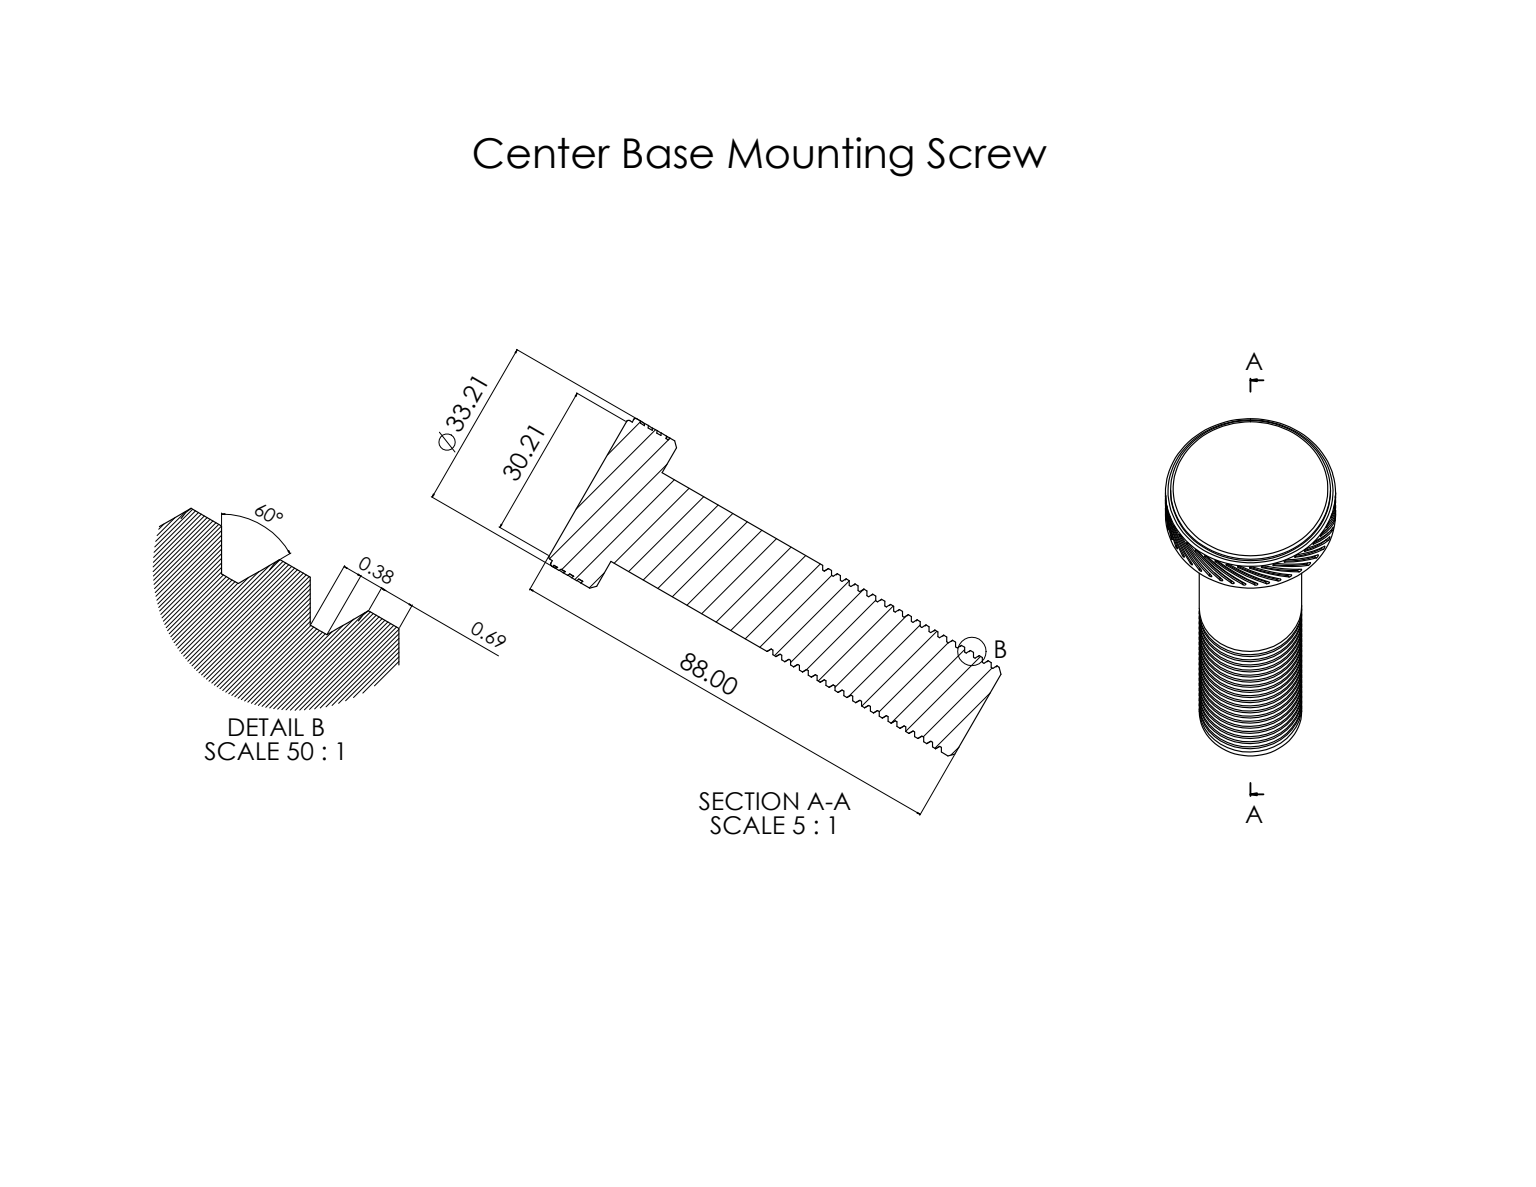
ISO-10303-21;
HEADER;
FILE_DESCRIPTION (('STEP AP214'),
    '1' );
FILE_NAME ('Center Base Mounting Screw.step',
    '2026-10-24T22:31:37',
    ( '' ),
    ( '' ),
    'SwSTEP 2.0',
    'SolidWorks 2025',
    '' );
FILE_SCHEMA (( 'AUTOMOTIVE_DESIGN' ));
ENDSEC;

DATA;
#1=CARTESIAN_POINT ( 'NONE',  ( 23.65144817020273749, 15.78380873178787347, -6.180339887498949025 ) ) ;
#3=DIRECTION ( 'NONE',  ( 0.6270036013472524150, 0.3336146661356817478, 0.7039657224870777830 ) ) ;
#10=CARTESIAN_POINT ( 'NONE',  ( 33.33147356615550194, 41.01751292744059896, 6.180339887498949913 ) ) ;
#11=CARTESIAN_POINT ( 'NONE',  ( 35.05240415091495976, 28.43677371833803846, -10.00000000000000355 ) ) ;
#13=CARTESIAN_POINT ( 'NONE',  ( 72.98662891910291250, 70.81012252529507123, 7.400885746516181030 ) ) ;
#14=CARTESIAN_POINT ( 'NONE',  ( 67.19710446998851694, 67.37600790391256567, -7.293204404656055573 ) ) ;
#18=CARTESIAN_POINT ( 'NONE',  ( 80.56168512721397690, 49.66943426028002762, 14.25699872614796249 ) ) ;
#25=CARTESIAN_POINT ( 'NONE',  ( 78.90549422596571105, 46.47045305960070039, 12.99985401326298984 ) ) ;
#28=CARTESIAN_POINT ( 'NONE',  ( 21.21387930172907588, 35.18080186712593616, 3.090169943749475401 ) ) ;
#37=CARTESIAN_POINT ( 'NONE',  ( 67.11298872355467893, 67.73948000908561085, -6.511686963657441929 ) ) ;
#38=CARTESIAN_POINT ( 'NONE',  ( 73.03670947328784280, 70.42367050102286896, -8.076464510798354368 ) ) ;
#40=CARTESIAN_POINT ( 'NONE',  ( 81.58428055322238492, 41.63658381244528073, 5.723166745212680873 ) ) ;
#45=CARTESIAN_POINT ( 'NONE',  ( 25.22600817569196963, 38.65659080271452552, -1.878358725466461243E-16 ) ) ;
#47=CARTESIAN_POINT ( 'NONE',  ( 87.34642337659644795, 43.20430561321286689, -4.696387144280492735E-07 ) ) ;
#53=CARTESIAN_POINT ( 'NONE',  ( 45.00959873851216031, 26.39040679176986970, 1.333680081654574804E-15 ) ) ;
#54=CARTESIAN_POINT ( 'NONE',  ( 82.57385212973971989, 41.04541115053230982, -1.138833187496899768 ) ) ;
#56=CARTESIAN_POINT ( 'NONE',  ( 66.42592059512334401, 67.89756533557547868, 6.603446877074300225 ) ) ;
#65=CARTESIAN_POINT ( 'NONE',  ( 15.07770630580378501, 30.74646525600389424, 2.839279412974139660 ) ) ;
#67=CARTESIAN_POINT ( 'NONE',  ( 71.88182444303143370, 59.07920979518379312, 15.37605134340125090 ) ) ;
#70=CARTESIAN_POINT ( 'NONE',  ( 4.275827057391709651, 20.65586893147753500, -7.433330006724137462 ) ) ;
#71=CARTESIAN_POINT ( 'NONE',  ( 75.23698744953621542, 53.54332355648684683, -16.05067780448434078 ) ) ;
#72=CARTESIAN_POINT ( 'NONE',  ( 87.14941533941508567, 43.54552546780055877, 0.3078308432578384934 ) ) ;
#77=CARTESIAN_POINT ( 'NONE',  ( 71.49780929996677514, 71.35361720523084728, -4.112299254006656746 ) ) ;
#78=CARTESIAN_POINT ( 'NONE',  ( 76.99791550217098290, 63.80129665876799550, 14.94914524525639266 ) ) ;
#80=ORIENTED_EDGE ( 'NONE', *, *, #23057, .F. ) ;
#86=CARTESIAN_POINT ( 'NONE',  ( 80.05322980421331636, 57.68292478952277946, 16.60179730502024853 ) ) ;
#87=CARTESIAN_POINT ( 'NONE',  ( 66.50947442187053582, 69.16636744153423422, -3.269992574601006119 ) ) ;
#95=ORIENTED_EDGE ( 'NONE', *, *, #9124, .F. ) ;
#98=CARTESIAN_POINT ( 'NONE',  ( 78.41477381124543911, 47.32040575020751305, -14.22103711521623559 ) ) ;
#103=CARTESIAN_POINT ( 'NONE',  ( 83.68415435101742617, 52.28560849428279766, 14.71934805883068975 ) ) ;
#115=CARTESIAN_POINT ( 'NONE',  ( 70.01037705890988150, 67.69997893903554598, 9.246301564518420335 ) ) ;
#119=CARTESIAN_POINT ( 'NONE',  ( 78.58712697892576671, 47.46528512289431490, 14.24466080792137923 ) ) ;
#121=VERTEX_POINT ( 'NONE', #65704 ) ;
#123=CARTESIAN_POINT ( 'NONE',  ( 70.63585127456710211, 66.25873673130102759, 11.15280021666221266 ) ) ;
#124=CARTESIAN_POINT ( 'NONE',  ( 87.74659634842467426, 45.27479573043824246, -7.097702524348068920 ) ) ;
#125=CARTESIAN_POINT ( 'NONE',  ( 79.09597600355056102, 46.01113921700726195, 13.22013416637107674 ) ) ;
#127=CARTESIAN_POINT ( 'NONE',  ( 80.54938030787035075, 54.28115242235315208, -16.20956398890630368 ) ) ;
#129=CARTESIAN_POINT ( 'NONE',  ( 69.87848390701969947, 64.97149032717396722, -11.85179110244203926 ) ) ;
#132=CARTESIAN_POINT ( 'NONE',  ( 72.22030775602182473, 71.51030902015637025, 5.034539909834746751 ) ) ;
#136=CARTESIAN_POINT ( 'NONE',  ( 67.15772368909350121, 67.74692886573922124, -6.548511843863573212 ) ) ;
#140=CARTESIAN_POINT ( 'NONE',  ( 85.75095722755503402, 48.73152497522561788, -11.95392408748539381 ) ) ;
#142=CARTESIAN_POINT ( 'NONE',  ( 70.62071346605948463, 62.04983420565448426, 13.98037766351442457 ) ) ;
#146=CARTESIAN_POINT ( 'NONE',  ( 82.03168081927420019, 41.83908362533459524, -5.586039627916139949 ) ) ;
#150=ORIENTED_EDGE ( 'NONE', *, *, #60128, .F. ) ;
#155=CARTESIAN_POINT ( 'NONE',  ( 17.22757050757671493, 15.11029122506293554, -8.090169943749478065 ) ) ;
#158=DIRECTION ( 'NONE',  ( -0.4755282581475737680, 0.8236391035463299648, -0.3090169943749573878 ) ) ;
#163=CARTESIAN_POINT ( 'NONE',  ( 72.59198933040177337, 57.21847231819964463, 16.35083922987430327 ) ) ;
#165=CARTESIAN_POINT ( 'NONE',  ( 66.48182541455327055, 68.83268692814938561, -4.376997617227660342 ) ) ;
#172=CARTESIAN_POINT ( 'NONE',  ( 30.35763184873497877, 26.03085787977764198, 9.188101187500006262 ) ) ;
#174=EDGE_CURVE ( 'NONE', #25263, #42575, #10857, .T. ) ;
#177=CARTESIAN_POINT ( 'NONE',  ( 68.73278530260755304, 67.96956153877513884, 8.699763636338595063 ) ) ;
#178=CARTESIAN_POINT ( 'NONE',  ( 66.40112479374357690, 68.71345452083818373, 2.354737509933789941 ) ) ;
#183=CARTESIAN_POINT ( 'NONE',  ( 16.06339478488542127, 14.98920272979925272, 7.433330006724137462 ) ) ;
#184=VERTEX_POINT ( 'NONE', #13527 ) ;
#193=ORIENTED_EDGE ( 'NONE', *, *, #79471, .F. ) ;
#196=CARTESIAN_POINT ( 'NONE',  ( 72.70339454587075068, 70.80219159916109106, 7.145408444353458677 ) ) ;
#204=CARTESIAN_POINT ( 'NONE',  ( 69.57540738265171854, 62.56329180587877659, 13.35759117457639533 ) ) ;
#208=CARTESIAN_POINT ( 'NONE',  ( 81.41173721124711449, 42.57291668893481784, -7.675381966840256531 ) ) ;
#218=EDGE_CURVE ( 'NONE', #7931, #29087, #34574, .T. ) ;
#220=CARTESIAN_POINT ( 'NONE',  ( 90.04477061917849312, 44.76220097505219542, 0.000000000000000000 ) ) ;
#224=CARTESIAN_POINT ( 'NONE',  ( 82.66575685400569284, 54.08976349579732812, -15.88644314918171929 ) ) ;
#227=CARTESIAN_POINT ( 'NONE',  ( 11.61360469066603507, 28.74646525600389069, 2.839279412974139660 ) ) ;
#229=CARTESIAN_POINT ( 'NONE',  ( 85.68485941944550177, 48.66523437743575187, 11.91861461389294163 ) ) ;
#238=CARTESIAN_POINT ( 'NONE',  ( 80.58987807051757102, 46.20205379198799989, -12.14270396900382742 ) ) ;
#248=B_SPLINE_CURVE_WITH_KNOTS ( 'NONE', 3,
 ( #65678, #27199, #81432, #4384, #59558, #20106, #51479, #97613, #89544, #13499, #59053, #74319, #21105, #43869, #50975, #81927, #67174, #28181, #12503, #36275, #83920, #90535, #6867, #75301, #21584, #82446, #82923, #43372, #90024, #4902, #51985, #5389, #13010, #98098, #74811, #52469, #20596, #35785, #67678, #29191, #68662, #60058, #44369, #28675, #66678, #13984 ),
 .UNSPECIFIED., .F., .F.,
 ( 4, 1, 1, 1, 2, 2, 1, 1, 1, 2, 2, 1, 1, 2, 2, 1, 1, 2, 2, 1, 1, 2, 2, 1, 2, 2, 1, 2, 2, 4 ),
 ( 0.000000000000000000, 0.06249999999999578115, 0.09374999999999281131, 0.1093749999999927697, 0.1171874999999917982, 0.1249999999999908268, 0.1874999999999810985, 0.2187499999999757694, 0.2343749999999731048, 0.2421874999999721889, 0.2499999999999712730, 0.3124999999999665823, 0.3437499999999636957, 0.3593749999999625855, 0.3749999999999614753, 0.4374999999999584777, 0.4687499999999559241, 0.4843749999999560907, 0.4999999999999562572, 0.5624999999999540368, 0.5937499999999539257, 0.6093749999999549249, 0.6249999999999558131, 0.6874999999999583666, 0.7187499999999606981, 0.7499999999999630296, 0.8124999999999696909, 0.8437499999999743538, 0.8749999999999790168, 1.000000000000000000 ),
 .UNSPECIFIED. ) ;
#258=CARTESIAN_POINT ( 'NONE',  ( 84.80990162342361316, 46.15601649245774496, -9.987538208358218483 ) ) ;
#263=CARTESIAN_POINT ( 'NONE',  ( 74.05204724713870235, 68.33764315531155376, -11.67956189741113349 ) ) ;
#277=DIRECTION ( 'NONE',  ( -0.8660254037844377084, -0.5000000000000015543, -0.000000000000000000 ) ) ;
#278=CARTESIAN_POINT ( 'NONE',  ( 69.28790557221618940, 69.26308972205728764, 6.048929301421852145 ) ) ;
#285=CARTESIAN_POINT ( 'NONE',  ( 17.19404571121151548, 18.43085787977762280, -9.188101187500008038 ) ) ;
#294=CARTESIAN_POINT ( 'NONE',  ( 43.17480782474465428, 33.43085787977766898, -9.188101187500008038 ) ) ;
#296=CARTESIAN_POINT ( 'NONE',  ( 81.30975366074838462, 56.24313983998633404, -16.44754541364716971 ) ) ;
#299=CARTESIAN_POINT ( 'NONE',  ( 33.38390286057418166, 24.98920272979928470, 7.433330006724137462 ) ) ;
#300=DIRECTION ( 'NONE',  ( 0.4145187862775202015, -0.7179675985244525771, -0.5591929034707450175 ) ) ;
#301=CARTESIAN_POINT ( 'NONE',  ( 81.38004395914478550, 48.63429429711172247, 14.01118663915790030 ) ) ;
#307=CARTESIAN_POINT ( 'NONE',  ( 84.83590989842353736, 50.19589791021755332, -13.76099895038702847 ) ) ;
#308=CARTESIAN_POINT ( 'NONE',  ( 75.63268008801900066, 65.14737934564519151, -14.41129995628930516 ) ) ;
#310=CARTESIAN_POINT ( 'NONE',  ( 73.99515186948657686, 54.97541550358009488, -16.60506967685200408 ) ) ;
#313=CARTESIAN_POINT ( 'NONE',  ( 73.43248428410468875, 69.89844921070914552, 9.717079046730820124 ) ) ;
#314=CARTESIAN_POINT ( 'NONE',  ( 38.69312636016019269, 30.84335787977765619, 9.188101187500006262 ) ) ;
#315=VERTEX_POINT ( 'NONE', #76800 ) ;
#319=ORIENTED_EDGE ( 'NONE', *, *, #9183, .T. ) ;
#320=CARTESIAN_POINT ( 'NONE',  ( 86.52915347386752387, 47.38364953835303339, -10.30352551399626648 ) ) ;
#324=CARTESIAN_POINT ( 'NONE',  ( 41.44395331530407844, 35.87878583063845639, -9.188101187500006262 ) ) ;
#325=CARTESIAN_POINT ( 'NONE',  ( 80.05943320740847469, 44.70013682444275815, 11.13689609985222617 ) ) ;
#329=VERTEX_POINT ( 'NONE', #37789 ) ;
#330=CARTESIAN_POINT ( 'NONE',  ( 81.35074466249913883, 55.80872010294902452, 16.38725056492407361 ) ) ;
#335=DIRECTION ( 'NONE',  ( -0.5000000000000015543, 0.8660254037844378194, 0.000000000000000000 ) ) ;
#336=CARTESIAN_POINT ( 'NONE',  ( 35.42939366167109938, 22.58380873178788306, 6.180339887498953466 ) ) ;
#339=CARTESIAN_POINT ( 'NONE',  ( 82.56576626489119519, 41.03778865018932720, 1.100605105531167416 ) ) ;
#342=EDGE_CURVE ( 'NONE', #62365, #23265, #62078, .T. ) ;
#347=CARTESIAN_POINT ( 'NONE',  ( 70.49910835669693654, 60.86989013130169468, -15.00567599565220434 ) ) ;
#348=CARTESIAN_POINT ( 'NONE',  ( 41.71939737199939202, 29.80170272979930246, 7.433330006724137462 ) ) ;
#351=EDGE_CURVE ( 'NONE', #45858, #78719, #48667, .T. ) ;
#358=CARTESIAN_POINT ( 'NONE',  ( 72.39980299547302423, 63.20348272691148139, 13.94953712136970836 ) ) ;
#361=ORIENTED_EDGE ( 'NONE', *, *, #84758, .T. ) ;
#374=CARTESIAN_POINT ( 'NONE',  ( 70.01283242295177445, 62.80173547756309915, -13.36538303052352816 ) ) ;
#378=CARTESIAN_POINT ( 'NONE',  ( 72.32867159652951727, 65.47220889536410482, 12.56686077310279082 ) ) ;
#385=CARTESIAN_POINT ( 'NONE',  ( 23.13271821863878230, 13.75978393459164195, -1.583844403245362020 ) ) ;
#388=CARTESIAN_POINT ( 'NONE',  ( 82.68215287466908592, 53.55713939286302150, -15.73562046651999502 ) ) ;
#396=CARTESIAN_POINT ( 'NONE',  ( 84.87359499838788679, 50.02211777990267194, -13.22747082306951327 ) ) ;
#398=CARTESIAN_POINT ( 'NONE',  ( 73.56775416758397057, 69.23451306489744184, -10.00871374113025070 ) ) ;
#399=CARTESIAN_POINT ( 'NONE',  ( 75.97293632993350343, 51.42040260576536781, 16.16535879681820731 ) ) ;
#409=CARTESIAN_POINT ( 'NONE',  ( 75.75493378409400691, 65.86437009324525604, -14.07593894684414693 ) ) ;
#410=EDGE_CURVE ( 'NONE', #10093, #75363, #77822, .T. ) ;
#413=CARTESIAN_POINT ( 'NONE',  ( 66.36268096397610350, 69.44190093015801324, 9.875986171954755521E-07 ) ) ;
#415=CARTESIAN_POINT ( 'NONE',  ( 27.04628097738780212, 27.56628583063842086, 9.188101187500006262 ) ) ;
#417=CARTESIAN_POINT ( 'NONE',  ( 81.38192374540615504, 47.39962897157295885, -12.69884445555879360 ) ) ;
#418=CARTESIAN_POINT ( 'NONE',  ( 11.61057445305848823, 22.10171378149917842, 9.188101187500008038 ) ) ;
#420=CARTESIAN_POINT ( 'NONE',  ( 77.30463285345523161, 63.36080703450485174, 15.53535672671000079 ) ) ;
#423=CARTESIAN_POINT ( 'NONE',  ( 67.41248320326423027, 66.37693208286884783, -8.946798147498746800 ) ) ;
#428=CARTESIAN_POINT ( 'NONE',  ( 80.28226457095783530, 55.01127608260450330, -15.95866588083628557 ) ) ;
#434=CARTESIAN_POINT ( 'NONE',  ( 82.50452235219570696, 53.86480448276186905, 15.85105177732747173 ) ) ;
#435=ORIENTED_EDGE ( 'NONE', *, *, #30362, .T. ) ;
#444=CARTESIAN_POINT ( 'NONE',  ( 82.09009853944208146, 44.85671956714123354, 10.87987463625776741 ) ) ;
#447=CARTESIAN_POINT ( 'NONE',  ( 23.73796034364816521, 35.74646525600390845, 2.839279412974139660 ) ) ;
#448=CARTESIAN_POINT ( 'NONE',  ( 79.97518497192163522, 44.56399469350409959, 11.74208085782137267 ) ) ;
#450=CARTESIAN_POINT ( 'NONE',  ( 75.08013308270209052, 67.09339902234967212, -13.09435070823463043 ) ) ;
#452=ORIENTED_EDGE ( 'NONE', *, *, #76491, .T. ) ;
#459=FACE_OUTER_BOUND ( 'NONE', #67397, .T. ) ;
#475=CARTESIAN_POINT ( 'NONE',  ( 67.16327201103491973, 67.73731889023997610, 6.573435314091265802 ) ) ;
#479=CARTESIAN_POINT ( 'NONE',  ( 81.11670802570714045, 56.15934143863493944, 16.10866441373284630 ) ) ;
#486=CARTESIAN_POINT ( 'NONE',  ( 82.41630873631589793, 41.31828431233920895, -3.367117793111288560 ) ) ;
#488=EDGE_LOOP ( 'NONE', ( #46553, #54812, #94039, #23503 ) ) ;
#489=CARTESIAN_POINT ( 'NONE',  ( 76.44840390471171077, 51.64438224287277279, -16.15499642960158155 ) ) ;
#497=CARTESIAN_POINT ( 'NONE',  ( 82.82785115793576836, 43.65967190867092285, -8.128949345812960914 ) ) ;
#500=CARTESIAN_POINT ( 'NONE',  ( 72.42095758685501039, 70.73706075180957953, 7.727740079816340035 ) ) ;
#501=CARTESIAN_POINT ( 'NONE',  ( 69.17735699518412673, 67.42632015883337715, -8.956856073786124028 ) ) ;
#502=ORIENTED_EDGE ( 'NONE', *, *, #85667, .F. ) ;
#508=EDGE_CURVE ( 'NONE', #53392, #59506, #69113, .T. ) ;
#516=FACE_BOUND ( 'NONE', #48775, .T. ) ;
#519=CARTESIAN_POINT ( 'NONE',  ( 32.89180500207565672, 24.15404122711135670, 8.090169943749479842 ) ) ;
#529=CARTESIAN_POINT ( 'NONE',  ( 13.40335115377346753, 31.23654200823201776, 1.583844403245363353 ) ) ;
#530=CARTESIAN_POINT ( 'NONE',  ( 81.82787295522399518, 41.24789425966510947, 5.851439987416612531 ) ) ;
#532=CARTESIAN_POINT ( 'NONE',  ( 22.06360519161784595, 36.23654200823203553, 1.583844403245363353 ) ) ;
#533=CARTESIAN_POINT ( 'NONE',  ( 30.89548221274965556, 26.03677371833803633, 10.00000000000000533 ) ) ;
#534=CARTESIAN_POINT ( 'NONE',  ( 86.35121876318000034, 43.08468197994678661, 0.3078304325362931637 ) ) ;
#538=CARTESIAN_POINT ( 'NONE',  ( 87.18439463908147502, 46.15779724344488244, -8.329569831597547491 ) ) ;
#544=CARTESIAN_POINT ( 'NONE',  ( 72.32117545662791258, 66.44659970230358681, -11.84374507886356831 ) ) ;
#548=CARTESIAN_POINT ( 'NONE',  ( 66.29454943693275482, 69.24199052626691753, -2.144636311159408226 ) ) ;
#552=LINE ( 'NONE', #17762, #100067 ) ;
#557=CARTESIAN_POINT ( 'NONE',  ( 19.25324864145614612, 26.51421378149919761, -9.188101187500004485 ) ) ;
#563=CARTESIAN_POINT ( 'NONE',  ( 7.601631632957885465, 27.49540643055185285, 3.479690158560446702E-15 ) ) ;
#564=DIRECTION ( 'NONE',  ( -0.4996954135095461047, 0.8654978445076770832, -0.03489949670251103753 ) ) ;
#568=CARTESIAN_POINT ( 'NONE',  ( 72.40022343535652283, 71.86297034063233014, -5.456689119915505870 ) ) ;
#571=ORIENTED_EDGE ( 'NONE', *, *, #75290, .T. ) ;
#572=ORIENTED_EDGE ( 'NONE', *, *, #79852, .F. ) ;
#574=CARTESIAN_POINT ( 'NONE',  ( 83.55937078812219454, 42.48588548430609535, -5.103737020810437564 ) ) ;
#577=PLANE ( 'NONE',  #1141 ) ;
#578=CARTESIAN_POINT ( 'NONE',  ( 72.73633344227268083, 57.02636325111804183, -16.39140812357083021 ) ) ;
#579=CARTESIAN_POINT ( 'NONE',  ( 76.64464310018406934, 63.53199411942404851, 15.34601863127964627 ) ) ;
#586=CARTESIAN_POINT ( 'NONE',  ( 26.72152145096863762, 27.37878583063842086, 9.188101187500006262 ) ) ;
#588=CARTESIAN_POINT ( 'NONE',  ( 78.31654463311403447, 47.36115395161638020, -14.27160036167827784 ) ) ;
#593=CARTESIAN_POINT ( 'NONE',  ( 83.35161352719694605, 52.40881748729520240, 14.85180384881482674 ) ) ;
#595=EDGE_LOOP ( 'NONE', ( #20192, #17699, #51168, #51804 ) ) ;
#596=CARTESIAN_POINT ( 'NONE',  ( 86.83016860379825630, 46.47919197584165119, 9.056981041330921300 ) ) ;
#597=CARTESIAN_POINT ( 'NONE',  ( 81.64670023727850889, 42.65128533460878657, -7.584980231169042852 ) ) ;
#601=ORIENTED_EDGE ( 'NONE', *, *, #47729, .T. ) ;
#608=ADVANCED_FACE ( 'NONE', ( #98877 ), #22352, .T. ) ;
#609=CARTESIAN_POINT ( 'NONE',  ( 69.00186724958503248, 65.47144582019447512, 10.96851354096545883 ) ) ;
#611=CARTESIAN_POINT ( 'NONE',  ( 67.43691672556117567, 66.98928061623196584, 9.017019808546432813 ) ) ;
#612=CARTESIAN_POINT ( 'NONE',  ( 70.21952773771840839, 65.49792867059230161, -11.57245437907510244 ) ) ;
#613=CARTESIAN_POINT ( 'NONE',  ( 78.41127520731549794, 47.42400182521100049, 14.27580055608907017 ) ) ;
#617=CARTESIAN_POINT ( 'NONE',  ( 69.93192355902827728, 64.35613849418326993, 12.34049615428977198 ) ) ;
#620=B_SPLINE_CURVE_WITH_KNOTS ( 'NONE', 3,
 ( #66257, #11575, #42433, #82510, #73367, #65740, #96694, #4966, #27759, #58631, #27263, #89605, #41953, #96197, #74384, #34355, #51036, #26758, #35849, #58146, #19678, #72382, #66742, #59118, #90091, #95716, #64767, #20659, #51548, #2992, #33882 ),
 .UNSPECIFIED., .F., .F.,
 ( 4, 3, 3, 3, 3, 3, 3, 3, 3, 3, 4 ),
 ( 0.000000000000000000, 0.1333490885032305451, 0.3007194338854253246, 0.4699862290244986029, 0.5844252810809236198, 0.6686540514502520294, 0.7354980260655306079, 0.8028463152565280536, 0.8633854507756927310, 0.9437142632666988273, 1.000000000000000000 ),
 .UNSPECIFIED. ) ;
#622=CARTESIAN_POINT ( 'NONE',  ( 83.88626965845651284, 51.63168102053428754, -14.39363241527635751 ) ) ;
#626=CARTESIAN_POINT ( 'NONE',  ( 72.54208641595317886, 71.58009272687419866, 5.313622202418648577 ) ) ;
#631=DIRECTION ( 'NONE',  ( -0.2347357813929480952, 0.4065742997269687908, 0.8829475928589233247 ) ) ;
#633=CARTESIAN_POINT ( 'NONE',  ( 83.18659939620825128, 40.82302332894202124, -0.8845490628100145525 ) ) ;
#636=CARTESIAN_POINT ( 'NONE',  ( 85.65412827366334625, 48.89905674914069067, -12.59087409094112253 ) ) ;
#638=DIRECTION ( 'NONE',  ( -0.2347357813929480952, 0.4065742997269687908, 0.8829475928589233247 ) ) ;
#646=CARTESIAN_POINT ( 'NONE',  ( 45.03145032967896100, 28.12755873383629890, -6.180339887498949025 ) ) ;
#649=CARTESIAN_POINT ( 'NONE',  ( 88.00349997577261263, 44.64923112938743088, 4.253506518527973235 ) ) ;
#651=CARTESIAN_POINT ( 'NONE',  ( 10.05297690690921897, 28.73705186507752529, -3.090169943749475845 ) ) ;
#653=CARTESIAN_POINT ( 'NONE',  ( 71.82703346931063493, 59.57451500028311386, -15.72875088550162914 ) ) ;
#658=CARTESIAN_POINT ( 'NONE',  ( 73.05975105895772970, 57.25024586824646633, 15.90232548103993615 ) ) ;
#660=CARTESIAN_POINT ( 'NONE',  ( 10.55946980724658069, 24.83478043621386888, -8.090169943749479842 ) ) ;
#662=AXIS2_PLACEMENT_3D ( 'NONE', #54067, #69781, #39856 ) ;
#667=CARTESIAN_POINT ( 'NONE',  ( 31.05045217176252237, 26.43085787977764767, -9.188101187500008038 ) ) ;
#670=EDGE_CURVE ( 'NONE', #48310, #39764, #20859, .T. ) ;
#675=CARTESIAN_POINT ( 'NONE',  ( 66.15645594251088824, 68.58591844969842555, 2.277906049505277863 ) ) ;
#681=CARTESIAN_POINT ( 'NONE',  ( 12.59929316974766955, 12.98920272979924739, 7.433330006724137462 ) ) ;
#685=CARTESIAN_POINT ( 'NONE',  ( 28.31825578742223115, 28.30066082961423390, -10.00000000000000533 ) ) ;
#692=FACE_OUTER_BOUND ( 'NONE', #1772, .T. ) ;
#693=ORIENTED_EDGE ( 'NONE', *, *, #11844, .T. ) ;
#698=CARTESIAN_POINT ( 'NONE',  ( 79.11723855630624769, 59.11194703662723526, -16.21433712332713739 ) ) ;
#700=CARTESIAN_POINT ( 'NONE',  ( 69.78994883848024244, 62.55969527080727488, 13.43020027970054819 ) ) ;
#708=CARTESIAN_POINT ( 'NONE',  ( 73.41033574890859370, 61.45318865418844467, 14.95304618059455670 ) ) ;
#718=CARTESIAN_POINT ( 'NONE',  ( 73.00396795756827828, 57.62093675928252878, -16.32480838619500219 ) ) ;
#719=CARTESIAN_POINT ( 'NONE',  ( 15.13723537722347778, 17.24335787977762280, -9.188101187500008038 ) ) ;
#722=CARTESIAN_POINT ( 'NONE',  ( 68.45344762042827824, 64.57392882346940155, 12.12708197196866600 ) ) ;
#729=CARTESIAN_POINT ( 'NONE',  ( 82.52967124556970191, 45.91001068904856197, -10.98309457076566886 ) ) ;
#733=DIRECTION ( 'NONE',  ( -0.8660254037844377084, -0.5000000000000014433, -0.000000000000000000 ) ) ;
#740=CARTESIAN_POINT ( 'NONE',  ( 82.39535249337586720, 40.37214158351728344, -0.8705103534316617209 ) ) ;
#743=CARTESIAN_POINT ( 'NONE',  ( 72.53309028193872621, 70.86290320417140265, 7.626211012637800657 ) ) ;
#745=CARTESIAN_POINT ( 'NONE',  ( 75.62238463899576857, 65.35737373615053514, 14.30258955018443956 ) ) ;
#747=ORIENTED_EDGE ( 'NONE', *, *, #72238, .F. ) ;
#749=VERTEX_POINT ( 'NONE', #78569 ) ;
#752=CARTESIAN_POINT ( 'NONE',  ( 85.52120238093419857, 46.04363271907506316, -9.405378037663709279 ) ) ;
#756=CARTESIAN_POINT ( 'NONE',  ( 74.45862791283336435, 68.29041308412308808, -11.43317454991487914 ) ) ;
#762=CARTESIAN_POINT ( 'NONE',  ( 30.11635425815369871, 39.16126292948897714, -6.180339887498951690 ) ) ;
#763=CARTESIAN_POINT ( 'NONE',  ( 80.25178558894602077, 57.14685393251872370, -16.23521980932009612 ) ) ;
#768=ADVANCED_FACE ( 'NONE', ( #79091 ), #73419, .T. ) ;
#774=DIRECTION ( 'NONE',  ( 0.000000000000000000, -0.5247752241694974007, 0.8512408378936325848 ) ) ;
#779=CARTESIAN_POINT ( 'NONE',  ( 10.91775413003093931, 21.70171378149917985, -9.188101187500004485 ) ) ;
#783=CARTESIAN_POINT ( 'NONE',  ( 66.10780414051450293, 68.63670250712272036, 1.777645618418523865 ) ) ;
#790=CARTESIAN_POINT ( 'NONE',  ( 85.94615330653621754, 47.59945275330427705, 10.87303975713271420 ) ) ;
#791=ORIENTED_EDGE ( 'NONE', *, *, #48139, .T. ) ;
#798=CARTESIAN_POINT ( 'NONE',  ( 84.41462708798377435, 43.37824213815624574, 7.154511429969321767 ) ) ;
#801=CARTESIAN_POINT ( 'NONE',  ( 72.40747426417379984, 71.81324781307232286, -5.589457107701495175 ) ) ;
#803=ORIENTED_EDGE ( 'NONE', *, *, #92983, .T. ) ;
#806=CARTESIAN_POINT ( 'NONE',  ( 41.82943821127123840, 26.01110640527295814, 2.839279412974134775 ) ) ;
#813=EDGE_LOOP ( 'NONE', ( #50961, #70079, #41428, #11684 ) ) ;
#814=CARTESIAN_POINT ( 'NONE',  ( 86.28449982416978514, 46.95005333036156969, -10.54182221192813884 ) ) ;
#816=B_SPLINE_CURVE_WITH_KNOTS ( 'NONE', 3,
 ( #20818, #38347, #96847, #7455, #100186, #69257, #36485, #58292, #57789, #43591, #88767, #82657, #28907, #43073, #13216, #19337 ),
 .UNSPECIFIED., .F., .F.,
 ( 4, 1, 2, 2, 2, 1, 2, 2, 4 ),
 ( 0.000000000000000000, 0.1249999999999972522, 0.1874999999999962530, 0.2499999999999952816, 0.4999999999999940048, 0.6249999999999944489, 0.6874999999999946709, 0.7499999999999947820, 1.000000000000000000 ),
 .UNSPECIFIED. ) ;
#819=CARTESIAN_POINT ( 'NONE',  ( 18.33840876668534037, 32.36126292948895866, 6.180339887498949913 ) ) ;
#822=CARTESIAN_POINT ( 'NONE',  ( 81.63517289312954972, 55.69097578121159131, -16.34528168754146904 ) ) ;
#826=VERTEX_POINT ( 'NONE', #48664 ) ;
#827=CARTESIAN_POINT ( 'NONE',  ( 77.13172709529845861, 49.47536214534034826, -14.94599358421776358 ) ) ;
#831=DIRECTION ( 'NONE',  ( -0.8660254037844378194, -0.5000000000000014433, -0.000000000000000000 ) ) ;
#832=CARTESIAN_POINT ( 'NONE',  ( 36.01802474176511026, 21.76426979415091978, 3.090169943749476733 ) ) ;
#833=CARTESIAN_POINT ( 'NONE',  ( 71.17767548612019368, 71.91738291818995776, 3.016136621268855844 ) ) ;
#840=CARTESIAN_POINT ( 'NONE',  ( 70.47294781783818962, 60.89548864084860469, -14.98891872237399348 ) ) ;
#841=CARTESIAN_POINT ( 'NONE',  ( 42.37730965384162829, 25.26216523072498532, -2.296566073217252530E-15 ) ) ;
#844=ADVANCED_FACE ( 'NONE', ( #61833 ), #9674, .T. ) ;
#845=CARTESIAN_POINT ( 'NONE',  ( 20.28716687417668751, 35.21091486745861232, 7.012934429366973338E-14 ) ) ;
#849=EDGE_CURVE ( 'NONE', #75378, #62754, #4045, .T. ) ;
#852=CARTESIAN_POINT ( 'NONE',  ( 71.63285926872011089, 60.29674625202430605, 14.96834098354499965 ) ) ;
#856=CARTESIAN_POINT ( 'NONE',  ( 76.73342198214220389, 54.11205231684652972, -16.50410611215824375 ) ) ;
#866=CYLINDRICAL_SURFACE ( 'NONE', #55855, 10.00000000000001066 ) ;
#883=CARTESIAN_POINT ( 'NONE',  ( 73.85662887421025857, 68.53912330967601463, 10.89787362795912884 ) ) ;
#892=CARTESIAN_POINT ( 'NONE',  ( 78.12422403393351544, 55.30668070268215075, 16.12263249026505108 ) ) ;
#896=B_SPLINE_CURVE_WITH_KNOTS ( 'NONE', 3,
 ( #59007, #89974, #13454, #81389, #49945, #20554, #82879, #57531, #35237, #51432, #12964, #43825, #5343, #36224, #19070, #67128, #59512, #90490, #21063, #37224, #7320, #38712, #91978, #13933, #99050, #14437, #61996, #23008, #75749, #53903, #38199, #68619, #99542, #68122, #14914, #21539, #36721, #5831, #45318, #45802, #69118, #100045, #76726, #23501, #52422, #69618 ),
 .UNSPECIFIED., .F., .F.,
 ( 4, 1, 2, 2, 1, 2, 2, 1, 1, 2, 2, 1, 1, 2, 2, 1, 1, 2, 2, 1, 1, 1, 2, 2, 1, 1, 1, 2, 2, 4 ),
 ( 0.000000000000000000, 0.06249999999999382438, 0.09374999999999200639, 0.1249999999999902023, 0.1874999999999839295, 0.2187499999999821532, 0.2499999999999804046, 0.3124999999999763522, 0.3437499999999758526, 0.3593749999999756306, 0.3749999999999754086, 0.4374999999999745759, 0.4687499999999757971, 0.4843749999999780731, 0.4999999999999803491, 0.5624999999999793499, 0.5937499999999791278, 0.6093749999999773515, 0.6249999999999755751, 0.6874999999999715783, 0.7187499999999709122, 0.7343749999999705791, 0.7421874999999703570, 0.7499999999999701350, 0.8124999999999732436, 0.8437499999999734657, 0.8593749999999736877, 0.8671874999999749090, 0.8749999999999761302, 1.000000000000000000 ),
 .UNSPECIFIED. ) ;
#897=CARTESIAN_POINT ( 'NONE',  ( 76.39060622948801438, 51.12702130622679420, 16.04935315526039474 ) ) ;
#904=CARTESIAN_POINT ( 'NONE',  ( 72.71381692756899895, 57.00322135356037023, -15.91178980316282043 ) ) ;
#905=EDGE_CURVE ( 'NONE', #18632, #67404, #6039, .T. ) ;
#909=CARTESIAN_POINT ( 'NONE',  ( 88.13330906385691321, 44.06097395418934326, 0.5526411241947467579 ) ) ;
#914=CARTESIAN_POINT ( 'NONE',  ( 77.22785773251615637, 49.24952049019824329, 15.36076451811752719 ) ) ;
#918=CARTESIAN_POINT ( 'NONE',  ( 33.49394369984602804, 21.19860640527294038, 2.839279412974134775 ) ) ;
#921=CARTESIAN_POINT ( 'NONE',  ( 17.79544559245429625, 15.98920272979925628, 7.433330006724137462 ) ) ;
#923=CARTESIAN_POINT ( 'NONE',  ( 76.72890798614155017, 63.86846200969244336, 14.87016573101661265 ) ) ;
#930=CARTESIAN_POINT ( 'NONE',  ( 79.71580056254293822, 55.22957162338799009, -16.02820282535946106 ) ) ;
#935=CARTESIAN_POINT ( 'NONE',  ( 77.14514041473603356, 49.33218330559527942, 15.40661048312039583 ) ) ;
#937=ORIENTED_EDGE ( 'NONE', *, *, #80216, .F. ) ;
#940=CARTESIAN_POINT ( 'NONE',  ( 70.23258906160542381, 68.89773635095485815, -7.744023681228862976 ) ) ;
#944=CARTESIAN_POINT ( 'NONE',  ( 79.57426776858704898, 46.24084366563779724, -13.18946159609117252 ) ) ;
#948=CARTESIAN_POINT ( 'NONE',  ( 33.34238925418374322, 21.11110640527294180, -2.839279412974138328 ) ) ;
#950=CARTESIAN_POINT ( 'NONE',  ( 80.01036472522686438, 44.36946922474368904, 11.55303063996890245 ) ) ;
#952=CARTESIAN_POINT ( 'NONE',  ( 75.00927956955034404, 66.36452684332685692, -13.11830550837433229 ) ) ;
#954=DIRECTION ( 'NONE',  ( -0.8845109580947964067, 0.1124011590738280275, 0.4527762631246092795 ) ) ;
#960=CARTESIAN_POINT ( 'NONE',  ( 67.96729249982780630, 66.07064282809847100, -10.47701906205939792 ) ) ;
#963=CARTESIAN_POINT ( 'NONE',  ( 32.41152252715882298, 42.21091486745863364, 7.012934429366973338E-14 ) ) ;
#969=EDGE_LOOP ( 'NONE', ( #9920, #90585, #63476, #91922 ) ) ;
#971=CARTESIAN_POINT ( 'NONE',  ( 77.91510949599519620, 62.18724900762369856, -15.97225761198294691 ) ) ;
#976=CARTESIAN_POINT ( 'NONE',  ( 79.89934654500854094, 44.60194503138297506, -11.13433824245048953 ) ) ;
#977=CARTESIAN_POINT ( 'NONE',  ( 66.62422707585170656, 67.62317984664836956, 6.187721633850552294 ) ) ;
#980=CARTESIAN_POINT ( 'NONE',  ( 83.22635668477047943, 47.66699298699816723, -12.18745831367220944 ) ) ;
#994=CARTESIAN_POINT ( 'NONE',  ( 88.25642124133898392, 44.32248799199468436, 4.097629997315074490 ) ) ;
#995=B_SPLINE_CURVE_WITH_KNOTS ( 'NONE', 3,
 ( #93557, #16517, #56515, #15503, #64120, #95070, #66486, #75593, #82240, #36571, #12816, #89829, #28998, #37076, #6178, #35591, #2850, #41302, #36075, #18038, #21388, #28478, #5193, #20405, #10938, #51799, #26130, #74107, #58860, #10430, #27981 ),
 .UNSPECIFIED., .F., .F.,
 ( 4, 3, 3, 3, 3, 3, 3, 3, 3, 3, 4 ),
 ( 0.000000000000000000, 0.1333490885032329043, 0.3007194338854308202, 0.4699862290245099827, 0.5844252810809248411, 0.6686540514502534727, 0.7354980260655189506, 0.8028463152565233907, 0.8633854507756654195, 0.9437142632666670750, 1.000000000000000000 ),
 .UNSPECIFIED. ) ;
#997=CARTESIAN_POINT ( 'NONE',  ( 81.50097959531993297, 43.67013008731806423, -9.164372295790522926 ) ) ;
#999=CARTESIAN_POINT ( 'NONE',  ( 36.28012939083434674, 26.11029122506296929, -8.090169943749478065 ) ) ;
#1003=CARTESIAN_POINT ( 'NONE',  ( 72.48280754011683769, 70.60311863597819126, 7.264376673680512653 ) ) ;
#1006=ORIENTED_EDGE ( 'NONE', *, *, #90756, .F. ) ;
#1009=CARTESIAN_POINT ( 'NONE',  ( 87.56313949369642557, 43.39506783062379469, 1.585011492977574488 ) ) ;
#1011=CARTESIAN_POINT ( 'NONE',  ( 83.81044542681900111, 52.09240911291835374, 14.60277729873947905 ) ) ;
#1018=FACE_BOUND ( 'NONE', #32836, .T. ) ;
#1020=CARTESIAN_POINT ( 'NONE',  ( 25.82140064434168636, 39.00034080476291365, -1.878358725466461243E-16 ) ) ;
#1033=CARTESIAN_POINT ( 'NONE',  ( 19.02883662497902861, 11.39040679176981996, 1.333680081654574804E-15 ) ) ;
#1037=CARTESIAN_POINT ( 'NONE',  ( 35.42939366167109938, 22.58380873178788306, 6.180339887498953466 ) ) ;
#1046=CARTESIAN_POINT ( 'NONE',  ( 73.36681650135379584, 66.22633458900254766, -12.49190051511774868 ) ) ;
#1047=B_SPLINE_CURVE_WITH_KNOTS ( 'NONE', 3,
 ( #4963, #35344, #52530, #58627, #50535, #97673, #89601, #44432, #35845, #21165 ),
 .UNSPECIFIED., .F., .F.,
 ( 4, 2, 2, 2, 4 ),
 ( 0.000000000000000000, 0.2499999999999983347, 0.4999999999999988898, 0.7499999999999994449, 1.000000000000000000 ),
 .UNSPECIFIED. ) ;
#1050=CARTESIAN_POINT ( 'NONE',  ( 72.74024025722111730, 70.77703717069299216, -7.960999691682594914 ) ) ;
#1058=CARTESIAN_POINT ( 'NONE',  ( 17.99393647837114329, 33.49540643055186706, 3.479690158560446702E-15 ) ) ;
#1065=CARTESIAN_POINT ( 'NONE',  ( 7.128892988474023085, 19.51421378149916563, -9.188101187500004485 ) ) ;
#1066=CARTESIAN_POINT ( 'NONE',  ( 88.24246443646677562, 44.29974554292944333, 4.047255302186846926 ) ) ;
#1067=CARTESIAN_POINT ( 'NONE',  ( 77.56650176279948994, 58.32259081542915879, -16.15928628467516859 ) ) ;
#1068=CARTESIAN_POINT ( 'NONE',  ( 87.95476553115707929, 44.23128429206734324, 2.820676398910382243 ) ) ;
#1069=ORIENTED_EDGE ( 'NONE', *, *, #50508, .F. ) ;
#1072=CARTESIAN_POINT ( 'NONE',  ( 72.37415438388894984, 71.90064624941815907, -5.324036893254605829 ) ) ;
#1074=CARTESIAN_POINT ( 'NONE',  ( 85.24521657786070250, 49.07911862026776362, 12.45208212324389763 ) ) ;
#1075=CARTESIAN_POINT ( 'NONE',  ( 84.13220800937075694, 41.60931624182121169, 2.733980135768734332 ) ) ;
#1079=CARTESIAN_POINT ( 'NONE',  ( 84.04471568993460551, 42.57412079040409481, -4.602180766856474037 ) ) ;
#1082=CARTESIAN_POINT ( 'NONE',  ( 72.09683433654826956, 72.38845567423071259, -3.220643376046866901 ) ) ;
#1084=CARTESIAN_POINT ( 'NONE',  ( 77.31919379202844311, 63.29706486701976331, 15.55867855103717545 ) ) ;
#1090=FACE_OUTER_BOUND ( 'NONE', #73993, .T. ) ;
#1094=CARTESIAN_POINT ( 'NONE',  ( 23.19008890107777177, 36.49540643055188838, 3.479690158560446702E-15 ) ) ;
#1099=CARTESIAN_POINT ( 'NONE',  ( 74.17419530692131957, 68.61376803465689989, 10.99684454571890591 ) ) ;
#1100=CARTESIAN_POINT ( 'NONE',  ( 82.15463706511577868, 40.84277258114416043, 1.595534587534165549 ) ) ;
#1104=CARTESIAN_POINT ( 'NONE',  ( 86.89671376885311815, 46.48613028513706524, 9.014139361656079430 ) ) ;
#1105=CARTESIAN_POINT ( 'NONE',  ( 85.23557152020472927, 43.11680246062262256, -4.179448767779550877 ) ) ;
#1115=CARTESIAN_POINT ( 'NONE',  ( 84.39378192592442929, 42.61420722820205498, -5.616381072414180942 ) ) ;
#1116=CARTESIAN_POINT ( 'NONE',  ( 67.53167658288728603, 67.09922345405099975, 8.942594108729585045 ) ) ;
#1117=CARTESIAN_POINT ( 'NONE',  ( 74.55495018319990663, 64.55344886072012400, -13.93350266944992555 ) ) ;
#1118=CARTESIAN_POINT ( 'NONE',  ( 78.05253372616796526, 47.80071866568432171, 14.02011486286742858 ) ) ;
#1128=CARTESIAN_POINT ( 'NONE',  ( 76.04961876167374157, 51.28812058955301723, -15.63847478383918421 ) ) ;
#1130=PLANE ( 'NONE',  #21880 ) ;
#1131=CARTESIAN_POINT ( 'NONE',  ( 71.96379157542388327, 72.26892066703038608, 0.6295764574549533865 ) ) ;
#1132=CARTESIAN_POINT ( 'NONE',  ( 72.04811769650319775, 71.35602353065117143, 5.168332083721276504 ) ) ;
#1137=B_SPLINE_CURVE_WITH_KNOTS ( 'NONE', 3,
 ( #78716, #23991, #63498, #54889, #85870, #16396, #88363, #18922, #65993, #11329 ),
 .UNSPECIFIED., .F., .F.,
 ( 4, 2, 2, 2, 4 ),
 ( 0.000000000000000000, 0.2500000000000000000, 0.5000000000000000000, 0.7500000000000000000, 1.000000000000000000 ),
 .UNSPECIFIED. ) ;
#1139=CARTESIAN_POINT ( 'NONE',  ( 83.55337146356914957, 41.01436309113273637, -0.4425042433306793921 ) ) ;
#1141=AXIS2_PLACEMENT_3D ( 'NONE', #13781, #6180, #37077 ) ;
#1142=CARTESIAN_POINT ( 'NONE',  ( 78.56356803705116931, 59.62236819939711552, -16.48917668510493684 ) ) ;
#1147=CARTESIAN_POINT ( 'NONE',  ( 67.71395807953069834, 69.70288697866548944, -0.3208651280214164792 ) ) ;
#1160=CARTESIAN_POINT ( 'NONE',  ( 18.95962131514559346, 16.11029122506294087, -8.090169943749478065 ) ) ;
#1163=CARTESIAN_POINT ( 'NONE',  ( 72.12578029244804156, 72.07013754146423423, 2.921549647394216631 ) ) ;
#1164=CARTESIAN_POINT ( 'NONE',  ( 2.161320418471442739, 24.18080186712590418, 3.090169943749475401 ) ) ;
#1169=CARTESIAN_POINT ( 'NONE',  ( 66.51865997380296847, 68.29495818825724029, -4.336921469600853563 ) ) ;
#1177=CARTESIAN_POINT ( 'NONE',  ( 27.72828276626169952, 36.98502408145593989, -5.678558825948271327 ) ) ;
#1183=CARTESIAN_POINT ( 'NONE',  ( 66.04647813311905225, 68.58207190585535784, 1.910909007557326511 ) ) ;
#1189=CARTESIAN_POINT ( 'NONE',  ( 8.675723883004064163, 25.98502408145591147, -5.678558825948271327 ) ) ;
#1200=CARTESIAN_POINT ( 'NONE',  ( 72.95595290250773246, 70.82077856083527934, 7.354924289292173789 ) ) ;
#1202=CARTESIAN_POINT ( 'NONE',  ( 69.03881359575697729, 65.98136758018425496, 11.20795008971583684 ) ) ;
#1206=CARTESIAN_POINT ( 'NONE',  ( 79.40841717930322829, 59.11818797871130471, -16.22797407547709625 ) ) ;
#1208=AXIS2_PLACEMENT_3D ( 'NONE', #24560, #55440, #15445 ) ;
#1209=CARTESIAN_POINT ( 'NONE',  ( 12.22230530498201873, 30.55466486950698624, -1.111400068045478839E-16 ) ) ;
#1219=CARTESIAN_POINT ( 'NONE',  ( 73.18653013103410387, 60.48222858781691258, 15.22147476568558844 ) ) ;
#1221=CARTESIAN_POINT ( 'NONE',  ( 67.16256804578091533, 66.80979783321161847, 8.146902435796070208 ) ) ;
#1230=CARTESIAN_POINT ( 'NONE',  ( 77.13133243787581250, 56.32679435582689109, -16.61903968960224276 ) ) ;
#1231=CARTESIAN_POINT ( 'NONE',  ( 17.52119783388727825, 25.51421378149919050, -9.188101187500004485 ) ) ;
#1240=ADVANCED_FACE ( 'NONE', ( #61718 ), #29070, .T. ) ;
#1241=CARTESIAN_POINT ( 'NONE',  ( 81.94105283978521470, 45.99306238629856836, -11.35642118984577742 ) ) ;
#1243=EDGE_CURVE ( 'NONE', #60091, #33639, #89459, .T. ) ;
#1249=EDGE_CURVE ( 'NONE', #55525, #87546, #43781, .T. ) ;
#1254=CARTESIAN_POINT ( 'NONE',  ( 82.12570432893160444, 40.77989999240937635, -1.063904901471852460 ) ) ;
#1259=CARTESIAN_POINT ( 'NONE',  ( 75.59751354683669433, 65.29851079375914935, 14.32525510856802065 ) ) ;
#1265=CYLINDRICAL_SURFACE ( 'NONE', #17844, 10.00000000000001066 ) ;
#1266=CARTESIAN_POINT ( 'NONE',  ( 33.48063555417975579, 19.73415679381824006, -6.890680421881970419E-14 ) ) ;
#1269=CARTESIAN_POINT ( 'NONE',  ( 74.16736989203016606, 68.80940149631990721, -11.31408104362165545 ) ) ;
#1274=ORIENTED_EDGE ( 'NONE', *, *, #51563, .T. ) ;
#1288=CARTESIAN_POINT ( 'NONE',  ( 69.81840073347110831, 69.95620362085875854, 5.184656770469231013 ) ) ;
#1295=CARTESIAN_POINT ( 'NONE',  ( 15.78795072819010770, 21.06628583063840665, -9.188101187500006262 ) ) ;
#1296=LINE ( 'NONE', #61575, #47588 ) ;
#1303=DIRECTION ( 'NONE',  ( 0.2925570654631164946, 0.000000000000000000, 0.9562480658530033706 ) ) ;
#1307=CARTESIAN_POINT ( 'NONE',  ( 86.22318085410130095, 47.68456650864125379, 10.79712569785469967 ) ) ;
#1308=ORIENTED_EDGE ( 'NONE', *, *, #3460, .T. ) ;
#1310=CARTESIAN_POINT ( 'NONE',  ( 75.53059436383961156, 63.11701598167661587, -15.26357697694628612 ) ) ;
#1313=CARTESIAN_POINT ( 'NONE',  ( 72.06470348997973474, 72.25603645428108734, 1.367373202405260946 ) ) ;
#1314=CARTESIAN_POINT ( 'NONE',  ( 79.30914410335456921, 50.55166203070548647, 14.90691090266632557 ) ) ;
#1322=CARTESIAN_POINT ( 'NONE',  ( 41.28156676870083430, 26.76004757982093452, 5.678558825948272215 ) ) ;
#1323=CARTESIAN_POINT ( 'NONE',  ( 86.25352412292622262, 43.32776165798921397, 4.621746443381918645 ) ) ;
#1328=CARTESIAN_POINT ( 'NONE',  ( 82.55913317860365908, 44.02162453438392475, -9.665417050538319899 ) ) ;
#1330=CARTESIAN_POINT ( 'NONE',  ( 86.50330892798304205, 47.09883604031134752, -10.56546389670383235 ) ) ;
#1340=DIRECTION ( 'NONE',  ( -0.8660254037844379305, -0.5000000000000014433, -0.000000000000000000 ) ) ;
#1343=CARTESIAN_POINT ( 'NONE',  ( 78.63827745602966957, 50.59572098740068924, 15.06237687010368909 ) ) ;
#1344=ORIENTED_EDGE ( 'NONE', *, *, #90823, .F. ) ;
#1349=CARTESIAN_POINT ( 'NONE',  ( 79.47185235748389687, 46.29617394947011633, 12.66262444679482257 ) ) ;
#1352=CARTESIAN_POINT ( 'NONE',  ( 76.90746743093833970, 62.93938289886319382, -15.23233999435671215 ) ) ;
#1357=VECTOR ( 'NONE', #24801, 1000.000000000000114 ) ;
#1358=ORIENTED_EDGE ( 'NONE', *, *, #76601, .F. ) ;
#1360=CARTESIAN_POINT ( 'NONE',  ( 82.07993970318088373, 43.40442941875307525, -9.247700843510214597 ) ) ;
#1367=CARTESIAN_POINT ( 'NONE',  ( 71.78650793969821109, 60.87908065824935022, 14.79100780097532919 ) ) ;
#1369=CARTESIAN_POINT ( 'NONE',  ( 79.51266829831004657, 58.44199966345352948, 16.61175003844716258 ) ) ;
#1375=CARTESIAN_POINT ( 'NONE',  ( 65.78143134570771622, 69.10410598619917266, -0.2546738380904993160 ) ) ;
#1391=CARTESIAN_POINT ( 'NONE',  ( 73.54766422090952460, 64.98954179014701538, 13.85985167941228546 ) ) ;
#1395=CARTESIAN_POINT ( 'NONE',  ( 74.07459009150333884, 68.62600853808264389, 11.43350474783683879 ) ) ;
#1397=CARTESIAN_POINT ( 'NONE',  ( 68.42167172887349125, 70.09380820080993146, 1.014016391010813978 ) ) ;
#1401=CARTESIAN_POINT ( 'NONE',  ( 66.81833236730544456, 68.44078315879002616, 5.955615777142785561 ) ) ;
#1405=CARTESIAN_POINT ( 'NONE',  ( 78.11592650351285272, 47.71665711652420327, 14.50685932715414239 ) ) ;
#1407=CARTESIAN_POINT ( 'NONE',  ( 78.06834474603437002, 54.98730760881699098, 16.09275306223789315 ) ) ;
#1409=CARTESIAN_POINT ( 'NONE',  ( 77.85473067527519220, 62.02510648819682615, 15.65027994488795215 ) ) ;
#1410=CARTESIAN_POINT ( 'NONE',  ( 67.05596152584389813, 66.86776152947172136, 8.884023177476819910 ) ) ;
#1411=CARTESIAN_POINT ( 'NONE',  ( 76.06974868155622005, 51.35906999481754553, 15.65069530268658404 ) ) ;
#1416=CARTESIAN_POINT ( 'NONE',  ( 71.65180518398884146, 72.09936778357817388, 3.358463432740978138 ) ) ;
#1421=CARTESIAN_POINT ( 'NONE',  ( 88.37445845132181432, 44.20200228399612286, 0.05334810252746784165 ) ) ;
#1425=CARTESIAN_POINT ( 'NONE',  ( 77.48284268753138804, 49.21606489196949497, 15.29539255787453911 ) ) ;
#1429=CARTESIAN_POINT ( 'NONE',  ( 29.91980124543643171, 22.98920272979927759, 7.433330006724137462 ) ) ;
#1431=CARTESIAN_POINT ( 'NONE',  ( 81.84538571332693380, 47.30605694451114829, -12.45174469400575035 ) ) ;
#1432=CARTESIAN_POINT ( 'NONE',  ( 8.584303441219292452, 23.14336893147753571, 7.433330006724141015 ) ) ;
#1441=CARTESIAN_POINT ( 'NONE',  ( 76.78612666066324266, 56.27578982940967478, -16.16415727311750672 ) ) ;
#1446=ORIENTED_EDGE ( 'NONE', *, *, #13820, .F. ) ;
#1447=CARTESIAN_POINT ( 'NONE',  ( 77.68170011982932976, 49.37347120871703510, 15.31094863473072998 ) ) ;
#1453=CARTESIAN_POINT ( 'NONE',  ( 72.78091084507063613, 68.76417989200491832, -9.950453267798913259 ) ) ;
#1457=CARTESIAN_POINT ( 'NONE',  ( 72.44040225518423881, 71.75621485965102408, 5.770394931239938963 ) ) ;
#1460=EDGE_LOOP ( 'NONE', ( #77178, #31949, #62735, #10441 ) ) ;
#1461=CARTESIAN_POINT ( 'NONE',  ( 28.30082151474694285, 24.84335787977763843, 9.188101187500006262 ) ) ;
#1463=CARTESIAN_POINT ( 'NONE',  ( 75.25625879159228759, 66.47192257091543865, -13.14164885170834829 ) ) ;
#1464=CARTESIAN_POINT ( 'NONE',  ( 83.51651814802133345, 48.25154606481438435, -12.48491116408185242 ) ) ;
#1467=ADVANCED_FACE ( 'NONE', ( #100006 ), #21020, .T. ) ;
#1471=CARTESIAN_POINT ( 'NONE',  ( 68.17803913764699075, 65.49435412443665427, 10.45721739836550945 ) ) ;
#1472=CARTESIAN_POINT ( 'NONE',  ( 67.95004079286472631, 65.25863045202757462, -10.56757888573983273 ) ) ;
#1483=CARTESIAN_POINT ( 'NONE',  ( 78.14988184308933228, 61.89697373328141339, -16.07278474554906467 ) ) ;
#1488=EDGE_CURVE ( 'NONE', #43189, #82089, #98518, .T. ) ;
#1489=CARTESIAN_POINT ( 'NONE',  ( 80.02629435240551459, 44.46182459010558574, -11.62687173039730304 ) ) ;
#1491=CARTESIAN_POINT ( 'NONE',  ( 81.20643963274024202, 55.68550677472633481, 16.38154045842715334 ) ) ;
#1500=EDGE_LOOP ( 'NONE', ( #32127, #61385, #61163, #87761 ) ) ;
#1503=CARTESIAN_POINT ( 'NONE',  ( 75.81625539762656274, 65.12695345013474935, -14.47344923651660054 ) ) ;
#1504=CARTESIAN_POINT ( 'NONE',  ( 19.15050853525752927, 34.55466486950700045, 7.012934429366973338E-14 ) ) ;
#1507=CARTESIAN_POINT ( 'NONE',  ( 87.82600437409995209, 44.28008912978396694, 4.743525404917309451 ) ) ;
#1509=CARTESIAN_POINT ( 'NONE',  ( 84.86869520348948015, 43.75225087683188718, -6.313702690781472171 ) ) ;
#1510=EDGE_CURVE ( 'NONE', #25763, #18263, #85329, .T. ) ;
#1520=VECTOR ( 'NONE', #88040, 1000.000000000000114 ) ;
#1522=DIRECTION ( 'NONE',  ( 0.8660254037844377084, 0.5000000000000015543, 0.000000000000000000 ) ) ;
#1531=CARTESIAN_POINT ( 'NONE',  ( 76.21540257404608099, 63.22959166649816609, -14.98001016604830937 ) ) ;
#1533=CARTESIAN_POINT ( 'NONE',  ( 73.83419370605903964, 55.14121766272175051, 16.60004764102358976 ) ) ;
#1535=CARTESIAN_POINT ( 'NONE',  ( 34.63914548426571827, 22.12755873383627758, -6.180339887498949025 ) ) ;
#1542=DIRECTION ( 'NONE',  ( 0.7467472232290855993, 0.000000000000000000, 0.6651079495838628786 ) ) ;
#1546=CARTESIAN_POINT ( 'NONE',  ( 81.38228331512368641, 42.18052851754683275, 8.075145019496558163 ) ) ;
#1549=FACE_OUTER_BOUND ( 'NONE', #81417, .T. ) ;
#1550=CARTESIAN_POINT ( 'NONE',  ( 32.81602777569660390, 24.11029122506295863, -8.090169943749478065 ) ) ;
#1554=CARTESIAN_POINT ( 'NONE',  ( 81.86130692232174511, 42.15755783746833885, 7.590521390274829194 ) ) ;
#1555=CARTESIAN_POINT ( 'NONE',  ( 87.17901322616850734, 46.26306768054848817, -8.477718022526687491 ) ) ;
#1559=CARTESIAN_POINT ( 'NONE',  ( 72.05627613218693739, 66.49406252133579187, -11.67341081358113009 ) ) ;
#1564=CARTESIAN_POINT ( 'NONE',  ( 77.21724311172287969, 49.67724645580758391, -14.99754053603360759 ) ) ;
#1566=EDGE_CURVE ( 'NONE', #78218, #96180, #31528, .T. ) ;
#1574=CARTESIAN_POINT ( 'NONE',  ( 23.25741983583088413, 25.37878583063841376, 9.188101187500006262 ) ) ;
#1580=CARTESIAN_POINT ( 'NONE',  ( 12.27453364332850505, 12.80170272979924739, 7.433330006724137462 ) ) ;
#1581=CARTESIAN_POINT ( 'NONE',  ( 75.89814051312130516, 58.95594745416783411, -15.95455651496020444 ) ) ;
#1582=CARTESIAN_POINT ( 'NONE',  ( 71.79363655647949827, 72.51690322118082577, -1.318798153274830076 ) ) ;
#1597=CARTESIAN_POINT ( 'NONE',  ( 71.80779569229208903, 72.11915028389421423, -3.640749997624285417 ) ) ;
#1598=CARTESIAN_POINT ( 'NONE',  ( 72.95919681002737889, 57.42441093631072846, -15.86686462681733900 ) ) ;
#1599=FACE_OUTER_BOUND ( 'NONE', #7023, .T. ) ;
#1601=B_SPLINE_CURVE_WITH_KNOTS ( 'NONE', 3,
 ( #2491, #88138, #64277, #3972, #56156, #87151, #33373, #49083, #10585, #17683, #48583, #1984, #65270, #18684, #19202, #72906, #86633, #80016 ),
 .UNSPECIFIED., .F., .F.,
 ( 4, 2, 2, 1, 2, 2, 2, 2, 1, 4 ),
 ( 0.000000000000000000, 0.1185760491640068387, 0.1482200614550078510, 0.1778640737460088217, 0.2371520983280109851, 0.2964401229100130930, 0.3557281474920152564, 0.3853721597830173096, 0.4150161720740193072, 0.4743041966560226363 ),
 .UNSPECIFIED. ) ;
#1607=ORIENTED_EDGE ( 'NONE', *, *, #96781, .F. ) ;
#1608=CARTESIAN_POINT ( 'NONE',  ( 21.45803809350889679, 35.49540643055188127, 3.479690158560446702E-15 ) ) ;
#1610=CARTESIAN_POINT ( 'NONE',  ( 78.58598452914725385, 47.91960314448038361, -14.47352538085859486 ) ) ;
#1613=CARTESIAN_POINT ( 'NONE',  ( 73.93840856004327122, 68.59252082510937498, 10.89217114877860659 ) ) ;
#1632=CARTESIAN_POINT ( 'NONE',  ( 75.85858666007513307, 65.60472725796547877, 13.84649109559921420 ) ) ;
#1633=CARTESIAN_POINT ( 'NONE',  ( 72.92312356590035449, 64.99263871788808444, -13.11958098651873250 ) ) ;
#1640=LINE ( 'NONE', #9219, #16588 ) ;
#1642=CARTESIAN_POINT ( 'NONE',  ( 83.70956241415673560, 51.66838590121233210, -14.83800726304596118 ) ) ;
#1648=CARTESIAN_POINT ( 'NONE',  ( 74.66818547213321722, 67.01009517369644186, 12.98877810528427013 ) ) ;
#1655=CARTESIAN_POINT ( 'NONE',  ( 85.67021663899103601, 48.38166113680176750, -11.71697781433778651 ) ) ;
#1656=CARTESIAN_POINT ( 'NONE',  ( 88.06181012395556706, 44.63806904432505007, -4.156701318329214523 ) ) ;
#1657=CARTESIAN_POINT ( 'NONE',  ( 80.12748291632911446, 44.63541364795098332, -11.72772784125804080 ) ) ;
#1659=CARTESIAN_POINT ( 'NONE',  ( 82.28509353309422636, 41.51255840690875232, -5.852911540032354587 ) ) ;
#1664=B_SPLINE_SURFACE_WITH_KNOTS ( 'NONE', 3, 1, ( 
 ( #78285, #14961 ),
 ( #70666, #32165 ),
 ( #63069, #94012 ),
 ( #47849, #40254 ),
 ( #71194, #1787 ),
 ( #53463, #45849 ),
 ( #7365, #38250 ),
 ( #65072, #96021 ),
 ( #95019, #26584 ),
 ( #79818, #3783 ),
 ( #80833, #33689 ),
 ( #4263, #10887 ),
 ( #57457, #65567 ),
 ( #49373, #88951 ),
 ( #80316, #64074 ),
 ( #35162, #72709 ),
 ( #64583, #19506 ),
 ( #18488, #73189 ),
 ( #34665, #3299 ),
 ( #95535, #66072 ),
 ( #88436, #48884 ),
 ( #17471, #41763 ),
 ( #81317, #25582 ),
 ( #50363, #2294 ),
 ( #11888, #34178 ),
 ( #18997, #25065 ),
 ( #9894, #26083 ),
 ( #55941, #2802 ),
 ( #49872, #33174 ),
 ( #72195, #11401 ),
 ( #56468, #86939 ) ),
 .UNSPECIFIED., .F., .F., .F.,
 ( 4, 3, 3, 3, 3, 3, 3, 3, 3, 3, 4 ),
 ( 2, 2 ),
 ( 0.000000000000000000, 0.1122669598086777770, 0.2243161639709639332, 0.3396355846219138996, 0.4553962076585105212, 0.5677860799922255230, 0.6749047109689485513, 0.7773884377078289498, 0.8775581155834147884, 0.9782364162377931160, 1.000000000000000000 ),
 ( 0.000000000000000000, 1.000000000000000000 ),
 .UNSPECIFIED. ) ;
#1665=CARTESIAN_POINT ( 'NONE',  ( 78.86766380650875874, 52.46362257666628182, -15.56641557883455818 ) ) ;
#1669=CARTESIAN_POINT ( 'NONE',  ( 87.74913801566610516, 44.74219947183942026, 5.012341453613225362 ) ) ;
#1671=CARTESIAN_POINT ( 'NONE',  ( 20.42956747364522485, 12.76426979415089313, 3.090169943749476733 ) ) ;
#1674=LINE ( 'NONE', #94391, #78214 ) ;
#1675=CARTESIAN_POINT ( 'NONE',  ( 12.36470590445056317, 8.108019796199268825, 3.090169943749476733 ) ) ;
#1680=CARTESIAN_POINT ( 'NONE',  ( 66.76293781782166548, 68.40909042380869209, -4.422493503458938768 ) ) ;
#1687=CARTESIAN_POINT ( 'NONE',  ( 41.60632629512001301, 26.94754757982092741, 5.678558825948272215 ) ) ;
#1694=CARTESIAN_POINT ( 'NONE',  ( 66.05284405871212527, 69.03255062257417762, 2.566972579851455993 ) ) ;
#1697=SHAPE_REPRESENTATION_RELATIONSHIP ( 'NONE' , 'NONE' ,  #46310, #3033 ) ;
#1700=CARTESIAN_POINT ( 'NONE',  ( 11.45782370926791849, 18.56628583063839244, 9.188101187500006262 ) ) ;
#1713=CARTESIAN_POINT ( 'NONE',  ( 86.11363163537949106, 47.05074959952599301, 10.74854466831323840 ) ) ;
#1714=ORIENTED_EDGE ( 'NONE', *, *, #95099, .F. ) ;
#1715=CARTESIAN_POINT ( 'NONE',  ( 20.44744908501035496, 27.50829794293880681, -10.00000000000000355 ) ) ;
#1719=CARTESIAN_POINT ( 'NONE',  ( 78.96380797632822635, 59.43460744216078950, -16.52597720501997358 ) ) ;
#1724=CARTESIAN_POINT ( 'NONE',  ( 20.43632886220093070, 13.92755873383625698, 6.180339887498953466 ) ) ;
#1727=CARTESIAN_POINT ( 'NONE',  ( 6.396987757676594555, 15.64441083166260427, 0.000000000000000000 ) ) ;
#1729=CARTESIAN_POINT ( 'NONE',  ( 34.97582608256301739, 32.14441083166263979, 10.00000000000000533 ) ) ;
#1735=CARTESIAN_POINT ( 'NONE',  ( 73.34097623508702668, 61.15009553395870512, 15.04177895589568337 ) ) ;
#1739=ADVANCED_FACE ( 'NONE', ( #30463 ), #38042, .T. ) ;
#1740=CARTESIAN_POINT ( 'NONE',  ( 82.34639549499804900, 46.43828254362050956, 11.54952222346724966 ) ) ;
#1741=CARTESIAN_POINT ( 'NONE',  ( 71.58674681710026277, 69.69452789951117211, 7.786173541551400845 ) ) ;
#1747=CARTESIAN_POINT ( 'NONE',  ( 22.57541804695699028, 15.96004757982090183, -5.678558825948276656 ) ) ;
#1751=ORIENTED_EDGE ( 'NONE', *, *, #46900, .F. ) ;
#1759=VERTEX_POINT ( 'NONE', #6673 ) ;
#1765=CARTESIAN_POINT ( 'NONE',  ( 82.46956611399556891, 40.45592067260756863, -1.389944151191353505 ) ) ;
#1768=EDGE_CURVE ( 'NONE', #70878, #65992, #27919, .T. ) ;
#1770=CARTESIAN_POINT ( 'NONE',  ( 75.94843506473843320, 65.47918399976401815, 14.33637728062728556 ) ) ;
#1772=EDGE_LOOP ( 'NONE', ( #89350, #83464, #66589, #34713 ) ) ;
#1776=CARTESIAN_POINT ( 'NONE',  ( 69.34433977682154193, 70.64122323216504640, 0.8389772499948148221 ) ) ;
#1777=CARTESIAN_POINT ( 'NONE',  ( 26.33642183074452703, 30.90829794293881960, 10.00000000000000355 ) ) ;
#1778=CARTESIAN_POINT ( 'NONE',  ( 82.35975313173908319, 41.41624149291901347, 5.521678208619407613 ) ) ;
#1779=CARTESIAN_POINT ( 'NONE',  ( 82.23066470189330346, 42.55849650999721945, 6.877359557377351607 ) ) ;
#1787=CARTESIAN_POINT ( 'NONE',  ( 68.78537064792701017, 63.83817091373786212, -12.21312428423394536 ) ) ;
#1795=ORIENTED_EDGE ( 'NONE', *, *, #38607, .F. ) ;
#1798=CARTESIAN_POINT ( 'NONE',  ( 11.52878981408637848, 24.84336893147754921, -7.433330006724137462 ) ) ;
#1800=DIRECTION ( 'NONE',  ( -0.8660254037844377084, -0.5000000000000014433, -0.000000000000000000 ) ) ;
#1804=CARTESIAN_POINT ( 'NONE',  ( 26.98754258172029452, 23.78052372038641238, -10.00000000000000355 ) ) ;
#1808=CARTESIAN_POINT ( 'NONE',  ( 86.36553431312867701, 47.62854645161011291, 10.65446341473505321 ) ) ;
#1809=ORIENTED_EDGE ( 'NONE', *, *, #66514, .F. ) ;
#1811=CARTESIAN_POINT ( 'NONE',  ( 16.82306525903893046, 33.21091486745860522, -1.111400068045478839E-16 ) ) ;
#1813=VERTEX_POINT ( 'NONE', #37550 ) ;
#1814=CARTESIAN_POINT ( 'NONE',  ( 72.10789540236547168, 72.29255521243572957, 1.270859788509655974 ) ) ;
#1816=CARTESIAN_POINT ( 'NONE',  ( 79.38695290519767411, 50.85501981317847964, 15.00243835328062936 ) ) ;
#1817=CARTESIAN_POINT ( 'NONE',  ( 83.90589546250612329, 51.88876590914236431, -14.49782437550669734 ) ) ;
#1818=EDGE_CURVE ( 'NONE', #2161, #41560, #5184, .T. ) ;
#1823=ADVANCED_FACE ( 'NONE', ( #29965 ), #60842, .T. ) ;
#1824=CARTESIAN_POINT ( 'NONE',  ( 37.26657704017246431, 36.91421378149922816, 9.188101187500008038 ) ) ;
#1832=CARTESIAN_POINT ( 'NONE',  ( 86.52979389935374854, 47.15173288509246419, -10.60481917042622868 ) ) ;
#1836=CARTESIAN_POINT ( 'NONE',  ( 6.965316927136144365, 15.97253583063838711, -10.00000000000000533 ) ) ;
#1837=CARTESIAN_POINT ( 'NONE',  ( 80.51741848527098000, 44.46186292381598548, 11.37106337338451922 ) ) ;
#1842=ORIENTED_EDGE ( 'NONE', *, *, #75121, .F. ) ;
#1843=CARTESIAN_POINT ( 'NONE',  ( 77.33513981957392502, 49.70526746924971206, -15.49639835079455352 ) ) ;
#1849=CARTESIAN_POINT ( 'NONE',  ( 25.52770680675560655, 38.23654200823203553, 1.583844403245397769 ) ) ;
#1854=LINE ( 'NONE', #84976, #51747 ) ;
#1857=CARTESIAN_POINT ( 'NONE',  ( 70.59331980588027022, 60.81386183084845243, -15.05063277410530276 ) ) ;
#1891=B_SPLINE_CURVE_WITH_KNOTS ( 'NONE', 3,
 ( #60396, #97942, #91352, #83761, #37601, #14322, #5232, #68512, #74655, #22417, #59399, #53308, #84263, #20442, #51311, #82281, #45693, #36112, #76621, #38090, #13342, #75143, #69002, #12853, #67016, #28516, #5721, #123, #32000, #8717, #17311, #16810, #92847, #8220, #77635, #85258, #39089, #23904, #617, #32522, #63415, #70002, #24416, #69509, #15804, #94354 ),
 .UNSPECIFIED., .F., .F.,
 ( 4, 1, 2, 2, 1, 2, 2, 1, 1, 2, 2, 1, 1, 2, 2, 1, 1, 2, 2, 1, 1, 1, 2, 2, 1, 1, 1, 2, 2, 4 ),
 ( 0.000000000000000000, 0.06249999999998623323, 0.09374999999997925271, 0.1249999999999722722, 0.1874999999999620859, 0.2187499999999555633, 0.2499999999999490408, 0.3124999999999369393, 0.3437499999999324984, 0.3593749999999296674, 0.3749999999999268363, 0.4374999999999081846, 0.4687499999998982481, 0.4843749999998948064, 0.4999999999998913092, 0.5624999999998865352, 0.5937499999998842037, 0.6093749999998808731, 0.6249999999998775424, 0.6874999999998750999, 0.7187499999998721023, 0.7343749999998727684, 0.7421874999998735456, 0.7499999999998744338, 0.8124999999998896438, 0.8437499999998965272, 0.8593749999999006350, 0.8671874999999048539, 0.8749999999999091838, 1.000000000000000000 ),
 .UNSPECIFIED. ) ;
#1893=CARTESIAN_POINT ( 'NONE',  ( 73.05912352472130067, 69.60491006942920933, 9.219028434792550186 ) ) ;
#1894=CARTESIAN_POINT ( 'NONE',  ( 74.40909250051804236, 68.25437571282814986, 11.42766049309473786 ) ) ;
#1896=CARTESIAN_POINT ( 'NONE',  ( 67.16990927169524639, 66.79708245693809943, -9.067759095298582039 ) ) ;
#1898=CARTESIAN_POINT ( 'NONE',  ( 67.12017456359353673, 66.69520300484214204, 8.276391925158705476 ) ) ;
#1899=CARTESIAN_POINT ( 'NONE',  ( 87.97374987192618789, 44.76517282144749288, -4.661398658539860129 ) ) ;
#1900=CARTESIAN_POINT ( 'NONE',  ( 76.48640248419295062, 51.58918322513654431, 15.64831315713033355 ) ) ;
#1905=CARTESIAN_POINT ( 'NONE',  ( 78.28914660356475963, 61.64131563665610969, 15.78308208647086985 ) ) ;
#1911=CARTESIAN_POINT ( 'NONE',  ( 77.74985625145598078, 55.20120347894719970, -16.12416396296487520 ) ) ;
#1915=CARTESIAN_POINT ( 'NONE',  ( 76.98305832116996328, 63.37377475765585899, -15.46912589935254623 ) ) ;
#1918=CARTESIAN_POINT ( 'NONE',  ( 88.06041215430452951, 44.01892986890200632, 0.5558169716948772043 ) ) ;
#1920=CARTESIAN_POINT ( 'NONE',  ( 82.34202771369412233, 42.93952482416137428, -8.411501796766556183 ) ) ;
#1923=CARTESIAN_POINT ( 'NONE',  ( 27.11724708220625857, 33.84336893147757763, -7.433330006724137462 ) ) ;
#1924=CARTESIAN_POINT ( 'NONE',  ( 80.93147017124917397, 45.39363699920941286, 11.98508622504169985 ) ) ;
#1927=CARTESIAN_POINT ( 'NONE',  ( 24.28581821943125263, 16.94754757982090254, 5.678558825948272215 ) ) ;
#1929=CARTESIAN_POINT ( 'NONE',  ( 76.59052817429427762, 63.78587366202882691, 14.87114199683171734 ) ) ;
#1930=CARTESIAN_POINT ( 'NONE',  ( 82.56047309644807797, 54.07683023134062239, -15.52634518316282630 ) ) ;
#1939=CARTESIAN_POINT ( 'NONE',  ( 82.31027433114240921, 53.67166805628563964, 15.82896004337745310 ) ) ;
#1948=CARTESIAN_POINT ( 'NONE',  ( 72.49874796052694137, 71.64632196231394801, 6.095118657294443132 ) ) ;
#1952=CARTESIAN_POINT ( 'NONE',  ( 30.11465696128792757, 23.10170272979928541, -7.433330006724141015 ) ) ;
#1953=CARTESIAN_POINT ( 'NONE',  ( 84.68046352546232924, 50.54697168049320055, -14.01127729920333742 ) ) ;
#1955=ORIENTED_EDGE ( 'NONE', *, *, #57301, .T. ) ;
#1962=CARTESIAN_POINT ( 'NONE',  ( 68.11204775988159099, 65.46590518901473388, 10.44757278393263888 ) ) ;
#1966=CARTESIAN_POINT ( 'NONE',  ( 38.51650576605270970, 30.43677371833804202, -10.00000000000000355 ) ) ;
#1970=CARTESIAN_POINT ( 'NONE',  ( 79.31323107047896315, 59.76145823410249136, 16.51491591541846304 ) ) ;
#1980=CARTESIAN_POINT ( 'NONE',  ( 80.04850862667662170, 44.86057290276260545, -11.28600205406214663 ) ) ;
#1984=CARTESIAN_POINT ( 'NONE',  ( 84.65630082135325551, 42.18976564707919152, -0.8137823442531888496 ) ) ;
#1985=CARTESIAN_POINT ( 'NONE',  ( 81.63649175858802209, 48.05684571567061880, -13.06511883598228430 ) ) ;
#1992=CARTESIAN_POINT ( 'NONE',  ( 75.86452061248199641, 65.14283366293828692, -14.47928019947265277 ) ) ;
#1996=CARTESIAN_POINT ( 'NONE',  ( 88.05221915382541908, 44.76013711945522289, 4.532355379009165297 ) ) ;
#2005=VERTEX_POINT ( 'NONE', #16260 ) ;
#2006=DIRECTION ( 'NONE',  ( -0.3213938048432640748, 0.5566703992264119272, -0.7660444431189857850 ) ) ;
#2010=CARTESIAN_POINT ( 'NONE',  ( 83.37579341631962393, 51.76272850660085822, 14.96038908820327507 ) ) ;
#2015=CARTESIAN_POINT ( 'NONE',  ( 76.47821338308438044, 63.12304481703771586, -15.07910235800729204 ) ) ;
#2017=CARTESIAN_POINT ( 'NONE',  ( 73.70322323093775196, 55.31382080484373631, 16.11694223268900927 ) ) ;
#2019=CARTESIAN_POINT ( 'NONE',  ( 31.51172446742527100, 30.14441083166263269, 10.00000000000000533 ) ) ;
#2028=CARTESIAN_POINT ( 'NONE',  ( 82.19827357919754718, 47.83406103887718075, 12.71279386660662958 ) ) ;
#2031=CARTESIAN_POINT ( 'NONE',  ( 26.65225264301594166, 37.16126292948896293, -6.180339887498951690 ) ) ;
#2033=CARTESIAN_POINT ( 'NONE',  ( 81.97703060113059337, 41.73519428853659718, 5.412281464924958208 ) ) ;
#2037=CARTESIAN_POINT ( 'NONE',  ( 37.82368544302515545, 30.03677371833804699, 10.00000000000000533 ) ) ;
#2041=CARTESIAN_POINT ( 'NONE',  ( 81.22934400301913627, 56.18010474871477555, 16.10233499384894174 ) ) ;
#2047=CARTESIAN_POINT ( 'NONE',  ( 84.02300986820688422, 51.73893231647485180, 14.78971152351953045 ) ) ;
#2051=CARTESIAN_POINT ( 'NONE',  ( 71.79182426994934474, 66.53813379304610010, -11.50093241856152559 ) ) ;
#2055=CARTESIAN_POINT ( 'NONE',  ( 67.31503155234506153, 66.65634768321555725, -8.484550801122479058 ) ) ;
#2058=CARTESIAN_POINT ( 'NONE',  ( 67.28733722124985661, 66.41312804726935326, -8.801120809818232971 ) ) ;
#2061=AXIS2_PLACEMENT_3D ( 'NONE', #98573, #23019, #29156 ) ;
#2066=CARTESIAN_POINT ( 'NONE',  ( 32.62131273085646654, 21.76004757982090965, 5.678558825948272215 ) ) ;
#2072=CARTESIAN_POINT ( 'NONE',  ( 14.66449673273962162, 9.262165230724928477, -2.296566073217252530E-15 ) ) ;
#2075=CARTESIAN_POINT ( 'NONE',  ( 73.31883174054932795, 59.80927123552942959, -15.43389514559521558 ) ) ;
#2076=CARTESIAN_POINT ( 'NONE',  ( 71.47791206682282450, 72.34364865201936823, -1.216664393387151488 ) ) ;
#2089=CARTESIAN_POINT ( 'NONE',  ( 73.12133584826474930, 57.41764960941905827, -15.88333458976553381 ) ) ;
#2090=LINE ( 'NONE', #85219, #22466 ) ;
#2091=B_SPLINE_CURVE_WITH_KNOTS ( 'NONE', 3,
 ( #32829, #40909, #48543, #9556, #85594, #39411, #85070, #62718, #93166, #100255, #79483, #10046, #93675, #31816, #31327, #94672, #30837, #16135, #47033, #71352, #61723, #94176, #77950, #940, #24239, #24727, #48025, #15617, #54112, #25229, #78969, #92670, #55117, #46515, #77453, #47526, #9036, #39908, #70841, #1453, #40419, #86594, #56116, #19162, #75216, #43788 ),
 .UNSPECIFIED., .F., .F.,
 ( 4, 1, 1, 1, 2, 2, 1, 1, 1, 2, 2, 1, 1, 2, 2, 1, 1, 2, 2, 1, 1, 2, 2, 1, 2, 2, 1, 2, 2, 4 ),
 ( 0.000000000000000000, 0.06250000000000756339, 0.09375000000001003364, 0.1093750000000108941, 0.1171875000000097977, 0.1250000000000086875, 0.1875000000000000278, 0.2187499999999972800, 0.2343749999999944489, 0.2421874999999930334, 0.2499999999999916178, 0.3124999999999925060, 0.3437499999999928946, 0.3593749999999915623, 0.3749999999999902300, 0.4374999999999908962, 0.4687499999999912292, 0.4843749999999913958, 0.4999999999999915623, 0.5624999999999952260, 0.5937499999999971134, 0.6093749999999963363, 0.6249999999999955591, 0.6874999999999895639, 0.7187499999999882316, 0.7499999999999868994, 0.8124999999999877875, 0.8437499999999895639, 0.8749999999999913403, 1.000000000000000000 ),
 .UNSPECIFIED. ) ;
#2099=CARTESIAN_POINT ( 'NONE',  ( 31.23567208480136514, 20.96004757982091604, -5.678558825948276656 ) ) ;
#2101=CARTESIAN_POINT ( 'NONE',  ( 71.07376813403469384, 70.69339414025402846, -6.375625711488249969 ) ) ;
#2103=CARTESIAN_POINT ( 'NONE',  ( 73.83553503644242255, 68.51229284434135991, 10.91127707145445314 ) ) ;
#2108=CARTESIAN_POINT ( 'NONE',  ( 76.22354811720457235, 58.03663319312042290, -16.07154475767281099 ) ) ;
#2109=CARTESIAN_POINT ( 'NONE',  ( 83.55665905661119552, 42.82685997504432862, -5.889658287066807496 ) ) ;
#2122=CARTESIAN_POINT ( 'NONE',  ( 67.25018235246020026, 66.88641011210830811, 9.010392920173572406 ) ) ;
#2123=CARTESIAN_POINT ( 'NONE',  ( 73.65118521283083908, 64.80899555395295408, -13.49371764281556807 ) ) ;
#2124=DIRECTION ( 'NONE',  ( -0.2033683215378938036, 0.3522442655536374700, -0.9135454576426059736 ) ) ;
#2132=CARTESIAN_POINT ( 'NONE',  ( 83.52018940653934465, 51.62319858702418429, -14.86581989589152819 ) ) ;
#2135=CARTESIAN_POINT ( 'NONE',  ( 80.34072333937859867, 58.10214405650913250, -16.60604606379114401 ) ) ;
#2137=CARTESIAN_POINT ( 'NONE',  ( 71.76701767287354983, 72.15843607843383722, 0.5844455542204934906 ) ) ;
#2141=EDGE_CURVE ( 'NONE', #77129, #80395, #48652, .T. ) ;
#2147=CARTESIAN_POINT ( 'NONE',  ( 85.47443485840854294, 48.29312219740740630, -11.73648896724759716 ) ) ;
#2152=CARTESIAN_POINT ( 'NONE',  ( 69.93729631481735964, 70.68432073330353660, -3.157426850868849666 ) ) ;
#2153=ADVANCED_FACE ( 'NONE', ( #3897 ), #88553, .T. ) ;
#2160=DIRECTION ( 'NONE',  ( 0.5000000000000014433, -0.8660254037844378194, 0.000000000000000000 ) ) ;
#2161=VERTEX_POINT ( 'NONE', #19119 ) ;
#2165=CARTESIAN_POINT ( 'NONE',  ( 13.94779419600527959, 26.79103043416548147, 8.090169943749478065 ) ) ;
#2167=CARTESIAN_POINT ( 'NONE',  ( 79.57660877456937953, 50.05937193655102391, -15.15852024261339537 ) ) ;
#2169=CARTESIAN_POINT ( 'NONE',  ( 71.88679598306705998, 71.95097395942667617, 2.841373724777338960 ) ) ;
#2178=EDGE_CURVE ( 'NONE', #53490, #54109, #93351, .T. ) ;
#2183=CARTESIAN_POINT ( 'NONE',  ( 34.65648599653719231, 40.98502408145595410, -5.678558825948271327 ) ) ;
#2186=FACE_OUTER_BOUND ( 'NONE', #78731, .T. ) ;
#2187=CARTESIAN_POINT ( 'NONE',  ( 21.78279761992806129, 35.68290643055188838, 3.479690158560446702E-15 ) ) ;
#2195=CARTESIAN_POINT ( 'NONE',  ( 10.59299460361177125, 21.51421378149917274, -9.188101187500004485 ) ) ;
#2197=CARTESIAN_POINT ( 'NONE',  ( 23.27484393518965788, 15.29860640527292226, -2.839279412974138328 ) ) ;
#2203=VERTEX_POINT ( 'NONE', #35786 ) ;
#2204=CARTESIAN_POINT ( 'NONE',  ( 32.31170220804710880, 20.78380873178788946, -6.180339887498949025 ) ) ;
#2206=DIRECTION ( 'NONE',  ( 0.2033683215378999376, -0.3522442655536480172, -0.9135454576426004225 ) ) ;
#2210=ORIENTED_EDGE ( 'NONE', *, *, #40001, .T. ) ;
#2213=CARTESIAN_POINT ( 'NONE',  ( 86.43056390414663781, 47.56170780119803254, 10.54448901942590311 ) ) ;
#2215=CARTESIAN_POINT ( 'NONE',  ( 77.75543676104368274, 57.50219656113497280, 16.18064258310643311 ) ) ;
#2218=CARTESIAN_POINT ( 'NONE',  ( 38.67678797688638070, 22.73415679381825072, -6.890680421881970419E-14 ) ) ;
#2219=CARTESIAN_POINT ( 'NONE',  ( 79.44952676368946243, 59.15621205895340040, -16.22681862362401262 ) ) ;
#2220=AXIS2_PLACEMENT_3D ( 'NONE', #6260, #68551, #76187 ) ;
#2221=CARTESIAN_POINT ( 'NONE',  ( 21.35627990119762032, 12.73415679381821519, 1.333680081654574804E-15 ) ) ;
#2228=EDGE_LOOP ( 'NONE', ( #75387, #38719, #43530, #51865 ) ) ;
#2230=CARTESIAN_POINT ( 'NONE',  ( 40.33962347462181697, 28.45404122711136452, -8.090169943749478065 ) ) ;
#2233=CARTESIAN_POINT ( 'NONE',  ( 74.06167665414214696, 64.39312597440692798, 13.88171286573246910 ) ) ;
#2237=CARTESIAN_POINT ( 'NONE',  ( 84.42663183290279960, 49.91580812419739743, -13.73522929182741059 ) ) ;
#2241=CARTESIAN_POINT ( 'NONE',  ( 73.13476967714908028, 57.39438153525127007, 15.88807208273858684 ) ) ;
#2242=DIRECTION ( 'NONE',  ( -0.2938926261462390666, 0.5090369604551334692, 0.8090169943749425663 ) ) ;
#2247=CARTESIAN_POINT ( 'NONE',  ( 22.22900788544320605, 15.76004757982089544, 5.678558825948272215 ) ) ;
#2252=FACE_OUTER_BOUND ( 'NONE', #24255, .T. ) ;
#2257=DIRECTION ( 'NONE',  ( 0.5000000000000013323, -0.8660254037844378194, 0.000000000000000000 ) ) ;
#2260=CARTESIAN_POINT ( 'NONE',  ( 7.095368192108828076, 22.83478043621386178, -8.090169943749479842 ) ) ;
#2266=CARTESIAN_POINT ( 'NONE',  ( 82.18753490691527475, 40.78579184768809540, -0.6546124752527298085 ) ) ;
#2270=CARTESIAN_POINT ( 'NONE',  ( 75.76889645089327985, 65.47676480558789081, 14.28475327549652540 ) ) ;
#2276=EDGE_CURVE ( 'NONE', #36092, #45167, #84729, .T. ) ;
#2278=CARTESIAN_POINT ( 'NONE',  ( 79.73293522532485156, 47.11546486241463327, -13.12060147480491601 ) ) ;
#2287=CIRCLE ( 'NONE', #37664, 0.5000000000000004441 ) ;
#2290=CARTESIAN_POINT ( 'NONE',  ( 82.56263159380813477, 44.11904566611071488, 8.977829394507185867 ) ) ;
#2291=VECTOR ( 'NONE', #19767, 1000.000000000000114 ) ;
#2294=CARTESIAN_POINT ( 'NONE',  ( 68.97555762870663898, 64.32427639738035907, -11.91833701315977301 ) ) ;
#2298=CARTESIAN_POINT ( 'NONE',  ( 73.52959106948154044, 67.84374563276222148, -11.86275638489837014 ) ) ;
#2306=CARTESIAN_POINT ( 'NONE',  ( 18.92609651878039756, 19.43085787977762280, -9.188101187500008038 ) ) ;
#2307=CARTESIAN_POINT ( 'NONE',  ( 75.25521838011508180, 66.92519264401985879, 13.27308740013157262 ) ) ;
#2311=EDGE_CURVE ( 'NONE', #56696, #93369, #14094, .T. ) ;
#2323=CARTESIAN_POINT ( 'NONE',  ( 79.86762560990425186, 52.96440835099240019, 15.56858714322070014 ) ) ;
#2326=CARTESIAN_POINT ( 'NONE',  ( 75.01736285511192648, 53.01766956676284792, -16.01582039744900143 ) ) ;
#2329=CARTESIAN_POINT ( 'NONE',  ( 35.68911091587340678, 42.64646525600393545, -2.839279412974133887 ) ) ;
#2334=CARTESIAN_POINT ( 'NONE',  ( 87.51038571601205263, 44.12602541333317419, -4.835627537363936135 ) ) ;
#2335=EDGE_LOOP ( 'NONE', ( #36448, #29872, #78999, #49639 ) ) ;
#2336=CARTESIAN_POINT ( 'NONE',  ( 78.82690945070837074, 60.06733921958858247, 16.11100571342160492 ) ) ;
#2338=CARTESIAN_POINT ( 'NONE',  ( 28.28448313147312021, 16.73415679381822230, 1.333680081654574804E-15 ) ) ;
#2339=CARTESIAN_POINT ( 'NONE',  ( 76.06280709947594687, 52.62385153157702433, -15.89955354223746298 ) ) ;
#2346=CARTESIAN_POINT ( 'NONE',  ( 81.19301662773271744, 55.65398007790845014, 16.37810844063417548 ) ) ;
#2348=ADVANCED_FACE ( 'NONE', ( #8376 ), #70664, .T. ) ;
#2350=CARTESIAN_POINT ( 'NONE',  ( 88.32078559155080200, 44.16791947909882765, 0.3596700509409204716 ) ) ;
#2351=CARTESIAN_POINT ( 'NONE',  ( 78.95994887262315842, 51.98449323110317266, 15.44357915373326406 ) ) ;
#2352=ORIENTED_EDGE ( 'NONE', *, *, #58095, .T. ) ;
#2366=CARTESIAN_POINT ( 'NONE',  ( 70.67451223566608576, 61.02758652436570941, -14.45160611066157941 ) ) ;
#2368=CARTESIAN_POINT ( 'NONE',  ( 41.76871284172324295, 36.06628583063844928, -9.188101187500006262 ) ) ;
#2370=CARTESIAN_POINT ( 'NONE',  ( 21.20711791317337003, 34.01751292744057054, 6.180339887498949913 ) ) ;
#2377=CARTESIAN_POINT ( 'NONE',  ( 76.87325692288003154, 51.52439226058535837, -16.07951750168037819 ) ) ;
#2384=VERTEX_POINT ( 'NONE', #69662 ) ;
#2398=CARTESIAN_POINT ( 'NONE',  ( 74.17388174154397973, 65.32774866087831356, -13.41372763693923531 ) ) ;
#2401=CARTESIAN_POINT ( 'NONE',  ( 73.76584831522595209, 68.38082682530665579, 11.49424229391075514 ) ) ;
#2403=CARTESIAN_POINT ( 'NONE',  ( 67.38523018514564455, 69.28993244173518917, 2.473534599136319123 ) ) ;
#2407=CARTESIAN_POINT ( 'NONE',  ( 88.06692388374393943, 44.73466778012474521, -4.429792403987857341 ) ) ;
#2411=CARTESIAN_POINT ( 'NONE',  ( 77.71263964979601724, 53.15247193762592559, 15.85337299538524469 ) ) ;
#2414=CARTESIAN_POINT ( 'NONE',  ( 76.47997935286269922, 51.56731111080835461, 15.64421333830926741 ) ) ;
#2416=CARTESIAN_POINT ( 'NONE',  ( 70.96429761875693032, 61.15374941679502996, 14.99935025239129871 ) ) ;
#2419=CARTESIAN_POINT ( 'NONE',  ( 79.14484663501158934, 45.92919831353032833, -13.14721640033899241 ) ) ;
#2422=CARTESIAN_POINT ( 'NONE',  ( 73.65406247650449245, 69.69847601991219221, 9.512545074604176421 ) ) ;
#2428=AXIS2_PLACEMENT_3D ( 'NONE', #79203, #33564, #78168 ) ;
#2429=CARTESIAN_POINT ( 'NONE',  ( 76.97945238447553606, 53.12258697838318966, -16.36430810493287424 ) ) ;
#2430=CARTESIAN_POINT ( 'NONE',  ( 85.19480112191604348, 49.06367757593693568, -12.43476213627227089 ) ) ;
#2434=CARTESIAN_POINT ( 'NONE',  ( 29.31840136419365450, 25.43085787977764056, -9.188101187500008038 ) ) ;
#2436=CARTESIAN_POINT ( 'NONE',  ( 79.40534888915426848, 47.81769003582009958, -13.62930039999817033 ) ) ;
#2438=CARTESIAN_POINT ( 'NONE',  ( 13.26084062165525523, 25.84336893147755276, -7.433330006724137462 ) ) ;
#2445=CARTESIAN_POINT ( 'NONE',  ( 86.50957498950597824, 47.24826369376732771, 10.71680696257866394 ) ) ;
#2448=CARTESIAN_POINT ( 'NONE',  ( 75.21948224091696034, 53.29821691096760361, 16.02883939873531105 ) ) ;
#2450=CARTESIAN_POINT ( 'NONE',  ( 82.12724052554919751, 54.15063765581061972, 15.62772812625948582 ) ) ;
#2455=EDGE_LOOP ( 'NONE', ( #48973, #51200, #92435, #11325 ) ) ;
#2458=CARTESIAN_POINT ( 'NONE',  ( 72.50318959249285911, 71.67715071215087619, 6.033079537162470807 ) ) ;
#2462=ORIENTED_EDGE ( 'NONE', *, *, #78688, .F. ) ;
#2464=CARTESIAN_POINT ( 'NONE',  ( 28.76090768559789979, 38.64646525600391413, -2.839279412974133887 ) ) ;
#2465=CARTESIAN_POINT ( 'NONE',  ( 80.08281979147555774, 44.31827980528016298, 11.46924030742146883 ) ) ;
#2466=CARTESIAN_POINT ( 'NONE',  ( 74.95832312740790826, 66.37231070943815325, -13.09348500807924509 ) ) ;
#2467=CARTESIAN_POINT ( 'NONE',  ( 82.43495555929192165, 48.51766243573657533, -13.06424617837711644 ) ) ;
#2473=CARTESIAN_POINT ( 'NONE',  ( 67.63749347275029322, 65.82635250199255950, 10.53419884080181035 ) ) ;
#2474=CARTESIAN_POINT ( 'NONE',  ( 87.85430303351097336, 43.89859490532884223, 0.3596698246726173775 ) ) ;
#2484=CARTESIAN_POINT ( 'NONE',  ( 78.08890065365325484, 61.45839965263433413, -16.15943835942215756 ) ) ;
#2488=CARTESIAN_POINT ( 'NONE',  ( 80.44297273222078104, 44.73620253183693762, -11.65665792485825669 ) ) ;
#2491=CARTESIAN_POINT ( 'NONE',  ( 82.41630873631589793, 41.31828431233920895, -3.367117793111288560 ) ) ;
#2492=CARTESIAN_POINT ( 'NONE',  ( 78.95335204094531889, 48.73056600144941086, -14.23687683951352412 ) ) ;
#2495=ORIENTED_EDGE ( 'NONE', *, *, #3717, .T. ) ;
#2499=B_SPLINE_SURFACE_WITH_KNOTS ( 'NONE', 3, 1, ( 
 ( #45972, #76888 ),
 ( #63193, #69789 ),
 ( #8994, #39865 ),
 ( #399, #85030 ),
 ( #46479, #46998 ),
 ( #99712, #84538 ),
 ( #53584, #94134 ),
 ( #31287, #15083 ),
 ( #70802, #16094 ),
 ( #77409, #8014 ),
 ( #38886, #54569 ),
 ( #62174, #77912 ),
 ( #93126, #38381 ),
 ( #8501, #1411 ),
 ( #32292, #30804 ),
 ( #68788, #85553 ),
 ( #39371, #70285 ),
 ( #24690, #55572 ),
 ( #897, #7488 ),
 ( #86556, #62679 ),
 ( #93632, #24199 ),
 ( #69294, #55080 ),
 ( #61684, #17088 ),
 ( #76420, #61186 ),
 ( #6992, #92634 ),
 ( #30301, #23183 ),
 ( #54075, #37877 ),
 ( #56589, #2414 ),
 ( #17596, #33292 ),
 ( #63697, #95145 ),
 ( #25710, #95655 ) ),
 .UNSPECIFIED., .F., .F., .F.,
 ( 4, 3, 3, 3, 3, 3, 3, 3, 3, 3, 4 ),
 ( 2, 2 ),
 ( 0.000000000000000000, 0.1122669598086765003, 0.2243161639709622401, 0.3396355846219112906, 0.4553962076585172380, 0.5677860799922342938, 0.6749047109689697566, 0.7773884377078434937, 0.8775581155834070168, 0.9782364162377823469, 1.000000000000000000 ),
 ( 0.000000000000000000, 1.000000000000000000 ),
 .UNSPECIFIED. ) ;
#2504=CARTESIAN_POINT ( 'NONE',  ( 71.61522850875250867, 69.38231080192815625, -8.322070056553526385 ) ) ;
#2505=CARTESIAN_POINT ( 'NONE',  ( 87.76310869853918462, 45.07707962072153407, -6.704660406813174767 ) ) ;
#2507=CARTESIAN_POINT ( 'NONE',  ( 88.26308438319264837, 44.34169033064829080, 4.149168146237482091 ) ) ;
#2508=VERTEX_POINT ( 'NONE', #48265 ) ;
#2514=ADVANCED_FACE ( 'NONE', ( #86321 ), #71585, .T. ) ;
#2521=CYLINDRICAL_SURFACE ( 'NONE', #94827, 10.00000000000001066 ) ;
#2523=CARTESIAN_POINT ( 'NONE',  ( 77.95656630038031665, 61.79485276963480089, 16.07049939491896851 ) ) ;
#2527=ORIENTED_EDGE ( 'NONE', *, *, #11654, .T. ) ;
#2533=CARTESIAN_POINT ( 'NONE',  ( 36.78662229117171734, 22.20801979619930933, -3.090169943749474069 ) ) ;
#2542=CARTESIAN_POINT ( 'NONE',  ( 81.86138060899043012, 46.81554957853204968, 12.09595161180856060 ) ) ;
#2545=LINE ( 'NONE', #70423, #19259 ) ;
#2546=CARTESIAN_POINT ( 'NONE',  ( 71.95319803722021845, 72.64445964553972601, -0.8526933041427806614 ) ) ;
#2549=CARTESIAN_POINT ( 'NONE',  ( 29.86737195101774844, 39.01751292744058475, 6.180339887498949913 ) ) ;
#2554=CARTESIAN_POINT ( 'NONE',  ( 73.34023794504622629, 66.76775327374055280, 12.61468185384920559 ) ) ;
#2555=CARTESIAN_POINT ( 'NONE',  ( 81.55798275936130892, 41.98492694272253800, 7.594723423486053449 ) ) ;
#2557=CARTESIAN_POINT ( 'NONE',  ( 83.61138909378800577, 52.00041238365412255, 15.00249647689079247 ) ) ;
#2559=( BOUNDED_CURVE ( )  B_SPLINE_CURVE ( 2, ( #99215, #23184, #22201, #45486, #53095, #99713, #69295 ),
 .UNSPECIFIED., .F., .T. ) 
 B_SPLINE_CURVE_WITH_KNOTS ( ( 3, 2, 2, 3 ),
 ( 0.000000000000000000, 0.005000000000000000104, 0.01000000000000000021, 0.01250000000000000243 ),
 .UNSPECIFIED. ) 
 CURVE ( )  GEOMETRIC_REPRESENTATION_ITEM ( )  RATIONAL_B_SPLINE_CURVE ( ( 1.000000000000000000, 0.9510565162951535312, 1.000000000000000000, 0.9510565162951535312, 1.000000000000000000, 0.9755282581475768211, 0.9755282581475768211 ) ) 
 REPRESENTATION_ITEM ( '' )  );
#2560=CARTESIAN_POINT ( 'NONE',  ( 70.52080361708803480, 66.70997956558090891, -10.64257139366791449 ) ) ;
#2561=CARTESIAN_POINT ( 'NONE',  ( 28.94742091202107304, 40.21091486745862653, 7.012934429366973338E-14 ) ) ;
#2570=CARTESIAN_POINT ( 'NONE',  ( 82.80564809338142140, 40.64392876451550762, -1.326136484204851973 ) ) ;
#2571=CARTESIAN_POINT ( 'NONE',  ( 66.06214068257196459, 68.71579393632853794, -0.4716098740908659659 ) ) ;
#2572=CARTESIAN_POINT ( 'NONE',  ( 85.64506726322308339, 45.94279376922860791, -9.832067947323890778 ) ) ;
#2573=CARTESIAN_POINT ( 'NONE',  ( 22.20737081713591010, 33.79752408145593279, -5.678558825948271327 ) ) ;
#2579=CARTESIAN_POINT ( 'NONE',  ( 11.83670304002995444, 9.760047579820874120, 5.678558825948272215 ) ) ;
#2584=CARTESIAN_POINT ( 'NONE',  ( 72.23967728755036433, 71.11445379834010794, -6.005443314427597379 ) ) ;
#2585=CARTESIAN_POINT ( 'NONE',  ( 85.04377965201177858, 48.84687674572034410, 12.36303725827022149 ) ) ;
#2587=LINE ( 'NONE', #33473, #33463 ) ;
#2595=CARTESIAN_POINT ( 'NONE',  ( 72.74059857843660382, 57.24590185972273559, -15.87550358816797136 ) ) ;
#2596=CARTESIAN_POINT ( 'NONE',  ( 76.69221233506321767, 63.60975152925200859, 15.32791472565302016 ) ) ;
#2605=CARTESIAN_POINT ( 'NONE',  ( 29.48198420892518357, 37.99752408145594273, 5.678558825948277544 ) ) ;
#2607=CARTESIAN_POINT ( 'NONE',  ( 78.53400660641976572, 48.00963154751628537, -13.98445158027483259 ) ) ;
#2609=CARTESIAN_POINT ( 'NONE',  ( 74.10605571268695257, 68.62492193873490010, 11.45106078344676526 ) ) ;
#2616=CARTESIAN_POINT ( 'NONE',  ( 84.43521566569499726, 42.96028256297638137, -5.024410855636625151 ) ) ;
#2621=CARTESIAN_POINT ( 'NONE',  ( 67.32255408704899935, 69.10951546266757362, -3.098682020105078649 ) ) ;
#2623=CARTESIAN_POINT ( 'NONE',  ( 82.02303788424785580, 52.21633268006980444, -15.43096719693068586 ) ) ;
#2628=CARTESIAN_POINT ( 'NONE',  ( 86.32721218574307898, 47.55264674982593931, -11.12316258729872054 ) ) ;
#2632=CARTESIAN_POINT ( 'NONE',  ( 87.33262174781505394, 44.32265804349968619, -4.467604021659223434 ) ) ;
#2633=CARTESIAN_POINT ( 'NONE',  ( 84.59927265645079331, 42.67612751815072869, 3.880141412610480955 ) ) ;
#2638=CARTESIAN_POINT ( 'NONE',  ( 83.80076462262509551, 51.77978008689729705, -14.86347872566931549 ) ) ;
#2640=CARTESIAN_POINT ( 'NONE',  ( 80.47503692277169307, 57.63887959601478883, -16.59359448248663682 ) ) ;
#2648=DIRECTION ( 'NONE',  ( 0.8660254037844379305, 0.5000000000000014433, 0.000000000000000000 ) ) ;
#2650=CARTESIAN_POINT ( 'NONE',  ( 85.51230132848702681, 48.33290926536287913, -12.21747540207229932 ) ) ;
#2659=CARTESIAN_POINT ( 'NONE',  ( 78.71885683147529278, 52.51053486998128506, -15.59668387851618476 ) ) ;
#2666=CARTESIAN_POINT ( 'NONE',  ( 16.38795500122288473, 25.16454794089041513, -10.00000000000000355 ) ) ;
#2673=CARTESIAN_POINT ( 'NONE',  ( 1.874387969441054569, 24.58029201028039168, 1.583844403245364241 ) ) ;
#2685=CARTESIAN_POINT ( 'NONE',  ( 40.97001837269192492, 24.44966523072497822, -2.296566073217252530E-15 ) ) ;
#2689=CARTESIAN_POINT ( 'NONE',  ( 31.10096393961467598, 36.14336893147757479, 7.433330006724141015 ) ) ;
#2693=CARTESIAN_POINT ( 'NONE',  ( 40.24855657362158468, 31.43677371833804912, -10.00000000000000355 ) ) ;
#2695=CARTESIAN_POINT ( 'NONE',  ( 16.39654754030849659, 10.26216523072493203, -2.296566073217252530E-15 ) ) ;
#2697=CARTESIAN_POINT ( 'NONE',  ( 23.10163885443276754, 15.19860640527292261, 2.839279412974134775 ) ) ;
#2710=CARTESIAN_POINT ( 'NONE',  ( 66.25740745690036704, 68.21673160025993354, 4.121950718744524345 ) ) ;
#2711=CARTESIAN_POINT ( 'NONE',  ( 87.85893154554855755, 45.08040635541047436, 6.601944857759015406 ) ) ;
#2716=CARTESIAN_POINT ( 'NONE',  ( 86.54431918921495992, 47.23684621844409293, 10.68448168089783756 ) ) ;
#2717=EDGE_LOOP ( 'NONE', ( #33273, #74366, #47400, #87529 ) ) ;
#2718=CARTESIAN_POINT ( 'NONE',  ( 77.90008039292268904, 58.37449120656814472, 16.15501551646137202 ) ) ;
#2722=CARTESIAN_POINT ( 'NONE',  ( 28.14208253200458287, 39.18080186712595037, 3.090169943749475401 ) ) ;
#2725=EDGE_CURVE ( 'NONE', #31346, #2508, #57850, .T. ) ;
#2731=VERTEX_POINT ( 'NONE', #90801 ) ;
#2739=LINE ( 'NONE', #56902, #44417 ) ;
#2741=CARTESIAN_POINT ( 'NONE',  ( 82.28003896795380001, 40.62557011406286733, -3.142018250819523129 ) ) ;
#2744=CARTESIAN_POINT ( 'NONE',  ( 71.79993839105814857, 70.08644720081231583, 7.366185827508974882 ) ) ;
#2746=CARTESIAN_POINT ( 'NONE',  ( 82.54140815357128247, 53.47864718817667296, -15.73643156343348615 ) ) ;
#2750=CARTESIAN_POINT ( 'NONE',  ( 25.69310950058096310, 17.76004757982090254, 5.678558825948272215 ) ) ;
#2758=ORIENTED_EDGE ( 'NONE', *, *, #49682, .F. ) ;
#2763=DIRECTION ( 'NONE',  ( 0.03487823687205911238, -0.06041087834082882468, 0.9975640502598247528 ) ) ;
#2774=CARTESIAN_POINT ( 'NONE',  ( 82.68332475418115735, 40.58172727773597899, -1.414306879930183003 ) ) ;
#2786=EDGE_CURVE ( 'NONE', #42053, #90329, #81164, .T. ) ;
#2788=EDGE_CURVE ( 'NONE', #19489, #21672, #32129, .T. ) ;
#2789=CARTESIAN_POINT ( 'NONE',  ( 68.71788151997813543, 70.18350386356217996, 1.720494083608670843 ) ) ;
#2790=AXIS2_PLACEMENT_3D ( 'NONE', #51162, #80630, #11206 ) ;
#2794=CARTESIAN_POINT ( 'NONE',  ( 68.80540557632873799, 64.07494415132596544, 12.03686799599169888 ) ) ;
#2799=CARTESIAN_POINT ( 'NONE',  ( 82.66344616542426138, 44.30278114141059831, 9.141997255372078968 ) ) ;
#2802=CARTESIAN_POINT ( 'NONE',  ( 69.10645821515414866, 64.33862435200268237, -11.96736273993547961 ) ) ;
#2806=CARTESIAN_POINT ( 'NONE',  ( 72.70941816336303987, 68.00343649803248525, -11.28160401705123306 ) ) ;
#2814=CARTESIAN_POINT ( 'NONE',  ( 24.72364882272980324, 19.98920272979926693, 7.433330006724137462 ) ) ;
#2820=VERTEX_POINT ( 'NONE', #28959 ) ;
#2826=CARTESIAN_POINT ( 'NONE',  ( 81.59257867409928622, 55.89534513097626700, -16.02158239418033503 ) ) ;
#2832=CARTESIAN_POINT ( 'NONE',  ( 72.12312422658187927, 72.33562412997507352, 0.9419202200955228976 ) ) ;
#2835=CARTESIAN_POINT ( 'NONE',  ( 83.60735424973495356, 51.47225398191811507, -14.39433507971101278 ) ) ;
#2836=CARTESIAN_POINT ( 'NONE',  ( 71.25277716278617390, 71.82511101822419164, -0.9037114356811193350 ) ) ;
#2840=CARTESIAN_POINT ( 'NONE',  ( 14.09675671201943992, 9.108019796199272378, 3.090169943749476733 ) ) ;
#2843=CARTESIAN_POINT ( 'NONE',  ( 78.20977235749720080, 61.70939135586247204, 16.12143617465002166 ) ) ;
#2847=EDGE_CURVE ( 'NONE', #31137, #38635, #21356, .T. ) ;
#2848=CARTESIAN_POINT ( 'NONE',  ( 79.12311323331778112, 59.82187722400571062, 16.49858871944914540 ) ) ;
#2850=CARTESIAN_POINT ( 'NONE',  ( 88.28491662655248717, 43.90562524633402575, -2.137378875048265403 ) ) ;
#2856=ADVANCED_FACE ( 'NONE', ( #60323 ), #21845, .T. ) ;
#2859=ADVANCED_FACE ( 'NONE', ( #54721 ), #40018, .T. ) ;
#2868=CARTESIAN_POINT ( 'NONE',  ( 82.15643586640744900, 40.65243239225524974, 3.555191510540661071 ) ) ;
#2873=CARTESIAN_POINT ( 'NONE',  ( 87.00377149549910882, 43.01292419151745605, -0.4974700842552756685 ) ) ;
#2877=CARTESIAN_POINT ( 'NONE',  ( 75.37843707191279918, 53.50823561223473490, 16.04097401286667335 ) ) ;
#2878=ORIENTED_EDGE ( 'NONE', *, *, #11365, .F. ) ;
#2879=CARTESIAN_POINT ( 'NONE',  ( 31.10880476808887352, 18.36477965099641096, 1.583844403245330712 ) ) ;
#2890=CARTESIAN_POINT ( 'NONE',  ( 76.32868100360434482, 51.65245485454531860, -16.17077658888306857 ) ) ;
#2895=CARTESIAN_POINT ( 'NONE',  ( 66.22186792372609432, 68.80901709827284662, 0.1133511356784482477 ) ) ;
#2896=EDGE_LOOP ( 'NONE', ( #21191, #88784, #5315, #91705 ) ) ;
#2898=PLANE ( 'NONE',  #3113 ) ;
#2899=EDGE_CURVE ( 'NONE', #63730, #72252, #75026, .T. ) ;
#2908=ORIENTED_EDGE ( 'NONE', *, *, #44734, .F. ) ;
#2909=CARTESIAN_POINT ( 'NONE',  ( 70.01283242295176024, 62.80173547756309915, -13.36538303052352283 ) ) ;
#2910=ADVANCED_FACE ( 'NONE', ( #3559 ), #18753, .T. ) ;
#2912=CARTESIAN_POINT ( 'NONE',  ( 70.18173327330886480, 66.19638441240277871, -10.95949337109657762 ) ) ;
#2915=CARTESIAN_POINT ( 'NONE',  ( 80.62087421845698998, 43.38634220051089585, -9.432027624119850628 ) ) ;
#2916=CARTESIAN_POINT ( 'NONE',  ( 69.27034135246833557, 70.64205536240437766, -0.1784889401922611085 ) ) ;
#2926=CARTESIAN_POINT ( 'NONE',  ( 81.59425157384957572, 59.39892931189028502, 0.4045084971874712831 ) ) ;
#2931=CARTESIAN_POINT ( 'NONE',  ( 76.52674025845067263, 55.63219038539143924, -16.16525125865949164 ) ) ;
#2934=CARTESIAN_POINT ( 'NONE',  ( 73.52963229642551823, 69.81563172817719476, 9.291775542480344541 ) ) ;
#2937=CARTESIAN_POINT ( 'NONE',  ( 76.67567146729665239, 63.34086528488000312, -15.41964329106466103 ) ) ;
#2938=EDGE_CURVE ( 'NONE', #92910, #45021, #93153, .T. ) ;
#2947=CARTESIAN_POINT ( 'NONE',  ( 34.12723495145388597, 35.10171378149922816, 9.188101187500008038 ) ) ;
#2948=CARTESIAN_POINT ( 'NONE',  ( 82.78961024920913303, 51.80492193425784819, 15.12833883139485636 ) ) ;
#2951=CARTESIAN_POINT ( 'NONE',  ( 11.39049277451480080, 29.68290643055186706, 3.479690158560446702E-15 ) ) ;
#2953=LINE ( 'NONE', #20500, #70774 ) ;
#2960=CARTESIAN_POINT ( 'NONE',  ( 72.16246046514868340, 71.47350907076796034, 5.042997787714098124 ) ) ;
#2963=CARTESIAN_POINT ( 'NONE',  ( 74.72784533871833901, 53.57696346259629649, 16.08082742858022129 ) ) ;
#2975=CARTESIAN_POINT ( 'NONE',  ( 72.09527832497458633, 71.67135281093830201, 5.495264124482682533 ) ) ;
#2979=ORIENTED_EDGE ( 'NONE', *, *, #57729, .F. ) ;
#2980=CARTESIAN_POINT ( 'NONE',  ( 27.02885687802902837, 37.64646525600391413, -2.839279412974133887 ) ) ;
#2981=CARTESIAN_POINT ( 'NONE',  ( 79.78397074742090922, 49.18318286717641286, -14.22441051831706460 ) ) ;
#2982=CARTESIAN_POINT ( 'NONE',  ( 79.11275361910446691, 46.11146926033848814, 13.27945046499837112 ) ) ;
#2983=ADVANCED_FACE ( 'NONE', ( #20247 ), #43009, .T. ) ;
#2986=ORIENTED_EDGE ( 'NONE', *, *, #68263, .F. ) ;
#2990=CARTESIAN_POINT ( 'NONE',  ( 68.23738887302573630, 65.53295183940775814, 10.45289023565593389 ) ) ;
#2992=CARTESIAN_POINT ( 'NONE',  ( 85.29796244568555608, 48.43343408700369679, 12.39349753750686034 ) ) ;
#2999=CARTESIAN_POINT ( 'NONE',  ( 79.22635074364777097, 59.80166750096645245, 16.50638431802919470 ) ) ;
#3005=ORIENTED_EDGE ( 'NONE', *, *, #44476, .T. ) ;
#3008=CARTESIAN_POINT ( 'NONE',  ( 32.64838280634442214, 30.80066082961423746, 10.00000000000000533 ) ) ;
#3010=DIRECTION ( 'NONE',  ( 0.9532659690011952014, -0.2314883312386644132, -0.1941575258509203872 ) ) ;
#3014=ORIENTED_EDGE ( 'NONE', *, *, #73824, .F. ) ;
#3018=CARTESIAN_POINT ( 'NONE',  ( 75.98901751930753790, 65.25029023645535631, -14.46192986472697584 ) ) ;
#3020=CARTESIAN_POINT ( 'NONE',  ( 69.59202289449447676, 69.33098532997668428, -6.332424716581326329 ) ) ;
#3023=CARTESIAN_POINT ( 'NONE',  ( 87.53579730927835101, 44.58748639555269477, 4.920146826978176513 ) ) ;
#3032=CARTESIAN_POINT ( 'NONE',  ( 81.13608137687064925, 42.60696278352305200, 7.988320930663086905 ) ) ;
#3033=ADVANCED_BREP_SHAPE_REPRESENTATION ( '', ( #9388, #68784 ), #26785 ) ;
#3038=CARTESIAN_POINT ( 'NONE',  ( 83.13802928724584262, 52.17454805837402176, 14.80588059101579645 ) ) ;
#3048=CARTESIAN_POINT ( 'NONE',  ( 28.38430345058481308, 38.16126292948897714, -6.180339887498951690 ) ) ;
#3053=CARTESIAN_POINT ( 'NONE',  ( 81.88482396345729342, 43.19773723414667188, -8.246544634686086894 ) ) ;
#3056=CARTESIAN_POINT ( 'NONE',  ( 81.05870138697780192, 44.81917051076717939, 10.73315104669606512 ) ) ;
#3060=CARTESIAN_POINT ( 'NONE',  ( 14.27891468289787191, 30.01751292744055633, 6.180339887498949913 ) ) ;
#3061=CARTESIAN_POINT ( 'NONE',  ( 72.09830524877247626, 72.30916584571114925, -0.9965686167420374497 ) ) ;
#3066=CARTESIAN_POINT ( 'NONE',  ( 31.25301259707286050, 39.81751292744058901, -6.180339887498951690 ) ) ;
#3074=CARTESIAN_POINT ( 'NONE',  ( 83.37296956034944628, 51.74080471427829764, 14.95189368521466733 ) ) ;
#3079=ORIENTED_EDGE ( 'NONE', *, *, #9028, .T. ) ;
#3088=CARTESIAN_POINT ( 'NONE',  ( 29.87828763904599683, 19.11110640527293469, -2.839279412974138328 ) ) ;
#3093=CARTESIAN_POINT ( 'NONE',  ( 15.46319120177094142, 20.87878583063840665, -9.188101187500006262 ) ) ;
#3113=AXIS2_PLACEMENT_3D ( 'NONE', #32758, #10474, #42348 ) ;
#3115=CARTESIAN_POINT ( 'NONE',  ( 72.99394114207360929, 57.42839372474189474, -15.86952975956620193 ) ) ;
#3116=CARTESIAN_POINT ( 'NONE',  ( 78.36638819403545142, 61.52197373328140628, -15.82278474554905578 ) ) ;
#3125=CARTESIAN_POINT ( 'NONE',  ( 30.86762485498029207, 38.79752408145593989, -5.678558825948271327 ) ) ;
#3127=CARTESIAN_POINT ( 'NONE',  ( 78.14223614238626681, 47.72510913427617396, -13.95591167936428612 ) ) ;
#3129=CARTESIAN_POINT ( 'NONE',  ( 73.79815732168846409, 68.46225211080071915, 10.93730676814644553 ) ) ;
#3133=EDGE_LOOP ( 'NONE', ( #72550, #571, #30596, #36949 ) ) ;
#3136=CARTESIAN_POINT ( 'NONE',  ( 78.70624514232692093, 57.96118622721134983, 16.60064729657024074 ) ) ;
#3149=CARTESIAN_POINT ( 'NONE',  ( 84.12081806601244693, 44.16637391680080782, -7.839909042555411212 ) ) ;
#3150=CARTESIAN_POINT ( 'NONE',  ( 83.43076169397228625, 41.65753570452999099, 2.225996872481429190 ) ) ;
#3154=DIRECTION ( 'NONE',  ( 0.9364604334398946017, -0.2023802897980881699, 0.2865031848039507056 ) ) ;
#3156=CARTESIAN_POINT ( 'NONE',  ( 80.24454609401104221, 57.41156006636176556, -16.59009416930489422 ) ) ;
#3167=CARTESIAN_POINT ( 'NONE',  ( 21.02495994229494514, 13.10801979619928304, 3.090169943749476733 ) ) ;
#3170=DIRECTION ( 'NONE',  ( -0.8660254037844361541, -0.5000000000000042188, 0.000000000000000000 ) ) ;
#3173=( BOUNDED_CURVE ( )  B_SPLINE_CURVE ( 2, ( #35403, #88672, #19246, #67297, #97243, #96753, #58203, #20722, #43983, #50596, #35899, #90145, #51607 ),
 .UNSPECIFIED., .F., .T. ) 
 B_SPLINE_CURVE_WITH_KNOTS ( ( 3, 2, 2, 2, 2, 2, 3 ),
 ( 0.1125000000000000028, 0.1150000000000000050, 0.1199999999999999956, 0.1250000000000000000, 0.1300000000000000044, 0.1350000000000000089, 0.1375000000000000111 ),
 .UNSPECIFIED. ) 
 CURVE ( )  GEOMETRIC_REPRESENTATION_ITEM ( )  RATIONAL_B_SPLINE_CURVE ( ( 0.9755282581475768211, 0.9755282581475768211, 1.000000000000000000, 0.9510565162951535312, 1.000000000000000000, 0.9510565162951535312, 1.000000000000000000, 0.9510565162951535312, 1.000000000000000000, 0.9510565162951535312, 1.000000000000000000, 0.9755282581475768211, 0.9755282581475768211 ) ) 
 REPRESENTATION_ITEM ( '' )  );
#3175=CARTESIAN_POINT ( 'NONE',  ( 76.43834045353088413, 53.21192047009603954, -15.94639307102674586 ) ) ;
#3180=B_SPLINE_CURVE_WITH_KNOTS ( 'NONE', 3,
 ( #99700, #14095, #46466, #54064, #85019, #44475, #91130, #75917, #22695, #5992 ),
 .UNSPECIFIED., .F., .F.,
 ( 4, 2, 2, 2, 4 ),
 ( 0.000000000000000000, 0.0002622400424272788768, 0.0005244800848545577536, 0.0007867201272818366304, 0.001048960169709115507 ),
 .UNSPECIFIED. ) ;
#3185=CARTESIAN_POINT ( 'NONE',  ( 26.76913962382671031, 17.58380873178787951, 6.180339887498953466 ) ) ;
#3187=CARTESIAN_POINT ( 'NONE',  ( 66.22544472841278207, 69.36168339246577830, 0.1681495645362227065 ) ) ;
#3190=CARTESIAN_POINT ( 'NONE',  ( 73.89341774252514483, 54.96439960668192981, -16.13050749448415289 ) ) ;
#3196=AXIS2_PLACEMENT_3D ( 'NONE', #73864, #72891, #65255 ) ;
#3201=CARTESIAN_POINT ( 'NONE',  ( 40.59535201087842182, 25.29860640527295601, -2.839279412974138328 ) ) ;
#3204=CARTESIAN_POINT ( 'NONE',  ( 29.80674373534435162, 38.18502408145592852, 5.678558825948277544 ) ) ;
#3205=CARTESIAN_POINT ( 'NONE',  ( 75.31289280905393468, 53.62176160565092431, -16.53289957284814093 ) ) ;
#3209=CARTESIAN_POINT ( 'NONE',  ( 4.886862741447147940, 23.79752408145590081, -5.678558825948271327 ) ) ;
#3211=CARTESIAN_POINT ( 'NONE',  ( 21.36958804686389612, 14.19860640527291906, 2.839279412974134775 ) ) ;
#3218=ORIENTED_EDGE ( 'NONE', *, *, #62509, .F. ) ;
#3220=CARTESIAN_POINT ( 'NONE',  ( 66.10853026158757473, 68.52245927072395659, 4.666879336207867546 ) ) ;
#3221=CARTESIAN_POINT ( 'NONE',  ( 87.62713558190685603, 45.48188874142729787, 6.789248154466972274 ) ) ;
#3223=ORIENTED_EDGE ( 'NONE', *, *, #23057, .T. ) ;
#3225=CARTESIAN_POINT ( 'NONE',  ( 86.35455787144825024, 47.24910468700996091, 10.80869237663237570 ) ) ;
#3226=ORIENTED_EDGE ( 'NONE', *, *, #91621, .T. ) ;
#3230=CARTESIAN_POINT ( 'NONE',  ( 78.32967510012902324, 61.10706999557027075, -15.90745784467399382 ) ) ;
#3233=CARTESIAN_POINT ( 'NONE',  ( 19.55501378379531019, 16.45404122711132899, -8.090169943749478065 ) ) ;
#3241=EDGE_LOOP ( 'NONE', ( #64627, #79209, #100249, #86032 ) ) ;
#3249=CARTESIAN_POINT ( 'NONE',  ( 69.97819147249884963, 66.34545571799995400, 10.67815867109653638 ) ) ;
#3250=LINE ( 'NONE', #26535, #30696 ) ;
#3256=CARTESIAN_POINT ( 'NONE',  ( 22.95008440877049338, 15.11110640527292226, -2.839279412974138328 ) ) ;
#3262=CARTESIAN_POINT ( 'NONE',  ( 69.40440858250356371, 62.73539878346245757, 13.77383303921267377 ) ) ;
#3275=FACE_OUTER_BOUND ( 'NONE', #67716, .T. ) ;
#3286=CARTESIAN_POINT ( 'NONE',  ( 88.30098027080434520, 44.15648434567072655, 0.4058311546344762766 ) ) ;
#3290=CARTESIAN_POINT ( 'NONE',  ( 68.55513178119723250, 64.39780669069259034, 11.67030924314737206 ) ) ;
#3296=CARTESIAN_POINT ( 'NONE',  ( 82.18584245047638603, 43.47170607935511555, 8.378381801397722484 ) ) ;
#3299=CARTESIAN_POINT ( 'NONE',  ( 68.82157586999431942, 64.23696645290118568, -11.91704851694915135 ) ) ;
#3301=DIRECTION ( 'NONE',  ( 0.2503889871761774688, 0.9681453171404013069, 0.000000000000000000 ) ) ;
#3303=DIRECTION ( 'NONE',  ( -1.000000000000000000, 0.000000000000000000, 0.000000000000000000 ) ) ;
#3307=EDGE_CURVE ( 'NONE', #70075, #55525, #71850, .T. ) ;
#3311=LINE ( 'NONE', #43763, #61127 ) ;
#3313=CARTESIAN_POINT ( 'NONE',  ( 22.55376741186237055, 15.94754757982089544, 5.678558825948272215 ) ) ;
#3314=CARTESIAN_POINT ( 'NONE',  ( 74.95681149046626501, 67.19672641238656752, 12.53511022654090290 ) ) ;
#3318=CARTESIAN_POINT ( 'NONE',  ( 22.49293824011677856, 13.39040679176982707, 1.333680081654574804E-15 ) ) ;
#3324=CARTESIAN_POINT ( 'NONE',  ( 81.44563236102617054, 56.14986361120382696, -16.42609089136781364 ) ) ;
#3326=CARTESIAN_POINT ( 'NONE',  ( 73.41722143124820832, 65.21547532963855076, -13.68388213405907194 ) ) ;
#3331=CARTESIAN_POINT ( 'NONE',  ( 71.92952260767445694, 72.55458961131338924, 1.705568256100856273 ) ) ;
#3333=CARTESIAN_POINT ( 'NONE',  ( 83.85849937899710937, 52.02177296427104380, -14.56386478986045496 ) ) ;
#3340=CARTESIAN_POINT ( 'NONE',  ( 1.572689338377429191, 25.00034080476287457, -1.878358725466461243E-16 ) ) ;
#3347=ORIENTED_EDGE ( 'NONE', *, *, #35077, .F. ) ;
#3348=CARTESIAN_POINT ( 'NONE',  ( 79.22635074364777097, 59.80166750096645245, 16.50638431802919825 ) ) ;
#3351=CARTESIAN_POINT ( 'NONE',  ( 77.21081030551935953, 52.27152845490210353, -15.72840955207014879 ) ) ;
#3353=CARTESIAN_POINT ( 'NONE',  ( 81.47460321488800616, 41.92273497686812789, -7.570820128221508405 ) ) ;
#3360=DIRECTION ( 'NONE',  ( -0.8660254037844379305, -0.5000000000000014433, -0.000000000000000000 ) ) ;
#3363=CARTESIAN_POINT ( 'NONE',  ( 74.25393038840245197, 55.45593832152543712, 16.12141555578006091 ) ) ;
#3365=ORIENTED_EDGE ( 'NONE', *, *, #21554, .T. ) ;
#3366=CARTESIAN_POINT ( 'NONE',  ( 82.30911433263591448, 41.22987874057414359, 3.253666625269970858 ) ) ;
#3370=B_SPLINE_CURVE_WITH_KNOTS ( 'NONE', 3,
 ( #69167, #62047, #37765, #84910, #75806, #29196, #14963, #15453, #93000, #38252, #45368, #36776, #6390, #46351, #31158, #76774 ),
 .UNSPECIFIED., .F., .F.,
 ( 4, 1, 2, 2, 2, 1, 2, 2, 4 ),
 ( 0.000000000000000000, 0.1249999999999972800, 0.1874999999999960310, 0.2499999999999947820, 0.4999999999999953371, 0.6249999999999955591, 0.6874999999999958922, 0.7499999999999961142, 1.000000000000000000 ),
 .UNSPECIFIED. ) ;
#3371=FACE_OUTER_BOUND ( 'NONE', #26021, .T. ) ;
#3377=CARTESIAN_POINT ( 'NONE',  ( 36.18707552304946518, 42.93396525600392977, 2.839279412974139660 ) ) ;
#3380=VERTEX_POINT ( 'NONE', #64739 ) ;
#3383=CARTESIAN_POINT ( 'NONE',  ( 76.27979237450192329, 64.97140225463311936, -14.28508825889822376 ) ) ;
#3388=CARTESIAN_POINT ( 'NONE',  ( 68.91022223105564137, 64.71151235087043574, -12.22836756590942997 ) ) ;
#3396=CARTESIAN_POINT ( 'NONE',  ( 81.27257538021680716, 44.83877995622705726, -10.61750955095084592 ) ) ;
#3399=CARTESIAN_POINT ( 'NONE',  ( 88.26624674143728555, 44.30546972661463911, 2.125762532784985837 ) ) ;
#3404=CARTESIAN_POINT ( 'NONE',  ( 80.26979669126045280, 58.08567880715743570, 16.26339599281328674 ) ) ;
#3408=CARTESIAN_POINT ( 'NONE',  ( 80.84396924949311369, 43.27153703455048372, -9.948315819065333798 ) ) ;
#3418=DIRECTION ( 'NONE',  ( -0.8660254037844379305, -0.5000000000000014433, -0.000000000000000000 ) ) ;
#3425=CARTESIAN_POINT ( 'NONE',  ( 82.03542799465949997, 53.49766676369745255, -15.45754095158874186 ) ) ;
#3428=CARTESIAN_POINT ( 'NONE',  ( 77.07149570696485341, 63.73492570656748057, -15.36167024187155228 ) ) ;
#3431=CARTESIAN_POINT ( 'NONE',  ( 87.73298548431468191, 44.18903561216112763, 4.633618514853090176 ) ) ;
#3436=CARTESIAN_POINT ( 'NONE',  ( 30.58134869734400851, 35.84336893147758474, -7.433330006724137462 ) ) ;
#3437=CARTESIAN_POINT ( 'NONE',  ( 77.56105267981614304, 49.72783448595330924, -15.46007777815280981 ) ) ;
#3440=CARTESIAN_POINT ( 'NONE',  ( 22.90017757337614768, 16.14754757982090183, -5.678558825948276656 ) ) ;
#3445=CARTESIAN_POINT ( 'NONE',  ( 86.61846192408904699, 47.19909516036467068, 10.60101820161781561 ) ) ;
#3446=CARTESIAN_POINT ( 'NONE',  ( 72.04811769650321196, 71.35602353065118564, 5.168332083721268511 ) ) ;
#3451=CARTESIAN_POINT ( 'NONE',  ( 20.95177465265983585, 30.83478043621388665, -8.090169943749479842 ) ) ;
#3460=EDGE_CURVE ( 'NONE', #15274, #25562, #39990, .T. ) ;
#3463=EDGE_CURVE ( 'NONE', #86428, #91729, #26751, .T. ) ;
#3466=CARTESIAN_POINT ( 'NONE',  ( 83.95255218473330672, 50.75189519228615609, 14.35568035062530967 ) ) ;
#3469=CARTESIAN_POINT ( 'NONE',  ( 31.76492312988469280, 26.84335787977765264, 9.188101187500006262 ) ) ;
#3470=CARTESIAN_POINT ( 'NONE',  ( 82.71201993963725840, 48.44912912001353789, -12.92290741477395422 ) ) ;
#3475=VECTOR ( 'NONE', #70481, 1000.000000000000114 ) ;
#3480=CARTESIAN_POINT ( 'NONE',  ( 85.35443477132466228, 48.30880629543902671, -11.80360700664790663 ) ) ;
#3494=CARTESIAN_POINT ( 'NONE',  ( 87.20555836939593064, 45.98127448902955905, -8.722945138008007859 ) ) ;
#3506=CARTESIAN_POINT ( 'NONE',  ( 29.94731862920856358, 22.45404122711134676, -8.090169943749478065 ) ) ;
#3508=CARTESIAN_POINT ( 'NONE',  ( 70.90832346156993538, 69.40020835857261261, -7.639751975664101025 ) ) ;
#3510=CARTESIAN_POINT ( 'NONE',  ( 69.68654088143662761, 62.27729828303051107, -13.56154521557472314 ) ) ;
#3512=DIRECTION ( 'NONE',  ( -0.4556638457577291690, 0.000000000000000000, -0.8901519306664882336 ) ) ;
#3516=CARTESIAN_POINT ( 'NONE',  ( 81.96170391062356941, 40.98971803353019538, -3.100310559334822802 ) ) ;
#3519=CARTESIAN_POINT ( 'NONE',  ( 83.13520543127567919, 52.15262426605146118, 14.79738518802719049 ) ) ;
#3526=CARTESIAN_POINT ( 'NONE',  ( 83.50487366122874278, 51.96486753097844513, 15.01313857892666803 ) ) ;
#3533=CARTESIAN_POINT ( 'NONE',  ( 84.14312167556933275, 48.98415679381830756, 0.000000000000000000 ) ) ;
#3535=CARTESIAN_POINT ( 'NONE',  ( 38.93409909807770219, 22.28848085856233752, 1.475505719884397138E-15 ) ) ;
#3540=CARTESIAN_POINT ( 'NONE',  ( 87.21930977929280004, 43.81522300531741365, -2.732277708072506250 ) ) ;
#3541=ADVANCED_FACE ( 'NONE', ( #73107 ), #23429, .T. ) ;
#3545=CARTESIAN_POINT ( 'NONE',  ( 87.29394575703194903, 46.02912284201620707, 8.718719511823859847 ) ) ;
#3549=CARTESIAN_POINT ( 'NONE',  ( 87.37270799788964837, 45.80620788475513905, 8.330021955613661433 ) ) ;
#3551=CARTESIAN_POINT ( 'NONE',  ( 41.47628181354097165, 29.11029122506297995, -8.090169943749478065 ) ) ;
#3557=CARTESIAN_POINT ( 'NONE',  ( 83.37579341631962393, 51.76272850660086533, 14.96038908820327329 ) ) ;
#3559=FACE_OUTER_BOUND ( 'NONE', #16522, .T. ) ;
#3563=ORIENTED_EDGE ( 'NONE', *, *, #24551, .F. ) ;
#3566=CARTESIAN_POINT ( 'NONE',  ( 67.26028111370726492, 66.44647860927366878, -8.734192759284999497 ) ) ;
#3567=EDGE_LOOP ( 'NONE', ( #87993, #56635, #95728, #2527 ) ) ;
#3571=CARTESIAN_POINT ( 'NONE',  ( 24.12344523961532161, 25.87878583063842086, -9.188101187500006262 ) ) ;
#3572=CARTESIAN_POINT ( 'NONE',  ( 73.06604476908140100, 70.70555935200820841, -7.638416365798065044 ) ) ;
#3576=ORIENTED_EDGE ( 'NONE', *, *, #62774, .T. ) ;
#3577=CARTESIAN_POINT ( 'NONE',  ( 14.66813190280496570, 26.65586893147755276, -7.433330006724137462 ) ) ;
#3579=CARTESIAN_POINT ( 'NONE',  ( 77.77867966053455007, 61.43039905302717330, -16.12786080876373873 ) ) ;
#3580=EDGE_CURVE ( 'NONE', #75751, #55973, #71245, .T. ) ;
#3582=CARTESIAN_POINT ( 'NONE',  ( 71.99762221142530905, 71.50039512193581004, -5.770478025556951884 ) ) ;
#3585=CARTESIAN_POINT ( 'NONE',  ( 70.85892616739612038, 65.15884113644888487, -12.74389673638816944 ) ) ;
#3593=CARTESIAN_POINT ( 'NONE',  ( 71.92782195476812035, 71.87540567707925732, -4.706787814905536216 ) ) ;
#3594=CARTESIAN_POINT ( 'NONE',  ( 77.99937045744943021, 62.11896432438783933, -16.00068414206377554 ) ) ;
#3598=EDGE_CURVE ( 'NONE', #18179, #41317, #8430, .T. ) ;
#3603=CARTESIAN_POINT ( 'NONE',  ( 37.81746515356308436, 24.76004757982092741, 5.678558825948272215 ) ) ;
#3611=ORIENTED_EDGE ( 'NONE', *, *, #57154, .T. ) ;
#3613=CARTESIAN_POINT ( 'NONE',  ( 77.41840195283046455, 57.61794442662724691, -16.16528434754481580 ) ) ;
#3614=CARTESIAN_POINT ( 'NONE',  ( 88.05252050592584112, 44.08395231509391721, 3.677241261923597460 ) ) ;
#3616=DIRECTION ( 'NONE',  ( -0.8660254037844378194, -0.5000000000000013323, -0.000000000000000000 ) ) ;
#3618=B_SPLINE_CURVE_WITH_KNOTS ( 'NONE', 3,
 ( #52140, #13174, #65841, #44030, #82608, #74971, #36437, #66355, #67344, #75463, #98271, #28859, #90705, #34458, #26864, #88720, #42538, #73471, #4054, #29848, #30347, #52632, #45038, #15626, #7538, #69344, #60223, #15124, #77464, #6556, #60717, #93175, #46525, #22242, #45529, #53143, #83588, #61233, #37429, #47043, #68835, #31339, #46019, #38429, #30845, #61731 ),
 .UNSPECIFIED., .F., .F.,
 ( 4, 1, 2, 2, 1, 2, 2, 1, 1, 2, 2, 1, 1, 2, 2, 1, 1, 2, 2, 1, 1, 1, 2, 2, 1, 1, 1, 2, 2, 4 ),
 ( 0.000000000000000000, 0.06250000000000467681, 0.09375000000000667522, 0.1250000000000086875, 0.1875000000000168754, 0.2187500000000201505, 0.2500000000000234257, 0.3125000000000278111, 0.3437500000000300870, 0.3593750000000310307, 0.3750000000000320299, 0.4375000000000314748, 0.4687500000000301426, 0.4843750000000304201, 0.5000000000000306422, 0.5625000000000296430, 0.5937500000000290878, 0.6093750000000288658, 0.6250000000000285327, 0.6875000000000228706, 0.7187500000000199840, 0.7343750000000185407, 0.7421875000000177636, 0.7500000000000169864, 0.8125000000000105471, 0.8437500000000067724, 0.8593750000000044409, 0.8671875000000036637, 0.8750000000000029976, 1.000000000000000000 ),
 .UNSPECIFIED. ) ;
#3624=CARTESIAN_POINT ( 'NONE',  ( 71.41016749218992743, 59.45273978182970609, 15.69346469599747174 ) ) ;
#3635=CARTESIAN_POINT ( 'NONE',  ( 75.51323141522172477, 65.35427051582675517, 13.87231131232226744 ) ) ;
#3637=ORIENTED_EDGE ( 'NONE', *, *, #82056, .F. ) ;
#3638=CARTESIAN_POINT ( 'NONE',  ( 80.41409615687595647, 57.98253562157035645, -16.60360993379744343 ) ) ;
#3649=CARTESIAN_POINT ( 'NONE',  ( 13.69704499135956155, 32.00034080476289944, -1.878358725466461243E-16 ) ) ;
#3657=EDGE_CURVE ( 'NONE', #99249, #18043, #18277, .T. ) ;
#3658=CARTESIAN_POINT ( 'NONE',  ( 78.05914692549418987, 52.71672065815211994, -15.71920831139273211 ) ) ;
#3659=ORIENTED_EDGE ( 'NONE', *, *, #78524, .F. ) ;
#3667=CARTESIAN_POINT ( 'NONE',  ( 20.17205688044380452, 16.81029122506294371, 8.090169943749479842 ) ) ;
#3670=CARTESIAN_POINT ( 'NONE',  ( 72.02714983513547509, 72.27104924840581646, -3.542005090554713576 ) ) ;
#3672=CARTESIAN_POINT ( 'NONE',  ( 73.91582514665041970, 54.93225018311873953, -16.13162452324062102 ) ) ;
#3675=CARTESIAN_POINT ( 'NONE',  ( 74.71692913107121115, 67.15988951933469764, 12.46506041926016728 ) ) ;
#3676=CARTESIAN_POINT ( 'NONE',  ( 27.47308016966368882, 31.56454794089043503, 10.00000000000000355 ) ) ;
#3680=CARTESIAN_POINT ( 'NONE',  ( 83.37296956034944628, 51.74080471427829764, 14.95189368521466733 ) ) ;
#3682=CARTESIAN_POINT ( 'NONE',  ( 37.28583507901048932, 30.03085787977765975, 9.188101187500006262 ) ) ;
#3685=CARTESIAN_POINT ( 'NONE',  ( 40.42214693012152793, 25.19860640527295104, 2.839279412974134775 ) ) ;
#3692=CARTESIAN_POINT ( 'NONE',  ( 6.089662503932698812, 18.91421378149916421, 9.188101187500008038 ) ) ;
#3694=CARTESIAN_POINT ( 'NONE',  ( 12.04840505635704417, 25.14336893147754282, 7.433330006724141015 ) ) ;
#3699=CARTESIAN_POINT ( 'NONE',  ( 81.10883903633204284, 42.55625711771581621, 7.933723778126640092 ) ) ;
#3704=CARTESIAN_POINT ( 'NONE',  ( 29.42114147039228200, 17.39040679176983772, 1.333680081654574804E-15 ) ) ;
#3709=CARTESIAN_POINT ( 'NONE',  ( 85.85265132163431190, 47.44586991713101298, 10.77177032529229983 ) ) ;
#3711=CARTESIAN_POINT ( 'NONE',  ( 77.46027058111894803, 55.89456704637984785, 16.15791935774714361 ) ) ;
#3713=ORIENTED_EDGE ( 'NONE', *, *, #64048, .T. ) ;
#3714=CARTESIAN_POINT ( 'NONE',  ( 38.63240046701410080, 22.70852965304481330, 1.583844403245330712 ) ) ;
#3715=CARTESIAN_POINT ( 'NONE',  ( 78.81221140396398539, 50.25556598462433300, -14.90820057926957176 ) ) ;
#3717=EDGE_CURVE ( 'NONE', #5821, #7928, #4334, .T. ) ;
#3719=CARTESIAN_POINT ( 'NONE',  ( 80.70996417611414131, 43.44255574045367041, 9.435838178707639301 ) ) ;
#3720=ORIENTED_EDGE ( 'NONE', *, *, #32301, .F. ) ;
#3723=CARTESIAN_POINT ( 'NONE',  ( 73.18824967679846338, 57.61170437758888596, 15.86128386422620196 ) ) ;
#3726=CARTESIAN_POINT ( 'NONE',  ( 42.18527710189642477, 24.75978393459168458, -1.583844403245396437 ) ) ;
#3736=CARTESIAN_POINT ( 'NONE',  ( 69.63741438990557242, 65.54831403221679409, 11.22893310010135437 ) ) ;
#3739=CARTESIAN_POINT ( 'NONE',  ( 86.61622014653730162, 43.24285245142148426, 0.7059395827112208144 ) ) ;
#3745=CARTESIAN_POINT ( 'NONE',  ( 28.38260615371904905, 22.10170272979928185, -7.433330006724141015 ) ) ;
#3761=CARTESIAN_POINT ( 'NONE',  ( 82.76725405737721530, 40.62549709574067691, -1.366123307036881229 ) ) ;
#3770=DIRECTION ( 'NONE',  ( 0.5000000000000014433, -0.8660254037844378194, 0.000000000000000000 ) ) ;
#3779=CARTESIAN_POINT ( 'NONE',  ( 83.35260738844563377, 45.68874033332231477, 10.31089094078401303 ) ) ;
#3783=CARTESIAN_POINT ( 'NONE',  ( 68.70848240496243875, 63.96496568607160071, -12.08092966280174529 ) ) ;
#3785=CARTESIAN_POINT ( 'NONE',  ( 81.07888283437659993, 54.57333583963867341, 16.21189145771869988 ) ) ;
#3794=CARTESIAN_POINT ( 'NONE',  ( 85.29362735876655677, 48.41412782346650800, 12.38048700662147716 ) ) ;
#3797=CARTESIAN_POINT ( 'NONE',  ( 19.57800816787531417, 26.70171378149919050, -9.188101187500004485 ) ) ;
#3807=CARTESIAN_POINT ( 'NONE',  ( 87.73298548431469612, 44.18903561216111342, 4.633618514853094617 ) ) ;
#3809=CARTESIAN_POINT ( 'NONE',  ( 81.78211920620266540, 55.43645730098403135, -15.94077319035399221 ) ) ;
#3813=CARTESIAN_POINT ( 'NONE',  ( 86.01647438233806042, 46.20655162549090988, 9.232364010202251947 ) ) ;
#3814=CARTESIAN_POINT ( 'NONE',  ( 80.05167170976248769, 53.91814069023228484, 15.77049608246057488 ) ) ;
#3819=CARTESIAN_POINT ( 'NONE',  ( 45.09207854535236493, 28.96004757982094446, -5.678558825948276656 ) ) ;
#3821=ORIENTED_EDGE ( 'NONE', *, *, #28259, .T. ) ;
#3822=DIRECTION ( 'NONE',  ( 0.5000000000000013323, -0.8660254037844378194, 0.000000000000000000 ) ) ;
#3826=CARTESIAN_POINT ( 'NONE',  ( 78.98760635313000478, 59.78900401997537273, 16.49402793498109432 ) ) ;
#3830=CARTESIAN_POINT ( 'NONE',  ( 76.49585787082935440, 52.49147331306175346, -15.83840385325085265 ) ) ;
#3831=CARTESIAN_POINT ( 'NONE',  ( 80.55977923476241642, 44.53388773478042140, 11.41474457639882978 ) ) ;
#3832=CARTESIAN_POINT ( 'NONE',  ( 84.51897762134323955, 49.81277137233040264, -13.22473897856888847 ) ) ;
#3838=CARTESIAN_POINT ( 'NONE',  ( 77.06564511512083016, 49.52831132331507291, 14.97822083552720329 ) ) ;
#3840=EDGE_CURVE ( 'NONE', #54783, #63867, #44032, .T. ) ;
#3841=CARTESIAN_POINT ( 'NONE',  ( 75.32469880294877385, 60.28293755603083071, 15.62353883029713408 ) ) ;
#3845=CARTESIAN_POINT ( 'NONE',  ( 82.34058838678610925, 40.67931664917913537, 3.225392581287613414 ) ) ;
#3853=CARTESIAN_POINT ( 'NONE',  ( 75.63696794127041301, 54.59993838101707553, 16.11484836142631494 ) ) ;
#3854=CARTESIAN_POINT ( 'NONE',  ( 11.99908958663318970, 18.87878583063839955, -9.188101187500006262 ) ) ;
#3856=CARTESIAN_POINT ( 'NONE',  ( 85.42558612123971784, 48.32295466858820987, -12.24938428992805406 ) ) ;
#3857=ORIENTED_EDGE ( 'NONE', *, *, #24551, .T. ) ;
#3866=CARTESIAN_POINT ( 'NONE',  ( 88.27690704811887201, 44.27260258506650814, -1.937958420041432595 ) ) ;
#3869=VECTOR ( 'NONE', #18612, 1000.000000000000114 ) ;
#3878=CARTESIAN_POINT ( 'NONE',  ( 88.01573842283471549, 44.26461227791823205, 2.810035873497462422 ) ) ;
#3883=CARTESIAN_POINT ( 'NONE',  ( 75.77888672275405213, 61.25515952569155331, -15.46323051080574373 ) ) ;
#3897=FACE_OUTER_BOUND ( 'NONE', #16165, .T. ) ;
#3904=CARTESIAN_POINT ( 'NONE',  ( 79.48115437758207236, 54.55162964910791601, -15.95922698054103783 ) ) ;
#3905=CARTESIAN_POINT ( 'NONE',  ( 75.20489394095216085, 55.31235798330321529, -16.61246018749456610 ) ) ;
#3909=CARTESIAN_POINT ( 'NONE',  ( 77.39025700982266187, 52.99708388390572367, -16.30678418076230329 ) ) ;
#3915=CARTESIAN_POINT ( 'NONE',  ( 84.05461052688725943, 48.09452081518995925, -12.67959057290721603 ) ) ;
#3917=VERTEX_POINT ( 'NONE', #4056 ) ;
#3918=CARTESIAN_POINT ( 'NONE',  ( 15.78795072819010770, 21.06628583063840665, -9.188101187500006262 ) ) ;
#3923=CARTESIAN_POINT ( 'NONE',  ( 86.32803123799460820, 47.24229282936711627, 10.81726845165080064 ) ) ;
#3926=LINE ( 'NONE', #42890, #56608 ) ;
#3929=CARTESIAN_POINT ( 'NONE',  ( 74.72588123256606707, 53.65605547442924461, 16.08708352512548245 ) ) ;
#3945=CARTESIAN_POINT ( 'NONE',  ( 32.45774345291223995, 27.24335787977765833, -9.188101187500008038 ) ) ;
#3946=CARTESIAN_POINT ( 'NONE',  ( 74.55827288133576758, 60.13454576714501343, -15.53984938263620030 ) ) ;
#3953=CARTESIAN_POINT ( 'NONE',  ( 68.19833798964504012, 65.85959993625948528, 10.83357887337748338 ) ) ;
#3955=CARTESIAN_POINT ( 'NONE',  ( 85.75965168945023720, 48.55180427257402442, -11.81072568050767657 ) ) ;
#3958=CARTESIAN_POINT ( 'NONE',  ( 70.40802990919080173, 60.99707565408044729, 14.93107424293364360 ) ) ;
#3969=CARTESIAN_POINT ( 'NONE',  ( 87.12419840511867619, 46.02342392002756810, -8.190366543198424054 ) ) ;
#3972=CARTESIAN_POINT ( 'NONE',  ( 83.30594405552706405, 41.61771957242412867, -2.403535763665288538 ) ) ;
#3980=ORIENTED_EDGE ( 'NONE', *, *, #55904, .F. ) ;
#3981=DIRECTION ( 'NONE',  ( -0.2925570654631255985, 0.000000000000000000, 0.9562480658530004840 ) ) ;
#3983=CARTESIAN_POINT ( 'NONE',  ( 68.68961001230228192, 69.20649816010151767, -5.408517505406226888 ) ) ;
#3985=CARTESIAN_POINT ( 'NONE',  ( 69.67644213241599971, 62.68400490086408183, -13.31948877326700931 ) ) ;
#3990=CARTESIAN_POINT ( 'NONE',  ( 81.51672219897599803, 48.01526152666208702, 13.05833413880630722 ) ) ;
#3993=CARTESIAN_POINT ( 'NONE',  ( 25.48331929688331243, 38.21091486745862653, 7.012934429366973338E-14 ) ) ;
#4000=CARTESIAN_POINT ( 'NONE',  ( 80.44641172169940546, 52.15703007935309188, 15.27578981345033959 ) ) ;
#4001=CARTESIAN_POINT ( 'NONE',  ( 69.44037796687385367, 70.26988621369126520, -3.529725965421429468 ) ) ;
#4003=CARTESIAN_POINT ( 'NONE',  ( 83.41128051646016672, 51.86661034151835281, 14.99497567496408479 ) ) ;
#4012=ADVANCED_FACE ( 'NONE', ( #54121 ), #76811, .T. ) ;
#4013=CARTESIAN_POINT ( 'NONE',  ( 28.14208253200458287, 39.18080186712595037, 3.090169943749475401 ) ) ;
#4016=CARTESIAN_POINT ( 'NONE',  ( 82.14625348271364658, 43.20029849263703170, -8.033064318764047584 ) ) ;
#4017=( BOUNDED_CURVE ( )  B_SPLINE_CURVE ( 2, ( #2561, #56737, #80086, #95798, #65822, #49633, #58228, #96787, #11658, #82086, #87719, #25861, #26848 ),
 .UNSPECIFIED., .F., .T. ) 
 B_SPLINE_CURVE_WITH_KNOTS ( ( 3, 2, 2, 2, 2, 2, 3 ),
 ( 0.7625000000000000666, 0.7650000000000000133, 0.7700000000000000178, 0.7750000000000000222, 0.7800000000000000266, 0.7850000000000000311, 0.7875000000000000888 ),
 .UNSPECIFIED. ) 
 CURVE ( )  GEOMETRIC_REPRESENTATION_ITEM ( )  RATIONAL_B_SPLINE_CURVE ( ( 0.9755282581475767101, 0.9755282581475772652, 1.000000000000000000, 0.9510565162951535312, 1.000000000000000000, 0.9510565162951535312, 1.000000000000000000, 0.9510565162951535312, 1.000000000000000000, 0.9510565162951535312, 1.000000000000000000, 0.9755282581475761550, 0.9755282581475767101 ) ) 
 REPRESENTATION_ITEM ( '' )  );
#4021=CARTESIAN_POINT ( 'NONE',  ( 86.79998443407272646, 45.86195168027221314, 8.882059948630848467 ) ) ;
#4023=CARTESIAN_POINT ( 'NONE',  ( 82.25567614043384879, 41.32243640453275901, 5.438163968954911276 ) ) ;
#4027=CARTESIAN_POINT ( 'NONE',  ( 38.71056063283548809, 34.30066082961425167, -10.00000000000000533 ) ) ;
#4043=CARTESIAN_POINT ( 'NONE',  ( 67.26837558547590845, 67.21133208665345649, -8.574135192023929264 ) ) ;
#4045=LINE ( 'NONE', #25870, #94487 ) ;
#4048=CARTESIAN_POINT ( 'NONE',  ( 31.76492312988469280, 26.84335787977765264, 9.188101187500006262 ) ) ;
#4050=CARTESIAN_POINT ( 'NONE',  ( 74.14312167556930433, 66.30466486950707861, 1.224646799147354045E-15 ) ) ;
#4053=CARTESIAN_POINT ( 'NONE',  ( 18.06126741312425921, 22.37878583063840310, 9.188101187500006262 ) ) ;
#4054=CARTESIAN_POINT ( 'NONE',  ( 75.93655505379200576, 59.57132730434130963, 15.86584733416168014 ) ) ;
#4056=CARTESIAN_POINT ( 'NONE',  ( 85.85265132163429769, 47.44586991713102009, 10.77177032529229450 ) ) ;
#4068=CARTESIAN_POINT ( 'NONE',  ( 66.35522338032015455, 68.72304060489808819, -2.132035597865990173 ) ) ;
#4070=CARTESIAN_POINT ( 'NONE',  ( 81.37739665788856769, 55.81704345181816507, 16.38624498997419110 ) ) ;
#4071=CARTESIAN_POINT ( 'NONE',  ( 79.14312167556931854, 57.64441083166269664, 0.000000000000000000 ) ) ;
#4075=ADVANCED_FACE ( 'NONE', ( #24250 ), #92238, .T. ) ;
#4078=ORIENTED_EDGE ( 'NONE', *, *, #41371, .T. ) ;
#4079=CARTESIAN_POINT ( 'NONE',  ( 33.64972468124413751, 31.37878583063843152, 9.188101187500006262 ) ) ;
#4106=CARTESIAN_POINT ( 'NONE',  ( 86.95125388468488836, 44.27950943365674163, -4.934478059872851041 ) ) ;
#4110=CARTESIAN_POINT ( 'NONE',  ( 75.31417462687399222, 64.08252782891483434, 14.41125185447981139 ) ) ;
#4121=CARTESIAN_POINT ( 'NONE',  ( 68.78984366447195953, 69.70809013107415808, 4.131647041545672749 ) ) ;
#4124=CARTESIAN_POINT ( 'NONE',  ( 14.28567607145357421, 31.18080186712592550, 3.090169943749475401 ) ) ;
#4140=CARTESIAN_POINT ( 'NONE',  ( 22.16161828121410338, 13.76426979415089491, 3.090169943749476733 ) ) ;
#4145=CARTESIAN_POINT ( 'NONE',  ( 73.80791270665581294, 55.11249867311061479, -16.60035380508545089 ) ) ;
#4147=CARTESIAN_POINT ( 'NONE',  ( 76.93253562831463910, 60.43031639469479188, 16.23105599402710197 ) ) ;
#4155=CARTESIAN_POINT ( 'NONE',  ( 80.63243328097439644, 57.57134443808153890, -16.24110709809310293 ) ) ;
#4158=CARTESIAN_POINT ( 'NONE',  ( 36.84800447571193160, 26.98920272979929180, 7.433330006724137462 ) ) ;
#4164=CARTESIAN_POINT ( 'NONE',  ( 8.259543914800127951, 22.95586893147753571, 7.433330006724141015 ) ) ;
#4166=CARTESIAN_POINT ( 'NONE',  ( 16.65397613197454518, 21.56628583063840310, 9.188101187500006262 ) ) ;
#4170=CARTESIAN_POINT ( 'NONE',  ( 18.55511606660780899, 34.21091486745861232, -1.111400068045478839E-16 ) ) ;
#4171=CARTESIAN_POINT ( 'NONE',  ( 74.93188263267299476, 53.45048654396977383, -16.53684691294480302 ) ) ;
#4177=CARTESIAN_POINT ( 'NONE',  ( 66.34264438788950713, 68.59982612598324181, 4.834438131297811303 ) ) ;
#4178=CARTESIAN_POINT ( 'NONE',  ( 87.53878856671160236, 45.51437473004847334, 6.953484175700196168 ) ) ;
#4180=EDGE_LOOP ( 'NONE', ( #9809, #20008, #50289, #27909 ) ) ;
#4201=EDGE_CURVE ( 'NONE', #45691, #25393, #5328, .T. ) ;
#4205=EDGE_CURVE ( 'NONE', #55813, #64236, #62786, .T. ) ;
#4208=FACE_OUTER_BOUND ( 'NONE', #14757, .T. ) ;
#4210=CARTESIAN_POINT ( 'NONE',  ( 82.40357584069326435, 53.81685777417739303, 15.85384499771503464 ) ) ;
#4218=CARTESIAN_POINT ( 'NONE',  ( 77.34929714582419535, 49.75066375701363341, -14.99659801915009893 ) ) ;
#4224=CARTESIAN_POINT ( 'NONE',  ( 41.98060738119045965, 32.43677371833805978, -10.00000000000000355 ) ) ;
#4238=CARTESIAN_POINT ( 'NONE',  ( 23.08833070876649529, 13.73415679381821874, 1.333680081654574804E-15 ) ) ;
#4246=CARTESIAN_POINT ( 'NONE',  ( 73.98997032606590096, 68.61244119570729083, 11.40121143613688304 ) ) ;
#4248=CARTESIAN_POINT ( 'NONE',  ( 74.62401959271109320, 66.89443057110609914, 13.05059976691390311 ) ) ;
#4254=CARTESIAN_POINT ( 'NONE',  ( 73.89337880468768560, 68.29732366427398915, -11.63451623248603006 ) ) ;
#4261=ADVANCED_FACE ( 'NONE', ( #28878 ), #5568, .T. ) ;
#4263=CARTESIAN_POINT ( 'NONE',  ( 68.48685824045450943, 64.40307437426383785, -12.27912010813812138 ) ) ;
#4270=CARTESIAN_POINT ( 'NONE',  ( 68.29626324166530082, 66.69358781172817885, 9.212701310791057807 ) ) ;
#4276=CARTESIAN_POINT ( 'NONE',  ( 15.95033727479334651, 30.18502408145591787, 5.678558825948277544 ) ) ;
#4277=CARTESIAN_POINT ( 'NONE',  ( 74.72173318163055455, 67.07206250228034605, 12.96729955693541747 ) ) ;
#4279=B_SPLINE_CURVE_WITH_KNOTS ( 'NONE', 3,
 ( #20640, #59097, #66236, #21630, #6433, #97173, #43418, #43914, #27739, #29234, #81969, #58608, #97655, #59603, #75344, #12045, #89584, #35324, #13053, #91066, #98145, #89107, #19657, #83460, #12545, #90070, #90583, #50519, #5434, #81471, #51525, #42898, #36316, #67220, #60101 ),
 .UNSPECIFIED., .F., .F.,
 ( 4, 2, 2, 2, 2, 2, 1, 2, 2, 1, 2, 2, 1, 2, 2, 1, 1, 1, 1, 2, 4 ),
 ( 0.000000000000000000, 0.1115121842044346223, 0.1672682763066525302, 0.2230243684088704381, 0.3345365526133051159, 0.3902926447155220524, 0.4460487368177389889, 0.4739267828688474293, 0.5018048289199559253, 0.5575609210221736944, 0.6133170131243914636, 0.6690731052266091217, 0.7248291973288267798, 0.7387682203543819437, 0.7527072433799371076, 0.7805852894310503221, 0.8363413815332770840, 0.8642194275843916307, 0.8781584506099474607, 0.8851279621227241545, 0.8920974736355009593 ),
 .UNSPECIFIED. ) ;
#4281=CARTESIAN_POINT ( 'NONE',  ( 74.96142304803882439, 67.14338225477067112, 13.01358479607535301 ) ) ;
#4282=CARTESIAN_POINT ( 'NONE',  ( 17.05992553822454383, 21.80066082961421259, 10.00000000000000533 ) ) ;
#4288=CARTESIAN_POINT ( 'NONE',  ( 81.60881798005151211, 55.57634303931474307, -16.32954282162994630 ) ) ;
#4289=ORIENTED_EDGE ( 'NONE', *, *, #15269, .T. ) ;
#4290=CARTESIAN_POINT ( 'NONE',  ( 68.82014897516015139, 66.62176625695347809, 9.652166363822647810 ) ) ;
#4292=CARTESIAN_POINT ( 'NONE',  ( 71.92208958328382096, 72.24687304073742666, 0.6003283116912437878 ) ) ;
#4293=CARTESIAN_POINT ( 'NONE',  ( 85.28397160125511789, 44.79186958938679197, 7.782623374060775312 ) ) ;
#4296=CARTESIAN_POINT ( 'NONE',  ( 72.21207746560659757, 71.58261399135965064, -5.866756630810175288 ) ) ;
#4300=CARTESIAN_POINT ( 'NONE',  ( 4.482002306134333480, 24.36126292948892669, 6.180339887498949913 ) ) ;
#4303=CARTESIAN_POINT ( 'NONE',  ( 73.75884458225044682, 55.19329439359383116, 16.59761296138449538 ) ) ;
#4307=CARTESIAN_POINT ( 'NONE',  ( 79.45469543192598394, 59.63697030301000979, 16.53293242656297224 ) ) ;
#4308=FACE_OUTER_BOUND ( 'NONE', #57649, .T. ) ;
#4309=CARTESIAN_POINT ( 'NONE',  ( 87.73591684602568819, 43.42914754852260018, 0.5750851355217611038 ) ) ;
#4314=CARTESIAN_POINT ( 'NONE',  ( 76.52406481382922721, 52.48284444663511294, -15.83437973198601867 ) ) ;
#4316=CARTESIAN_POINT ( 'NONE',  ( 73.31376544620394498, 70.15701068496694859, -9.311920139903870464 ) ) ;
#4317=CARTESIAN_POINT ( 'NONE',  ( 84.51862751403463392, 49.89385305662934655, -13.69084041065644897 ) ) ;
#4327=B_SPLINE_CURVE_WITH_KNOTS ( 'NONE', 3,
 ( #50927, #80392, #19573, #48953, #49942, #11473, #27654, #64653, #95603, #2873, #34245, #65634 ),
 .UNSPECIFIED., .F., .F.,
 ( 4, 2, 2, 2, 2, 4 ),
 ( 0.000000000000000000, 0.1937403633080442278, 0.3874807266160884556, 0.5812210899241326834, 0.6780912715781548528, 0.7749614532321769111 ),
 .UNSPECIFIED. ) ;
#4330=CARTESIAN_POINT ( 'NONE',  ( 75.64162694863910019, 61.89125772273574455, 15.26202274178806739 ) ) ;
#4334=( BOUNDED_CURVE ( )  B_SPLINE_CURVE ( 2, ( #4554, #81111, #5065, #97776, #82107, #35454, #51661, #82610, #34460, #26866, #13176, #96807, #27857 ),
 .UNSPECIFIED., .F., .T. ) 
 B_SPLINE_CURVE_WITH_KNOTS ( ( 3, 2, 2, 2, 2, 2, 3 ),
 ( 0.2374999999999999889, 0.2399999999999999911, 0.2449999999999999956, 0.2500000000000000000, 0.2550000000000000044, 0.2600000000000000089, 0.2625000000000000111 ),
 .UNSPECIFIED. ) 
 CURVE ( )  GEOMETRIC_REPRESENTATION_ITEM ( )  RATIONAL_B_SPLINE_CURVE ( ( 0.9755282581475768211, 0.9755282581475768211, 1.000000000000000000, 0.9510565162951535312, 1.000000000000000000, 0.9510565162951535312, 1.000000000000000000, 0.9510565162951535312, 1.000000000000000000, 0.9510565162951535312, 1.000000000000000000, 0.9755282581475768211, 0.9755282581475768211 ) ) 
 REPRESENTATION_ITEM ( '' )  );
#4335=CARTESIAN_POINT ( 'NONE',  ( 82.25473147846066979, 40.64636554663949397, 3.297339663603231941 ) ) ;
#4336=FACE_OUTER_BOUND ( 'NONE', #76567, .T. ) ;
#4340=CARTESIAN_POINT ( 'NONE',  ( 79.14312167556931854, 57.64441083166269664, 0.000000000000000000 ) ) ;
#4348=CARTESIAN_POINT ( 'NONE',  ( 85.51230132848702681, 48.33290926536287913, -12.21747540207229221 ) ) ;
#4358=CARTESIAN_POINT ( 'NONE',  ( 88.41177868068123757, 44.08414425260226466, -2.750064808092239410 ) ) ;
#4361=CARTESIAN_POINT ( 'NONE',  ( 66.34509500891661560, 68.88037130226740601, 0.1021054603021520624 ) ) ;
#4369=CARTESIAN_POINT ( 'NONE',  ( 88.15895072599572302, 44.32995048785090120, 2.709407056482791898 ) ) ;
#4375=CARTESIAN_POINT ( 'NONE',  ( 71.52376905861159173, 65.98510282706405405, -11.84387761488746804 ) ) ;
#4378=CARTESIAN_POINT ( 'NONE',  ( 80.77778805714483212, 43.59742387627670723, -9.572361431960153766 ) ) ;
#4384=CARTESIAN_POINT ( 'NONE',  ( 77.79465598582810060, 50.60749197390607890, 15.20047523612101692 ) ) ;
#4387=CARTESIAN_POINT ( 'NONE',  ( 77.50346144362303846, 52.20099699948093530, 15.68093582552386067 ) ) ;
#4391=CARTESIAN_POINT ( 'NONE',  ( 84.45465033531688448, 50.16481452220934756, 13.87013043972112847 ) ) ;
#4396=FACE_OUTER_BOUND ( 'NONE', #89210, .T. ) ;
#4400=CARTESIAN_POINT ( 'NONE',  ( 72.90436461565970205, 57.14737113808597258, 15.90414412829909629 ) ) ;
#4407=CARTESIAN_POINT ( 'NONE',  ( 34.84050961144773595, 32.06628583063844218, -9.188101187500006262 ) ) ;
#4410=ORIENTED_EDGE ( 'NONE', *, *, #58194, .T. ) ;
#4411=CARTESIAN_POINT ( 'NONE',  ( 28.70736568013821355, 22.28920272979928185, -7.433330006724141015 ) ) ;
#4413=CARTESIAN_POINT ( 'NONE',  ( 8.751641773298651117, 23.79103043416547081, 8.090169943749478065 ) ) ;
#4416=ORIENTED_EDGE ( 'NONE', *, *, #70885, .F. ) ;
#4417=CARTESIAN_POINT ( 'NONE',  ( 86.44281908042910345, 47.25702098485090374, 10.76508247627446302 ) ) ;
#4419=CARTESIAN_POINT ( 'NONE',  ( 72.42375743991897252, 71.58586897710435437, 5.137075947767138828 ) ) ;
#4422=CARTESIAN_POINT ( 'NONE',  ( 74.86122959240560704, 53.28810031052174168, 16.52678853274738913 ) ) ;
#4424=ORIENTED_EDGE ( 'NONE', *, *, #74556, .T. ) ;
#4426=VERTEX_POINT ( 'NONE', #91692 ) ;
#4428=CARTESIAN_POINT ( 'NONE',  ( 66.22369928180467014, 68.54468502351485881, 4.796181935161453858 ) ) ;
#4430=CARTESIAN_POINT ( 'NONE',  ( 77.15970654835309972, 62.92887492094936874, -15.28573681817205099 ) ) ;
#4433=CARTESIAN_POINT ( 'NONE',  ( 3.886609837484615415, 24.01751292744053856, 6.180339887498949913 ) ) ;
#4435=CARTESIAN_POINT ( 'NONE',  ( 87.89481703180801730, 44.20627101738029552, -4.400163950806246227 ) ) ;
#4436=CARTESIAN_POINT ( 'NONE',  ( 83.30270248594673888, 48.09331988551172543, 12.99346492355625493 ) ) ;
#4437=B_SPLINE_CURVE_WITH_KNOTS ( 'NONE', 3,
 ( #64718, #34306, #26215, #65206, #73806, #19134, #4400, #57591, #88572, #50007 ),
 .UNSPECIFIED., .F., .F.,
 ( 4, 2, 2, 2, 4 ),
 ( 0.000000000000000000, 0.2500000000000000000, 0.5000000000000000000, 0.7500000000000000000, 1.000000000000000000 ),
 .UNSPECIFIED. ) ;
#4438=CARTESIAN_POINT ( 'NONE',  ( 38.16387531507685793, 24.96004757982092315, -5.678558825948275768 ) ) ;
#4439=CARTESIAN_POINT ( 'NONE',  ( 75.11394087589162893, 59.95852931487045367, -15.66470097906968739 ) ) ;
#4446=CARTESIAN_POINT ( 'NONE',  ( 68.31114388777692170, 65.60375069781311197, 10.42464132957602096 ) ) ;
#4448=CARTESIAN_POINT ( 'NONE',  ( 85.65560247527419335, 48.36830939525689388, -11.71305587975093054 ) ) ;
#4458=ORIENTED_EDGE ( 'NONE', *, *, #93100, .T. ) ;
#4460=EDGE_CURVE ( 'NONE', #68256, #29855, #91909, .T. ) ;
#4466=ORIENTED_EDGE ( 'NONE', *, *, #77991, .F. ) ;
#4469=CARTESIAN_POINT ( 'NONE',  ( 71.48247391640994408, 59.13597001042445811, 15.29777321559891412 ) ) ;
#4481=CARTESIAN_POINT ( 'NONE',  ( 83.40135606954622460, 47.43196963034611002, 11.92714562067884465 ) ) ;
#4483=CARTESIAN_POINT ( 'NONE',  ( 69.54685086556757767, 62.58220806599024399, -13.90877278120082572 ) ) ;
#4486=CIRCLE ( 'NONE', #17429, 15.60714546451156970 ) ;
#4488=CARTESIAN_POINT ( 'NONE',  ( 71.05939029094800219, 61.29899699392983337, 14.43395936496894372 ) ) ;
#4489=CARTESIAN_POINT ( 'NONE',  ( 82.17449527959013267, 40.64114721183973700, -3.468282653352762424 ) ) ;
#4492=CARTESIAN_POINT ( 'NONE',  ( 76.13392677502470463, 51.08280539179364865, -16.07326884494762353 ) ) ;
#4495=CARTESIAN_POINT ( 'NONE',  ( 80.28488664218848214, 51.35788028056815335, 15.03242532107574903 ) ) ;
#4499=CARTESIAN_POINT ( 'NONE',  ( 77.74340892523753155, 61.62887588481113710, 16.08014808546132457 ) ) ;
#4504=CARTESIAN_POINT ( 'NONE',  ( 40.33962347462181697, 28.45404122711136452, -8.090169943749478065 ) ) ;
#4505=CARTESIAN_POINT ( 'NONE',  ( 67.16990927169524639, 66.79708245693809943, -9.067759095298582039 ) ) ;
#4508=CARTESIAN_POINT ( 'NONE',  ( 83.90373659686035523, 43.27808524138897894, -6.473827899055408786 ) ) ;
#4510=CARTESIAN_POINT ( 'NONE',  ( 71.29042387187584495, 72.21982342411818934, 1.426054166102403542 ) ) ;
#4512=VECTOR ( 'NONE', #59448, 1000.000000000000000 ) ;
#4514=CARTESIAN_POINT ( 'NONE',  ( 87.37955803993382631, 45.91052472906853410, 8.478299845497456744 ) ) ;
#4516=CARTESIAN_POINT ( 'NONE',  ( 71.70445494439258027, 72.46184198916859032, -1.357087204883099751 ) ) ;
#4518=AXIS2_PLACEMENT_3D ( 'NONE', #55902, #40207, #25540 ) ;
#4519=CARTESIAN_POINT ( 'NONE',  ( 86.99418556918212175, 46.03399372306155612, 8.963501050606421217 ) ) ;
#4522=CARTESIAN_POINT ( 'NONE',  ( 41.98060738119045254, 32.43677371833805978, -10.00000000000000355 ) ) ;
#4531=CARTESIAN_POINT ( 'NONE',  ( 87.65912573706349065, 45.31011780831707370, -7.252675111195947544 ) ) ;
#4537=ORIENTED_EDGE ( 'NONE', *, *, #66771, .F. ) ;
#4540=CARTESIAN_POINT ( 'NONE',  ( 67.30093204598001932, 67.22481299031751689, -8.581777852237747695 ) ) ;
#4541=ORIENTED_EDGE ( 'NONE', *, *, #13452, .F. ) ;
#4545=CARTESIAN_POINT ( 'NONE',  ( 26.65419051621551461, 38.49540643055190259, 3.479690158560446702E-15 ) ) ;
#4547=CARTESIAN_POINT ( 'NONE',  ( 86.44477669634372319, 47.51534994824657332, -10.48323238175251504 ) ) ;
#4551=CARTESIAN_POINT ( 'NONE',  ( 16.17646586176480739, 17.84335787977762422, 9.188101187500006262 ) ) ;
#4554=CARTESIAN_POINT ( 'NONE',  ( 20.76088743254790003, 12.39040679176982529, 1.333680081654574804E-15 ) ) ;
#4559=CARTESIAN_POINT ( 'NONE',  ( 70.29419212219671920, 65.26512559587472140, -12.42138800992322345 ) ) ;
#4568=CARTESIAN_POINT ( 'NONE',  ( 66.10902144195793539, 69.14947487106338997, -2.045211508994028815 ) ) ;
#4570=CARTESIAN_POINT ( 'NONE',  ( 82.39721099668476256, 40.42262220707492304, 1.474573639734339192 ) ) ;
#4571=CARTESIAN_POINT ( 'NONE',  ( 78.14027010749673252, 61.52421145379764766, -16.15198519767693242 ) ) ;
#4572=CARTESIAN_POINT ( 'NONE',  ( 72.08258120803394320, 72.26635199662449338, -1.519792127538861504 ) ) ;
#4579=B_SPLINE_CURVE_WITH_KNOTS ( 'NONE', 3,
 ( #95889, #89295, #94872, #19849, #9761, #87320, #12244, #98344, #59296, #5134 ),
 .UNSPECIFIED., .F., .F.,
 ( 4, 2, 2, 2, 4 ),
 ( 0.000000000000000000, 0.2500000000000000000, 0.5000000000000000000, 0.7500000000000000000, 1.000000000000000000 ),
 .UNSPECIFIED. ) ;
#4585=CARTESIAN_POINT ( 'NONE',  ( 75.06695094285400671, 67.05599132900850634, -12.66018568268392208 ) ) ;
#4589=CARTESIAN_POINT ( 'NONE',  ( 81.41589984655307433, 56.11952908245346805, 16.07747354504519421 ) ) ;
#4592=ORIENTED_EDGE ( 'NONE', *, *, #75401, .T. ) ;
#4593=CARTESIAN_POINT ( 'NONE',  ( 75.28832949877902081, 62.89817645449259942, -14.85265024749852003 ) ) ;
#4602=VECTOR ( 'NONE', #6037, 1000.000000000000114 ) ;
#4612=ORIENTED_EDGE ( 'NONE', *, *, #79519, .T. ) ;
#4613=CARTESIAN_POINT ( 'NONE',  ( 81.51908546427152658, 44.28658535684733266, -9.904776572929741008 ) ) ;
#4617=CARTESIAN_POINT ( 'NONE',  ( 74.48086480164226941, 59.59897794796569315, 15.66551120389625140 ) ) ;
#4620=CARTESIAN_POINT ( 'NONE',  ( 76.83839478644495102, 56.36739346141288109, 16.18311125838449627 ) ) ;
#4622=( BOUNDED_CURVE ( )  B_SPLINE_CURVE ( 2, ( #31584, #22005, #52901, #55868, #3233, #17397, #87872, #80247, #9306, #79749, #9825, #78718, #1209 ),
 .UNSPECIFIED., .F., .T. ) 
 B_SPLINE_CURVE_WITH_KNOTS ( ( 3, 2, 2, 2, 2, 2, 3 ),
 ( 0.2874999999999999778, 0.2899999999999999800, 0.2949999999999999845, 0.2999999999999999889, 0.3049999999999999933, 0.3099999999999999978, 0.3125000000000000000 ),
 .UNSPECIFIED. ) 
 CURVE ( )  GEOMETRIC_REPRESENTATION_ITEM ( )  RATIONAL_B_SPLINE_CURVE ( ( 0.9755282581475768211, 0.9755282581475768211, 1.000000000000000000, 0.9510565162951535312, 1.000000000000000000, 0.9510565162951535312, 1.000000000000000000, 0.9510565162951535312, 1.000000000000000000, 0.9510565162951535312, 1.000000000000000000, 0.9755282581475768211, 0.9755282581475768211 ) ) 
 REPRESENTATION_ITEM ( '' )  );
#4628=CARTESIAN_POINT ( 'NONE',  ( 68.45839193658751753, 69.34571607991892961, 4.633211366208406012 ) ) ;
#4632=CARTESIAN_POINT ( 'NONE',  ( 17.48767303752208235, 28.83478043621388309, -8.090169943749479842 ) ) ;
#4635=CARTESIAN_POINT ( 'NONE',  ( 41.24097861217908445, 35.76159833115055164, -9.594050593750004907 ) ) ;
#4642=EDGE_CURVE ( 'NONE', #14677, #64537, #68885, .T. ) ;
#4649=CARTESIAN_POINT ( 'NONE',  ( 19.14394661871191161, 29.79103043416549212, 8.090169943749478065 ) ) ;
#4650=CARTESIAN_POINT ( 'NONE',  ( 85.35014107232977665, 49.09618135595809463, 12.41884494283699070 ) ) ;
#4666=CARTESIAN_POINT ( 'NONE',  ( 72.69493809724967548, 71.16443809380129437, -7.267007365939472052 ) ) ;
#4667=CARTESIAN_POINT ( 'NONE',  ( 79.24135755033685768, 59.96798256686211204, 16.14279214841722521 ) ) ;
#4668=CARTESIAN_POINT ( 'NONE',  ( 37.36761971798259196, 27.28920272979929607, -7.433330006724141015 ) ) ;
#4676=VECTOR ( 'NONE', #52790, 1000.000000000000000 ) ;
#4677=CARTESIAN_POINT ( 'NONE',  ( 12.79778405566451482, 30.49540643055186351, 3.479690158560446702E-15 ) ) ;
#4678=CARTESIAN_POINT ( 'NONE',  ( 71.55389639452420170, 72.40420208557203807, 1.000837480472094088 ) ) ;
#4679=CARTESIAN_POINT ( 'NONE',  ( 82.40357584069326435, 53.81685777417738592, 15.85384499771503819 ) ) ;
#4682=VERTEX_POINT ( 'NONE', #72775 ) ;
#4685=CARTESIAN_POINT ( 'NONE',  ( 75.15016756581449897, 53.62953826938981905, -16.54102740569554086 ) ) ;
#4686=CARTESIAN_POINT ( 'NONE',  ( 81.35004932177496073, 42.10696970585722454, 7.989028237409868005 ) ) ;
#4696=EDGE_CURVE ( 'NONE', #44705, #30119, #60256, .T. ) ;
#4702=CARTESIAN_POINT ( 'NONE',  ( 80.75322455565131463, 57.27148952657292824, 16.56885343786527898 ) ) ;
#4705=DIRECTION ( 'NONE',  ( -0.8660254037844377084, -0.5000000000000014433, -0.000000000000000000 ) ) ;
#4706=CARTESIAN_POINT ( 'NONE',  ( 76.73837805473348794, 50.85003728428209513, -15.44848974388898810 ) ) ;
#4707=ADVANCED_FACE ( 'NONE', ( #4336 ), #34241, .T. ) ;
#4710=CARTESIAN_POINT ( 'NONE',  ( 80.96449997289272460, 43.55881912823607394, 9.398159779699934546 ) ) ;
#4715=CARTESIAN_POINT ( 'NONE',  ( 73.69818273017419585, 59.72407691843551447, 15.50369470924484716 ) ) ;
#4717=ORIENTED_EDGE ( 'NONE', *, *, #51666, .T. ) ;
#4727=CARTESIAN_POINT ( 'NONE',  ( 87.11349487006070547, 46.19076519147612458, 8.411924245371466213 ) ) ;
#4730=CARTESIAN_POINT ( 'NONE',  ( 19.66861660350102881, 11.75978393459163662, -1.583844403245362020 ) ) ;
#4740=VERTEX_POINT ( 'NONE', #65451 ) ;
#4741=CARTESIAN_POINT ( 'NONE',  ( 87.86298961015023679, 44.89260222163544256, 6.207647304897665919 ) ) ;
#4746=CARTESIAN_POINT ( 'NONE',  ( 15.99984526765731907, 17.43677371833800649, -10.00000000000000355 ) ) ;
#4754=EDGE_CURVE ( 'NONE', #64642, #50553, #91712, .T. ) ;
#4769=CARTESIAN_POINT ( 'NONE',  ( 71.45648812236639458, 71.78579786804675678, -2.123707775780323992 ) ) ;
#4771=CARTESIAN_POINT ( 'NONE',  ( 5.882932626810616128, 22.13478043621385893, 8.090169943749478065 ) ) ;
#4772=AXIS2_PLACEMENT_3D ( 'NONE', #91117, #15549, #68267 ) ;
#4777=B_SPLINE_CURVE_WITH_KNOTS ( 'NONE', 3,
 ( #15994, #71215, #46893, #32690, #86960, #17495, #12409, #97042, #56981, #42770 ),
 .UNSPECIFIED., .F., .F.,
 ( 4, 2, 2, 2, 4 ),
 ( 0.000000000000000000, 0.2500000000000000000, 0.5000000000000000000, 0.7500000000000000000, 1.000000000000000000 ),
 .UNSPECIFIED. ) ;
#4779=CARTESIAN_POINT ( 'NONE',  ( 79.11171798038404290, 59.41904482235663920, -16.53441574648432422 ) ) ;
#4780=EDGE_CURVE ( 'NONE', #45021, #96468, #68694, .T. ) ;
#4785=CARTESIAN_POINT ( 'NONE',  ( 81.00366901594098579, 53.98193135160821754, 16.09339324300580287 ) ) ;
#4787=CARTESIAN_POINT ( 'NONE',  ( 73.29014998154374894, 69.82456558858999074, 9.114582937199678270 ) ) ;
#4790=CARTESIAN_POINT ( 'NONE',  ( 72.52494868832852148, 57.36103174889360190, 16.32214684599243881 ) ) ;
#4792=CARTESIAN_POINT ( 'NONE',  ( 68.30731939365449534, 66.71466498842660542, 9.194818449662610860 ) ) ;
#4793=FACE_OUTER_BOUND ( 'NONE', #53542, .T. ) ;
#4794=ORIENTED_EDGE ( 'NONE', *, *, #46383, .F. ) ;
#4797=CARTESIAN_POINT ( 'NONE',  ( 82.66943193480358332, 42.37244407833836846, 7.179986229313780832 ) ) ;
#4799=CARTESIAN_POINT ( 'NONE',  ( 21.78279761992806129, 35.68290643055188838, 3.479690158560446702E-15 ) ) ;
#4805=CARTESIAN_POINT ( 'NONE',  ( 68.55513178119723250, 64.39780669069259034, 11.67030924314737916 ) ) ;
#4807=B_SPLINE_CURVE_WITH_KNOTS ( 'NONE', 3,
 ( #9845, #79770, #17939, #87409, #72140, #56907, #18438, #49328, #3736, #32620, #18942, #65514, #80778, #3249, #25010, #34614, #10335, #49819, #80267, #95971, #79272, #63517, #86380, #71646, #11350, #33119, #56414, #40197, #34132, #48837, #41201, #55889, #78733, #64021, #71140, #1741, #42206, #65025, #2744, #9323, #33633, #40706, #94961, #86883, #64527, #26534 ),
 .UNSPECIFIED., .F., .F.,
 ( 4, 1, 1, 1, 2, 2, 1, 1, 1, 2, 2, 1, 1, 2, 2, 1, 1, 2, 2, 1, 1, 2, 2, 1, 2, 2, 1, 2, 2, 4 ),
 ( 0.000000000000000000, 0.06249999999997776778, 0.09374999999996665168, 0.1093749999999626965, 0.1171874999999631406, 0.1249999999999635847, 0.1874999999999612255, 0.2187499999999591438, 0.2343749999999581168, 0.2421874999999576172, 0.2499999999999570899, 0.3124999999999558131, 0.3437499999999572564, 0.3593749999999596434, 0.3749999999999620304, 0.4374999999999680256, 0.4687499999999711897, 0.4843749999999705791, 0.4999999999999700240, 0.5624999999999753530, 0.5937499999999779066, 0.6093749999999785727, 0.6249999999999791278, 0.6874999999999807931, 0.7187499999999830136, 0.7499999999999852340, 0.8124999999999895639, 0.8437499999999916733, 0.8749999999999936717, 1.000000000000000000 ),
 .UNSPECIFIED. ) ;
#4812=CARTESIAN_POINT ( 'NONE',  ( 4.600586583810874153, 20.84336893147753500, -7.433330006724137462 ) ) ;
#4813=ORIENTED_EDGE ( 'NONE', *, *, #76838, .F. ) ;
#4814=CARTESIAN_POINT ( 'NONE',  ( 70.50125601336765158, 69.59879263790479342, 6.833936649965831833 ) ) ;
#4816=CARTESIAN_POINT ( 'NONE',  ( 77.55425247552874168, 49.72899633274018782, 14.94892306696621631 ) ) ;
#4818=CARTESIAN_POINT ( 'NONE',  ( 69.81003220229767692, 70.90474864260643528, 1.346364422161295815 ) ) ;
#4820=ORIENTED_EDGE ( 'NONE', *, *, #24292, .T. ) ;
#4821=EDGE_CURVE ( 'NONE', #92014, #20280, #94267, .T. ) ;
#4823=CARTESIAN_POINT ( 'NONE',  ( 9.667034506031535912, 13.78052372038638218, -10.00000000000000355 ) ) ;
#4826=CARTESIAN_POINT ( 'NONE',  ( 66.10228174255657052, 68.64626758096548542, 4.271897712742703135 ) ) ;
#4827=CARTESIAN_POINT ( 'NONE',  ( 86.28449982416978514, 46.95005333036156969, -10.54182221192812818 ) ) ;
#4834=CARTESIAN_POINT ( 'NONE',  ( 74.73487060833782891, 53.69418506457893869, 16.08953207461605928 ) ) ;
#4835=EDGE_LOOP ( 'NONE', ( #60725, #46809, #97039, #22506 ) ) ;
#4839=B_SPLINE_CURVE_WITH_KNOTS ( 'NONE', 3,
 ( #43033, #87743, #80614, #88727, #17781, #34465, #41046, #57254, #25888, #11191, #3585, #89232, #4559, #18284, #49178, #10677 ),
 .UNSPECIFIED., .F., .F.,
 ( 4, 1, 2, 2, 2, 1, 2, 2, 4 ),
 ( 0.000000000000000000, 0.1250000000000006661, 0.1875000000000011102, 0.2500000000000015543, 0.5000000000000035527, 0.6250000000000026645, 0.6875000000000022204, 0.7500000000000017764, 1.000000000000000000 ),
 .UNSPECIFIED. ) ;
#4840=CARTESIAN_POINT ( 'NONE',  ( 84.75777273949843504, 49.85283236070215196, -13.16649314506352475 ) ) ;
#4845=CARTESIAN_POINT ( 'NONE',  ( 88.46339282683516103, 43.84930607083626342, 0.06358566718628017034 ) ) ;
#4853=FACE_OUTER_BOUND ( 'NONE', #2335, .T. ) ;
#4860=CARTESIAN_POINT ( 'NONE',  ( 77.05881501368067177, 62.08228305079084919, 15.47689417538831869 ) ) ;
#4861=CARTESIAN_POINT ( 'NONE',  ( 12.18311320154372801, 9.960047579820882291, -5.678558825948276656 ) ) ;
#4862=EDGE_CURVE ( 'NONE', #74723, #66013, #40873, .T. ) ;
#4866=CARTESIAN_POINT ( 'NONE',  ( 82.41933087055697627, 40.38430946167127900, -0.8419157719606891188 ) ) ;
#4868=CARTESIAN_POINT ( 'NONE',  ( 78.13885432066443570, 47.60678095579073243, -13.89854567155110665 ) ) ;
#4869=CARTESIAN_POINT ( 'NONE',  ( 76.18015836404990182, 65.31175638499995273, -14.08199309598906801 ) ) ;
#4871=CARTESIAN_POINT ( 'NONE',  ( 77.49342303783743091, 51.34850931301296839, -15.95500110091012047 ) ) ;
#4877=CARTESIAN_POINT ( 'NONE',  ( 66.42665093650496999, 68.92825192741007356, 0.05375612720383066145 ) ) ;
#4885=CARTESIAN_POINT ( 'NONE',  ( 88.47356364199694667, 43.97712956045978672, 1.870819122003379187 ) ) ;
#4890=CARTESIAN_POINT ( 'NONE',  ( 22.61461015039527922, 36.55466486950700755, 7.012934429366973338E-14 ) ) ;
#4891=CARTESIAN_POINT ( 'NONE',  ( 79.90415527835997977, 58.06450031769458775, 16.26805976162004441 ) ) ;
#4895=CARTESIAN_POINT ( 'NONE',  ( 80.68090781023890656, 43.23449616528987605, -9.208455255847814769 ) ) ;
#4899=CARTESIAN_POINT ( 'NONE',  ( 87.64597162258272078, 44.36656289597981839, -4.061167644325248460 ) ) ;
#4902=CARTESIAN_POINT ( 'NONE',  ( 78.88416877887701162, 55.54717536121699339, 16.10259716625749249 ) ) ;
#4906=CARTESIAN_POINT ( 'NONE',  ( 84.61344793860607183, 50.61789989419376212, 13.66347863740807078 ) ) ;
#4914=DIRECTION ( 'NONE',  ( 0.5000000000000014433, -0.8660254037844378194, 0.000000000000000000 ) ) ;
#4916=EDGE_CURVE ( 'NONE', #9076, #7688, #31192, .T. ) ;
#4918=CARTESIAN_POINT ( 'NONE',  ( 13.89351337401799391, 10.94754757982087945, 5.678558825948272215 ) ) ;
#4919=CARTESIAN_POINT ( 'NONE',  ( 67.88638817726504726, 65.66482337939683589, 10.84849054539563440 ) ) ;
#4925=CARTESIAN_POINT ( 'NONE',  ( 75.59751354683669433, 65.29851079375914935, 14.32525510856801709 ) ) ;
#4927=CARTESIAN_POINT ( 'NONE',  ( 35.39919958817179690, 22.29860640527294535, -2.839279412974138328 ) ) ;
#4929=CARTESIAN_POINT ( 'NONE',  ( 75.09434506655878749, 58.72130435028955731, 16.35444582053638740 ) ) ;
#4931=CARTESIAN_POINT ( 'NONE',  ( 22.39019813391814751, 21.43085787977763701, -9.188101187500008038 ) ) ;
#4936=( BOUNDED_CURVE ( )  B_SPLINE_CURVE ( 2, ( #9777, #2673, #1164, #41134, #55336, #33052, #18368, #86312, #23944, #64458, #1675, #16847, #78672 ),
 .UNSPECIFIED., .F., .T. ) 
 B_SPLINE_CURVE_WITH_KNOTS ( ( 3, 2, 2, 2, 2, 2, 3 ),
 ( 0.01250000000000000069, 0.01499999999999999944, 0.02000000000000000042, 0.02500000000000000139, 0.02999999999999999889, 0.03500000000000000333, 0.03750000000000000555 ),
 .UNSPECIFIED. ) 
 CURVE ( )  GEOMETRIC_REPRESENTATION_ITEM ( )  RATIONAL_B_SPLINE_CURVE ( ( 0.9755282581475768211, 0.9755282581475768211, 1.000000000000000000, 0.9510565162951535312, 1.000000000000000000, 0.9510565162951535312, 1.000000000000000000, 0.9510565162951535312, 1.000000000000000000, 0.9510565162951535312, 1.000000000000000000, 0.9755282581475767101, 0.9755282581475768211 ) ) 
 REPRESENTATION_ITEM ( '' )  );
#4937=CARTESIAN_POINT ( 'NONE',  ( 70.99470838923255656, 61.07944878815018086, 14.50894906648577631 ) ) ;
#4943=ORIENTED_EDGE ( 'NONE', *, *, #20110, .F. ) ;
#4944=CARTESIAN_POINT ( 'NONE',  ( 86.53615271802112829, 45.81344646433711887, -9.028428416148619462 ) ) ;
#4947=LINE ( 'NONE', #28729, #87156 ) ;
#4948=CARTESIAN_POINT ( 'NONE',  ( 81.46395823134524505, 41.91769605856590886, -7.572882635748096725 ) ) ;
#4950=CARTESIAN_POINT ( 'NONE',  ( 66.90909321525144549, 68.17756947874360662, -6.600776075497404527 ) ) ;
#4955=CARTESIAN_POINT ( 'NONE',  ( 88.19523698511710563, 44.46804064255652378, -4.670053027270651747 ) ) ;
#4957=CARTESIAN_POINT ( 'NONE',  ( 36.57375671714491006, 36.51421378149921537, -9.188101187500004485 ) ) ;
#4958=CARTESIAN_POINT ( 'NONE',  ( 75.60606471573575504, 59.79559749501326849, -15.76384363349462525 ) ) ;
#4961=VERTEX_POINT ( 'NONE', #42512 ) ;
#4963=CARTESIAN_POINT ( 'NONE',  ( 81.13608137687064925, 42.60696278352305200, 7.988320930663086905 ) ) ;
#4964=CARTESIAN_POINT ( 'NONE',  ( 68.35176054198142026, 65.66817991788700226, 10.38336397426687974 ) ) ;
#4966=CARTESIAN_POINT ( 'NONE',  ( 85.85757975920050455, 48.54684933318403495, 12.22929488966399880 ) ) ;
#4973=CARTESIAN_POINT ( 'NONE',  ( 78.96564777457507489, 59.77152385746119023, 16.49451479044646973 ) ) ;
#4977=CYLINDRICAL_SURFACE ( 'NONE', #57701, 10.00000000000001066 ) ;
#4980=ORIENTED_EDGE ( 'NONE', *, *, #23312, .F. ) ;
#4982=FACE_OUTER_BOUND ( 'NONE', #28219, .T. ) ;
#4983=CARTESIAN_POINT ( 'NONE',  ( 72.04273812837081437, 59.28583566120335746, 15.34548535902080246 ) ) ;
#4985=CARTESIAN_POINT ( 'NONE',  ( 17.84779077618757626, 10.70852965304478843, 1.583844403245364907 ) ) ;
#4996=CARTESIAN_POINT ( 'NONE',  ( 82.54497950703030540, 45.20829423347827714, 10.29466844316771734 ) ) ;
#4998=CARTESIAN_POINT ( 'NONE',  ( 69.60866448817320418, 62.38574252042192114, -13.47313703376398664 ) ) ;
#5000=ORIENTED_EDGE ( 'NONE', *, *, #27630, .F. ) ;
#5006=PLANE ( 'NONE',  #7937 ) ;
#5009=CARTESIAN_POINT ( 'NONE',  ( 79.83603558536034939, 49.47464228346785831, 14.36412132351409454 ) ) ;
#5010=CARTESIAN_POINT ( 'NONE',  ( 67.81775003199867058, 69.65792968701072141, -1.625205651952876362 ) ) ;
#5016=CARTESIAN_POINT ( 'NONE',  ( 73.62324627567660684, 69.69863374744915063, -9.485613227022392735 ) ) ;
#5017=CYLINDRICAL_SURFACE ( 'NONE', #67393, 16.60714546451156792 ) ;
#5019=CARTESIAN_POINT ( 'NONE',  ( 31.53257425345116260, 33.90829794293883026, 10.00000000000000355 ) ) ;
#5024=CARTESIAN_POINT ( 'NONE',  ( 68.19623763041657583, 68.89888936764938876, 6.646214744952141373 ) ) ;
#5027=CARTESIAN_POINT ( 'NONE',  ( 86.72622664077024979, 46.44337019134223965, 9.089705772931038652 ) ) ;
#5029=CARTESIAN_POINT ( 'NONE',  ( 71.88488839165290756, 72.57896392602057745, -1.213109508826733407 ) ) ;
#5034=CARTESIAN_POINT ( 'NONE',  ( 44.94038342867872871, 31.11029122506298705, -8.090169943749478065 ) ) ;
#5039=CARTESIAN_POINT ( 'NONE',  ( 72.04713214249291298, 67.71874806291776849, -10.56511915099177301 ) ) ;
#5052=CARTESIAN_POINT ( 'NONE',  ( 67.36095123383401528, 66.69455278167134793, -8.467567626117057600 ) ) ;
#5056=CARTESIAN_POINT ( 'NONE',  ( 77.38344707992527560, 49.10671604805792612, -15.27628165681131200 ) ) ;
#5057=CARTESIAN_POINT ( 'NONE',  ( 36.43182450750798296, 23.96004757982092315, -5.678558825948276656 ) ) ;
#5062=CARTESIAN_POINT ( 'NONE',  ( 14.44441505419593064, 16.84335787977761711, 9.188101187500006262 ) ) ;
#5063=CARTESIAN_POINT ( 'NONE',  ( 31.19757978783344399, 18.41603393254327514, -1.583844403245396437 ) ) ;
#5064=CARTESIAN_POINT ( 'NONE',  ( 66.99161703481539121, 69.18407532166969531, -1.591805497166421945 ) ) ;
#5065=CARTESIAN_POINT ( 'NONE',  ( 20.60277255440211164, 12.86426979415089278, -3.090169943749474069 ) ) ;
#5076=CARTESIAN_POINT ( 'NONE',  ( 66.53579232977513414, 68.81352912635834684, -2.225901204553964785 ) ) ;
#5079=CARTESIAN_POINT ( 'NONE',  ( 78.30540700459937398, 61.08339965263432703, -15.90943835942215046 ) ) ;
#5084=EDGE_LOOP ( 'NONE', ( #74785, #58142, #55551, #51440, #84394, #91008, #53504, #361, #23654, #60146, #29901, #3223, #97416, #15997, #95497, #76627, #21383, #28632, #92804, #28886, #85462, #84718, #77866, #34111, #37819, #44393, #51263, #95450, #94208, #85865, #42078, #72803, #47076, #98970, #17943, #96689, #19077, #57033, #66177, #56161, #81298, #65066, #5120, #81849 ) ) ;
#5092=CARTESIAN_POINT ( 'NONE',  ( 81.80121988122709809, 55.57996685460995678, 16.31202477726384004 ) ) ;
#5097=CARTESIAN_POINT ( 'NONE',  ( 76.66170733860469966, 62.40948344195681585, -15.31146014519883991 ) ) ;
#5098=CARTESIAN_POINT ( 'NONE',  ( 87.25031752591065981, 43.70243236605378456, -1.741586274254640188 ) ) ;
#5104=CARTESIAN_POINT ( 'NONE',  ( 76.12675507841289857, 51.10280720933135967, -16.07849684238113497 ) ) ;
#5113=CARTESIAN_POINT ( 'NONE',  ( 88.03035862218379748, 44.39407565500617636, 4.731894665149351198 ) ) ;
#5114=CARTESIAN_POINT ( 'NONE',  ( 69.82040969387803386, 67.81765696479247651, -9.721210921651175951 ) ) ;
#5115=CARTESIAN_POINT ( 'NONE',  ( 79.95816027405184911, 44.45915948752763569, -10.97504526610144993 ) ) ;
#5117=CARTESIAN_POINT ( 'NONE',  ( 74.95033118751130985, 62.00148963258062906, 15.10603149014151647 ) ) ;
#5120=ORIENTED_EDGE ( 'NONE', *, *, #93977, .T. ) ;
#5121=CARTESIAN_POINT ( 'NONE',  ( 77.34464417660132085, 59.58687695751251567, 16.02097068141453562 ) ) ;
#5128=CARTESIAN_POINT ( 'NONE',  ( 70.30735548187293205, 71.13048692529430639, 1.811214889704019226 ) ) ;
#5132=CARTESIAN_POINT ( 'NONE',  ( 12.79584618246493477, 29.16126292948894516, -6.180339887498951690 ) ) ;
#5134=CARTESIAN_POINT ( 'NONE',  ( 82.10990542498430500, 41.84899041517284957, 5.504228460268151046 ) ) ;
#5142=EDGE_CURVE ( 'NONE', #63156, #86521, #95046, .T. ) ;
#5147=CARTESIAN_POINT ( 'NONE',  ( 84.74286529925647926, 43.14323271637052670, 6.350952207087867230 ) ) ;
#5148=CARTESIAN_POINT ( 'NONE',  ( 30.99507739981537213, 18.86426979415090699, -3.090169943749474069 ) ) ;
#5149=CARTESIAN_POINT ( 'NONE',  ( 68.11396990072297797, 66.09066184265174115, -10.54551009852403354 ) ) ;
#5151=CARTESIAN_POINT ( 'NONE',  ( 72.05747908138206981, 72.41062208079183904, -3.017343731799825512 ) ) ;
#5152=CARTESIAN_POINT ( 'NONE',  ( 74.18348328006130998, 55.49302420257691892, -16.11862618869125896 ) ) ;
#5153=EDGE_CURVE ( 'NONE', #48577, #62465, #95325, .T. ) ;
#5157=CARTESIAN_POINT ( 'NONE',  ( 74.67374711520119490, 67.12383300063542890, 12.47279688402123199 ) ) ;
#5163=CARTESIAN_POINT ( 'NONE',  ( 72.87252120309180725, 71.00776288696197014, -7.711505026642229588 ) ) ;
#5165=CARTESIAN_POINT ( 'NONE',  ( 45.79150443358504674, 28.29860640527296667, -2.839279412974138328 ) ) ;
#5168=CARTESIAN_POINT ( 'NONE',  ( 22.92804849793282784, 21.43677371833801715, -10.00000000000000355 ) ) ;
#5172=CARTESIAN_POINT ( 'NONE',  ( 15.46319120177094142, 20.87878583063840665, -9.188101187500006262 ) ) ;
#5173=CARTESIAN_POINT ( 'NONE',  ( 71.66539077729501628, 72.47145342129384460, 0.9585255015204100504 ) ) ;
#5174=CARTESIAN_POINT ( 'NONE',  ( 82.22659455697501585, 54.23696157584255673, 15.63556931923067239 ) ) ;
#5181=CARTESIAN_POINT ( 'NONE',  ( 81.11262804297332707, 42.45350992371406562, 7.766723531211875198 ) ) ;
#5183=ORIENTED_EDGE ( 'NONE', *, *, #20011, .F. ) ;
#5184=LINE ( 'NONE', #99385, #95961 ) ;
#5185=CARTESIAN_POINT ( 'NONE',  ( 67.96380970210620376, 69.83446729340751347, 0.3907781913280385377 ) ) ;
#5193=CARTESIAN_POINT ( 'NONE',  ( 88.14497077207560949, 43.82233299356100531, -2.120619512623201253 ) ) ;
#5194=CARTESIAN_POINT ( 'NONE',  ( 80.26984573713558291, 57.41310870600725025, -16.58958131739138508 ) ) ;
#5198=CARTESIAN_POINT ( 'NONE',  ( 81.17457202243787151, 43.12509331780193378, 9.545365352588273566 ) ) ;
#5208=CARTESIAN_POINT ( 'NONE',  ( 90.04477061917849312, 44.76220097505219542, 0.000000000000000000 ) ) ;
#5212=ORIENTED_EDGE ( 'NONE', *, *, #56220, .F. ) ;
#5220=EDGE_CURVE ( 'NONE', #63028, #67404, #8246, .T. ) ;
#5224=CARTESIAN_POINT ( 'NONE',  ( 74.46886260449439021, 57.89172860934509401, -15.95710879220658995 ) ) ;
#5231=ORIENTED_EDGE ( 'NONE', *, *, #15630, .F. ) ;
#5232=CARTESIAN_POINT ( 'NONE',  ( 72.06483804294512652, 69.71054388629096366, 8.252314821295385627 ) ) ;
#5233=CARTESIAN_POINT ( 'NONE',  ( 83.36864264039709838, 41.16137561131296962, 2.770299137610701123 ) ) ;
#5234=ADVANCED_FACE ( 'NONE', ( #75210 ), #43779, .T. ) ;
#5240=CARTESIAN_POINT ( 'NONE',  ( 85.27608704655584404, 46.23732751045460532, 10.40392852235657450 ) ) ;
#5245=B_SPLINE_CURVE_WITH_KNOTS ( 'NONE', 3,
 ( #15012, #23605, #54002, #15506, #76352, #23111, #68221, #14541, #31215, #29733, #30734, #822, #68721, #37321, #84962, #39297, #8427, #22633, #7420, #46925, #7941, #84471, #22133, #38313, #99145, #54499, #60607, #69222, #53519, #77332, #62103 ),
 .UNSPECIFIED., .F., .F.,
 ( 4, 3, 3, 3, 3, 3, 3, 3, 3, 3, 4 ),
 ( 0.000000000000000000, 0.1333490885032332374, 0.3007194338854220494, 0.4699862290245090390, 0.5844252810809320575, 0.6686540514502788968, 0.7354980260655487045, 0.8028463152565534777, 0.8633854507757111607, 0.9437142632667073761, 1.000000000000000000 ),
 .UNSPECIFIED. ) ;
#5248=CARTESIAN_POINT ( 'NONE',  ( 84.62367088353330757, 50.61169820936780184, 13.65639662624268702 ) ) ;
#5254=CARTESIAN_POINT ( 'NONE',  ( 74.29176946830207839, 67.89628765651626452, -11.69942945965017422 ) ) ;
#5257=CARTESIAN_POINT ( 'NONE',  ( 81.67837127500261829, 41.48712589271562479, -5.236831772534292107 ) ) ;
#5258=CARTESIAN_POINT ( 'NONE',  ( 8.995063969029878592, 17.14441083166259006, 10.00000000000000533 ) ) ;
#5260=DIRECTION ( 'NONE',  ( -6.123233995736786990E-17, 1.060575238724905929E-16, 1.000000000000000000 ) ) ;
#5262=B_SPLINE_CURVE_WITH_KNOTS ( 'NONE', 3,
 ( #60180, #6514, #28298, #91144, #84054, #66802, #52591, #21706, #99219, #20224, #14110, #37392, #59175, #90664, #60676, #36899, #90148, #12629, #44991, #75936, #68296, #98227, #91637, #35902 ),
 .UNSPECIFIED., .F., .F.,
 ( 4, 2, 2, 2, 2, 2, 2, 2, 2, 2, 2, 4 ),
 ( 0.000000000000000000, 0.1249999999999811262, 0.2499999999999622524, 0.3749999999999433786, 0.4374999999999501510, 0.4999999999999569233, 0.5624999999999636957, 0.6249999999999704681, 0.6874999999999772404, 0.7499999999999840128, 0.8749999999999916733, 1.000000000000000000 ),
 .UNSPECIFIED. ) ;
#5265=CARTESIAN_POINT ( 'NONE',  ( 79.05300200689269730, 59.41537015362478513, -16.53193985632129426 ) ) ;
#5271=ADVANCED_FACE ( 'NONE', ( #77703 ), #29589, .T. ) ;
#5272=CARTESIAN_POINT ( 'NONE',  ( 66.81631347157465939, 68.63490661804873127, -5.506013109174251241 ) ) ;
#5274=CARTESIAN_POINT ( 'NONE',  ( 71.55076955509966297, 59.02864663040953275, -15.83821917523768619 ) ) ;
#5275=CARTESIAN_POINT ( 'NONE',  ( 73.57121657643290291, 69.82745460598127352, 9.896087309288359890 ) ) ;
#5279=CARTESIAN_POINT ( 'NONE',  ( 68.35978272809893497, 66.81434282768250910, 9.109814194020067646 ) ) ;
#5280=CARTESIAN_POINT ( 'NONE',  ( 66.16222611801360642, 68.48874123133123248, -4.854165969021398297 ) ) ;
#5286=CARTESIAN_POINT ( 'NONE',  ( 22.53213034355506750, 33.98502408145593279, -5.678558825948271327 ) ) ;
#5291=CARTESIAN_POINT ( 'NONE',  ( 74.70353909524752112, 67.05423462026553239, 12.97237599094835758 ) ) ;
#5292=CARTESIAN_POINT ( 'NONE',  ( 68.89885689118237622, 64.10311179774262769, 12.05621680499958082 ) ) ;
#5300=ORIENTED_EDGE ( 'NONE', *, *, #14158, .F. ) ;
#5301=CARTESIAN_POINT ( 'NONE',  ( 70.99214648936349192, 70.33938369507340838, 5.954994780460230785 ) ) ;
#5305=CARTESIAN_POINT ( 'NONE',  ( 77.71268576465143951, 49.44357064982640537, 15.32985931323573325 ) ) ;
#5311=ORIENTED_EDGE ( 'NONE', *, *, #87580, .F. ) ;
#5313=CARTESIAN_POINT ( 'NONE',  ( 12.29152061481545566, 25.83478043621387243, -8.090169943749479842 ) ) ;
#5315=ORIENTED_EDGE ( 'NONE', *, *, #29918, .T. ) ;
#5316=CARTESIAN_POINT ( 'NONE',  ( 74.24569808078352651, 55.17391705787447620, 16.60426680768635421 ) ) ;
#5328=LINE ( 'NONE', #21043, #11674 ) ;
#5334=CARTESIAN_POINT ( 'NONE',  ( 81.86540518833783153, 52.37565918963163369, 15.11782163349261410 ) ) ;
#5336=CARTESIAN_POINT ( 'NONE',  ( 75.09907887158918527, 59.19784231363958327, 15.80952553784205428 ) ) ;
#5343=CARTESIAN_POINT ( 'NONE',  ( 71.78973387874195566, 68.32824629913071135, -9.790379935438130232 ) ) ;
#5346=CARTESIAN_POINT ( 'NONE',  ( 75.95060373600504988, 56.00093423504673495, 16.15035647359714588 ) ) ;
#5347=CARTESIAN_POINT ( 'NONE',  ( 4.685401460390529849, 24.74646525600388003, 2.839279412974139660 ) ) ;
#5351=ORIENTED_EDGE ( 'NONE', *, *, #54261, .T. ) ;
#5360=CARTESIAN_POINT ( 'NONE',  ( 84.97346864989049209, 42.47303927933469936, 1.910285522896328469 ) ) ;
#5361=CARTESIAN_POINT ( 'NONE',  ( 88.43398120015881148, 44.08421024288151102, -2.684292198961160114 ) ) ;
#5364=CARTESIAN_POINT ( 'NONE',  ( 73.08335586614711588, 62.87131163969772274, -14.31063855017556286 ) ) ;
#5369=CARTESIAN_POINT ( 'NONE',  ( 83.36188103862497201, 44.67940999285032433, -9.129105138708005995 ) ) ;
#5372=CARTESIAN_POINT ( 'NONE',  ( 88.38522318935277156, 43.99954571450756191, 2.365518284841155783 ) ) ;
#5374=VERTEX_POINT ( 'NONE', #10791 ) ;
#5375=ORIENTED_EDGE ( 'NONE', *, *, #4862, .T. ) ;
#5379=CARTESIAN_POINT ( 'NONE',  ( 85.74702290878657607, 48.70847181056628727, -12.40582123554878891 ) ) ;
#5382=CARTESIAN_POINT ( 'NONE',  ( 84.16162000085680006, 46.04706940539106341, 10.25047128361154058 ) ) ;
#5389=CARTESIAN_POINT ( 'NONE',  ( 78.92796571603908262, 55.80079471467821861, 16.12519358965519345 ) ) ;
#5393=CARTESIAN_POINT ( 'NONE',  ( 78.16852457591994607, 54.24206277777997798, -15.97971777959419271 ) ) ;
#5398=CARTESIAN_POINT ( 'NONE',  ( 84.14828671478454680, 50.48813722287673045, 13.74412682973423649 ) ) ;
#5406=FACE_OUTER_BOUND ( 'NONE', #3133, .T. ) ;
#5413=CARTESIAN_POINT ( 'NONE',  ( 80.52908760376209329, 44.46502938403837391, 11.36794461543396473 ) ) ;
#5414=CARTESIAN_POINT ( 'NONE',  ( 34.45502471548058310, 41.93396525600392977, 2.839279412974139660 ) ) ;
#5418=CARTESIAN_POINT ( 'NONE',  ( 28.84566271970979301, 17.44966523072494979, -2.296566073217252530E-15 ) ) ;
#5419=DIRECTION ( 'NONE',  ( 0.8660254037844377084, 0.5000000000000015543, 0.000000000000000000 ) ) ;
#5423=LINE ( 'NONE', #36305, #59896 ) ;
#5424=CARTESIAN_POINT ( 'NONE',  ( 76.00688113039353766, 65.27918228371470377, -14.45284717766215721 ) ) ;
#5429=CARTESIAN_POINT ( 'NONE',  ( 88.27857211938396631, 44.33912310488177866, -2.307176908786845893 ) ) ;
#5432=ORIENTED_EDGE ( 'NONE', *, *, #7896, .F. ) ;
#5434=CARTESIAN_POINT ( 'NONE',  ( 83.28320137151804659, 41.40174392785183954, 0.7055483525344276030 ) ) ;
#5436=ORIENTED_EDGE ( 'NONE', *, *, #15521, .T. ) ;
#5440=CARTESIAN_POINT ( 'NONE',  ( 12.91273316327571052, 9.583808731787851087, 6.180339887498953466 ) ) ;
#5442=CARTESIAN_POINT ( 'NONE',  ( 87.81919554331292943, 44.17710153608190637, -4.445631852975250098 ) ) ;
#5445=CARTESIAN_POINT ( 'NONE',  ( 33.80247542503471436, 34.91421378149921395, 9.188101187500008038 ) ) ;
#5446=CARTESIAN_POINT ( 'NONE',  ( 73.05987329793948959, 60.57830585426727055, -15.15309607717232687 ) ) ;
#5448=CARTESIAN_POINT ( 'NONE',  ( 87.63520241360411944, 45.47292483007888109, 6.761783866543302324 ) ) ;
#5450=ORIENTED_EDGE ( 'NONE', *, *, #20114, .T. ) ;
#5451=CARTESIAN_POINT ( 'NONE',  ( 87.14453225490829880, 46.27907944775106586, -9.173786573548373013 ) ) ;
#5452=DIRECTION ( 'NONE',  ( 0.4556638457577371626, 0.000000000000000000, -0.8901519306664841258 ) ) ;
#5457=CARTESIAN_POINT ( 'NONE',  ( 71.03830642738165579, 61.94422969780909938, -14.15059485863699607 ) ) ;
#5458=CARTESIAN_POINT ( 'NONE',  ( 82.16240693639510084, 40.80627634428258688, 1.120954036452832980 ) ) ;
#5460=CARTESIAN_POINT ( 'NONE',  ( 77.02134436793002692, 63.41470467299149760, -15.46275534251473438 ) ) ;
#5462=CARTESIAN_POINT ( 'NONE',  ( 78.86219776201926379, 59.55369065033505649, 16.50996775951927020 ) ) ;
#5464=ORIENTED_EDGE ( 'NONE', *, *, #26433, .T. ) ;
#5469=CARTESIAN_POINT ( 'NONE',  ( 87.17064494550572817, 46.10325694261842244, -8.264880744854202987 ) ) ;
#5472=CARTESIAN_POINT ( 'NONE',  ( 68.26658298682237103, 69.66286806335898518, 4.977088283642358668 ) ) ;
#5474=CARTESIAN_POINT ( 'NONE',  ( 73.91058561509676395, 55.40454524342042930, -16.11566030560718588 ) ) ;
#5480=ORIENTED_EDGE ( 'NONE', *, *, #76353, .F. ) ;
#5481=DIRECTION ( 'NONE',  ( -0.3297783986044530158, -0.8484238185761759921, -0.4140328874455538322 ) ) ;
#5490=CARTESIAN_POINT ( 'NONE',  ( 82.53374931873412379, 40.90496126830478829, -3.689593570638290743 ) ) ;
#5493=CARTESIAN_POINT ( 'NONE',  ( 72.14269493036653103, 72.23228066185846785, 3.937576401637835843 ) ) ;
#5494=CARTESIAN_POINT ( 'NONE',  ( 82.34150913319267318, 40.80060775105380344, -3.714726174206739895 ) ) ;
#5496=CARTESIAN_POINT ( 'NONE',  ( 79.04312205966233762, 46.85810355056803900, 13.20029221486031368 ) ) ;
#5498=CARTESIAN_POINT ( 'NONE',  ( 68.82403863051547432, 70.06653083274885319, -2.813536757197747651 ) ) ;
#5504=CARTESIAN_POINT ( 'NONE',  ( 66.35881563399601646, 68.82796675089451810, 1.446283243008493313 ) ) ;
#5505=CARTESIAN_POINT ( 'NONE',  ( 73.27328646083024921, 70.16270934360545652, -9.274526489422589393 ) ) ;
#5509=CARTESIAN_POINT ( 'NONE',  ( 71.71174882302005926, 58.93038559421764688, -15.88944412480316259 ) ) ;
#5510=( BOUNDED_CURVE ( )  B_SPLINE_CURVE ( 2, ( #68750, #67769, #90107, #52064, #53548, #60142, #45935, #7449, #91104, #83007, #29763, #84013, #20680 ),
 .UNSPECIFIED., .F., .T. ) 
 B_SPLINE_CURVE_WITH_KNOTS ( ( 3, 2, 2, 2, 2, 2, 3 ),
 ( 0.6375000000000000666, 0.6400000000000000133, 0.6450000000000000178, 0.6500000000000000222, 0.6550000000000000266, 0.6600000000000000311, 0.6625000000000000888 ),
 .UNSPECIFIED. ) 
 CURVE ( )  GEOMETRIC_REPRESENTATION_ITEM ( )  RATIONAL_B_SPLINE_CURVE ( ( 0.9755282581475767101, 0.9755282581475772652, 1.000000000000000000, 0.9510565162951535312, 1.000000000000000000, 0.9510565162951535312, 1.000000000000000000, 0.9510565162951535312, 1.000000000000000000, 0.9510565162951535312, 1.000000000000000000, 0.9755282581475761550, 0.9755282581475767101 ) ) 
 REPRESENTATION_ITEM ( '' )  );
#5512=CARTESIAN_POINT ( 'NONE',  ( 72.28940563590052193, 72.06213100273473060, 3.327866248218421585 ) ) ;
#5518=CARTESIAN_POINT ( 'NONE',  ( 80.95490552855073929, 50.32613945632080288, -14.46254378829325660 ) ) ;
#5519=CARTESIAN_POINT ( 'NONE',  ( 71.91886814437489761, 72.60555707853946217, -1.127020781340661193 ) ) ;
#5522=CARTESIAN_POINT ( 'NONE',  ( 20.05074681235918277, 34.68290643055188127, 3.479690158560446702E-15 ) ) ;
#5525=CARTESIAN_POINT ( 'NONE',  ( 7.453652514893187586, 19.70171378149916919, -9.188101187500004485 ) ) ;
#5529=CARTESIAN_POINT ( 'NONE',  ( 73.12786766706317110, 63.39850902397307664, 14.05984965185791502 ) ) ;
#5530=CARTESIAN_POINT ( 'NONE',  ( 86.30977306730703447, 47.58285218899635538, -10.62438056216880611 ) ) ;
#5537=VERTEX_POINT ( 'NONE', #35571 ) ;
#5540=DIRECTION ( 'NONE',  ( 0.4635919272833914917, -0.8029647720336136052, 0.3746065934159158450 ) ) ;
#5542=LINE ( 'NONE', #59727, #4602 ) ;
#5543=ORIENTED_EDGE ( 'NONE', *, *, #98251, .F. ) ;
#5544=DIRECTION ( 'NONE',  ( 0.2649596321166021728, -0.4589235447807153423, -0.8480480961564252906 ) ) ;
#5545=CARTESIAN_POINT ( 'NONE',  ( 79.16669127013743434, 45.83075451395571775, -13.07232462202737366 ) ) ;
#5548=CARTESIAN_POINT ( 'NONE',  ( 86.51323263660401608, 47.18218208451981610, -10.10578519018193333 ) ) ;
#5551=CARTESIAN_POINT ( 'NONE',  ( 22.77687932801360660, 15.01110640527292261, 2.839279412974134775 ) ) ;
#5552=CARTESIAN_POINT ( 'NONE',  ( 68.94535929113044403, 64.35437313888181166, 12.52085547237679286 ) ) ;
#5553=CARTESIAN_POINT ( 'NONE',  ( 71.72726194589085935, 70.29524283496927239, -6.982538226112097846 ) ) ;
#5563=CARTESIAN_POINT ( 'NONE',  ( 66.08237217692345666, 68.53364664378331383, -2.343639106938055328 ) ) ;
#5568=CYLINDRICAL_SURFACE ( 'NONE', #58572, 10.00000000000001066 ) ;
#5569=ORIENTED_EDGE ( 'NONE', *, *, #23704, .T. ) ;
#5573=CARTESIAN_POINT ( 'NONE',  ( 82.39721099668476256, 40.42262220707492304, 1.474573639734337860 ) ) ;
#5574=VERTEX_POINT ( 'NONE', #36552 ) ;
#5575=ORIENTED_EDGE ( 'NONE', *, *, #14158, .T. ) ;
#5580=CARTESIAN_POINT ( 'NONE',  ( 81.86683804372771078, 55.45883585039843666, 16.28524382593451136 ) ) ;
#5587=FACE_OUTER_BOUND ( 'NONE', #47590, .T. ) ;
#5591=CARTESIAN_POINT ( 'NONE',  ( 73.23646752216983202, 69.77611894600212850, -9.099901738753176872 ) ) ;
#5592=CARTESIAN_POINT ( 'NONE',  ( 76.17161704303337899, 51.04481688019111374, -15.56989386545701848 ) ) ;
#5599=CARTESIAN_POINT ( 'NONE',  ( 81.62374368218522136, 41.76230689378201788, 5.959470817902202455 ) ) ;
#5607=CARTESIAN_POINT ( 'NONE',  ( 72.73213343415878285, 70.95121167556251862, 7.670646158728287922 ) ) ;
#5613=CARTESIAN_POINT ( 'NONE',  ( 80.78918961562681034, 43.20779693872438543, -9.098606657379765039 ) ) ;
#5614=CARTESIAN_POINT ( 'NONE',  ( 73.72378779666912862, 69.49084951233950846, -9.812509676730275743 ) ) ;
#5619=CARTESIAN_POINT ( 'NONE',  ( 17.57657260583443559, 33.08080186712592763, -3.090169943749475845 ) ) ;
#5624=CARTESIAN_POINT ( 'NONE',  ( 76.28872632190459058, 51.00282802105012081, -16.03419075268624994 ) ) ;
#5629=CARTESIAN_POINT ( 'NONE',  ( 66.80351077683091887, 68.15053363805938602, -6.532535086774335475 ) ) ;
#5632=ADVANCED_FACE ( 'NONE', ( #98387 ), #85815, .T. ) ;
#5634=CARTESIAN_POINT ( 'NONE',  ( 20.35638218401011912, 30.49103043416549497, -8.090169943749479842 ) ) ;
#5635=DIRECTION ( 'NONE',  ( 0.4635919272833914917, -0.8029647720336136052, 0.3746065934159158450 ) ) ;
#5641=CARTESIAN_POINT ( 'NONE',  ( 75.58345210230092448, 53.75839974157640455, 16.53437228110026780 ) ) ;
#5653=CARTESIAN_POINT ( 'NONE',  ( 36.18707552304946518, 42.93396525600392977, 2.839279412974139660 ) ) ;
#5658=LINE ( 'NONE', #83193, #78425 ) ;
#5661=CARTESIAN_POINT ( 'NONE',  ( 13.01786573420820226, 22.91421378149917842, 9.188101187500008038 ) ) ;
#5663=CARTESIAN_POINT ( 'NONE',  ( 82.79017490736518425, 53.74338802490922973, 15.39689667775746251 ) ) ;
#5668=CARTESIAN_POINT ( 'NONE',  ( 80.53812798300913300, 46.07492565378247207, -12.69342001902709072 ) ) ;
#5669=CARTESIAN_POINT ( 'NONE',  ( 81.38935016679909040, 42.00105843850820975, 7.782619590129813858 ) ) ;
#5674=CARTESIAN_POINT ( 'NONE',  ( 66.45324346747356969, 68.19700524679973341, 4.520682066448438619 ) ) ;
#5683=CARTESIAN_POINT ( 'NONE',  ( 80.46835216585913031, 57.85139773374410055, -16.60023610630909019 ) ) ;
#5690=CARTESIAN_POINT ( 'NONE',  ( 74.54230909194660626, 63.39697481222554387, 14.46401092357988638 ) ) ;
#5702=CARTESIAN_POINT ( 'NONE',  ( 73.34397377724333467, 69.83796661625983404, 9.136125499330086441 ) ) ;
#5704=CARTESIAN_POINT ( 'NONE',  ( 82.59507288524608271, 53.86809943430368719, 15.83774089001703800 ) ) ;
#5707=EDGE_CURVE ( 'NONE', #98408, #58918, #92961, .T. ) ;
#5712=CARTESIAN_POINT ( 'NONE',  ( 80.93527952113549873, 55.40317981316568563, -16.00817129638969760 ) ) ;
#5715=CARTESIAN_POINT ( 'NONE',  ( 67.14930737951127071, 66.86624931644598746, 8.959152673661975541 ) ) ;
#5721=CARTESIAN_POINT ( 'NONE',  ( 70.66892005943768140, 66.34497638887206961, 11.09326023022040530 ) ) ;
#5722=CARTESIAN_POINT ( 'NONE',  ( 85.39557543340885104, 43.32749037753681165, 5.933140306914251205 ) ) ;
#5723=CARTESIAN_POINT ( 'NONE',  ( 79.25911175516624496, 45.79062382720663749, 13.00842035693561272 ) ) ;
#5725=CARTESIAN_POINT ( 'NONE',  ( 76.81923273335645774, 55.69533986730546360, -16.60453251139683317 ) ) ;
#5736=CARTESIAN_POINT ( 'NONE',  ( 81.56753329430793542, 59.44520672954722329, 0.3596699001693225983 ) ) ;
#5743=CARTESIAN_POINT ( 'NONE',  ( 70.08719291027311726, 71.11346239110757494, -0.2046584118080456149 ) ) ;
#5744=CARTESIAN_POINT ( 'NONE',  ( 76.54006514935311145, 51.19995672389920571, 16.04627313578386705 ) ) ;
#5745=CYLINDRICAL_SURFACE ( 'NONE', #91974, 16.60714546451156792 ) ;
#5757=CARTESIAN_POINT ( 'NONE',  ( 12.91273316327571052, 9.583808731787852864, 6.180339887498953466 ) ) ;
#5759=CARTESIAN_POINT ( 'NONE',  ( 71.66596873478475516, 59.16830023791868598, -15.31655212997402060 ) ) ;
#5760=CARTESIAN_POINT ( 'NONE',  ( 73.11654091825437263, 69.80299609433679109, 9.611781565164262631 ) ) ;
#5762=EDGE_CURVE ( 'NONE', #77711, #94602, #73467, .T. ) ;
#5764=FACE_OUTER_BOUND ( 'NONE', #34174, .T. ) ;
#5772=CARTESIAN_POINT ( 'NONE',  ( 20.80007953598619963, 32.98502408145593279, -5.678558825948271327 ) ) ;
#5775=CARTESIAN_POINT ( 'NONE',  ( 83.55324616867257248, 51.62071861895685743, -14.85649312488210860 ) ) ;
#5779=CARTESIAN_POINT ( 'NONE',  ( 68.86387196620182749, 64.09141771346156702, 12.04978999048449850 ) ) ;
#5780=EDGE_LOOP ( 'NONE', ( #15528, #40462, #67662, #74007 ) ) ;
#5787=CARTESIAN_POINT ( 'NONE',  ( 72.08189555467076559, 71.77589625233247261, 3.913479549830300108 ) ) ;
#5788=CARTESIAN_POINT ( 'NONE',  ( 84.27190106046026585, 41.73435386644143819, -2.959663762035162460 ) ) ;
#5797=CARTESIAN_POINT ( 'NONE',  ( 72.59661365748412720, 57.20633740541691736, -16.35330217628511207 ) ) ;
#5799=ORIENTED_EDGE ( 'NONE', *, *, #94947, .F. ) ;
#5801=CARTESIAN_POINT ( 'NONE',  ( 14.35886136108867994, 13.45404122711132011, -8.090169943749478065 ) ) ;
#5803=ORIENTED_EDGE ( 'NONE', *, *, #42310, .T. ) ;
#5806=CARTESIAN_POINT ( 'NONE',  ( 86.53256316603656728, 45.00470303126988370, -7.040634408676482714 ) ) ;
#5816=CARTESIAN_POINT ( 'NONE',  ( 81.63469519429038712, 42.65045104992751845, -7.594666505242645194 ) ) ;
#5820=CARTESIAN_POINT ( 'NONE',  ( 88.33060278926279807, 43.77373715677852317, 0.1867717842524382055 ) ) ;
#5821=VERTEX_POINT ( 'NONE', #76932 ) ;
#5822=LINE ( 'NONE', #13927, #36916 ) ;
#5831=CARTESIAN_POINT ( 'NONE',  ( 67.94274346924396468, 68.32429110883670376, -6.362094354891789649 ) ) ;
#5835=CARTESIAN_POINT ( 'NONE',  ( 65.97757591540607791, 68.67073303864405887, -0.1440890505035684610 ) ) ;
#5836=CARTESIAN_POINT ( 'NONE',  ( 13.56875384759882763, 10.76004757982087767, 5.678558825948272215 ) ) ;
#5846=ADVANCED_FACE ( 'NONE', ( #90701 ), #92195, .T. ) ;
#5849=CARTESIAN_POINT ( 'NONE',  ( 77.56105267981614304, 49.72783448595330924, -15.46007777815280981 ) ) ;
#5850=CIRCLE ( 'NONE', #33324, 16.10714546451156082 ) ;
#5854=VERTEX_POINT ( 'NONE', #29844 ) ;
#5856=CARTESIAN_POINT ( 'NONE',  ( 71.92239571885137650, 63.18146859836171103, -13.81142053453491059 ) ) ;
#5863=CARTESIAN_POINT ( 'NONE',  ( 87.43898003897845683, 44.70913447485149561, -5.303997024264144322 ) ) ;
#5866=CARTESIAN_POINT ( 'NONE',  ( 30.45164419685804447, 25.78052372038641948, -10.00000000000000355 ) ) ;
#5868=ORIENTED_EDGE ( 'NONE', *, *, #64011, .F. ) ;
#5872=FACE_OUTER_BOUND ( 'NONE', #81594, .T. ) ;
#5874=CARTESIAN_POINT ( 'NONE',  ( 84.93582513569069192, 42.31612956156499195, 0.5963448692699542253 ) ) ;
#5876=CARTESIAN_POINT ( 'NONE',  ( 68.38018342861622045, 66.23482706493213357, 10.56038378207740358 ) ) ;
#5880=CARTESIAN_POINT ( 'NONE',  ( 87.67819772848358184, 44.37415200095301770, -4.027115429479418474 ) ) ;
#5884=CARTESIAN_POINT ( 'NONE',  ( 82.21058008569970355, 52.79855391407854626, -15.17934502883119308 ) ) ;
#5889=CARTESIAN_POINT ( 'NONE',  ( 84.49887294678060812, 50.66939116110540908, 13.73193151845090831 ) ) ;
#5902=CARTESIAN_POINT ( 'NONE',  ( 80.02025975469349817, 44.34820518763979180, 11.52912450659341381 ) ) ;
#5904=CARTESIAN_POINT ( 'NONE',  ( 38.30461122658549300, 34.06628583063844928, -9.188101187500006262 ) ) ;
#5906=CARTESIAN_POINT ( 'NONE',  ( 81.74119788692269140, 59.14441083166271795, 0.000000000000000000 ) ) ;
#5908=CARTESIAN_POINT ( 'NONE',  ( 20.27082849090286487, 27.10171378149918908, 9.188101187500008038 ) ) ;
#5912=CARTESIAN_POINT ( 'NONE',  ( 82.30224259357629535, 41.51585266698759114, -5.837696018585297075 ) ) ;
#5916=CARTESIAN_POINT ( 'NONE',  ( 70.80077772051866702, 60.95163764393168293, 15.04332542951107676 ) ) ;
#5929=CARTESIAN_POINT ( 'NONE',  ( 86.39040197603725346, 47.55452816739963140, -10.55219518323342243 ) ) ;
#5931=CARTESIAN_POINT ( 'NONE',  ( 84.85964987685913741, 50.19146562821751445, 13.75030272624154470 ) ) ;
#5935=CARTESIAN_POINT ( 'NONE',  ( 30.11829213135327166, 40.49540643055188838, 3.479690158560446702E-15 ) ) ;
#5937=CARTESIAN_POINT ( 'NONE',  ( 72.14715343843565165, 60.82528180842287924, -14.87966352528053449 ) ) ;
#5943=ORIENTED_EDGE ( 'NONE', *, *, #51314, .T. ) ;
#5944=CARTESIAN_POINT ( 'NONE',  ( 87.24292777721575476, 46.11748857515735267, -8.882011181227387198 ) ) ;
#5950=CARTESIAN_POINT ( 'NONE',  ( 73.76765479342118681, 61.19218300593534821, -15.11731574097786712 ) ) ;
#5951=CARTESIAN_POINT ( 'NONE',  ( 82.32489299410643468, 40.36065608818346107, 1.262906813034385456 ) ) ;
#5953=CARTESIAN_POINT ( 'NONE',  ( 77.28356520717616718, 63.39747816212522480, -15.14739555479249589 ) ) ;
#5958=ORIENTED_EDGE ( 'NONE', *, *, #16226, .T. ) ;
#5960=CARTESIAN_POINT ( 'NONE',  ( 34.18979426048110781, 28.24335787977765122, -9.188101187500008038 ) ) ;
#5963=CARTESIAN_POINT ( 'NONE',  ( 74.20878020607858616, 68.72316200637693839, -11.41572480156362879 ) ) ;
#5976=CARTESIAN_POINT ( 'NONE',  ( 83.38724336809534066, 47.38832907623395840, 11.89773227219856899 ) ) ;
#5984=CARTESIAN_POINT ( 'NONE',  ( 82.44254630377066917, 40.85897994371414654, -3.714870737426086755 ) ) ;
#5989=CARTESIAN_POINT ( 'NONE',  ( 84.14612687645852418, 44.79878194911968592, 8.715766578047444924 ) ) ;
#5992=CARTESIAN_POINT ( 'NONE',  ( 70.81316579126399802, 61.41551742065354347, -14.85192641751565468 ) ) ;
#6002=CARTESIAN_POINT ( 'NONE',  ( 81.95770423786879633, 58.76941083166271795, 0.2500000000000019984 ) ) ;
#6004=CARTESIAN_POINT ( 'NONE',  ( 35.31250668086032363, 42.16126292948897714, -6.180339887498951690 ) ) ;
#6007=CARTESIAN_POINT ( 'NONE',  ( 72.00818181938288376, 72.30390281540809383, 3.363530094501230305 ) ) ;
#6012=CARTESIAN_POINT ( 'NONE',  ( 77.35960201006287207, 51.36102757442933608, -15.48319045058203791 ) ) ;
#6013=CARTESIAN_POINT ( 'NONE',  ( 71.47791206682282450, 72.34364865201938244, -1.216664393387148380 ) ) ;
#6015=CARTESIAN_POINT ( 'NONE',  ( 16.58664519722142927, 32.68290643055186706, 3.479690158560446702E-15 ) ) ;
#6018=CARTESIAN_POINT ( 'NONE',  ( 12.50787272796288896, 10.14754757982087874, -5.678558825948276656 ) ) ;
#6023=CARTESIAN_POINT ( 'NONE',  ( 69.96286275937281118, 67.88719041800112564, -8.946398746998555751 ) ) ;
#6027=CARTESIAN_POINT ( 'NONE',  ( 81.92111866118570163, 41.12818642295167848, 3.752801100571455883 ) ) ;
#6037=DIRECTION ( 'NONE',  ( -0.4330127018922203530, 0.7500000000000046629, 0.4999999999999919509 ) ) ;
#6039=LINE ( 'NONE', #91672, #29731 ) ;
#6040=CARTESIAN_POINT ( 'NONE',  ( 79.18083756185062327, 46.29419887370401909, -12.77432615883756206 ) ) ;
#6047=CARTESIAN_POINT ( 'NONE',  ( 24.83671989960918935, 22.84335787977763488, 9.188101187500006262 ) ) ;
#6048=CARTESIAN_POINT ( 'NONE',  ( 79.96701105519208852, 44.50246225239077091, 11.69262897647518962 ) ) ;
#6049=CARTESIAN_POINT ( 'NONE',  ( 72.00092472038465985, 70.29460662667155191, -7.277950757834694251 ) ) ;
#6057=EDGE_CURVE ( 'NONE', #52772, #56685, #69882, .T. ) ;
#6063=CARTESIAN_POINT ( 'NONE',  ( 81.71596569511639530, 55.69046771286013353, 16.33797717450969955 ) ) ;
#6069=CARTESIAN_POINT ( 'NONE',  ( 70.62955678152276562, 60.80479719363771807, -15.06269029744276011 ) ) ;
#6072=VECTOR ( 'NONE', #7591, 1000.000000000000114 ) ;
#6077=CARTESIAN_POINT ( 'NONE',  ( 76.22741562560636908, 65.24129761985034293, 14.53304928680089603 ) ) ;
#6078=CARTESIAN_POINT ( 'NONE',  ( 74.91863663735624357, 66.38413888100485849, -13.07019282884167843 ) ) ;
#6079=CARTESIAN_POINT ( 'NONE',  ( 34.61729389309891758, 20.39040679176985549, -6.890680421881970419E-14 ) ) ;
#6081=CARTESIAN_POINT ( 'NONE',  ( 81.83839218517164227, 55.52280113860526711, 16.29901351018851230 ) ) ;
#6083=CARTESIAN_POINT ( 'NONE',  ( 72.62665088832551419, 69.64092492267511147, 8.780471156129905808 ) ) ;
#6084=CARTESIAN_POINT ( 'NONE',  ( 87.54989630752690744, 45.07147448993673322, 6.930566558073853578 ) ) ;
#6086=( BOUNDED_CURVE ( )  B_SPLINE_CURVE ( 2, ( #98590, #45347, #60041, #6852, #76752, #5866, #21569, #37738, #77252, #91490, #75282, #38228, #61036 ),
 .UNSPECIFIED., .F., .T. ) 
 B_SPLINE_CURVE_WITH_KNOTS ( ( 3, 2, 2, 2, 2, 2, 3 ),
 ( 0.6375000000000000666, 0.6400000000000000133, 0.6450000000000000178, 0.6500000000000000222, 0.6550000000000000266, 0.6600000000000000311, 0.6625000000000000888 ),
 .UNSPECIFIED. ) 
 CURVE ( )  GEOMETRIC_REPRESENTATION_ITEM ( )  RATIONAL_B_SPLINE_CURVE ( ( 0.9755282581475767101, 0.9755282581475772652, 1.000000000000000000, 0.9510565162951535312, 1.000000000000000000, 0.9510565162951535312, 1.000000000000000000, 0.9510565162951535312, 1.000000000000000000, 0.9510565162951535312, 1.000000000000000000, 0.9755282581475761550, 0.9755282581475767101 ) ) 
 REPRESENTATION_ITEM ( '' )  );
#6091=CARTESIAN_POINT ( 'NONE',  ( 76.09996437315240314, 51.13569808109860304, -15.59936768269888852 ) ) ;
#6099=CARTESIAN_POINT ( 'NONE',  ( 88.10887562929657690, 44.41668309952778060, 4.665177569529614487 ) ) ;
#6100=CARTESIAN_POINT ( 'NONE',  ( 86.69825349856462537, 45.38628583907267000, 7.498776714496921514 ) ) ;
#6101=CARTESIAN_POINT ( 'NONE',  ( 87.90374476427271588, 44.03065798963926625, -1.770940394083930780 ) ) ;
#6104=CARTESIAN_POINT ( 'NONE',  ( 74.91863663735624357, 66.38413888100485849, -13.07019282884167843 ) ) ;
#6105=EDGE_LOOP ( 'NONE', ( #98707, #48806, #30843, #99519 ) ) ;
#6106=CARTESIAN_POINT ( 'NONE',  ( 77.10620603181371280, 57.94243604226648614, 16.15307470803915635 ) ) ;
#6108=CARTESIAN_POINT ( 'NONE',  ( 72.58826525418655251, 71.51553178166663827, -5.516888840409344574 ) ) ;
#6109=VECTOR ( 'NONE', #40967, 1000.000000000000000 ) ;
#6110=CARTESIAN_POINT ( 'NONE',  ( 79.86290868560162437, 47.38898415025740718, 13.23194629791669463 ) ) ;
#6111=CARTESIAN_POINT ( 'NONE',  ( 73.30483403957811106, 69.17932697374328654, -9.895411455429695025 ) ) ;
#6118=CARTESIAN_POINT ( 'NONE',  ( 18.33840876668534037, 32.36126292948895866, 6.180339887498949913 ) ) ;
#6121=CARTESIAN_POINT ( 'NONE',  ( 25.63248128490755562, 16.92755873383626408, 6.180339887498953466 ) ) ;
#6127=VERTEX_POINT ( 'NONE', #27748 ) ;
#6128=AXIS2_PLACEMENT_3D ( 'NONE', #11069, #70858, #80496 ) ;
#6130=CARTESIAN_POINT ( 'NONE',  ( 72.99813893926936714, 70.38310088471868653, -8.105588444390599889 ) ) ;
#6134=CARTESIAN_POINT ( 'NONE',  ( 22.93916872074224855, 35.01751292744056343, 6.180339887498949913 ) ) ;
#6137=CARTESIAN_POINT ( 'NONE',  ( 81.38451658133408273, 39.76220097505215278, 2.033788753608857291E-15 ) ) ;
#6159=CARTESIAN_POINT ( 'NONE',  ( 13.17245041747802148, 29.64646525600389637, -2.839279412974133887 ) ) ;
#6161=CARTESIAN_POINT ( 'NONE',  ( 71.41401697283629346, 59.26550905095592725, 15.74935196026153150 ) ) ;
#6166=CARTESIAN_POINT ( 'NONE',  ( 74.96950070121518195, 53.51615853226594055, -16.54031916057799023 ) ) ;
#6167=CARTESIAN_POINT ( 'NONE',  ( 81.30291217968080275, 42.41553967202970199, 7.523264834473000207 ) ) ;
#6170=CARTESIAN_POINT ( 'NONE',  ( 68.61511293431414060, 70.22156159657447461, -0.4539256867429169451 ) ) ;
#6171=CARTESIAN_POINT ( 'NONE',  ( 77.19265361661118163, 63.55806316509790577, 15.06964695689175926 ) ) ;
#6173=ORIENTED_EDGE ( 'NONE', *, *, #4201, .T. ) ;
#6177=VERTEX_POINT ( 'NONE', #96184 ) ;
#6178=CARTESIAN_POINT ( 'NONE',  ( 88.32926345284593594, 43.93619003093853337, -2.170256470903187740 ) ) ;
#6180=DIRECTION ( 'NONE',  ( -0.3613624741150673336, -0.7937185950816985081, -0.4893137583626402387 ) ) ;
#6181=CARTESIAN_POINT ( 'NONE',  ( 80.42701765378497214, 57.95285881342197598, 16.25594651261488011 ) ) ;
#6183=ORIENTED_EDGE ( 'NONE', *, *, #87161, .F. ) ;
#6184=CARTESIAN_POINT ( 'NONE',  ( 87.68484451513312194, 45.24243923569854786, -6.260370172860385551 ) ) ;
#6191=ORIENTED_EDGE ( 'NONE', *, *, #2725, .T. ) ;
#6196=CARTESIAN_POINT ( 'NONE',  ( 42.09650208215185074, 24.70852965304482396, 1.583844403245330712 ) ) ;
#6198=CARTESIAN_POINT ( 'NONE',  ( 83.47960489914133575, 52.40473646238481820, 14.81961029483872494 ) ) ;
#6199=ORIENTED_EDGE ( 'NONE', *, *, #83155, .T. ) ;
#6202=CARTESIAN_POINT ( 'NONE',  ( 73.67141920324468174, 69.63945410956655735, 9.591121436403057032 ) ) ;
#6204=CARTESIAN_POINT ( 'NONE',  ( 82.36618331495026268, 53.78214551141627453, 15.85029956610786428 ) ) ;
#6208=VECTOR ( 'NONE', #6353, 1000.000000000000000 ) ;
#6209=DIRECTION ( 'NONE',  ( 0.4145187862775202015, -0.7179675985244525771, -0.5591929034707450175 ) ) ;
#6212=CARTESIAN_POINT ( 'NONE',  ( 70.96339409936065579, 72.09815267950916962, -0.4058125698486632071 ) ) ;
#6217=CARTESIAN_POINT ( 'NONE',  ( 75.46068616328098244, 54.40098703217916665, -16.11819300020396994 ) ) ;
#6226=CARTESIAN_POINT ( 'NONE',  ( 72.24563128311258708, 71.52449707465140705, 5.035610742599487821 ) ) ;
#6239=CARTESIAN_POINT ( 'NONE',  ( 72.86041354566070538, 69.04060312456013548, 9.737600754264374103 ) ) ;
#6243=CARTESIAN_POINT ( 'NONE',  ( 81.69339766308513617, 41.48081229801229597, -5.200024030478571646 ) ) ;
#6250=CARTESIAN_POINT ( 'NONE',  ( 79.13712759260107532, 59.42437504702359519, -16.53516983581164013 ) ) ;
#6257=CARTESIAN_POINT ( 'NONE',  ( 5.618660645053492608, 25.01751292744054567, 6.180339887498949913 ) ) ;
#6259=CARTESIAN_POINT ( 'NONE',  ( 71.68833228970933646, 59.19930892918411303, -15.31119584666944711 ) ) ;
#6260=CARTESIAN_POINT ( 'NONE',  ( 81.65569285109127406, 59.29250989802573457, 0.4698463103929529372 ) ) ;
#6265=CARTESIAN_POINT ( 'NONE',  ( 72.68142160263464291, 57.13787751540092330, 16.37077060121746541 ) ) ;
#6274=CARTESIAN_POINT ( 'NONE',  ( 23.04210978301307122, 28.70171378149919406, -9.188101187500004485 ) ) ;
#6277=CARTESIAN_POINT ( 'NONE',  ( 83.65902391768069890, 51.64235791857056768, -14.83937710116058639 ) ) ;
#6278=CARTESIAN_POINT ( 'NONE',  ( 76.62156306105930526, 63.43458379359962152, 15.37592086074862685 ) ) ;
#6279=CARTESIAN_POINT ( 'NONE',  ( 88.05378287308985819, 43.82556038557745381, 2.467578420128289540 ) ) ;
#6280=CARTESIAN_POINT ( 'NONE',  ( 75.03253579078814539, 67.12707870640632279, 13.05283704309126236 ) ) ;
#6286=CARTESIAN_POINT ( 'NONE',  ( 74.41171749419693526, 66.31585784636642700, -13.36723480910198170 ) ) ;
#6288=CARTESIAN_POINT ( 'NONE',  ( 3.825981621811214151, 23.18502408145589300, 5.678558825948276656 ) ) ;
#6292=CARTESIAN_POINT ( 'NONE',  ( 85.92832551797569351, 42.38550953085665896, -0.9154095918151041733 ) ) ;
#6293=CARTESIAN_POINT ( 'NONE',  ( 75.42612112994180507, 53.21573441260188275, 16.48906790374613962 ) ) ;
#6294=CARTESIAN_POINT ( 'NONE',  ( 71.64550269418319317, 72.08018802489503685, 0.6977335431020577072 ) ) ;
#6298=CARTESIAN_POINT ( 'NONE',  ( 68.25873685495425036, 69.52711191031835369, 3.726232860363765109 ) ) ;
#6301=CARTESIAN_POINT ( 'NONE',  ( 8.827418999677703937, 23.83478043621386178, -8.090169943749479842 ) ) ;
#6308=EDGE_LOOP ( 'NONE', ( #44167, #47915, #87686, #32478 ) ) ;
#6312=CARTESIAN_POINT ( 'NONE',  ( 84.56954683517940907, 47.31801974212991979, -11.83040963924886135 ) ) ;
#6313=CARTESIAN_POINT ( 'NONE',  ( 88.05624235485146301, 44.55787864911079765, -5.145732200269208967 ) ) ;
#6318=CARTESIAN_POINT ( 'NONE',  ( 81.29786749816629765, 42.48536220638202110, -7.641147779553272734 ) ) ;
#6324=ORIENTED_EDGE ( 'NONE', *, *, #7725, .T. ) ;
#6333=CARTESIAN_POINT ( 'NONE',  ( 82.69413518930780072, 53.98739327922660891, -15.48440177962634223 ) ) ;
#6337=CARTESIAN_POINT ( 'NONE',  ( 9.991594722369004700, 23.95586893147753926, 7.433330006724141015 ) ) ;
#6338=AXIS2_PLACEMENT_3D ( 'NONE', #79925, #49983, #80429 ) ;
#6353=DIRECTION ( 'NONE',  ( -0.2649596321165964552, 0.4589235447807054058, -0.8480480961564325071 ) ) ;
#6354=AXIS2_PLACEMENT_3D ( 'NONE', #78714, #55373, #24494 ) ;
#6357=CARTESIAN_POINT ( 'NONE',  ( 70.16720293958557875, 63.56956892108868118, -12.96925824068795130 ) ) ;
#6365=CARTESIAN_POINT ( 'NONE',  ( 72.10582633461223168, 72.29069366366150007, 1.276487819798711065 ) ) ;
#6368=CARTESIAN_POINT ( 'NONE',  ( 76.15850628665211275, 65.36065209603508208, 14.05241843883173125 ) ) ;
#6377=CARTESIAN_POINT ( 'NONE',  ( 86.03398505837640187, 43.07944667279475226, 2.211680798076963494 ) ) ;
#6379=CARTESIAN_POINT ( 'NONE',  ( 84.08331625476169791, 45.85772664244242947, 10.09099698929909827 ) ) ;
#6384=CARTESIAN_POINT ( 'NONE',  ( 66.04530551455397358, 69.02646038902410908, 2.576574233892690469 ) ) ;
#6386=LINE ( 'NONE', #45364, #45312 ) ;
#6390=CARTESIAN_POINT ( 'NONE',  ( 81.73819839763727657, 45.44352528469654118, 11.62212099951958244 ) ) ;
#6401=EDGE_CURVE ( 'NONE', #78746, #28265, #28686, .T. ) ;
#6402=CARTESIAN_POINT ( 'NONE',  ( 11.38685760444945672, 12.28920272979924988, -7.433330006724141015 ) ) ;
#6406=DIRECTION ( 'NONE',  ( 0.9619696745371175695, -0.2731562652969027893, 0.000000000000000000 ) ) ;
#6407=CARTESIAN_POINT ( 'NONE',  ( 18.70427805463205218, 12.92755873383625520, 6.180339887498953466 ) ) ;
#6408=CARTESIAN_POINT ( 'NONE',  ( 84.64900121116050968, 42.46421430546889297, -2.907483025300086510 ) ) ;
#6412=CARTESIAN_POINT ( 'NONE',  ( 39.09967052555147404, 28.28920272979929962, -7.433330006724141015 ) ) ;
#6414=CYLINDRICAL_SURFACE ( 'NONE', #58792, 16.60714546451156792 ) ;
#6416=CARTESIAN_POINT ( 'NONE',  ( 30.20304716546516133, 19.29860640527293469, -2.839279412974138328 ) ) ;
#6417=VECTOR ( 'NONE', #8640, 1000.000000000000114 ) ;
#6421=EDGE_CURVE ( 'NONE', #74992, #58510, #40103, .T. ) ;
#6422=EDGE_CURVE ( 'NONE', #51335, #15648, #995, .T. ) ;
#6424=CARTESIAN_POINT ( 'NONE',  ( 70.73318623536759731, 60.92596017579931811, 15.03791421717386001 ) ) ;
#6431=CARTESIAN_POINT ( 'NONE',  ( 73.28147120125912295, 69.89235501152899133, 9.618937042358501444 ) ) ;
#6433=CARTESIAN_POINT ( 'NONE',  ( 86.60633125366983620, 44.49099921560663518, 5.921673564571794834 ) ) ;
#6436=CARTESIAN_POINT ( 'NONE',  ( 86.37020013017546205, 47.54260244662367541, -11.08968936411753781 ) ) ;
#6439=FACE_OUTER_BOUND ( 'NONE', #76343, .T. ) ;
#6441=CARTESIAN_POINT ( 'NONE',  ( 33.95706010830453181, 41.64646525600393545, -2.839279412974133887 ) ) ;
#6443=VECTOR ( 'NONE', #20342, 1000.000000000000000 ) ;
#6445=CARTESIAN_POINT ( 'NONE',  ( 87.59596448155561177, 45.49737888473278247, 6.855467717104687608 ) ) ;
#6448=CARTESIAN_POINT ( 'NONE',  ( 72.07457202599672996, 72.29788378598240683, -0.9408228227147766853 ) ) ;
#6450=CARTESIAN_POINT ( 'NONE',  ( 79.70163802149302512, 56.48321831271363180, 16.19055457390075503 ) ) ;
#6454=CARTESIAN_POINT ( 'NONE',  ( 69.33396002066325536, 69.83223954795549560, 6.100251480823068562 ) ) ;
#6455=CARTESIAN_POINT ( 'NONE',  ( 76.44872654795528888, 60.25863428232945296, -15.81057438280002536 ) ) ;
#6458=CARTESIAN_POINT ( 'NONE',  ( 77.14345524627998429, 62.92765389764069539, -15.28297779662353761 ) ) ;
#6463=CARTESIAN_POINT ( 'NONE',  ( 37.70440764347101492, 39.95586893147758900, 7.433330006724141015 ) ) ;
#6471=CARTESIAN_POINT ( 'NONE',  ( 69.02410329663756272, 70.46522642847207862, 3.828157181349015392 ) ) ;
#6473=EDGE_LOOP ( 'NONE', ( #27778, #75629, #27689, #63250 ) ) ;
#6475=ORIENTED_EDGE ( 'NONE', *, *, #66651, .F. ) ;
#6483=CARTESIAN_POINT ( 'NONE',  ( 82.63223242006407077, 45.40567870588363064, 10.45052338476836873 ) ) ;
#6493=EDGE_CURVE ( 'NONE', #15032, #95607, #95796, .T. ) ;
#6494=CARTESIAN_POINT ( 'NONE',  ( 71.81276634784433099, 72.21619144530795609, 3.256612196116187352 ) ) ;
#6495=ADVANCED_FACE ( 'NONE', ( #56262 ), #8093, .T. ) ;
#6496=CARTESIAN_POINT ( 'NONE',  ( 84.58839726686360905, 45.66716180150288551, 9.521216735525740660 ) ) ;
#6497=CARTESIAN_POINT ( 'NONE',  ( 68.10039974585599509, 65.18542567973287305, -10.72853162865224519 ) ) ;
#6500=CARTESIAN_POINT ( 'NONE',  ( 82.53793375827495993, 54.22719885510827709, -15.94096427280454087 ) ) ;
#6503=CARTESIAN_POINT ( 'NONE',  ( 77.59577977556848793, 61.80410179206373300, 15.66623212455446890 ) ) ;
#6512=CARTESIAN_POINT ( 'NONE',  ( 41.88317952681261858, 32.38052372038644933, 10.00000000000000533 ) ) ;
#6514=CARTESIAN_POINT ( 'NONE',  ( 82.78960406368588565, 53.73890389198745510, 15.39558355803757728 ) ) ;
#6515=CARTESIAN_POINT ( 'NONE',  ( 71.92161918111298746, 71.97213927130549393, 2.836694015421989956 ) ) ;
#6521=CARTESIAN_POINT ( 'NONE',  ( 81.19178922867995141, 50.25691689511806004, -14.37495122601996655 ) ) ;
#6522=CARTESIAN_POINT ( 'NONE',  ( 72.02678134044498393, 72.22633079433387593, -1.610807377262633899 ) ) ;
#6524=CARTESIAN_POINT ( 'NONE',  ( 25.16147942602835030, 23.03085787977763843, 9.188101187500006262 ) ) ;
#6527=CARTESIAN_POINT ( 'NONE',  ( 44.85148386036637191, 26.86426979415093541, -3.090169943749474069 ) ) ;
#6533=CARTESIAN_POINT ( 'NONE',  ( 72.34119125645204917, 60.41698090225992956, 15.06063977213209881 ) ) ;
#6547=EDGE_LOOP ( 'NONE', ( #90408, #59140, #77188, #91238 ) ) ;
#6549=CARTESIAN_POINT ( 'NONE',  ( 79.30106977174941107, 46.37009440408895244, -12.77856967582355985 ) ) ;
#6550=CARTESIAN_POINT ( 'NONE',  ( 71.41016749218992743, 59.45273978182970609, 15.69346469599747174 ) ) ;
#6551=CARTESIAN_POINT ( 'NONE',  ( 84.83882459461941039, 41.93430961319199213, 2.331212101531141112 ) ) ;
#6555=CARTESIAN_POINT ( 'NONE',  ( 23.10466909204031083, 21.84335787977763133, 9.188101187500006262 ) ) ;
#6556=CARTESIAN_POINT ( 'NONE',  ( 75.52901062100019658, 57.36030880927751952, 16.09556828531399120 ) ) ;
#6557=CARTESIAN_POINT ( 'NONE',  ( 69.50278484786903732, 70.03302840163392773, -4.514860484484302994 ) ) ;
#6565=CARTESIAN_POINT ( 'NONE',  ( 78.96783115249304785, 50.21060704042795209, -14.86080133530415992 ) ) ;
#6571=CARTESIAN_POINT ( 'NONE',  ( 81.22503698233943226, 55.71330003141861198, 16.38398667929945773 ) ) ;
#6580=CARTESIAN_POINT ( 'NONE',  ( 72.27760156895793386, 60.37162225583013253, -15.57713023393894147 ) ) ;
#6587=CARTESIAN_POINT ( 'NONE',  ( 67.11284809570460652, 67.67925989217837923, 6.627993865167674414 ) ) ;
#6589=CARTESIAN_POINT ( 'NONE',  ( 81.53115339410010165, 41.92267797703283350, -7.515177224638171616 ) ) ;
#6590=CARTESIAN_POINT ( 'NONE',  ( 81.50373498261929228, 55.81176558511297969, 16.37496158676513858 ) ) ;
#6592=CARTESIAN_POINT ( 'NONE',  ( 71.24781679453236904, 66.22908028783459145, 11.48236923496973461 ) ) ;
#6593=CARTESIAN_POINT ( 'NONE',  ( 87.52489256634972037, 45.06004022996453529, 6.936227203615889181 ) ) ;
#6594=ORIENTED_EDGE ( 'NONE', *, *, #97048, .F. ) ;
#6597=CARTESIAN_POINT ( 'NONE',  ( 76.18516340950158394, 51.05281452121147368, -16.05953048902229341 ) ) ;
#6607=CARTESIAN_POINT ( 'NONE',  ( 86.99715697556658256, 45.94190566429735867, 8.138834009077100973 ) ) ;
#6610=CARTESIAN_POINT ( 'NONE',  ( 72.91771958014867039, 70.92947700147982459, 7.881516594485344918 ) ) ;
#6611=EDGE_CURVE ( 'NONE', #96074, #69981, #4947, .T. ) ;
#6612=CARTESIAN_POINT ( 'NONE',  ( 68.70919837959567644, 67.43310744183247607, -8.574709995985422495 ) ) ;
#6613=EDGE_LOOP ( 'NONE', ( #62285, #28371, #75099, #89383 ) ) ;
#6616=CARTESIAN_POINT ( 'NONE',  ( 72.26490814316112221, 71.11794692069462087, -6.031233613558444340 ) ) ;
#6618=CARTESIAN_POINT ( 'NONE',  ( 73.72239016385701404, 69.47467296629645261, -9.830903513004800587 ) ) ;
#6627=CARTESIAN_POINT ( 'NONE',  ( 27.36453209247643414, 17.92755873383626408, 6.180339887498953466 ) ) ;
#6630=CARTESIAN_POINT ( 'NONE',  ( 24.23155096423127475, 19.15404122711133894, 8.090169943749479842 ) ) ;
#6638=CARTESIAN_POINT ( 'NONE',  ( 67.08288010347953900, 67.73116597731298327, -6.493375440012594701 ) ) ;
#6639=CARTESIAN_POINT ( 'NONE',  ( 72.97800438629489861, 70.36521761891982862, -8.115508188870068196 ) ) ;
#6644=CARTESIAN_POINT ( 'NONE',  ( 32.72712820738424000, 19.86426979415091054, -3.090169943749474069 ) ) ;
#6645=CARTESIAN_POINT ( 'NONE',  ( 85.31730801475342219, 49.09321715058120361, 12.43107433435324616 ) ) ;
#6657=CARTESIAN_POINT ( 'NONE',  ( 39.32338737416051089, 38.10171378149922106, 9.188101187500008038 ) ) ;
#6664=CARTESIAN_POINT ( 'NONE',  ( 15.73863525846626032, 14.80170272979925272, 7.433330006724137462 ) ) ;
#6666=CARTESIAN_POINT ( 'NONE',  ( 71.91139111156488184, 59.09947579900738646, 15.37520130739997803 ) ) ;
#6670=CARTESIAN_POINT ( 'NONE',  ( 85.59433769663435498, 45.42763512727970010, -9.231865596844450295 ) ) ;
#6673=CARTESIAN_POINT ( 'NONE',  ( 6.396987757676564357, 15.64441083166258295, -10.00000000000000533 ) ) ;
#6674=CARTESIAN_POINT ( 'NONE',  ( 66.84604957904534217, 69.05321346016246764, 1.856603427880919366 ) ) ;
#6679=ORIENTED_EDGE ( 'NONE', *, *, #59058, .F. ) ;
#6685=CARTESIAN_POINT ( 'NONE',  ( 80.38256674825400694, 58.04436476229781761, -16.60504034864360179 ) ) ;
#6689=CARTESIAN_POINT ( 'NONE',  ( 87.66785150117509318, 45.41448820971019984, -6.605137624362326321 ) ) ;
#6692=CARTESIAN_POINT ( 'NONE',  ( 74.72968269109679795, 64.25080327513990142, 14.13526639238711979 ) ) ;
#6695=CARTESIAN_POINT ( 'NONE',  ( 78.34563248601955365, 47.34227125466418329, -14.25321530020122118 ) ) ;
#6713=CARTESIAN_POINT ( 'NONE',  ( 71.12867290548950905, 69.85259973772616604, 7.111628047231884686 ) ) ;
#6718=CARTESIAN_POINT ( 'NONE',  ( 78.26124923612431417, 47.74493931943022318, 13.93016830306222964 ) ) ;
#6722=CARTESIAN_POINT ( 'NONE',  ( 77.64951034529184426, 53.68749555020726660, -15.94746932111433857 ) ) ;
#6723=CARTESIAN_POINT ( 'NONE',  ( 82.89880969010835088, 40.77920605493923034, 2.125336176704005542 ) ) ;
#6724=CARTESIAN_POINT ( 'NONE',  ( 78.88804580972617941, 46.40278381930198037, 12.96229758350466810 ) ) ;
#6728=CARTESIAN_POINT ( 'NONE',  ( 79.14312167556931854, 57.64441083166269664, 0.000000000000000000 ) ) ;
#6743=CARTESIAN_POINT ( 'NONE',  ( 78.99848661620950452, 60.24637179098724005, -16.44349368446546222 ) ) ;
#6745=CARTESIAN_POINT ( 'NONE',  ( 72.62975712138512563, 68.37227089251233281, 10.30573641387579364 ) ) ;
#6746=PLANE ( 'NONE',  #33489 ) ;
#6747=B_SPLINE_SURFACE_WITH_KNOTS ( 'NONE', 3, 1, ( 
 ( #35362, #89621 ),
 ( #35861, #66759 ),
 ( #11589, #67257 ),
 ( #98183, #90104 ),
 ( #83002, #27772 ),
 ( #97690, #74885 ),
 ( #28258, #41967 ),
 ( #66272, #82524 ),
 ( #59646, #58646 ),
 ( #34852, #20183 ),
 ( #42448, #34370 ),
 ( #65756, #5469 ),
 ( #3494, #73383 ),
 ( #19692, #88634 ),
 ( #65267, #3969 ),
 ( #96211, #51050 ),
 ( #28764, #59133 ),
 ( #27278, #20675 ),
 ( #96710, #58160 ),
 ( #42936, #81508 ),
 ( #90617, #12078 ),
 ( #82009, #19200 ),
 ( #51564, #12583 ),
 ( #26774, #73875 ),
 ( #43456, #57655 ),
 ( #14569, #69246 ),
 ( #31240, #15530 ),
 ( #91588, #92590 ),
 ( #60633, #29760 ),
 ( #22159, #23134 ),
 ( #100174, #29270 ) ),
 .UNSPECIFIED., .F., .F., .F.,
 ( 4, 3, 3, 3, 3, 3, 3, 3, 3, 3, 4 ),
 ( 2, 2 ),
 ( 0.000000000000000000, 0.1333490885032394824, 0.3007194338854430882, 0.4699862290245251373, 0.5844252810809388299, 0.6686540514502711252, 0.7354980260655488156, 0.8028463152565757932, 0.8633854507757249275, 0.9437142632667384623, 1.000000000000000000 ),
 ( 0.000000000000000000, 1.000000000000000000 ),
 .UNSPECIFIED. ) ;
#6750=FACE_OUTER_BOUND ( 'NONE', #53772, .T. ) ;
#6752=CARTESIAN_POINT ( 'NONE',  ( 88.49573251350186354, 44.44521367694441949, 1.972556413651489717E-15 ) ) ;
#6754=ORIENTED_EDGE ( 'NONE', *, *, #48077, .T. ) ;
#6759=CARTESIAN_POINT ( 'NONE',  ( 13.67456932412660997, 8.864269794150878568, -3.090169943749474069 ) ) ;
#6762=CARTESIAN_POINT ( 'NONE',  ( 73.15133419349439237, 69.74273237385936852, 9.116647530793477117 ) ) ;
#6766=CARTESIAN_POINT ( 'NONE',  ( 72.94198659864277090, 57.16943012042473526, 15.90410001130455164 ) ) ;
#6767=CARTESIAN_POINT ( 'NONE',  ( 70.18403142648233484, 67.22621705619883414, 10.62750587675546576 ) ) ;
#6768=CARTESIAN_POINT ( 'NONE',  ( 66.45987627312771906, 68.25526039504281073, -4.355395359899360663 ) ) ;
#6774=CARTESIAN_POINT ( 'NONE',  ( 20.59861825492957621, 33.93396525600390845, 2.839279412974139660 ) ) ;
#6776=CARTESIAN_POINT ( 'NONE',  ( 83.74768966023471251, 52.21580090503303495, -15.05827679895701898 ) ) ;
#6777=DIRECTION ( 'NONE',  ( -0.6793907169778456989, 0.000000000000000000, 0.7337767056021393675 ) ) ;
#6778=CARTESIAN_POINT ( 'NONE',  ( 69.23475887354902625, 68.83203394105711936, 7.846736462262181355 ) ) ;
#6780=CARTESIAN_POINT ( 'NONE',  ( 68.72575050907364869, 64.26090759019037080, 12.49566804605334447 ) ) ;
#6784=CARTESIAN_POINT ( 'NONE',  ( 71.98645284171395531, 66.88534893327906161, -11.90698704647148531 ) ) ;
#6790=CARTESIAN_POINT ( 'NONE',  ( 71.80217098314240332, 72.17902961906311532, 0.5796836128640239227 ) ) ;
#6798=CARTESIAN_POINT ( 'NONE',  ( 17.30334773395576775, 15.15404122711132651, 8.090169943749479842 ) ) ;
#6803=CARTESIAN_POINT ( 'NONE',  ( 86.11128617339311120, 45.02157760453157920, -7.471804814321710175 ) ) ;
#6806=PLANE ( 'NONE',  #89668 ) ;
#6808=CARTESIAN_POINT ( 'NONE',  ( 69.40462582020063564, 62.82854907067461880, 13.14331805213147319 ) ) ;
#6814=CARTESIAN_POINT ( 'NONE',  ( 81.58540180393886487, 42.27212079091695784, -8.035051867169045181 ) ) ;
#6825=CARTESIAN_POINT ( 'NONE',  ( 82.86632025040690053, 53.49705537725820648, -15.32442982359594730 ) ) ;
#6827=CARTESIAN_POINT ( 'NONE',  ( 66.46320885748656337, 68.94986384069261476, 0.01364106734875079018 ) ) ;
#6828=CARTESIAN_POINT ( 'NONE',  ( 20.84336723938811176, 14.96004757982089828, -5.678558825948276656 ) ) ;
#6830=CARTESIAN_POINT ( 'NONE',  ( 80.65095556854913639, 57.57228308630150337, 16.58706730796346918 ) ) ;
#6842=CARTESIAN_POINT ( 'NONE',  ( 70.11758659987526698, 63.57919021067856846, -12.94399158718550069 ) ) ;
#6849=CARTESIAN_POINT ( 'NONE',  ( 87.93887446415499198, 44.76116579897428238, -4.704258403839747693 ) ) ;
#6850=CARTESIAN_POINT ( 'NONE',  ( 72.98735915780690675, 70.85324004147126686, 8.065790162528026386 ) ) ;
#6852=CARTESIAN_POINT ( 'NONE',  ( 32.90709467669683619, 21.12755873383627758, -6.180339887498949025 ) ) ;
#6858=CARTESIAN_POINT ( 'NONE',  ( 86.76444126019433156, 45.86660341771495553, -8.261827951889216592 ) ) ;
#6861=CARTESIAN_POINT ( 'NONE',  ( 83.81086367703072426, 45.25070890705758586, 9.560661162256756995 ) ) ;
#6866=CARTESIAN_POINT ( 'NONE',  ( 65.88310562893973099, 69.02589174555536999, 1.996831191813060347 ) ) ;
#6867=CARTESIAN_POINT ( 'NONE',  ( 78.58136487301973716, 53.95277478616699796, 15.90687120791058007 ) ) ;
#6878=CARTESIAN_POINT ( 'NONE',  ( 68.85610678100678683, 68.65685376360768544, 6.741963133850092049 ) ) ;
#6879=CARTESIAN_POINT ( 'NONE',  ( 67.00187114335926708, 67.08813303282481399, 8.529924657355552498 ) ) ;
#6880=CARTESIAN_POINT ( 'NONE',  ( 79.42866338260434134, 59.50128377535573776, 16.18467811310512872 ) ) ;
#6883=B_SPLINE_CURVE_WITH_KNOTS ( 'NONE', 3,
 ( #42848, #35273, #43858, #98086, #88046, #96623, #66179, #88540, #74799, #41875, #74310, #3404, #97123, #58562, #12493, #34278, #80938, #43360, #96125, #19103, #4891, #27188, #35772, #26679 ),
 .UNSPECIFIED., .F., .F.,
 ( 4, 2, 2, 2, 2, 2, 2, 2, 2, 2, 2, 4 ),
 ( 0.000000000000000000, 0.1249999999999770461, 0.2499999999999540923, 0.3749999999999311662, 0.4374999999999368283, 0.4999999999999424904, 0.5624999999999481526, 0.6249999999999537037, 0.6874999999999593658, 0.7499999999999649170, 0.8749999999999825695, 1.000000000000000000 ),
 .UNSPECIFIED. ) ;
#6886=CARTESIAN_POINT ( 'NONE',  ( 7.993722094130166766, 16.56628583063838533, 9.188101187500006262 ) ) ;
#6887=CARTESIAN_POINT ( 'NONE',  ( 80.20857538925844210, 44.21345027839176112, -11.30608575764589752 ) ) ;
#6888=DIRECTION ( 'NONE',  ( 0.5000000000000013323, -0.8660254037844378194, 0.000000000000000000 ) ) ;
#6890=CARTESIAN_POINT ( 'NONE',  ( 85.58122159723554034, 42.79555190012898436, -1.803223411638267493 ) ) ;
#6894=ADVANCED_FACE ( 'NONE', ( #12880 ), #5745, .T. ) ;
#6895=CARTESIAN_POINT ( 'NONE',  ( 44.05945362601616466, 27.29860640527295956, -2.839279412974138328 ) ) ;
#6897=FACE_BOUND ( 'NONE', #58603, .T. ) ;
#6899=CARTESIAN_POINT ( 'NONE',  ( 31.56043161122053320, 21.14754757982091249, -5.678558825948276656 ) ) ;
#6900=CARTESIAN_POINT ( 'NONE',  ( 73.85177649559180679, 63.65451359222425509, -14.63794785187609371 ) ) ;
#6904=CARTESIAN_POINT ( 'NONE',  ( 70.88562338225854376, 61.01594546643109851, 15.03711900572700877 ) ) ;
#6905=CARTESIAN_POINT ( 'NONE',  ( 75.97482311634344398, 65.22733265193998875, -14.46914695647701343 ) ) ;
#6912=CARTESIAN_POINT ( 'NONE',  ( 30.25658917092484756, 35.65586893147758474, -7.433330006724137462 ) ) ;
#6913=EDGE_LOOP ( 'NONE', ( #95348, #93355, #43011, #21885 ) ) ;
#6923=CARTESIAN_POINT ( 'NONE',  ( 36.96107555259132482, 29.84335787977765619, 9.188101187500006262 ) ) ;
#6924=CARTESIAN_POINT ( 'NONE',  ( 80.32771389996757705, 57.94408260071153194, -16.24746918486169633 ) ) ;
#6928=ORIENTED_EDGE ( 'NONE', *, *, #28905, .F. ) ;
#6929=ORIENTED_EDGE ( 'NONE', *, *, #34268, .F. ) ;
#6932=CARTESIAN_POINT ( 'NONE',  ( 79.76444659671797410, 57.08246710002341473, 16.23159459986195330 ) ) ;
#6936=CARTESIAN_POINT ( 'NONE',  ( 70.44156110210124666, 71.15467463549107663, 4.264815030697374887 ) ) ;
#6937=CARTESIAN_POINT ( 'NONE',  ( 76.73198439572453822, 60.14737954539558018, -15.86720150413332675 ) ) ;
#6940=CARTESIAN_POINT ( 'NONE',  ( 77.07812270435945834, 63.66946605146480209, -15.38604565157081794 ) ) ;
#6945=CARTESIAN_POINT ( 'NONE',  ( 43.97106342183892735, 31.10170272979931028, -7.433330006724141015 ) ) ;
#6949=ORIENTED_EDGE ( 'NONE', *, *, #21767, .T. ) ;
#6950=ADVANCED_FACE ( 'NONE', ( #6750 ), #24286, .T. ) ;
#6951=CARTESIAN_POINT ( 'NONE',  ( 73.84430631328980610, 68.30184443197676103, -11.60545323109705507 ) ) ;
#6957=CARTESIAN_POINT ( 'NONE',  ( 13.93250452138409479, 29.81751292744056059, -6.180339887498951690 ) ) ;
#6965=EDGE_CURVE ( 'NONE', #39921, #50534, #32024, .T. ) ;
#6975=B_SPLINE_SURFACE_WITH_KNOTS ( 'NONE', 3, 1, ( 
 ( #85711, #31433 ),
 ( #79089, #63347 ),
 ( #9672, #94285 ),
 ( #70445, #93280 ),
 ( #16746, #40533 ),
 ( #47634, #2058 ),
 ( #71467, #16246 ),
 ( #78567, #3566 ),
 ( #34446, #18262 ),
 ( #96793, #65345 ),
 ( #42526, #34933 ),
 ( #27353, #20255 ),
 ( #10659, #43016 ),
 ( #57234, #96284 ),
 ( #26853, #97276 ),
 ( #50631, #82092 ),
 ( #80595, #97762 ),
 ( #57728, #5052 ),
 ( #95804, #64857 ),
 ( #51130, #58235 ),
 ( #66834, #72975 ),
 ( #49157, #88708 ),
 ( #4043, #80092 ),
 ( #4540, #65828 ),
 ( #73955, #33973 ),
 ( #35932, #27843 ),
 ( #19763, #35440 ),
 ( #41535, #89215 ),
 ( #12665, #72479 ),
 ( #81098, #66343 ),
 ( #58720, #81585 ) ),
 .UNSPECIFIED., .F., .F., .F.,
 ( 4, 3, 3, 3, 3, 3, 3, 3, 3, 3, 4 ),
 ( 2, 2 ),
 ( 0.000000000000000000, 0.1122669598086814963, 0.2243161639709700950, 0.3396355846219198393, 0.4553962076585126861, 0.5677860799922443968, 0.6749047109689583213, 0.7773884377078411623, 0.8775581155834147884, 0.9782364162377933381, 1.000000000000000000 ),
 ( 0.000000000000000000, 1.000000000000000000 ),
 .UNSPECIFIED. ) ;
#6976=CARTESIAN_POINT ( 'NONE',  ( 73.30406195733340269, 68.46761453276084808, 10.59438808196635762 ) ) ;
#6980=CARTESIAN_POINT ( 'NONE',  ( 71.68255973785201718, 72.12657461437540007, 3.318624374305790603 ) ) ;
#6981=CARTESIAN_POINT ( 'NONE',  ( 83.76059554491119741, 44.12875889070350155, 8.054854059989002835 ) ) ;
#6983=CARTESIAN_POINT ( 'NONE',  ( 82.72605847261863232, 53.97080330652735825, -15.84526420522619539 ) ) ;
#6987=LINE ( 'NONE', #7479, #98083 ) ;
#6992=CARTESIAN_POINT ( 'NONE',  ( 76.56391922124960558, 51.24501030970186122, 16.05347363888732559 ) ) ;
#6993=B_SPLINE_CURVE_WITH_KNOTS ( 'NONE', 3,
 ( #14162, #29367, #22252, #76946, #52641, #98785, #22762, #28869, #61741, #82620, #99765, #30856, #68844, #90716, #84110, #52148 ),
 .UNSPECIFIED., .F., .F.,
 ( 4, 1, 2, 2, 2, 1, 2, 2, 4 ),
 ( 0.000000000000000000, 0.1250000000000023592, 0.1875000000000024980, 0.2500000000000026645, 0.5000000000000045519, 0.6250000000000039968, 0.6875000000000037748, 0.7500000000000034417, 1.000000000000000000 ),
 .UNSPECIFIED. ) ;
#6998=CARTESIAN_POINT ( 'NONE',  ( 72.23865006290041890, 71.95475215217993536, 3.607730569270008125 ) ) ;
#7002=CARTESIAN_POINT ( 'NONE',  ( 46.78603705595332229, 27.41603393254330712, -1.583844403245396437 ) ) ;
#7003=CARTESIAN_POINT ( 'NONE',  ( 82.32019150160303411, 49.92528730339438425, -13.92079164607254071 ) ) ;
#7008=CARTESIAN_POINT ( 'NONE',  ( 22.00287929847174695, 28.10171378149919263, 9.188101187500008038 ) ) ;
#7011=CARTESIAN_POINT ( 'NONE',  ( 14.23992353553176926, 11.14754757982088407, -5.678558825948276656 ) ) ;
#7013=CARTESIAN_POINT ( 'NONE',  ( 76.95477351241487440, 63.69079797318030955, 15.35326628456841824 ) ) ;
#7023=EDGE_LOOP ( 'NONE', ( #78278, #84620, #89349, #5803 ) ) ;
#7025=CARTESIAN_POINT ( 'NONE',  ( 77.30051420685094854, 49.22732157280278642, 15.33771541198130350 ) ) ;
#7035=B_SPLINE_CURVE_WITH_KNOTS ( 'NONE', 3,
 ( #40011, #48648, #63331, #24337, #86691, #62311, #85177, #85696, #31920, #70431, #71452, #79583, #55214, #39015, #87213, #46622, #2041, #94768, #10144, #93779, #41009, #78550, #77552, #9138 ),
 .UNSPECIFIED., .F., .F.,
 ( 4, 2, 2, 2, 2, 2, 2, 2, 2, 2, 2, 4 ),
 ( 0.000000000000000000, 0.1250000000000209277, 0.2500000000000418554, 0.3750000000000627831, 0.4375000000000565104, 0.5000000000000502931, 0.5625000000000439648, 0.6250000000000376366, 0.6875000000000314193, 0.7500000000000250910, 0.8750000000000125455, 1.000000000000000000 ),
 .UNSPECIFIED. ) ;
#7040=CARTESIAN_POINT ( 'NONE',  ( 18.65184876021338312, 28.95586893147755703, 7.433330006724141015 ) ) ;
#7051=CARTESIAN_POINT ( 'NONE',  ( 68.06773744437363405, 65.18829879967773877, -10.70695411350301818 ) ) ;
#7068=CARTESIAN_POINT ( 'NONE',  ( 67.15236828973634431, 67.72320738538478224, 6.588214651295674074 ) ) ;
#7071=CARTESIAN_POINT ( 'NONE',  ( 68.02005152741377003, 65.43521726584035036, 10.42530429588983054 ) ) ;
#7073=CARTESIAN_POINT ( 'NONE',  ( 70.18763995946753198, 63.26540913664066323, 13.15406633596375485 ) ) ;
#7077=VERTEX_POINT ( 'NONE', #73056 ) ;
#7078=CARTESIAN_POINT ( 'NONE',  ( 76.07595347892329585, 51.40484473107772345, -15.65947719172055486 ) ) ;
#7081=CARTESIAN_POINT ( 'NONE',  ( 75.88031102442633369, 65.78928292664191702, -14.15509851726639390 ) ) ;
#7088=CARTESIAN_POINT ( 'NONE',  ( 87.75230366022445594, 44.21248639555269477, 4.670146826978181842 ) ) ;
#7092=CARTESIAN_POINT ( 'NONE',  ( 87.97614123416462917, 44.06541336701370426, -1.724168466821650147 ) ) ;
#7094=CARTESIAN_POINT ( 'NONE',  ( 72.67799729538583620, 70.93760247754363490, 7.641220802698796888 ) ) ;
#7096=CARTESIAN_POINT ( 'NONE',  ( 68.45771554780012025, 67.43233330954889482, -8.366793215440479159 ) ) ;
#7100=CARTESIAN_POINT ( 'NONE',  ( 72.35093020053528790, 71.14706991326251284, -6.078630472467451362 ) ) ;
#7104=AXIS2_PLACEMENT_3D ( 'NONE', #35213, #58500, #89473 ) ;
#7105=LINE ( 'NONE', #76042, #38425 ) ;
#7110=CARTESIAN_POINT ( 'NONE',  ( 25.44954664093420149, 26.64441083166262203, -10.00000000000000533 ) ) ;
#7113=CARTESIAN_POINT ( 'NONE',  ( 15.73079442999205924, 32.58029201028040944, 1.583844403245363353 ) ) ;
#7118=CARTESIAN_POINT ( 'NONE',  ( 66.73473034183035679, 67.48348876847576605, -6.586817036978919404 ) ) ;
#7119=CARTESIAN_POINT ( 'NONE',  ( 72.54816569808835425, 70.68207713539275971, -7.935695741106848722 ) ) ;
#7121=CARTESIAN_POINT ( 'NONE',  ( 81.62507666485218749, 41.61289278366178479, 5.610847245266504579 ) ) ;
#7123=CARTESIAN_POINT ( 'NONE',  ( 21.20711791317337003, 34.01751292744057054, 6.180339887498949913 ) ) ;
#7124=CARTESIAN_POINT ( 'NONE',  ( 74.15479259499207387, 55.62765001666249276, -16.59030973340311022 ) ) ;
#7136=CARTESIAN_POINT ( 'NONE',  ( 41.76871284172324295, 36.06628583063844928, -9.188101187500006262 ) ) ;
#7138=EDGE_CURVE ( 'NONE', #46017, #14068, #4579, .T. ) ;
#7144=CARTESIAN_POINT ( 'NONE',  ( 18.92729281690869314, 22.87878583063841020, -9.188101187500006262 ) ) ;
#7145=CARTESIAN_POINT ( 'NONE',  ( 13.76346889243896321, 13.11029122506292843, -8.090169943749478065 ) ) ;
#7146=CARTESIAN_POINT ( 'NONE',  ( 71.84836080304555139, 59.06364556286701628, 15.87505501405348340 ) ) ;
#7150=CARTESIAN_POINT ( 'NONE',  ( 87.08523622459452440, 45.32592727123765286, -7.867701777046974598 ) ) ;
#7152=CARTESIAN_POINT ( 'NONE',  ( 81.87175288788205307, 42.17655061954369700, 7.612090732984669650 ) ) ;
#7156=CARTESIAN_POINT ( 'NONE',  ( 69.42645013659684139, 70.63508196826001040, -1.496691613166120982 ) ) ;
#7157=CARTESIAN_POINT ( 'NONE',  ( 76.63732740674304011, 63.83366213508917753, 14.86362707207269551 ) ) ;
#7160=ORIENTED_EDGE ( 'NONE', *, *, #55084, .T. ) ;
#7162=CARTESIAN_POINT ( 'NONE',  ( 80.74974841587442143, 43.27611110060701805, 10.01619596027649095 ) ) ;
#7164=VERTEX_POINT ( 'NONE', #28935 ) ;
#7166=CARTESIAN_POINT ( 'NONE',  ( 71.18266754637075167, 67.94496896153198406, 10.47851208213521446 ) ) ;
#7167=CARTESIAN_POINT ( 'NONE',  ( 80.22399782384964340, 57.81478883376428257, 16.60249858296848657 ) ) ;
#7173=EDGE_LOOP ( 'NONE', ( #69366, #3079, #91309, #12802 ) ) ;
#7179=CARTESIAN_POINT ( 'NONE',  ( 81.60871807086439844, 59.37387260405306932, -0.4240240480782162535 ) ) ;
#7184=CARTESIAN_POINT ( 'NONE',  ( 83.75851852475534542, 52.19494488360223983, 14.66139263155008798 ) ) ;
#7188=CARTESIAN_POINT ( 'NONE',  ( 86.54292033101232562, 46.25028892199808439, 8.970843135639702481 ) ) ;
#7189=CARTESIAN_POINT ( 'NONE',  ( 79.70677143361787387, 46.01134058561530793, 12.98241517792750699 ) ) ;
#7191=CARTESIAN_POINT ( 'NONE',  ( 82.33309958831539177, 53.73407448881687287, 15.84243556053685431 ) ) ;
#7198=CARTESIAN_POINT ( 'NONE',  ( 69.05858150271376417, 65.60398784760005242, 10.87676190501699836 ) ) ;
#7203=CARTESIAN_POINT ( 'NONE',  ( 78.44703544257603767, 47.42314817051035902, 14.26473360639000987 ) ) ;
#7206=CARTESIAN_POINT ( 'NONE',  ( 80.04801989711464216, 52.84706496129958708, -15.53468051483373991 ) ) ;
#7209=CARTESIAN_POINT ( 'NONE',  ( 79.17243950938065211, 45.84086033299786322, 13.07686966769901638 ) ) ;
#7214=CARTESIAN_POINT ( 'NONE',  ( 80.20448007545800806, 58.22194284664072939, -16.60717859687067843 ) ) ;
#7216=CARTESIAN_POINT ( 'NONE',  ( 72.56735714755242839, 71.56619014045929816, 5.379842731025054725 ) ) ;
#7220=CARTESIAN_POINT ( 'NONE',  ( 66.79023490949526831, 67.33564584442949297, -6.933441031880490435 ) ) ;
#7224=CARTESIAN_POINT ( 'NONE',  ( 82.20387338395363486, 40.63080856265045782, 3.356284137154774694 ) ) ;
#7227=CARTESIAN_POINT ( 'NONE',  ( 71.72736245888779649, 65.63246871389105763, 12.21051025674438506 ) ) ;
#7244=CARTESIAN_POINT ( 'NONE',  ( 8.399671500380161859, 16.80066082961419482, 10.00000000000000533 ) ) ;
#7246=CARTESIAN_POINT ( 'NONE',  ( 71.57792465326454590, 59.00132549361326539, -15.84990762337844572 ) ) ;
#7247=CARTESIAN_POINT ( 'NONE',  ( 73.17900167297862879, 69.84980244707995212, 9.598651498403647508 ) ) ;
#7252=CARTESIAN_POINT ( 'NONE',  ( 71.55555785148570180, 70.00198118308297524, 8.105299072955192585 ) ) ;
#7253=CARTESIAN_POINT ( 'NONE',  ( 8.207198731066840836, 28.23654200823201066, 1.583844403245363353 ) ) ;
#7260=CARTESIAN_POINT ( 'NONE',  ( 32.08968265630385019, 27.03085787977765264, 9.188101187500006262 ) ) ;
#7265=CARTESIAN_POINT ( 'NONE',  ( 68.31860697027661899, 67.22880204738007137, 9.390919083417214708 ) ) ;
#7267=CARTESIAN_POINT ( 'NONE',  ( 68.58219988125976840, 64.16363137176722375, 11.86921294676530891 ) ) ;
#7271=FACE_OUTER_BOUND ( 'NONE', #5084, .T. ) ;
#7273=CARTESIAN_POINT ( 'NONE',  ( 8.301057521190555732, 26.83396525600388571, -2.839279412974133887 ) ) ;
#7279=CARTESIAN_POINT ( 'NONE',  ( 71.75944102250285539, 72.15356206472488054, 0.5915691668053513208 ) ) ;
#7292=CARTESIAN_POINT ( 'NONE',  ( 82.19618238725253434, 45.38674811654465913, -10.67622378202659483 ) ) ;
#7296=CARTESIAN_POINT ( 'NONE',  ( 79.25704083171594050, 59.98661423191556707, -16.48971415753126735 ) ) ;
#7299=CARTESIAN_POINT ( 'NONE',  ( 69.98626866712953642, 62.70234947095676148, 13.41362294286624923 ) ) ;
#7303=CARTESIAN_POINT ( 'NONE',  ( 73.40082382908687464, 69.73317320774677341, -9.891058063621702701 ) ) ;
#7305=CARTESIAN_POINT ( 'NONE',  ( 81.41048206884038052, 42.10864841836186656, -7.936452042242466476 ) ) ;
#7306=VERTEX_POINT ( 'NONE', #76534 ) ;
#7307=VERTEX_POINT ( 'NONE', #92750 ) ;
#7309=CARTESIAN_POINT ( 'NONE',  ( 80.79947158083696479, 47.80592219649970076, 13.19143189947888750 ) ) ;
#7316=DIRECTION ( 'NONE',  ( 0.000000000000000000, 0.000000000000000000, -1.000000000000000000 ) ) ;
#7318=CARTESIAN_POINT ( 'NONE',  ( 80.93613592869992601, 42.95327845849681836, -9.503115154567232992 ) ) ;
#7320=CARTESIAN_POINT ( 'NONE',  ( 70.42618839682489806, 68.43364653649702234, -8.625854842549946611 ) ) ;
#7321=CARTESIAN_POINT ( 'NONE',  ( 79.11723855630626190, 59.11194703662724237, -16.21433712332713029 ) ) ;
#7322=CARTESIAN_POINT ( 'NONE',  ( 13.89352694080530171, 28.99752408145591076, 5.678558825948277544 ) ) ;
#7324=CARTESIAN_POINT ( 'NONE',  ( 80.14478464935454838, 57.78471241749841170, 16.60281329265515637 ) ) ;
#7330=CARTESIAN_POINT ( 'NONE',  ( 77.23208049594958879, 49.18074735263096642, -15.33539087807836765 ) ) ;
#7331=CARTESIAN_POINT ( 'NONE',  ( 68.11396990072299218, 66.09066184265174115, -10.54551009852403709 ) ) ;
#7340=B_SPLINE_CURVE_WITH_KNOTS ( 'NONE', 3,
 ( #95055, #25616, #56501, #87488, #77313, #70191, #23588, #46904, #801, #62586, #26116, #48917, #65599, #26614, #72744, #50399, #87975, #41288, #35199, #4296, #49406, #73223, #80353, #33725, #11923, #96549, #49906, #58002, #57492, #80864, #79853 ),
 .UNSPECIFIED., .F., .F.,
 ( 4, 3, 3, 3, 3, 3, 3, 3, 3, 3, 4 ),
 ( 0.000000000000000000, 0.1333490885032317108, 0.3007194338854392579, 0.4699862290245125918, 0.5844252810809411613, 0.6686540514502808952, 0.7354980260655639146, 0.8028463152565747940, 0.8633854507757208196, 0.9437142632667219200, 1.000000000000000000 ),
 .UNSPECIFIED. ) ;
#7342=CARTESIAN_POINT ( 'NONE',  ( 72.04401715163407971, 72.30798015014887881, 0.7277735660157971243 ) ) ;
#7355=CARTESIAN_POINT ( 'NONE',  ( 84.44632881057094664, 46.78574307426487167, 10.85411661781247084 ) ) ;
#7359=FACE_OUTER_BOUND ( 'NONE', #18145, .T. ) ;
#7364=CARTESIAN_POINT ( 'NONE',  ( 80.64483776220907885, 57.31469717126433494, -16.23318395240539758 ) ) ;
#7365=CARTESIAN_POINT ( 'NONE',  ( 68.52821507787726318, 64.25720321475604635, -12.41134622814902322 ) ) ;
#7372=CARTESIAN_POINT ( 'NONE',  ( 68.99418107762870989, 68.85582864506679357, 6.521622189437183081 ) ) ;
#7380=CARTESIAN_POINT ( 'NONE',  ( 11.76515913632831101, 28.83396525600389282, -2.839279412974133887 ) ) ;
#7381=CARTESIAN_POINT ( 'NONE',  ( 71.82426268295279215, 61.16778308377749340, -15.19677902312525219 ) ) ;
#7388=CARTESIAN_POINT ( 'NONE',  ( 40.83172133312034191, 29.28920272979929962, -7.433330006724141015 ) ) ;
#7390=FACE_BOUND ( 'NONE', #72110, .T. ) ;
#7392=CARTESIAN_POINT ( 'NONE',  ( 27.58635055662477953, 24.43085787977765122, -9.188101187500008038 ) ) ;
#7403=ORIENTED_EDGE ( 'NONE', *, *, #58194, .F. ) ;
#7404=CARTESIAN_POINT ( 'NONE',  ( 79.22511366827423274, 47.14223421634689970, -13.88362136263801005 ) ) ;
#7406=CARTESIAN_POINT ( 'NONE',  ( 30.33837380989695731, 32.91421378149920685, 9.188101187500008038 ) ) ;
#7410=CARTESIAN_POINT ( 'NONE',  ( 86.76627553996233644, 43.48886326763260968, 2.108659042064822575 ) ) ;
#7411=VERTEX_POINT ( 'NONE', #87195 ) ;
#7412=CARTESIAN_POINT ( 'NONE',  ( 86.32721218574307898, 47.55264674982593220, -11.12316258729872054 ) ) ;
#7414=CARTESIAN_POINT ( 'NONE',  ( 84.71425524834847920, 50.25098136614051469, 13.83365903171529077 ) ) ;
#7420=CARTESIAN_POINT ( 'NONE',  ( 81.54078422002766047, 55.47956193386177404, -16.32023236213573014 ) ) ;
#7428=CARTESIAN_POINT ( 'NONE',  ( 84.39448865303761238, 50.06170295690048988, 13.83095091856771219 ) ) ;
#7433=CARTESIAN_POINT ( 'NONE',  ( 72.26813344353081447, 61.62913406889816059, -14.61747620878596265 ) ) ;
#7434=CARTESIAN_POINT ( 'NONE',  ( 82.51358517225706635, 41.00440080157959954, 1.051676170051975223 ) ) ;
#7436=CARTESIAN_POINT ( 'NONE',  ( 77.02263550477385934, 63.85671778288190836, -15.30752586418454086 ) ) ;
#7441=CARTESIAN_POINT ( 'NONE',  ( 41.62797693021462209, 26.96004757982093381, -5.678558825948276656 ) ) ;
#7443=VERTEX_POINT ( 'NONE', #28184 ) ;
#7446=CARTESIAN_POINT ( 'NONE',  ( 72.22311968498431156, 63.76148163533759572, -13.58264511429491783 ) ) ;
#7449=CARTESIAN_POINT ( 'NONE',  ( 28.51231065420501309, 32.16454794089043645, -10.00000000000000355 ) ) ;
#7450=CARTESIAN_POINT ( 'NONE',  ( 74.06060638490031067, 55.49390267324601922, -16.11553875424677074 ) ) ;
#7455=CARTESIAN_POINT ( 'NONE',  ( 79.22526226284777806, 49.23273016502245980, 14.90489237802606759 ) ) ;
#7456=DIRECTION ( 'NONE',  ( -0.8660254037844378194, -0.5000000000000014433, -0.000000000000000000 ) ) ;
#7462=CARTESIAN_POINT ( 'NONE',  ( 81.32600941128136185, 42.90402669303311711, 8.279988871130893102 ) ) ;
#7469=CARTESIAN_POINT ( 'NONE',  ( 82.25663186038693198, 41.25091070164440055, -3.462110524831779834 ) ) ;
#7472=CARTESIAN_POINT ( 'NONE',  ( 82.66671967738665217, 42.53264105941079265, 6.324155599994208288 ) ) ;
#7473=CARTESIAN_POINT ( 'NONE',  ( 22.51478983128357925, 15.12755873383625982, -6.180339887498949025 ) ) ;
#7475=CARTESIAN_POINT ( 'NONE',  ( 82.57676729861134390, 54.19068042909008653, -15.92587557605580706 ) ) ;
#7479=CARTESIAN_POINT ( 'NONE',  ( 65.92723761088207368, 68.94945291059252668, -2.624861928015914003 ) ) ;
#7482=CARTESIAN_POINT ( 'NONE',  ( 78.72787672744944132, 47.58481813695765084, 14.26461805045499531 ) ) ;
#7487=CARTESIAN_POINT ( 'NONE',  ( 73.49482902488119862, 69.19712283778764572, -10.00323161215957768 ) ) ;
#7488=CARTESIAN_POINT ( 'NONE',  ( 76.25812641337097375, 51.35648307871889529, 15.62532910699416000 ) ) ;
#7501=CARTESIAN_POINT ( 'NONE',  ( 21.85012855468117721, 24.56628583063841376, 9.188101187500006262 ) ) ;
#7505=CARTESIAN_POINT ( 'NONE',  ( 9.796739006517501736, 23.84336893147754566, -7.433330006724137462 ) ) ;
#7507=CARTESIAN_POINT ( 'NONE',  ( 76.88515868761567162, 63.85673109229074385, 14.90669629514164463 ) ) ;
#7515=CARTESIAN_POINT ( 'NONE',  ( 78.88977525980774885, 55.53746465279655808, -16.10141863661490191 ) ) ;
#7516=CARTESIAN_POINT ( 'NONE',  ( 87.78256729009754622, 45.12882416216076820, -6.783508070075447982 ) ) ;
#7520=ORIENTED_EDGE ( 'NONE', *, *, #20042, .F. ) ;
#7521=CARTESIAN_POINT ( 'NONE',  ( 76.94662761810361928, 49.67608497600890871, 15.05378093682414509 ) ) ;
#7522=CARTESIAN_POINT ( 'NONE',  ( 82.66218641157266234, 53.85062555766313608, 15.82228755104997120 ) ) ;
#7537=CARTESIAN_POINT ( 'NONE',  ( 22.95008440877049338, 15.11110640527292226, -2.839279412974138328 ) ) ;
#7538=CARTESIAN_POINT ( 'NONE',  ( 75.71249384252782022, 58.31751109039055336, 16.01915597449171358 ) ) ;
#7547=CARTESIAN_POINT ( 'NONE',  ( 68.29626403325076467, 65.68998705335020816, -10.32719566005510181 ) ) ;
#7559=CARTESIAN_POINT ( 'NONE',  ( 13.35896364390118052, 31.21091486745859811, -1.111400068045478839E-16 ) ) ;
#7561=AXIS2_PLACEMENT_3D ( 'NONE', #72825, #3418, #34777 ) ;
#7562=ORIENTED_EDGE ( 'NONE', *, *, #81631, .T. ) ;
#7567=CARTESIAN_POINT ( 'NONE',  ( 67.15984093255737264, 67.73264523994713215, 6.578533426557070740 ) ) ;
#7572=CARTESIAN_POINT ( 'NONE',  ( 80.97708524682441578, 55.98081928642064753, 16.09453298904065832 ) ) ;
#7574=VECTOR ( 'NONE', #79278, 1000.000000000000000 ) ;
#7575=CARTESIAN_POINT ( 'NONE',  ( 71.72731785887494027, 67.47519123564113386, 10.61382998831304114 ) ) ;
#7581=CARTESIAN_POINT ( 'NONE',  ( 76.38099514367294773, 51.62635831307756007, -15.66874856699700835 ) ) ;
#7582=CARTESIAN_POINT ( 'NONE',  ( 76.27580996045810480, 65.11309384637550579, -14.21297909825325156 ) ) ;
#7590=CARTESIAN_POINT ( 'NONE',  ( 82.05742212450444129, 43.66019292712455524, -8.741533095782198615 ) ) ;
#7591=DIRECTION ( 'NONE',  ( -0.1039558454088829048, 0.1800568059919617214, 0.9781476007338041345 ) ) ;
#7593=CARTESIAN_POINT ( 'NONE',  ( 38.12578301810894033, 22.41603393254328935, -1.583844403245396437 ) ) ;
#7595=VECTOR ( 'NONE', #44915, 1000.000000000000114 ) ;
#7596=CARTESIAN_POINT ( 'NONE',  ( 72.62753967730402849, 70.91775434214520146, 7.625672695449478233 ) ) ;
#7597=CARTESIAN_POINT ( 'NONE',  ( 74.10896984709266633, 66.64336536303099479, -12.55719438977912894 ) ) ;
#7598=ORIENTED_EDGE ( 'NONE', *, *, #21938, .T. ) ;
#7601=CARTESIAN_POINT ( 'NONE',  ( 82.22237228838635303, 40.83607612262022002, 1.050915814309854479 ) ) ;
#7602=CARTESIAN_POINT ( 'NONE',  ( 80.24968131911825253, 48.58851929088046262, 13.79783264785077179 ) ) ;
#7611=CARTESIAN_POINT ( 'NONE',  ( 74.09603869131957765, 55.10132886373268946, 16.60403961883766755 ) ) ;
#7612=CARTESIAN_POINT ( 'NONE',  ( 21.04067422097218909, 35.08080186712593473, -3.090169943749475845 ) ) ;
#7623=CARTESIAN_POINT ( 'NONE',  ( 81.59433360772331412, 41.62595464265170619, 5.684377094819374143 ) ) ;
#7626=VECTOR ( 'NONE', #30044, 1000.000000000000114 ) ;
#7628=CARTESIAN_POINT ( 'NONE',  ( 34.87460501429023907, 19.94473085651394584, 1.475505719884397138E-15 ) ) ;
#7629=CARTESIAN_POINT ( 'NONE',  ( 83.07478186481714033, 41.77647167697862329, -3.762335041875428665 ) ) ;
#7638=CARTESIAN_POINT ( 'NONE',  ( 34.18796084459998497, 43.23654200823204263, 1.583844403245397769 ) ) ;
#7641=CARTESIAN_POINT ( 'NONE',  ( 67.34360286252885430, 66.37718443452089900, -8.893619794688017777 ) ) ;
#7646=EDGE_CURVE ( 'NONE', #71488, #58166, #68624, .T. ) ;
#7651=CARTESIAN_POINT ( 'NONE',  ( 21.45440292344354916, 18.10170272979926764, -7.433330006724141015 ) ) ;
#7652=CARTESIAN_POINT ( 'NONE',  ( 7.004301291108590455, 25.81751292744054282, -6.180339887498951690 ) ) ;
#7653=CARTESIAN_POINT ( 'NONE',  ( 72.04273812837081437, 59.28583566120335036, 15.84548535924249890 ) ) ;
#7658=ADVANCED_FACE ( 'NONE', ( #51872 ), #34214, .T. ) ;
#7660=CARTESIAN_POINT ( 'NONE',  ( 73.62988499754025895, 59.71431543555856791, -15.50958422211314769 ) ) ;
#7661=CARTESIAN_POINT ( 'NONE',  ( 81.33432549305550197, 42.42221510689188335, 7.504012747830186569 ) ) ;
#7664=ORIENTED_EDGE ( 'NONE', *, *, #85464, .F. ) ;
#7666=CARTESIAN_POINT ( 'NONE',  ( 71.62184359327899585, 71.38130220946494831, -4.266802885512482213 ) ) ;
#7667=CARTESIAN_POINT ( 'NONE',  ( 72.93869098254521077, 57.08676652230623461, 16.39928802407133190 ) ) ;
#7668=CARTESIAN_POINT ( 'NONE',  ( 83.78898797060510617, 41.32812536727200836, 2.261347060406205589 ) ) ;
#7673=CARTESIAN_POINT ( 'NONE',  ( 82.90655991062965313, 42.38495858070367461, -5.749555441042302206 ) ) ;
#7677=CARTESIAN_POINT ( 'NONE',  ( 79.83586840751161162, 57.89405847684007256, 16.26501041126315528 ) ) ;
#7688=VERTEX_POINT ( 'NONE', #99367 ) ;
#7690=CARTESIAN_POINT ( 'NONE',  ( 34.88136640284594847, 21.10801979619931146, 3.090169943749476733 ) ) ;
#7702=DIRECTION ( 'NONE',  ( 0.4996954135095463823, -0.8654978445076774163, -0.03489949670249753444 ) ) ;
#7706=CARTESIAN_POINT ( 'NONE',  ( 67.19619177694202961, 66.60445450608504814, 8.464027507732211575 ) ) ;
#7707=CARTESIAN_POINT ( 'NONE',  ( 72.55717859591010210, 65.07642316054428022, -12.92391924280964588 ) ) ;
#7708=CARTESIAN_POINT ( 'NONE',  ( 78.67232457920248123, 47.52898336996674544, 14.25219103194631032 ) ) ;
#7712=CARTESIAN_POINT ( 'NONE',  ( 83.16083141524212863, 41.41346057833686700, -1.656387949955075323 ) ) ;
#7713=CARTESIAN_POINT ( 'NONE',  ( 87.74379322371484591, 45.04902437494477851, -6.671288900681476619 ) ) ;
#7714=CARTESIAN_POINT ( 'NONE',  ( 79.38855964867086357, 46.21855749211306374, 12.64186050921641957 ) ) ;
#7719=VERTEX_POINT ( 'NONE', #29946 ) ;
#7722=CARTESIAN_POINT ( 'NONE',  ( 72.34273340409356479, 71.56583958283731306, 5.071847820242139981 ) ) ;
#7725=EDGE_CURVE ( 'NONE', #90569, #18043, #62500, .T. ) ;
#7736=LINE ( 'NONE', #62412, #94816 ) ;
#7739=CARTESIAN_POINT ( 'NONE',  ( 73.18372135689499203, 60.26031415148027293, 15.75792897287434435 ) ) ;
#7750=CARTESIAN_POINT ( 'NONE',  ( 85.05033292184569405, 46.62834512446820412, -10.94201510068669414 ) ) ;
#7752=CARTESIAN_POINT ( 'NONE',  ( 10.46840290624634306, 27.81751292744054993, -6.180339887498951690 ) ) ;
#7759=CARTESIAN_POINT ( 'NONE',  ( 73.01029701701182262, 57.12463796210177236, 16.39976797707190315 ) ) ;
#7761=CARTESIAN_POINT ( 'NONE',  ( 66.70287695511908055, 68.38935073730952752, -4.375220962393981061 ) ) ;
#7763=ADVANCED_FACE ( 'NONE', ( #8151 ), #86702, .T. ) ;
#7769=CARTESIAN_POINT ( 'NONE',  ( 36.75658403392715456, 24.14754757982092315, -5.678558825948276656 ) ) ;
#7770=DIRECTION ( 'NONE',  ( -0.8660254037844379305, -0.5000000000000014433, -0.000000000000000000 ) ) ;
#7774=CARTESIAN_POINT ( 'NONE',  ( 88.42017002704760387, 43.92753743058676719, 1.721442031696316377 ) ) ;
#7776=CARTESIAN_POINT ( 'NONE',  ( 66.17642628206915845, 69.10264375944338155, 2.573923083425510239 ) ) ;
#7778=CARTESIAN_POINT ( 'NONE',  ( 81.42668684898659137, 52.12787871455454081, 15.51728826852514587 ) ) ;
#7782=CARTESIAN_POINT ( 'NONE',  ( 11.99789328850488879, 15.43085787977761214, -9.188101187500008038 ) ) ;
#7783=EDGE_LOOP ( 'NONE', ( #72377, #54402, #75895, #30848 ) ) ;
#7794=ORIENTED_EDGE ( 'NONE', *, *, #25882, .T. ) ;
#7798=CARTESIAN_POINT ( 'NONE',  ( 73.04137136423049981, 70.75758827781731952, 7.534468892676039253 ) ) ;
#7799=ORIENTED_EDGE ( 'NONE', *, *, #28444, .F. ) ;
#7802=CARTESIAN_POINT ( 'NONE',  ( 84.74040462907180427, 45.11266949017006311, -8.735513756553579867 ) ) ;
#7805=CARTESIAN_POINT ( 'NONE',  ( 79.32558605478152458, 59.69129752972264669, -16.52184683405511834 ) ) ;
#7806=VECTOR ( 'NONE', #24913, 1000.000000000000114 ) ;
#7808=CARTESIAN_POINT ( 'NONE',  ( 69.81793561852694552, 62.72544707633330319, 13.91621835302064447 ) ) ;
#7816=ORIENTED_EDGE ( 'NONE', *, *, #22121, .T. ) ;
#7818=CARTESIAN_POINT ( 'NONE',  ( 73.43380971014073566, 61.55604703159713864, 14.92230597848644358 ) ) ;
#7821=CARTESIAN_POINT ( 'NONE',  ( 87.85893154554855755, 45.08040635541048857, 6.601944857759019847 ) ) ;
#7825=CYLINDRICAL_SURFACE ( 'NONE', #75652, 16.60714546451156792 ) ;
#7830=CARTESIAN_POINT ( 'NONE',  ( 82.74681249865726329, 53.90498867430740404, -15.82393922498146921 ) ) ;
#7833=CARTESIAN_POINT ( 'NONE',  ( 10.42942532566755354, 26.99752408145590721, 5.678558825948277544 ) ) ;
#7835=CARTESIAN_POINT ( 'NONE',  ( 33.00691499580853616, 42.55466486950702887, 7.012934429366973338E-14 ) ) ;
#7841=CARTESIAN_POINT ( 'NONE',  ( 80.08958074560355556, 44.70221173755660971, 11.12270814150613241 ) ) ;
#7842=CARTESIAN_POINT ( 'NONE',  ( 81.59622370732601837, 46.04426866650761241, -11.56528914279085996 ) ) ;
#7847=CARTESIAN_POINT ( 'NONE',  ( 75.06349586682163988, 67.01194365216522897, -13.14257922886206487 ) ) ;
#7867=CARTESIAN_POINT ( 'NONE',  ( 85.04690354554347209, 46.11796720474825406, -9.797488362679569462 ) ) ;
#7873=CARTESIAN_POINT ( 'NONE',  ( 82.79468719140261612, 43.39660814947434631, 7.776906916868496111 ) ) ;
#7891=CARTESIAN_POINT ( 'NONE',  ( 69.54386771901253894, 69.60617901769191462, 5.634068191784291635 ) ) ;
#7896=EDGE_CURVE ( 'NONE', #94177, #57995, #74956, .T. ) ;
#7900=CARTESIAN_POINT ( 'NONE',  ( 17.35761498915574563, 12.94754757982088300, 5.678558825948272215 ) ) ;
#7902=DIRECTION ( 'NONE',  ( 0.000000000000000000, 0.3470917258701495256, -0.9378311862123592801 ) ) ;
#7908=FACE_OUTER_BOUND ( 'NONE', #76573, .T. ) ;
#7913=CARTESIAN_POINT ( 'NONE',  ( 32.08968265630385019, 27.03085787977765264, 9.188101187500006262 ) ) ;
#7925=CARTESIAN_POINT ( 'NONE',  ( 73.07852875935716952, 69.76346136681742394, 9.633212380859575319 ) ) ;
#7927=CARTESIAN_POINT ( 'NONE',  ( 35.97235683590213284, 38.95586893147758190, 7.433330006724141015 ) ) ;
#7928=VERTEX_POINT ( 'NONE', #51128 ) ;
#7930=CARTESIAN_POINT ( 'NONE',  ( 89.29477061917849312, 46.06123908072883921, 1.850091733736755357E-15 ) ) ;
#7931=VERTEX_POINT ( 'NONE', #44519 ) ;
#7932=CARTESIAN_POINT ( 'NONE',  ( 86.46734690923850053, 47.05374834302038067, -10.53985889464877523 ) ) ;
#7934=CARTESIAN_POINT ( 'NONE',  ( 84.47262166381923976, 50.18302823219130460, 13.87459367389479326 ) ) ;
#7937=AXIS2_PLACEMENT_3D ( 'NONE', #20205, #12102, #34397 ) ;
#7940=CARTESIAN_POINT ( 'NONE',  ( 45.84141126897937824, 27.26216523072498532, -2.296566073217252530E-15 ) ) ;
#7941=CARTESIAN_POINT ( 'NONE',  ( 81.49556199178041993, 55.44509743070403118, -16.31886845347543158 ) ) ;
#7946=CARTESIAN_POINT ( 'NONE',  ( 87.13833003848017711, 45.89157147215227894, -8.651152695689850347 ) ) ;
#7959=CARTESIAN_POINT ( 'NONE',  ( 45.84141126897937824, 27.26216523072498887, -2.296566073217252530E-15 ) ) ;
#7963=ORIENTED_EDGE ( 'NONE', *, *, #4460, .F. ) ;
#7965=CARTESIAN_POINT ( 'NONE',  ( 76.39071540512284741, 62.51181499478219905, -15.22731582648911797 ) ) ;
#7968=CARTESIAN_POINT ( 'NONE',  ( 72.98212971150626061, 65.41051458920003370, 12.90293089110194380 ) ) ;
#7988=CARTESIAN_POINT ( 'NONE',  ( 71.69128320130467102, 63.41209966293108380, 13.59476739478700225 ) ) ;
#7994=CARTESIAN_POINT ( 'NONE',  ( 83.78033978848483798, 44.16145733190557365, 8.087935607909994218 ) ) ;
#7998=CARTESIAN_POINT ( 'NONE',  ( 84.13204908911603752, 50.42604040346916605, 13.71367173376234838 ) ) ;
#7999=CARTESIAN_POINT ( 'NONE',  ( 71.18060993283003768, 70.65244408663559739, -5.504285530961238848 ) ) ;
#8002=CARTESIAN_POINT ( 'NONE',  ( 69.28126399264922952, 70.99872114787820010, 2.214918965755282798 ) ) ;
#8006=ADVANCED_FACE ( 'NONE', ( #74695 ), #67047, .T. ) ;
#8009=CIRCLE ( 'NONE', #90565, 10.00000000000000711 ) ;
#8010=CARTESIAN_POINT ( 'NONE',  ( 78.66002983668515469, 59.34402786614296588, 16.16707823594543214 ) ) ;
#8011=CARTESIAN_POINT ( 'NONE',  ( 84.87890672887020571, 50.20346095951408927, -13.33159439321596196 ) ) ;
#8013=CARTESIAN_POINT ( 'NONE',  ( 73.46468938206548671, 69.84266834477836028, -9.805732075891272714 ) ) ;
#8014=CARTESIAN_POINT ( 'NONE',  ( 75.93802828010240091, 51.44302491467914251, 15.68598613182542501 ) ) ;
#8019=CARTESIAN_POINT ( 'NONE',  ( 73.12133584826474930, 57.41764960941905116, -15.88333458976553381 ) ) ;
#8024=CARTESIAN_POINT ( 'NONE',  ( 88.40016726344319409, 43.81338102853380434, 0.1423130075416286777 ) ) ;
#8026=CARTESIAN_POINT ( 'NONE',  ( 77.38944774667987758, 49.20504137781674814, 15.31118821561086740 ) ) ;
#8029=CARTESIAN_POINT ( 'NONE',  ( 27.91230638117223606, 28.06628583063842797, -9.188101187500006262 ) ) ;
#8031=CARTESIAN_POINT ( 'NONE',  ( 6.943673075435188302, 24.98502408145590437, -5.678558825948271327 ) ) ;
#8034=CARTESIAN_POINT ( 'NONE',  ( 82.75623256556472995, 53.92166175363784930, -15.45821587292255472 ) ) ;
#8038=B_SPLINE_CURVE_WITH_KNOTS ( 'NONE', 3,
 ( #29667, #22564, #28667, #84400, #90528, #67167, #83911, #60544, #51976, #6377, #14945, #82916, #13490, #14474, #30160, #37748, #44360, #75293, #45835, #5874, #84896, #21576, #76758, #61549 ),
 .UNSPECIFIED., .F., .F.,
 ( 4, 2, 2, 2, 1, 2, 2, 1, 1, 2, 2, 1, 2, 4 ),
 ( 0.000000000000000000, 0.1493091583479830842, 0.2239637375219751536, 0.2612910271089707859, 0.2986183166959664459, 0.3732728958699557120, 0.3919365406634525151, 0.4106001854569493736, 0.4479274750439458108, 0.4852547646309422480, 0.5225820542179386852, 0.5599093438049350668, 0.5785729885984347565, 0.5972366333919344461 ),
 .UNSPECIFIED. ) ;
#8039=CARTESIAN_POINT ( 'NONE',  ( 74.31895847488682705, 57.06360514179990417, -16.02672806696303809 ) ) ;
#8044=CARTESIAN_POINT ( 'NONE',  ( 77.39365065043905645, 49.53244676146400849, 14.91118474622092016 ) ) ;
#8045=CARTESIAN_POINT ( 'NONE',  ( 83.01075186827047503, 53.40825386585734691, 15.63370843945823019 ) ) ;
#8046=EDGE_LOOP ( 'NONE', ( #64127, #40262, #63002, #14828, #49382, #64510 ) ) ;
#8049=CARTESIAN_POINT ( 'NONE',  ( 71.62264301235484254, 72.47875319116253934, -0.1882495702471937982 ) ) ;
#8053=CARTESIAN_POINT ( 'NONE',  ( 65.84203434077124939, 68.97034509070658714, -2.213548117778525004 ) ) ;
#8057=CARTESIAN_POINT ( 'NONE',  ( 30.03287232231581072, 25.84335787977764554, 9.188101187500006262 ) ) ;
#8065=CARTESIAN_POINT ( 'NONE',  ( 67.87906010048776295, 65.45581163343211983, 10.32193553156050925 ) ) ;
#8066=CARTESIAN_POINT ( 'NONE',  ( 67.69188770687451040, 65.70569729239960566, -10.69268924707425406 ) ) ;
#8069=CARTESIAN_POINT ( 'NONE',  ( 41.54549712337441747, 24.39040679176986615, -6.890680421881970419E-14 ) ) ;
#8074=VECTOR ( 'NONE', #65142, 1000.000000000000114 ) ;
#8080=CARTESIAN_POINT ( 'NONE',  ( 79.61837626304058801, 45.86816547348837503, 12.91835716780937737 ) ) ;
#8083=ORIENTED_EDGE ( 'NONE', *, *, #9633, .F. ) ;
#8084=CARTESIAN_POINT ( 'NONE',  ( 66.44361335696784465, 67.86098865684965631, 6.695726806363200723 ) ) ;
#8088=CARTESIAN_POINT ( 'NONE',  ( 70.95953762786423624, 65.45173126332643676, 11.97092896923417094 ) ) ;
#8093=B_SPLINE_SURFACE_WITH_KNOTS ( 'NONE', 3, 1, ( 
 ( #57261, #18787 ),
 ( #42068, #78593 ),
 ( #73001, #9178 ),
 ( #31959, #24378 ),
 ( #19305, #96312 ),
 ( #50172, #13186 ),
 ( #44042, #12179 ),
 ( #81124, #35957 ),
 ( #82624, #35464 ),
 ( #27868, #58261 ),
 ( #83100, #5563 ),
 ( #81609, #43559 ),
 ( #36452, #43040 ),
 ( #74982, #52151 ),
 ( #50657, #11692 ),
 ( #51155, #34471 ),
 ( #44543, #20281 ),
 ( #20784, #59748 ),
 ( #67356, #42551 ),
 ( #73484, #21274 ),
 ( #98284, #13670 ),
 ( #4568, #4068 ),
 ( #73984, #34958 ),
 ( #28872, #90719 ),
 ( #26880, #82119 ),
 ( #28358, #51675 ),
 ( #65858, #58747 ),
 ( #89720, #66369 ),
 ( #97300, #12692 ),
 ( #74498, #5076 ),
 ( #66859, #27375 ) ),
 .UNSPECIFIED., .F., .F., .F.,
 ( 4, 3, 3, 3, 3, 3, 3, 3, 3, 3, 4 ),
 ( 2, 2 ),
 ( 0.000000000000000000, 0.1122669598086897952, 0.2243161639709869148, 0.3396355846219287211, 0.4553962076585368890, 0.5677860799922546109, 0.6749047109689865209, 0.7773884377078494889, 0.8775581155834415448, 0.9782364162377932271, 1.000000000000000000 ),
 ( 0.000000000000000000, 1.000000000000000000 ),
 .UNSPECIFIED. ) ;
#8096=CARTESIAN_POINT ( 'NONE',  ( 76.29399651998687659, 51.64836840559479469, -16.17400485107173225 ) ) ;
#8104=CARTESIAN_POINT ( 'NONE',  ( 82.97179646587753155, 43.66170675654236533, -8.010128394304160793 ) ) ;
#8106=CARTESIAN_POINT ( 'NONE',  ( 30.74868702942336895, 36.49103043416551628, -8.090169943749479842 ) ) ;
#8108=CARTESIAN_POINT ( 'NONE',  ( 72.42968441479126795, 70.75204143367579945, 7.711333220305030878 ) ) ;
#8109=B_SPLINE_CURVE_WITH_KNOTS ( 'NONE', 3,
 ( #7774, #83316, #31060, #38147, #53849, #46770, #84319, #61950, #52867, #90933, #69065, #8278, #39145, #99993, #45752, #98505, #83818, #29095, #59961, #15349, #21483, #52373, #13878, #45269, #44760, #6279, #76202, #23963, #56361, #85844, #70565 ),
 .UNSPECIFIED., .F., .F.,
 ( 4, 3, 3, 3, 3, 3, 3, 3, 3, 3, 4 ),
 ( 0.000000000000000000, 0.1333490885032350692, 0.3007194338854288218, 0.4699862290245104268, 0.5844252810809298371, 0.6686540514502736787, 0.7354980260655487045, 0.8028463152565475935, 0.8633854507757110497, 0.9437142632667278042, 1.000000000000000000 ),
 .UNSPECIFIED. ) ;
#8110=CARTESIAN_POINT ( 'NONE',  ( 72.53392552391629522, 67.03926855329653733, -11.49449286787162983 ) ) ;
#8116=CARTESIAN_POINT ( 'NONE',  ( 83.83362232629562527, 51.98300042451027991, 14.54734556420943292 ) ) ;
#8124=CARTESIAN_POINT ( 'NONE',  ( 74.16423100742596830, 55.12596566212364735, 16.60428178130680266 ) ) ;
#8126=CARTESIAN_POINT ( 'NONE',  ( 23.18815102787819526, 35.16126292948896293, -6.180339887498951690 ) ) ;
#8128=CARTESIAN_POINT ( 'NONE',  ( 67.44257088943837175, 67.25355904234817217, -8.657396272410815996 ) ) ;
#8135=CARTESIAN_POINT ( 'NONE',  ( 72.82118101371948171, 71.12637341421535098, -7.461520388884598454 ) ) ;
#8138=CARTESIAN_POINT ( 'NONE',  ( 23.49395736812309465, 37.65659080271452552, -1.878358725466461243E-16 ) ) ;
#8139=CARTESIAN_POINT ( 'NONE',  ( 84.64602481627416353, 42.28124168067370192, -1.971784886792609326 ) ) ;
#8141=CARTESIAN_POINT ( 'NONE',  ( 72.42633913402016788, 63.30405477351032317, 14.41398973578453102 ) ) ;
#8142=CARTESIAN_POINT ( 'NONE',  ( 84.32653914613003110, 47.10518720127514314, 11.76817659212875178 ) ) ;
#8151=FACE_OUTER_BOUND ( 'NONE', #20425, .T. ) ;
#8158=CARTESIAN_POINT ( 'NONE',  ( 23.79748941506785442, 22.24335787977763346, -9.188101187500008038 ) ) ;
#8160=CARTESIAN_POINT ( 'NONE',  ( 71.40067601551650966, 59.33978977576644098, 15.22537452595757657 ) ) ;
#8165=CARTESIAN_POINT ( 'NONE',  ( 8.350964356584899662, 25.79752408145590792, -5.678558825948271327 ) ) ;
#8166=CARTESIAN_POINT ( 'NONE',  ( 75.50015568109331809, 59.09779916697999624, -15.89073866529240675 ) ) ;
#8167=CARTESIAN_POINT ( 'NONE',  ( 81.57924373063931966, 42.55821344299342002, 7.494866049281546871 ) ) ;
#8169=( BOUNDED_CURVE ( )  B_SPLINE_CURVE ( 2, ( #17916, #95464, #2722, #42187, #81243, #96946, #73123, #79251, #34115, #11817, #26016, #3714, #2218 ),
 .UNSPECIFIED., .F., .T. ) 
 B_SPLINE_CURVE_WITH_KNOTS ( ( 3, 2, 2, 2, 2, 2, 3 ),
 ( 0.7625000000000000666, 0.7650000000000000133, 0.7700000000000000178, 0.7750000000000000222, 0.7800000000000000266, 0.7850000000000000311, 0.7875000000000000888 ),
 .UNSPECIFIED. ) 
 CURVE ( )  GEOMETRIC_REPRESENTATION_ITEM ( )  RATIONAL_B_SPLINE_CURVE ( ( 0.9755282581475767101, 0.9755282581475772652, 1.000000000000000000, 0.9510565162951535312, 1.000000000000000000, 0.9510565162951535312, 1.000000000000000000, 0.9510565162951535312, 1.000000000000000000, 0.9510565162951535312, 1.000000000000000000, 0.9755282581475761550, 0.9755282581475767101 ) ) 
 REPRESENTATION_ITEM ( '' )  );
#8171=CARTESIAN_POINT ( 'NONE',  ( 72.38671951208186783, 71.75852817245944948, -5.691748070601700960 ) ) ;
#8172=CARTESIAN_POINT ( 'NONE',  ( 20.86070775165960001, 33.81751292744056769, -6.180339887498951690 ) ) ;
#8173=CARTESIAN_POINT ( 'NONE',  ( 85.11007338816820322, 42.50720964942713209, 4.151688445370292690 ) ) ;
#8175=ORIENTED_EDGE ( 'NONE', *, *, #14170, .T. ) ;
#8178=CARTESIAN_POINT ( 'NONE',  ( 87.29749550895752463, 43.60436139353286222, -0.5288150457691258577 ) ) ;
#8181=LINE ( 'NONE', #52276, #91771 ) ;
#8182=CARTESIAN_POINT ( 'NONE',  ( 79.84564975497875139, 57.94052304378403306, 16.26602973072665392 ) ) ;
#8183=CARTESIAN_POINT ( 'NONE',  ( 76.67779265155198232, 63.58935824677200088, 15.33226443842420927 ) ) ;
#8191=CARTESIAN_POINT ( 'NONE',  ( 32.45774345291223995, 27.24335787977765833, -9.188101187500008038 ) ) ;
#8202=DIRECTION ( 'NONE',  ( -0.4145187862775162602, 0.7179675985244458047, -0.5591929034707565638 ) ) ;
#8211=CARTESIAN_POINT ( 'NONE',  ( 71.45246435704785881, 70.41140176850349519, 6.448010139539340102 ) ) ;
#8213=CARTESIAN_POINT ( 'NONE',  ( 67.50571429351523989, 67.05925936848247204, 8.976381766308007215 ) ) ;
#8214=CARTESIAN_POINT ( 'NONE',  ( 70.48980766314222990, 65.45931048306678690, -11.73774681883049098 ) ) ;
#8215=CARTESIAN_POINT ( 'NONE',  ( 78.74835927026373383, 47.64973151805292417, 14.29178299612483194 ) ) ;
#8217=ORIENTED_EDGE ( 'NONE', *, *, #57447, .F. ) ;
#8220=CARTESIAN_POINT ( 'NONE',  ( 70.24270501652357268, 65.21164827444138723, 11.83463923091347603 ) ) ;
#8225=CARTESIAN_POINT ( 'NONE',  ( 83.68493280611274088, 51.65299594367198210, -14.83749715326822205 ) ) ;
#8228=CARTESIAN_POINT ( 'NONE',  ( 80.37814466807276403, 57.92114694875621694, -16.24750869670133113 ) ) ;
#8230=CARTESIAN_POINT ( 'NONE',  ( 72.13809228306983812, 71.45234993612235996, 5.060403501811140181 ) ) ;
#8231=CARTESIAN_POINT ( 'NONE',  ( 74.63339219689319748, 67.07035889417386443, 12.49364407091348106 ) ) ;
#8240=CARTESIAN_POINT ( 'NONE',  ( 85.72774873836118559, 48.77901937666835153, -12.00006183775103352 ) ) ;
#8242=CARTESIAN_POINT ( 'NONE',  ( 71.09705276464538315, 63.61861273659285843, 13.28640888171760714 ) ) ;
#8246=B_SPLINE_CURVE_WITH_KNOTS ( 'NONE', 3,
 ( #50888, #90448, #66098, #12413, #28091, #50392, #66596, #4290, #82840, #73708, #97046, #27112, #89933, #27614, #19532, #74225, #35190, #29106, #90943, #21494, #20511, #59465, #58480, #81344, #44280, #13409, #89453, #52384, #4814, #74724, #12920, #35696, #44770, #51386, #5301, #36180, #67082, #98006, #28586, #82353, #20009, #88977, #21017, #81836, #5787, #83326 ),
 .UNSPECIFIED., .F., .F.,
 ( 4, 1, 1, 1, 2, 2, 1, 1, 1, 2, 2, 1, 1, 2, 2, 1, 1, 2, 2, 1, 1, 2, 2, 1, 2, 2, 1, 2, 2, 4 ),
 ( 0.000000000000000000, 0.06250000000000249800, 0.09375000000000141553, 0.1093750000000008743, 0.1171874999999998473, 0.1249999999999988343, 0.1874999999999915345, 0.2187499999999893141, 0.2343749999999881761, 0.2421874999999883982, 0.2499999999999885925, 0.3124999999999791278, 0.3437499999999751310, 0.3593749999999745759, 0.3749999999999739653, 0.4374999999999647504, 0.4687499999999613087, 0.4843749999999601985, 0.4999999999999590328, 0.5624999999999589217, 0.5937499999999593658, 0.6093749999999600320, 0.6249999999999608091, 0.6874999999999679146, 0.7187499999999724665, 0.7499999999999769074, 0.8124999999999835687, 0.8437499999999857891, 0.8749999999999878986, 1.000000000000000000 ),
 .UNSPECIFIED. ) ;
#8249=CARTESIAN_POINT ( 'NONE',  ( 82.09965751949748380, 41.85612385560651205, -5.535113643993918586 ) ) ;
#8257=CARTESIAN_POINT ( 'NONE',  ( 13.61667370911268193, 23.56454794089040661, 10.00000000000000355 ) ) ;
#8259=CARTESIAN_POINT ( 'NONE',  ( 14.97590445773717782, 13.81029122506293305, 8.090169943749479842 ) ) ;
#8260=CARTESIAN_POINT ( 'NONE',  ( 80.17333107395900527, 49.88587112779518407, -14.95505157533469820 ) ) ;
#8261=CARTESIAN_POINT ( 'NONE',  ( 72.02251067321300582, 59.31025418870372334, -15.33526842769922460 ) ) ;
#8267=CARTESIAN_POINT ( 'NONE',  ( 72.79574698827143209, 57.15038201193220857, 15.89495189336207304 ) ) ;
#8268=CARTESIAN_POINT ( 'NONE',  ( 71.90991478695079309, 70.64910724575318568, 7.404170080562185063 ) ) ;
#8269=CARTESIAN_POINT ( 'NONE',  ( 66.33153531111928203, 68.76406954428721008, -4.318981651738461380 ) ) ;
#8274=CARTESIAN_POINT ( 'NONE',  ( 25.90481151690805106, 33.14336893147756768, 7.433330006724141015 ) ) ;
#8278=CARTESIAN_POINT ( 'NONE',  ( 88.38522318935277156, 43.99954571450756902, 2.365518284841161556 ) ) ;
#8279=CARTESIAN_POINT ( 'NONE',  ( 66.06920883062277028, 68.60566076105189381, 1.839620377662104955 ) ) ;
#8284=CARTESIAN_POINT ( 'NONE',  ( 14.05589992062122917, 20.06628583063840310, -9.188101187500006262 ) ) ;
#8288=CARTESIAN_POINT ( 'NONE',  ( 88.30263053946062257, 44.32431199883396289, -2.152525388235255743 ) ) ;
#8289=CARTESIAN_POINT ( 'NONE',  ( 71.53080809438634446, 72.38941617099003167, 1.021674839914435085 ) ) ;
#8303=CARTESIAN_POINT ( 'NONE',  ( 74.14312167556930433, 66.30466486950707861, 1.224646799147354045E-15 ) ) ;
#8309=CARTESIAN_POINT ( 'NONE',  ( 69.37236052325044966, 62.78824976232480282, 13.73178353374107630 ) ) ;
#8316=ORIENTED_EDGE ( 'NONE', *, *, #94051, .F. ) ;
#8319=CARTESIAN_POINT ( 'NONE',  ( 72.82800908514342098, 58.96091748745875805, 15.56478197890324289 ) ) ;
#8324=CARTESIAN_POINT ( 'NONE',  ( 82.68100460170427368, 47.33644815824931840, 12.13400673372383665 ) ) ;
#8327=CARTESIAN_POINT ( 'NONE',  ( 82.73351218272506458, 53.30090480274827769, -15.28980472815078784 ) ) ;
#8329=CARTESIAN_POINT ( 'NONE',  ( 76.31890144197360826, 56.60031049123248437, -16.61185794330136289 ) ) ;
#8330=CARTESIAN_POINT ( 'NONE',  ( 13.34565549823491004, 29.74646525600389424, 2.839279412974139660 ) ) ;
#8339=LINE ( 'NONE', #26051, #52156 ) ;
#8340=CARTESIAN_POINT ( 'NONE',  ( 84.59171082261967456, 45.66142255087724777, -9.512095294586423222 ) ) ;
#8342=CARTESIAN_POINT ( 'NONE',  ( 72.04273812837080015, 59.28583566120335746, 15.84548535902080246 ) ) ;
#8343=EDGE_LOOP ( 'NONE', ( #85101, #79486, #80841, #57397 ) ) ;
#8346=CARTESIAN_POINT ( 'NONE',  ( 75.02238714290076871, 66.92454316053132857, -13.18498694845918706 ) ) ;
#8350=CARTESIAN_POINT ( 'NONE',  ( 82.11234663424232849, 40.76891643967551460, -1.025997306391484232 ) ) ;
#8352=CARTESIAN_POINT ( 'NONE',  ( 7.184267760421183091, 27.08080186712590631, -3.090169943749475845 ) ) ;
#8356=CARTESIAN_POINT ( 'NONE',  ( 75.71688963635942571, 65.45405155058689672, 14.28099675560567583 ) ) ;
#8362=EDGE_CURVE ( 'NONE', #7928, #41027, #47215, .T. ) ;
#8365=CARTESIAN_POINT ( 'NONE',  ( 86.62620551031615435, 45.88478951247049764, -8.398712350495802781 ) ) ;
#8376=FACE_OUTER_BOUND ( 'NONE', #40190, .T. ) ;
#8377=CARTESIAN_POINT ( 'NONE',  ( 80.63908856232002620, 57.54704143882187140, -16.24041183338051297 ) ) ;
#8390=CARTESIAN_POINT ( 'NONE',  ( 82.00425190520714125, 41.38475440514466186, -5.931279945963702005 ) ) ;
#8392=CARTESIAN_POINT ( 'NONE',  ( 13.26084062165525523, 25.84336893147755276, -7.433330006724137462 ) ) ;
#8394=DIRECTION ( 'NONE',  ( -0.3037402332698203589, -0.8935232438716380621, -0.3306933373297692436 ) ) ;
#8396=CARTESIAN_POINT ( 'NONE',  ( 87.14941533941508567, 43.54552546780055877, 0.3078308432578384934 ) ) ;
#8401=CARTESIAN_POINT ( 'NONE',  ( 81.40599722213572420, 56.18777044664494014, -16.43392898140639957 ) ) ;
#8413=CARTESIAN_POINT ( 'NONE',  ( 73.15617415350918407, 69.83382733437846923, 9.602067989434942774 ) ) ;
#8414=CARTESIAN_POINT ( 'NONE',  ( 30.11829213135327521, 40.49540643055189548, 3.479690158560446702E-15 ) ) ;
#8420=ADVANCED_FACE ( 'NONE', ( #49892 ), #80850, .T. ) ;
#8425=CARTESIAN_POINT ( 'NONE',  ( 86.69150557076659425, 44.85198809650525931, -7.441768515828623975 ) ) ;
#8426=CARTESIAN_POINT ( 'NONE',  ( 84.82070890866113189, 50.11195492342548619, -13.71672402108478295 ) ) ;
#8427=CARTESIAN_POINT ( 'NONE',  ( 81.57862098688173091, 55.52127002482139062, -16.32346926850663138 ) ) ;
#8429=ADVANCED_FACE ( 'NONE', ( #20001 ), #69543, .T. ) ;
#8430=B_SPLINE_CURVE_WITH_KNOTS ( 'NONE', 3,
 ( #40546, #80107, #31947, #56756, #40040, #16258, #78074, #79609, #63362, #25357, #71481, #86719, #70981, #17776, #24367, #1582, #24855, #39533, #94302, #62850, #64871, #85727, #71976, #47645, #48160, #55239, #86220, #32465, #16756, #55730, #2076 ),
 .UNSPECIFIED., .F., .F.,
 ( 4, 3, 3, 3, 3, 3, 3, 3, 3, 3, 4 ),
 ( 0.000000000000000000, 0.1333490885032380391, 0.3007194338854225490, 0.4699862290244999907, 0.5844252810809225096, 0.6686540514502540278, 0.7354980260655328284, 0.8028463152565535887, 0.8633854507757017238, 0.9437142632667037123, 1.000000000000000000 ),
 .UNSPECIFIED. ) ;
#8435=CARTESIAN_POINT ( 'NONE',  ( 77.13037345566432634, 49.39794710691812440, -14.91965009447810075 ) ) ;
#8444=CARTESIAN_POINT ( 'NONE',  ( 82.48604300211468399, 40.98759103253163261, 1.037444262390686545 ) ) ;
#8450=CARTESIAN_POINT ( 'NONE',  ( 34.24030602833327208, 37.95586893147758900, 7.433330006724141015 ) ) ;
#8452=ORIENTED_EDGE ( 'NONE', *, *, #49958, .T. ) ;
#8462=( BOUNDED_CURVE ( )  B_SPLINE_CURVE ( 2, ( #34554, #57845, #99733, #92174, #11286, #3676, #65452, #88826, #50250, #19391, #81204, #54146, #6079 ),
 .UNSPECIFIED., .F., .T. ) 
 B_SPLINE_CURVE_WITH_KNOTS ( ( 3, 2, 2, 2, 2, 2, 3 ),
 ( 0.6125000000000000444, 0.6149999999999999911, 0.6199999999999999956, 0.6250000000000000000, 0.6300000000000000044, 0.6350000000000000089, 0.6375000000000000666 ),
 .UNSPECIFIED. ) 
 CURVE ( )  GEOMETRIC_REPRESENTATION_ITEM ( )  RATIONAL_B_SPLINE_CURVE ( ( 0.9755282581475767101, 0.9755282581475772652, 1.000000000000000000, 0.9510565162951535312, 1.000000000000000000, 0.9510565162951535312, 1.000000000000000000, 0.9510565162951535312, 1.000000000000000000, 0.9510565162951535312, 1.000000000000000000, 0.9755282581475761550, 0.9755282581475767101 ) ) 
 REPRESENTATION_ITEM ( '' )  );
#8481=CARTESIAN_POINT ( 'NONE',  ( 72.58119924679503754, 61.32661626603242411, 15.29587950369362659 ) ) ;
#8482=ADVANCED_FACE ( 'NONE', ( #63475 ), #20983, .T. ) ;
#8489=CARTESIAN_POINT ( 'NONE',  ( 71.27925295011586115, 71.54457879798044928, -2.991972160359442245 ) ) ;
#8497=CARTESIAN_POINT ( 'NONE',  ( 78.18654183438681571, 55.67423588053517847, 16.15312830067003347 ) ) ;
#8500=CARTESIAN_POINT ( 'NONE',  ( 73.11394343355392778, 69.60018041412448042, -9.852821959973875110 ) ) ;
#8501=CARTESIAN_POINT ( 'NONE',  ( 76.20222849767326068, 51.12960822232545155, 16.07471935095281523 ) ) ;
#8513=CARTESIAN_POINT ( 'NONE',  ( 87.99782063670886600, 43.98249463337865706, 0.5325925290962013614 ) ) ;
#8516=CARTESIAN_POINT ( 'NONE',  ( 71.82992063434448937, 72.13096581328876766, -3.644439638307356955 ) ) ;
#8517=CARTESIAN_POINT ( 'NONE',  ( 68.44407863485662347, 70.43973750203463169, -2.495858633798906823 ) ) ;
#8519=CARTESIAN_POINT ( 'NONE',  ( 27.19903172117837542, 31.10171378149920329, 9.188101187500008038 ) ) ;
#8521=CARTESIAN_POINT ( 'NONE',  ( 83.07165552766419125, 47.06640118489292490, -11.74642504952208100 ) ) ;
#8522=CARTESIAN_POINT ( 'NONE',  ( 16.50122538818396478, 18.03085787977762422, 9.188101187500006262 ) ) ;
#8524=CARTESIAN_POINT ( 'NONE',  ( 77.00565391796482118, 63.79498567146314514, 14.95288047763914818 ) ) ;
#8529=CARTESIAN_POINT ( 'NONE',  ( 75.58399524922207036, 56.66972461617102397, -16.12440502727555014 ) ) ;
#8534=CARTESIAN_POINT ( 'NONE',  ( 77.07619724897867286, 49.54099758213720861, 15.49150516855853965 ) ) ;
#8542=VERTEX_POINT ( 'NONE', #87846 ) ;
#8549=CARTESIAN_POINT ( 'NONE',  ( 29.15721111571870949, 19.76004757982091320, 5.678558825948272215 ) ) ;
#8550=CARTESIAN_POINT ( 'NONE',  ( 80.05490797256598512, 44.33250473515553836, 11.49671090876265112 ) ) ;
#8551=CARTESIAN_POINT ( 'NONE',  ( 66.33640583476365293, 68.86678167005838702, -0.8053330239553019299 ) ) ;
#8552=CARTESIAN_POINT ( 'NONE',  ( 74.79265276366314197, 66.79451150088600286, -13.18326711696948017 ) ) ;
#8562=CARTESIAN_POINT ( 'NONE',  ( 67.68803865064251113, 65.73242611482004349, -10.66275132821461646 ) ) ;
#8573=ORIENTED_EDGE ( 'NONE', *, *, #24439, .F. ) ;
#8580=CARTESIAN_POINT ( 'NONE',  ( 80.11894959647150927, 44.23929697926691063, -11.37795504581926842 ) ) ;
#8584=CARTESIAN_POINT ( 'NONE',  ( 81.30363341997924920, 48.13948513678796814, -13.22891315866029238 ) ) ;
#8588=ORIENTED_EDGE ( 'NONE', *, *, #78491, .T. ) ;
#8591=ORIENTED_EDGE ( 'NONE', *, *, #97588, .F. ) ;
#8592=CARTESIAN_POINT ( 'NONE',  ( 24.26937655755794054, 14.41603393254325205, -1.583844403245362020 ) ) ;
#8593=CARTESIAN_POINT ( 'NONE',  ( 76.28082308479837081, 64.96498169073787210, -14.28860055222916081 ) ) ;
#8596=CARTESIAN_POINT ( 'NONE',  ( 87.60949802315384716, 44.65508912978396694, 4.993525404917304122 ) ) ;
#8614=EDGE_CURVE ( 'NONE', #54612, #60500, #78106, .T. ) ;
#8617=FACE_BOUND ( 'NONE', #44010, .T. ) ;
#8618=CARTESIAN_POINT ( 'NONE',  ( 79.27623980079764010, 52.27818998861121003, 15.92750218127481077 ) ) ;
#8619=VECTOR ( 'NONE', #17121, 1000.000000000000114 ) ;
#8620=CARTESIAN_POINT ( 'NONE',  ( 31.49087468139936874, 26.38052372038642091, 10.00000000000000533 ) ) ;
#8626=VECTOR ( 'NONE', #43275, 1000.000000000000114 ) ;
#8634=CARTESIAN_POINT ( 'NONE',  ( 29.20513097723256024, 32.56454794089043503, 10.00000000000000355 ) ) ;
#8635=CARTESIAN_POINT ( 'NONE',  ( 83.88249041513446969, 42.01244510319034475, -2.872826126902047417 ) ) ;
#8638=B_SPLINE_SURFACE_WITH_KNOTS ( 'NONE', 3, 1, ( 
 ( #5505, #73421 ),
 ( #36894, #74435 ),
 ( #97724, #52095 ),
 ( #36390, #5016 ),
 ( #42977, #28804 ),
 ( #67295, #73916 ),
 ( #59689, #35897 ),
 ( #13613, #44486 ),
 ( #92633, #30300 ),
 ( #60671, #31286 ),
 ( #61683, #54074 ),
 ( #8013, #84049 ),
 ( #85552, #38885 ),
 ( #69788, #37385 ),
 ( #61185, #77408 ),
 ( #62173, #45484 ),
 ( #46997, #99711 ),
 ( #62678, #77911 ),
 ( #23676, #23182 ),
 ( #68787, #398 ),
 ( #22199, #83542 ),
 ( #14106, #44987 ),
 ( #15082, #7487 ),
 ( #85029, #29799 ),
 ( #100218, #93125 ),
 ( #99213, #53093 ),
 ( #54568, #16093 ),
 ( #8500, #30803 ),
 ( #15576, #91632 ),
 ( #75930, #37876 ),
 ( #39370, #45971 ) ),
 .UNSPECIFIED., .F., .F., .F.,
 ( 4, 3, 3, 3, 3, 3, 3, 3, 3, 3, 4 ),
 ( 2, 2 ),
 ( 0.000000000000000000, 0.1333490885032358464, 0.3007194338854307092, 0.4699862290245053198, 0.5844252810809311693, 0.6686540514502750110, 0.7354980260655511470, 0.8028463152565725736, 0.8633854507757335872, 0.9437142632667383513, 1.000000000000000000 ),
 ( 0.000000000000000000, 1.000000000000000000 ),
 .UNSPECIFIED. ) ;
#8640=DIRECTION ( 'NONE',  ( -0.06958655048002569676, 0.1205274409548614395, -0.9902680687415721383 ) ) ;
#8645=CARTESIAN_POINT ( 'NONE',  ( 66.71817688721121442, 67.86101298462291709, 6.998882950237777401 ) ) ;
#8649=CARTESIAN_POINT ( 'NONE',  ( 80.44215978124604760, 58.39441083166272506, 0.000000000000000000 ) ) ;
#8653=CARTESIAN_POINT ( 'NONE',  ( 17.01121839442928163, 30.79752408145592568, -5.678558825948271327 ) ) ;
#8658=CARTESIAN_POINT ( 'NONE',  ( 6.527493107231251201, 21.95586893147753216, 7.433330006724141015 ) ) ;
#8660=CARTESIAN_POINT ( 'NONE',  ( 88.02262071555790612, 44.26851354062424804, 2.809628182802242691 ) ) ;
#8661=CARTESIAN_POINT ( 'NONE',  ( 45.82169850708434922, 28.58380873178791504, 6.180339887498953466 ) ) ;
#8664=CARTESIAN_POINT ( 'NONE',  ( 72.54340540113201996, 71.27809821757736586, -6.032689287156388858 ) ) ;
#8669=EDGE_CURVE ( 'NONE', #89530, #41986, #63554, .T. ) ;
#8673=CARTESIAN_POINT ( 'NONE',  ( 86.97441523645338179, 43.45437750576425628, -1.010700286482205446 ) ) ;
#8676=CARTESIAN_POINT ( 'NONE',  ( 71.92536400468701174, 72.18844424196340981, -3.635291937859653544 ) ) ;
#8677=CARTESIAN_POINT ( 'NONE',  ( 80.02542612678608691, 57.59583086733049129, 16.60012225046076040 ) ) ;
#8686=ORIENTED_EDGE ( 'NONE', *, *, #67834, .F. ) ;
#8687=CARTESIAN_POINT ( 'NONE',  ( 31.98500480842837490, 19.26216523072496400, -2.296566073217252530E-15 ) ) ;
#8692=CARTESIAN_POINT ( 'NONE',  ( 73.91288345017510153, 68.57868192222672121, 10.89134523673511623 ) ) ;
#8696=EDGE_LOOP ( 'NONE', ( #20584, #1358, #74403, #37075 ) ) ;
#8698=CARTESIAN_POINT ( 'NONE',  ( 86.55745248666850955, 46.28591021298573338, 9.008290149372946587 ) ) ;
#8709=CARTESIAN_POINT ( 'NONE',  ( 69.44407254868087875, 66.48165845397403473, 10.23672187717776083 ) ) ;
#8711=CARTESIAN_POINT ( 'NONE',  ( 67.46085622035505480, 67.01197793175170148, 9.005109031795694108 ) ) ;
#8712=CARTESIAN_POINT ( 'NONE',  ( 74.28630307215421169, 64.63373713051603886, -13.80664065817792263 ) ) ;
#8713=CARTESIAN_POINT ( 'NONE',  ( 77.98042497925951011, 47.87864476968928074, 14.07985687966458599 ) ) ;
#8717=CARTESIAN_POINT ( 'NONE',  ( 70.53859886870293394, 66.00395551958487772, 11.32651892520792458 ) ) ;
#8721=CARTESIAN_POINT ( 'NONE',  ( 83.88998279704740924, 51.95482724045139378, -14.52911814644455646 ) ) ;
#8724=CARTESIAN_POINT ( 'NONE',  ( 65.92723761088207368, 68.94945291059252668, -2.624861928015914003 ) ) ;
#8734=CARTESIAN_POINT ( 'NONE',  ( 85.50592849318395849, 48.29857843294553277, -11.72635531101612294 ) ) ;
#8736=CARTESIAN_POINT ( 'NONE',  ( 71.11978001288902362, 63.69250981634468189, 13.25087439340794226 ) ) ;
#8737=CARTESIAN_POINT ( 'NONE',  ( 84.14312167556933275, 48.98415679381830756, 0.000000000000000000 ) ) ;
#8740=CARTESIAN_POINT ( 'NONE',  ( 82.19821301579139572, 41.48612719278543182, -5.907191800152080674 ) ) ;
#8746=ORIENTED_EDGE ( 'NONE', *, *, #4780, .F. ) ;
#8747=ADVANCED_FACE ( 'NONE', ( #73789 ), #67892, .T. ) ;
#8749=CARTESIAN_POINT ( 'NONE',  ( 87.81665660121321082, 44.77054464327975580, 4.981472615147592542 ) ) ;
#8751=CARTESIAN_POINT ( 'NONE',  ( 10.15257209397493199, 21.56454794089039240, 10.00000000000000355 ) ) ;
#8754=CARTESIAN_POINT ( 'NONE',  ( 71.78531393134818472, 71.87200472712461874, 2.928372626719420335 ) ) ;
#8760=CARTESIAN_POINT ( 'NONE',  ( 66.77376812102318127, 68.41195941748605946, -4.433129028897188739 ) ) ;
#8761=( BOUNDED_CURVE ( )  B_SPLINE_CURVE ( 2, ( #10864, #57942, #26061, #27566, #25556, #96490, #72683, #56938, #96001, #18974, #33149, #49848, #4238 ),
 .UNSPECIFIED., .F., .T. ) 
 B_SPLINE_CURVE_WITH_KNOTS ( ( 3, 2, 2, 2, 2, 2, 3 ),
 ( 0.3125000000000000000, 0.3150000000000000022, 0.3200000000000000067, 0.3250000000000000111, 0.3300000000000000155, 0.3350000000000000200, 0.3375000000000000222 ),
 .UNSPECIFIED. ) 
 CURVE ( )  GEOMETRIC_REPRESENTATION_ITEM ( )  RATIONAL_B_SPLINE_CURVE ( ( 0.9755282581475768211, 0.9755282581475768211, 1.000000000000000000, 0.9510565162951535312, 1.000000000000000000, 0.9510565162951535312, 1.000000000000000000, 0.9510565162951535312, 1.000000000000000000, 0.9510565162951535312, 1.000000000000000000, 0.9755282581475768211, 0.9755282581475768211 ) ) 
 REPRESENTATION_ITEM ( '' )  );
#8769=CARTESIAN_POINT ( 'NONE',  ( 24.06271987006732616, 35.93396525600390845, 2.839279412974139660 ) ) ;
#8775=CARTESIAN_POINT ( 'NONE',  ( 66.28418275192433384, 69.17501406156587507, 2.517326374184488014 ) ) ;
#8779=DIRECTION ( 'NONE',  ( 0.3715724127386967335, -0.6435822975543782354, -0.6691306063588567943 ) ) ;
#8780=CARTESIAN_POINT ( 'NONE',  ( 9.725772901699041739, 17.56628583063838889, 9.188101187500006262 ) ) ;
#8782=CARTESIAN_POINT ( 'NONE',  ( 88.29579885706220921, 44.29800590334696153, -2.024579815269742067 ) ) ;
#8783=EDGE_CURVE ( 'NONE', #59656, #18632, #93742, .T. ) ;
#8793=CARTESIAN_POINT ( 'NONE',  ( 81.87359138893998534, 41.32955797152819599, 5.976920566253460798 ) ) ;
#8801=CARTESIAN_POINT ( 'NONE',  ( 8.118423711322263259, 28.18528772668516424, -1.583844403245363575 ) ) ;
#8802=CARTESIAN_POINT ( 'NONE',  ( 80.49736582374534066, 43.65955092740581733, 9.838849738494864994 ) ) ;
#8807=EDGE_LOOP ( 'NONE', ( #17709, #98056, #20655, #15252 ) ) ;
#8810=CARTESIAN_POINT ( 'NONE',  ( 73.87636433878275000, 63.53668594947264836, 14.23734624109727420 ) ) ;
#8815=CARTESIAN_POINT ( 'NONE',  ( 83.61782708266594000, 50.72174090158058846, 13.98667043904370644 ) ) ;
#8819=CARTESIAN_POINT ( 'NONE',  ( 82.56707315150609361, 53.27404436626156325, -15.30997931004315404 ) ) ;
#8822=CARTESIAN_POINT ( 'NONE',  ( 18.74326920199815305, 31.79752408145591858, -5.678558825948271327 ) ) ;
#8831=CARTESIAN_POINT ( 'NONE',  ( 83.28211300506427506, 45.81084018523562662, -10.47891480825111366 ) ) ;
#8832=AXIS2_PLACEMENT_3D ( 'NONE', #92468, #23015, #75259 ) ;
#8835=EDGE_LOOP ( 'NONE', ( #24603, #86146, #88509, #71785 ) ) ;
#8841=VECTOR ( 'NONE', #89682, 1000.000000000000114 ) ;
#8842=CARTESIAN_POINT ( 'NONE',  ( 82.37532108405909526, 40.36264586417863143, -0.9042686866734450657 ) ) ;
#8846=CARTESIAN_POINT ( 'NONE',  ( 75.72624665019681345, 65.60512238633357640, 13.80728453669184930 ) ) ;
#8847=EDGE_CURVE ( 'NONE', #4682, #46017, #62273, .T. ) ;
#8851=ORIENTED_EDGE ( 'NONE', *, *, #4696, .T. ) ;
#8856=CARTESIAN_POINT ( 'NONE',  ( 22.65899766026757689, 36.58029201028042365, 1.583844403245397769 ) ) ;
#8858=CARTESIAN_POINT ( 'NONE',  ( 82.24352131881794037, 42.57645519026166170, 6.897321416369183389 ) ) ;
#8859=CARTESIAN_POINT ( 'NONE',  ( 74.00349760290353629, 68.31608301643910863, -11.67389511724663009 ) ) ;
#8868=CARTESIAN_POINT ( 'NONE',  ( 80.30021992591166224, 57.12375492286918899, -16.23351995593440478 ) ) ;
#8876=CARTESIAN_POINT ( 'NONE',  ( 68.21143465159309471, 67.67609039233754231, 7.757874407560066743 ) ) ;
#8880=VERTEX_POINT ( 'NONE', #9885 ) ;
#8881=CARTESIAN_POINT ( 'NONE',  ( 73.88265267960163385, 56.39564808591543965, 16.54767161977011725 ) ) ;
#8884=CARTESIAN_POINT ( 'NONE',  ( 16.34664070491415444, 11.29860640527290983, -2.839279412974138328 ) ) ;
#8893=CARTESIAN_POINT ( 'NONE',  ( 43.87294039959300562, 25.73415679381825427, 1.333680081654574804E-15 ) ) ;
#8894=CARTESIAN_POINT ( 'NONE',  ( 86.08503991123366461, 47.67438411149250754, 10.86771628747278129 ) ) ;
#8901=CARTESIAN_POINT ( 'NONE',  ( 75.67384099942408682, 65.13299740138256766, -14.43017819244620803 ) ) ;
#8909=CARTESIAN_POINT ( 'NONE',  ( 38.77491099913230954, 28.10170272979929962, -7.433330006724141015 ) ) ;
#8910=ORIENTED_EDGE ( 'NONE', *, *, #50873, .T. ) ;
#8911=CARTESIAN_POINT ( 'NONE',  ( 66.45672647442243886, 68.66481161880344075, 4.836932588431464453 ) ) ;
#8916=CARTESIAN_POINT ( 'NONE',  ( 79.42866338260434134, 59.50128377535573776, 16.18467811310512516 ) ) ;
#8920=CARTESIAN_POINT ( 'NONE',  ( 17.46284523756094131, 33.58029201028041655, 1.583844403245363353 ) ) ;
#8923=CARTESIAN_POINT ( 'NONE',  ( 84.83229447964083647, 50.15339875539878989, -13.73726727158769023 ) ) ;
#8925=EDGE_CURVE ( 'NONE', #77173, #50839, #9198, .T. ) ;
#8930=ORIENTED_EDGE ( 'NONE', *, *, #75737, .T. ) ;
#8931=CARTESIAN_POINT ( 'NONE',  ( 81.17822002178407104, 55.59913327053874355, 16.37131925982175318 ) ) ;
#8933=CARTESIAN_POINT ( 'NONE',  ( 86.85107213257295200, 45.77346519082802700, -8.718545132792499430 ) ) ;
#8934=CARTESIAN_POINT ( 'NONE',  ( 79.18986863112007768, 53.11630500884587036, 15.70188359001152634 ) ) ;
#8940=CARTESIAN_POINT ( 'NONE',  ( 82.57820959284865125, 40.47900230139654099, 0.8910982540740166602 ) ) ;
#8946=CARTESIAN_POINT ( 'NONE',  ( 42.04415689841856363, 29.98920272979930246, 7.433330006724137462 ) ) ;
#8949=CARTESIAN_POINT ( 'NONE',  ( 30.23324123896446736, 19.58380873178788306, 6.180339887498953466 ) ) ;
#8955=CARTESIAN_POINT ( 'NONE',  ( 73.76584831522595209, 68.38082682530665579, 10.99424229391075514 ) ) ;
#8958=CARTESIAN_POINT ( 'NONE',  ( 26.99866280452971878, 37.36126292948897287, 6.180339887498949913 ) ) ;
#8967=FACE_OUTER_BOUND ( 'NONE', #14023, .T. ) ;
#8968=CARTESIAN_POINT ( 'NONE',  ( 69.13511649644314616, 71.04256955909853843, 2.869324681485878275E-06 ) ) ;
#8972=VERTEX_POINT ( 'NONE', #18478 ) ;
#8979=CARTESIAN_POINT ( 'NONE',  ( 85.22936087665587479, 47.20283195921787467, 10.81987217476543073 ) ) ;
#8980=CARTESIAN_POINT ( 'NONE',  ( 13.95435611255089725, 31.55466486950698268, -1.111400068045478839E-16 ) ) ;
#8982=CARTESIAN_POINT ( 'NONE',  ( 69.12254913399198131, 70.55341387760749683, 0.02902045130465960923 ) ) ;
#8985=CARTESIAN_POINT ( 'NONE',  ( 67.69237348538018750, 66.82088825431439716, 8.559571887000263501 ) ) ;
#8992=CARTESIAN_POINT ( 'NONE',  ( 78.06933962600676580, 61.94553563989994416, 15.69501238203493187 ) ) ;
#8994=CARTESIAN_POINT ( 'NONE',  ( 75.96907744678482288, 51.45858532960258458, 16.17359642618427173 ) ) ;
#9007=CARTESIAN_POINT ( 'NONE',  ( 88.54812304393657030, 43.90120638611161752, -0.3063217976418581845 ) ) ;
#9009=CARTESIAN_POINT ( 'NONE',  ( 71.78553924664423391, 72.10835861452468976, -3.632824164035485470 ) ) ;
#9010=CARTESIAN_POINT ( 'NONE',  ( 77.69386982215107196, 49.37577063231137942, 15.30935726915745931 ) ) ;
#9013=CARTESIAN_POINT ( 'NONE',  ( 30.02984208470827454, 19.19860640527293327, 2.839279412974134775 ) ) ;
#9016=CARTESIAN_POINT ( 'NONE',  ( 13.89351337401799391, 10.94754757982087945, 5.678558825948272215 ) ) ;
#9018=DIRECTION ( 'NONE',  ( 0.5000000000000014433, -0.8660254037844378194, 0.000000000000000000 ) ) ;
#9021=CARTESIAN_POINT ( 'NONE',  ( 69.64550182367553077, 63.14169069997384298, -13.61487806674371370 ) ) ;
#9024=CARTESIAN_POINT ( 'NONE',  ( 77.99503874021337424, 55.85935939106580150, -16.14935493097549113 ) ) ;
#9025=CARTESIAN_POINT ( 'NONE',  ( 87.62574851936349773, 45.15471363961356133, -6.154635046463404535 ) ) ;
#9028=EDGE_CURVE ( 'NONE', #15032, #19489, #51346, .T. ) ;
#9031=CARTESIAN_POINT ( 'NONE',  ( 77.25232559036803082, 49.49244633483773725, 14.92639236986914142 ) ) ;
#9033=ORIENTED_EDGE ( 'NONE', *, *, #18204, .T. ) ;
#9036=CARTESIAN_POINT ( 'NONE',  ( 72.23451590016303214, 68.82702540631112242, -9.493575677105072330 ) ) ;
#9040=ORIENTED_EDGE ( 'NONE', *, *, #14539, .F. ) ;
#9041=CARTESIAN_POINT ( 'NONE',  ( 79.40193053424152936, 46.39394473022984755, -12.75601862751888760 ) ) ;
#9046=CARTESIAN_POINT ( 'NONE',  ( 26.65055534615017763, 21.10170272979927830, -7.433330006724141015 ) ) ;
#9049=CARTESIAN_POINT ( 'NONE',  ( 75.28959155135937920, 66.52156427834158592, -13.12148920440117195 ) ) ;
#9050=CARTESIAN_POINT ( 'NONE',  ( 81.92605646210873260, 48.64405669687059941, -13.31366699692007316 ) ) ;
#9051=EDGE_CURVE ( 'NONE', #69981, #63769, #99813, .T. ) ;
#9060=CARTESIAN_POINT ( 'NONE',  ( 68.19908846357228072, 65.66916044190364232, -10.28971576526838483 ) ) ;
#9067=CARTESIAN_POINT ( 'NONE',  ( 79.12311323331778112, 59.82187722400571062, 16.49858871944914185 ) ) ;
#9073=CARTESIAN_POINT ( 'NONE',  ( 78.04817985968655591, 62.07294584189650521, -16.01854286150912898 ) ) ;
#9076=VERTEX_POINT ( 'NONE', #87692 ) ;
#9080=CARTESIAN_POINT ( 'NONE',  ( 67.79725476218452229, 65.71048819351143777, 10.00598338191753101 ) ) ;
#9081=CARTESIAN_POINT ( 'NONE',  ( 82.42161199636267099, 47.86338641862497667, -12.65011761261475520 ) ) ;
#9084=ORIENTED_EDGE ( 'NONE', *, *, #46651, .T. ) ;
#9085=ORIENTED_EDGE ( 'NONE', *, *, #51623, .F. ) ;
#9089=CARTESIAN_POINT ( 'NONE',  ( 75.89533479853247400, 64.71926289652466835, -14.30003966153671691 ) ) ;
#9093=CARTESIAN_POINT ( 'NONE',  ( 87.81385227123767834, 44.76907565500617636, 4.981894665149344981 ) ) ;
#9095=CARTESIAN_POINT ( 'NONE',  ( 81.80357686921180971, 43.66383732902560411, -8.936250712220841663 ) ) ;
#9102=DIRECTION ( 'NONE',  ( 0.9133924323370933296, -0.1624253398589802222, 0.3732723851573050422 ) ) ;
#9106=CARTESIAN_POINT ( 'NONE',  ( 83.66159036850885400, 42.08077760457628358, 3.673192525297190869 ) ) ;
#9110=ORIENTED_EDGE ( 'NONE', *, *, #2786, .F. ) ;
#9115=CARTESIAN_POINT ( 'NONE',  ( 73.60037652456395563, 55.60548681284689820, 16.10385087386687886 ) ) ;
#9116=CARTESIAN_POINT ( 'NONE',  ( 80.01979875032591849, 57.54866692369599690, 16.59896302490740538 ) ) ;
#9117=EDGE_CURVE ( 'NONE', #17646, #82741, #95005, .T. ) ;
#9118=CARTESIAN_POINT ( 'NONE',  ( 28.06847263831340555, 31.90829794293882316, 10.00000000000000355 ) ) ;
#9124=EDGE_CURVE ( 'NONE', #24743, #49291, #42008, .T. ) ;
#9128=DIRECTION ( 'NONE',  ( -0.6270036013472584102, -0.3336146661356741983, 0.7039657224870761176 ) ) ;
#9129=ORIENTED_EDGE ( 'NONE', *, *, #97429, .F. ) ;
#9132=CARTESIAN_POINT ( 'NONE',  ( 81.60968120880437482, 41.61943387927043148, 5.647669398712323208 ) ) ;
#9135=CARTESIAN_POINT ( 'NONE',  ( 37.75007554933399234, 22.76426979415092333, 3.090169943749476733 ) ) ;
#9136=CARTESIAN_POINT ( 'NONE',  ( 82.01156895356272969, 41.52670969893105735, -4.853141658140002868 ) ) ;
#9138=CARTESIAN_POINT ( 'NONE',  ( 80.96506752577832344, 55.91141337780396015, 16.08528190432092231 ) ) ;
#9143=CARTESIAN_POINT ( 'NONE',  ( 71.00261025973313167, 66.65379046055741696, -10.97453163846388513 ) ) ;
#9156=CARTESIAN_POINT ( 'NONE',  ( 28.52090319329063206, 17.26216523072495690, -2.296566073217252530E-15 ) ) ;
#9161=CARTESIAN_POINT ( 'NONE',  ( 42.07167428219069905, 29.45404122711137163, -8.090169943749478065 ) ) ;
#9163=CARTESIAN_POINT ( 'NONE',  ( 9.471979480098337234, 23.65586893147754566, -7.433330006724137462 ) ) ;
#9165=CARTESIAN_POINT ( 'NONE',  ( 73.29163036545841692, 59.81749283019145480, -15.42714291014837613 ) ) ;
#9166=CARTESIAN_POINT ( 'NONE',  ( 87.83435352734132096, 44.15087646923105780, 2.758404312169200345 ) ) ;
#9169=CARTESIAN_POINT ( 'NONE',  ( 72.48661302258760486, 71.52526770760661634, -5.337229783571229014 ) ) ;
#9172=B_SPLINE_CURVE_WITH_KNOTS ( 'NONE', 3,
 ( #55142, #78479, #86621, #79509, #32854, #40446, #94695, #17155, #48053, #71381, #25257, #56140, #87138, #10071, #71880, #27764 ),
 .UNSPECIFIED., .F., .F.,
 ( 4, 1, 2, 2, 2, 1, 2, 2, 4 ),
 ( 0.000000000000000000, 0.1249999999999995282, 0.1875000000000013878, 0.2500000000000032752, 0.5000000000000046629, 0.6250000000000072164, 0.6875000000000065503, 0.7500000000000057732, 1.000000000000000000 ),
 .UNSPECIFIED. ) ;
#9174=ORIENTED_EDGE ( 'NONE', *, *, #76170, .T. ) ;
#9176=CARTESIAN_POINT ( 'NONE',  ( 82.02953226466719627, 42.27987555721853141, -6.567708260245657570 ) ) ;
#9178=CARTESIAN_POINT ( 'NONE',  ( 66.12615603930825614, 68.50702530225942155, -2.650021266571979783 ) ) ;
#9179=CARTESIAN_POINT ( 'NONE',  ( 71.96596176604222705, 72.21842720279319394, -3.609932465874673646 ) ) ;
#9180=CARTESIAN_POINT ( 'NONE',  ( 80.02165461388095480, 57.57226732806287828, 16.59957571444259727 ) ) ;
#9183=EDGE_CURVE ( 'NONE', #3380, #8880, #89181, .T. ) ;
#9186=CIRCLE ( 'NONE', #73915, 9.000000000000007105 ) ;
#9189=CARTESIAN_POINT ( 'NONE',  ( 27.40352323984253502, 36.79752408145593279, -5.678558825948271327 ) ) ;
#9191=CARTESIAN_POINT ( 'NONE',  ( 78.60735446189906384, 47.91558663933584228, -14.46554740014634888 ) ) ;
#9193=CARTESIAN_POINT ( 'NONE',  ( 74.13497556468038852, 68.62018799133311120, 10.97049235834077408 ) ) ;
#9194=CARTESIAN_POINT ( 'NONE',  ( 35.21268636174862365, 20.73415679381824006, 1.333680081654574804E-15 ) ) ;
#9198=B_SPLINE_CURVE_WITH_KNOTS ( 'NONE', 3,
 ( #3290, #19971, #72183, #26573, #81798, #2794, #95009, #64572, #25569, #56458 ),
 .UNSPECIFIED., .F., .F.,
 ( 4, 2, 2, 2, 4 ),
 ( 0.000000000000000000, 0.2500000000000000000, 0.5000000000000000000, 0.7500000000000000000, 1.000000000000000000 ),
 .UNSPECIFIED. ) ;
#9201=CARTESIAN_POINT ( 'NONE',  ( 86.12405100256837898, 43.33680938231972135, -3.166424999297555942 ) ) ;
#9203=CARTESIAN_POINT ( 'NONE',  ( 77.31487416622417186, 50.45086608835270425, 15.74699347680645012 ) ) ;
#9204=VERTEX_POINT ( 'NONE', #59170 ) ;
#9212=CARTESIAN_POINT ( 'NONE',  ( 67.21548817476096360, 66.87675868597760598, 8.996481726798670309 ) ) ;
#9214=DIRECTION ( 'NONE',  ( -0.03487823687206607903, 0.06041087834084090530, 0.9975640502598237536 ) ) ;
#9219=CARTESIAN_POINT ( 'NONE',  ( 84.42663183290281381, 49.91580812419739033, -13.73522929182741947 ) ) ;
#9234=VECTOR ( 'NONE', #14483, 1000.000000000000000 ) ;
#9236=CARTESIAN_POINT ( 'NONE',  ( 85.35583701238070375, 48.33319239702164083, -12.28927654967825411 ) ) ;
#9239=B_SPLINE_SURFACE_WITH_KNOTS ( 'NONE', 3, 1, ( 
 ( #61775, #38973 ),
 ( #61277, #76501 ),
 ( #86153, #68383 ),
 ( #7081, #23272 ),
 ( #78001, #62263 ),
 ( #15674, #92242 ),
 ( #68873, #85643 ),
 ( #60761, #46568 ),
 ( #39457, #7582 ),
 ( #29888, #99802 ),
 ( #69877, #22791 ),
 ( #30387, #8593 ),
 ( #53671, #23776 ),
 ( #31378, #93217 ),
 ( #54665, #16189 ),
 ( #3018, #32386 ),
 ( #18694, #79019 ),
 ( #57666, #63282 ),
 ( #70897, #94226 ),
 ( #80025, #63782 ),
 ( #56680, #41978 ),
 ( #1992, #10594 ),
 ( #16686, #78505 ),
 ( #1503, #18197 ),
 ( #11108, #72915 ),
 ( #86646, #71403 ),
 ( #34383, #95740 ),
 ( #26293, #41467 ),
 ( #71903, #40471 ),
 ( #24777, #9089 ),
 ( #17694, #87663 ) ),
 .UNSPECIFIED., .F., .F., .F.,
 ( 4, 3, 3, 3, 3, 3, 3, 3, 3, 3, 4 ),
 ( 2, 2 ),
 ( 0.000000000000000000, 0.1333490885032302675, 0.3007194338854343174, 0.4699862290245060414, 0.5844252810809307253, 0.6686540514502736787, 0.7354980260655518132, 0.8028463152565562533, 0.8633854507757269259, 0.9437142632667357978, 1.000000000000000000 ),
 ( 0.000000000000000000, 1.000000000000000000 ),
 .UNSPECIFIED. ) ;
#9241=CARTESIAN_POINT ( 'NONE',  ( 68.59152374985116296, 70.15750495373214335, -1.449766717895635937 ) ) ;
#9251=EDGE_CURVE ( 'NONE', #121, #22248, #3173, .T. ) ;
#9256=CARTESIAN_POINT ( 'NONE',  ( 15.32787473065566530, 20.80066082961420904, 10.00000000000000533 ) ) ;
#9258=CARTESIAN_POINT ( 'NONE',  ( 16.37683477841346402, 11.58380873178785642, 6.180339887498953466 ) ) ;
#9260=CARTESIAN_POINT ( 'NONE',  ( 84.53604152985417386, 48.58536132937872765, -12.83955353848883441 ) ) ;
#9274=CARTESIAN_POINT ( 'NONE',  ( 38.58005528328081368, 27.98920272979929535, 7.433330006724137462 ) ) ;
#9280=CARTESIAN_POINT ( 'NONE',  ( 66.02078622378404305, 69.01578666960394060, 2.557315166718900468 ) ) ;
#9282=DIRECTION ( 'NONE',  ( -0.6355427771210596655, 0.000000000000000000, -0.7720656568254095076 ) ) ;
#9285=CARTESIAN_POINT ( 'NONE',  ( 11.30507296547734342, 15.03085787977761179, 9.188101187500006262 ) ) ;
#9287=B_SPLINE_CURVE_WITH_KNOTS ( 'NONE', 3,
 ( #41393, #71831, #72336, #2429, #3909, #10020, #65693, #49501, #18624, #40882, #80456, #26711, #88075, #81445, #33305, #96647 ),
 .UNSPECIFIED., .F., .F.,
 ( 4, 1, 2, 2, 2, 1, 2, 2, 4 ),
 ( 0.000000000000000000, 0.1250000000000000555, 0.1875000000000001388, 0.2500000000000002220, 0.5000000000000042188, 0.6250000000000081046, 0.6875000000000081046, 0.7500000000000081046, 1.000000000000000000 ),
 .UNSPECIFIED. ) ;
#9292=CARTESIAN_POINT ( 'NONE',  ( 87.66431508103863735, 45.37878918399155737, 6.534061628821841161 ) ) ;
#9303=CARTESIAN_POINT ( 'NONE',  ( 79.16072033191954915, 59.43364827697806163, -16.53552069436851824 ) ) ;
#9306=CARTESIAN_POINT ( 'NONE',  ( 14.02357142238433063, 26.83478043621387243, -8.090169943749479842 ) ) ;
#9312=CARTESIAN_POINT ( 'NONE',  ( 40.40883878445526278, 23.73415679381825782, -6.890680421881970419E-14 ) ) ;
#9317=CARTESIAN_POINT ( 'NONE',  ( 74.40110702076535176, 66.01700144621987931, 13.09005787277605926 ) ) ;
#9318=ORIENTED_EDGE ( 'NONE', *, *, #64617, .T. ) ;
#9322=CARTESIAN_POINT ( 'NONE',  ( 83.16451022896389134, 48.86124166517332412, 13.03494861915621250 ) ) ;
#9323=CARTESIAN_POINT ( 'NONE',  ( 71.90675068868807784, 70.27826969819891190, 7.152555901417152917 ) ) ;
#9330=CARTESIAN_POINT ( 'NONE',  ( 24.39888929631063519, 19.80170272979926693, 7.433330006724137462 ) ) ;
#9334=VERTEX_POINT ( 'NONE', #14608 ) ;
#9342=EDGE_LOOP ( 'NONE', ( #8851, #24414, #58746, #12168 ) ) ;
#9344=AXIS2_PLACEMENT_3D ( 'NONE', #41394, #34791, #87590 ) ;
#9349=CARTESIAN_POINT ( 'NONE',  ( 82.34602464792934029, 40.35042920187159154, -0.9760158778588673423 ) ) ;
#9353=CARTESIAN_POINT ( 'NONE',  ( 75.81472511161923933, 65.61200627121189655, 13.82990332215134899 ) ) ;
#9360=CARTESIAN_POINT ( 'NONE',  ( 68.66214101563461725, 70.14010656886952688, 1.798991495635525073 ) ) ;
#9361=CARTESIAN_POINT ( 'NONE',  ( 84.83259501155069415, 44.95299106343530582, 8.440442851456150919 ) ) ;
#9364=CARTESIAN_POINT ( 'NONE',  ( 74.13689204002625388, 68.84749506857346546, -11.26202041109552177 ) ) ;
#9385=CARTESIAN_POINT ( 'NONE',  ( 75.44414334788326926, 64.33299091768085987, 14.75074754958687429 ) ) ;
#9388=MANIFOLD_SOLID_BREP ( 'Fillet2', #24802 ) ;
#9390=CARTESIAN_POINT ( 'NONE',  ( 18.07869151248302941, 12.29860640527291338, -2.839279412974138328 ) ) ;
#9399=CARTESIAN_POINT ( 'NONE',  ( 31.74858474661088081, 18.73415679381823651, -6.890680421881970419E-14 ) ) ;
#9402=ORIENTED_EDGE ( 'NONE', *, *, #75737, .F. ) ;
#9405=CARTESIAN_POINT ( 'NONE',  ( 82.29734961797252879, 53.60383310410945512, 15.81226994477779790 ) ) ;
#9407=CARTESIAN_POINT ( 'NONE',  ( 75.72636783681542738, 65.12249353091223725, -14.45027308884206718 ) ) ;
#9415=CARTESIAN_POINT ( 'NONE',  ( 38.25529575686164208, 27.80170272979929535, 7.433330006724137462 ) ) ;
#9416=CARTESIAN_POINT ( 'NONE',  ( 73.01784879798562145, 70.40283164995553022, -8.092307369146576335 ) ) ;
#9418=CARTESIAN_POINT ( 'NONE',  ( 78.05395834205243943, 61.78695400133908322, 16.08488452160743165 ) ) ;
#9422=CARTESIAN_POINT ( 'NONE',  ( 79.43406943547307719, 59.55633321778628897, 16.18157302954037391 ) ) ;
#9425=CARTESIAN_POINT ( 'NONE',  ( 21.14026940803790566, 27.90829794293880539, 10.00000000000000355 ) ) ;
#9427=EDGE_CURVE ( 'NONE', #1759, #4426, #2559, .T. ) ;
#9428=CARTESIAN_POINT ( 'NONE',  ( 82.00481806099733717, 45.27543476315971560, -11.33045944147468020 ) ) ;
#9434=ORIENTED_EDGE ( 'NONE', *, *, #42423, .F. ) ;
#9435=CARTESIAN_POINT ( 'NONE',  ( 77.19776191479694205, 49.58695339317465312, -15.48335642945104595 ) ) ;
#9442=CARTESIAN_POINT ( 'NONE',  ( 70.71926666893401148, 71.45048000115950515, 3.795742845772093865 ) ) ;
#9455=CARTESIAN_POINT ( 'NONE',  ( 43.33837710268888799, 27.94754757982092741, 5.678558825948272215 ) ) ;
#9459=CARTESIAN_POINT ( 'NONE',  ( 83.92684454729288746, 43.42296649151629140, -7.738650150025851993 ) ) ;
#9462=CARTESIAN_POINT ( 'NONE',  ( 78.08206365161463225, 61.83366292688850763, -15.70979438352861735 ) ) ;
#9465=CARTESIAN_POINT ( 'NONE',  ( 73.53703480203567722, 67.51361842960002946, 11.62355896671093980 ) ) ;
#9469=CARTESIAN_POINT ( 'NONE',  ( 31.51172446742527100, 30.14441083166263269, 10.00000000000000533 ) ) ;
#9476=FACE_OUTER_BOUND ( 'NONE', #82869, .T. ) ;
#9484=EDGE_LOOP ( 'NONE', ( #93839, #48345, #75471, #1274 ) ) ;
#9491=EDGE_CURVE ( 'NONE', #73699, #56530, #68200, .T. ) ;
#9495=CARTESIAN_POINT ( 'NONE',  ( 74.35260113823048300, 68.48135296369000002, 11.70560402319359561 ) ) ;
#9498=CARTESIAN_POINT ( 'NONE',  ( 68.48067871107335236, 70.13512158218014747, 0.9310271535938260401 ) ) ;
#9501=CARTESIAN_POINT ( 'NONE',  ( 67.21538324255706698, 66.58946535461426208, 8.499949113996416727 ) ) ;
#9518=DIRECTION ( 'NONE',  ( -0.6793907169778431454, 0.000000000000000000, -0.7337767056021416989 ) ) ;
#9519=CARTESIAN_POINT ( 'NONE',  ( 73.81716743588172847, 56.51341352178555866, -16.05755937095091923 ) ) ;
#9522=CARTESIAN_POINT ( 'NONE',  ( 77.03509876804180578, 63.43842436480252900, -15.45738776637924516 ) ) ;
#9525=FACE_OUTER_BOUND ( 'NONE', #52660, .T. ) ;
#9526=CARTESIAN_POINT ( 'NONE',  ( 88.29618083833925368, 44.15377159048836830, 0.4144604853962327584 ) ) ;
#9528=CARTESIAN_POINT ( 'NONE',  ( 83.31851016613751426, 49.62898418713007231, -13.46204844297379388 ) ) ;
#9529=FACE_OUTER_BOUND ( 'NONE', #15122, .T. ) ;
#9533=CARTESIAN_POINT ( 'NONE',  ( 29.64435718874111458, 29.06628583063843152, -9.188101187500006262 ) ) ;
#9535=CARTESIAN_POINT ( 'NONE',  ( 78.55537653917157570, 48.00561504237174404, -13.97647359956260082 ) ) ;
#9537=CARTESIAN_POINT ( 'NONE',  ( 11.76515913632831101, 28.83396525600389282, -2.839279412974133887 ) ) ;
#9539=FACE_OUTER_BOUND ( 'NONE', #81835, .T. ) ;
#9543=CARTESIAN_POINT ( 'NONE',  ( 74.10110473074108484, 67.08709595610132226, 12.20209729311798341 ) ) ;
#9545=ORIENTED_EDGE ( 'NONE', *, *, #43878, .T. ) ;
#9547=CARTESIAN_POINT ( 'NONE',  ( 87.48880955142448101, 44.86412769470708639, -6.596395727433105094 ) ) ;
#9551=CARTESIAN_POINT ( 'NONE',  ( 86.36237991899166389, 47.04137177816882343, 10.01663566065926325 ) ) ;
#9556=CARTESIAN_POINT ( 'NONE',  ( 67.42721094069274557, 68.56443353946191621, -5.087393618767618975 ) ) ;
#9557=VERTEX_POINT ( 'NONE', #63072 ) ;
#9560=DIRECTION ( 'NONE',  ( 0.5000000000000013323, -0.8660254037844378194, 0.000000000000000000 ) ) ;
#9565=CARTESIAN_POINT ( 'NONE',  ( 29.59504171901726366, 22.80170272979927759, 7.433330006724137462 ) ) ;
#9566=CARTESIAN_POINT ( 'NONE',  ( 74.89653295760797391, 66.81943746227950953, -13.20645658646817999 ) ) ;
#9567=CARTESIAN_POINT ( 'NONE',  ( 78.71043930997907978, 49.45733721402466898, -14.60309932591205317 ) ) ;
#9591=ORIENTED_EDGE ( 'NONE', *, *, #59323, .T. ) ;
#9597=CARTESIAN_POINT ( 'NONE',  ( 82.14160159532623595, 47.93221979345100436, -12.80134787886038161 ) ) ;
#9602=ORIENTED_EDGE ( 'NONE', *, *, #69648, .F. ) ;
#9611=CARTESIAN_POINT ( 'NONE',  ( 88.00768034709845722, 44.38581256804975794, 4.745967170566630422 ) ) ;
#9614=CARTESIAN_POINT ( 'NONE',  ( 85.17088969497783069, 43.77888550337738138, -6.018426280060992895 ) ) ;
#9616=EDGE_CURVE ( 'NONE', #50075, #72450, #48853, .T. ) ;
#9627=CARTESIAN_POINT ( 'NONE',  ( 85.22848849487193945, 43.87423014350909511, 6.205650761890156630 ) ) ;
#9629=CARTESIAN_POINT ( 'NONE',  ( 83.17351638738638542, 52.27842989329151635, 14.84046717777660618 ) ) ;
#9633=EDGE_CURVE ( 'NONE', #55257, #35007, #54297, .T. ) ;
#9636=CARTESIAN_POINT ( 'NONE',  ( 72.40162949255979186, 64.46460395437595992, -13.26410053993346416 ) ) ;
#9637=CARTESIAN_POINT ( 'NONE',  ( 73.98409239102026902, 55.09210739743019758, 16.60304204205536394 ) ) ;
#9638=CARTESIAN_POINT ( 'NONE',  ( 69.84221642410084030, 62.80036841173330942, -13.30700940456985037 ) ) ;
#9639=CARTESIAN_POINT ( 'NONE',  ( 28.71959338928917305, 24.78052372038641593, -10.00000000000000355 ) ) ;
#9643=CYLINDRICAL_SURFACE ( 'NONE', #27497, 10.00000000000001066 ) ;
#9647=CARTESIAN_POINT ( 'NONE',  ( 82.28096079332273405, 48.10700144346920837, 12.86989513579583999 ) ) ;
#9651=DIRECTION ( 'NONE',  ( -0.7162481363636752363, 0.000000000000000000, -0.6978456900745050318 ) ) ;
#9652=CARTESIAN_POINT ( 'NONE',  ( 71.94509386275791485, 72.64380087153907084, -0.7818115889975479904 ) ) ;
#9655=CARTESIAN_POINT ( 'NONE',  ( 31.97641226934276659, 34.16454794089043645, -10.00000000000000355 ) ) ;
#9661=CARTESIAN_POINT ( 'NONE',  ( 83.55704177478077099, 51.98730140788479304, 15.00998877770037865 ) ) ;
#9672=CARTESIAN_POINT ( 'NONE',  ( 67.11050834814496113, 66.80207709080652023, -9.015407947737315908 ) ) ;
#9674=PLANE ( 'NONE',  #45900 ) ;
#9678=CARTESIAN_POINT ( 'NONE',  ( 25.58005199048888656, 32.95586893147756768, 7.433330006724141015 ) ) ;
#9683=CARTESIAN_POINT ( 'NONE',  ( 14.28983037092611319, 10.11110640527290627, -2.839279412974138328 ) ) ;
#9685=CARTESIAN_POINT ( 'NONE',  ( 79.53422710701454434, 57.48121895429935080, -16.24767348339593553 ) ) ;
#9687=ORIENTED_EDGE ( 'NONE', *, *, #57791, .T. ) ;
#9688=CARTESIAN_POINT ( 'NONE',  ( 72.21207746560659757, 71.58261399135965064, -5.866756630810175288 ) ) ;
#9689=CARTESIAN_POINT ( 'NONE',  ( 82.87596643829704135, 41.15858874971023340, 0.1873015203630768732 ) ) ;
#9696=CARTESIAN_POINT ( 'NONE',  ( 87.45625938901056884, 43.68296694889340870, -0.2840587573061720827 ) ) ;
#9698=CARTESIAN_POINT ( 'NONE',  ( 43.28410984748890655, 30.15404122711137447, 8.090169943749479842 ) ) ;
#9700=CARTESIAN_POINT ( 'NONE',  ( 72.60665278519202559, 57.41384979935430977, -16.32120458462707546 ) ) ;
#9701=CARTESIAN_POINT ( 'NONE',  ( 76.62156306105930526, 63.43458379359962152, 15.37592086074861619 ) ) ;
#9704=ADVANCED_FACE ( 'NONE', ( #88076 ), #72337, .T. ) ;
#9706=VECTOR ( 'NONE', #58487, 1000.000000000000114 ) ;
#9710=EDGE_LOOP ( 'NONE', ( #48029, #67394 ) ) ;
#9711=CARTESIAN_POINT ( 'NONE',  ( 35.44910642356613550, 21.26216523072496045, -2.296566073217252530E-15 ) ) ;
#9713=CARTESIAN_POINT ( 'NONE',  ( 71.34900412968279682, 70.70430146466247834, -6.675603849584609506 ) ) ;
#9717=CARTESIAN_POINT ( 'NONE',  ( 74.39841895140679640, 68.21392270468032848, 11.45628786500076046 ) ) ;
#9724=CARTESIAN_POINT ( 'NONE',  ( 85.13042836612673625, 43.09392175677057679, -4.294211889271497995 ) ) ;
#9729=CARTESIAN_POINT ( 'NONE',  ( 71.49202448901485241, 69.85859178648415480, -7.429879959600643069 ) ) ;
#9735=CARTESIAN_POINT ( 'NONE',  ( 66.36268096397610350, 69.44190093015801324, 9.875986171954755521E-07 ) ) ;
#9736=CARTESIAN_POINT ( 'NONE',  ( 67.37958206400872996, 66.94879931957503061, 9.026884747259803277 ) ) ;
#9742=CARTESIAN_POINT ( 'NONE',  ( 82.06353261700769508, 41.00057011406286733, -2.892018250819532454 ) ) ;
#9745=CARTESIAN_POINT ( 'NONE',  ( 83.72112933957373571, 51.48465111928251048, -14.37122866580464198 ) ) ;
#9748=CARTESIAN_POINT ( 'NONE',  ( 80.60151911206874331, 57.21366011616830605, -16.23031521152326206 ) ) ;
#9755=DIRECTION ( 'NONE',  ( -0.5000000000000014433, 0.8660254037844377084, 0.000000000000000000 ) ) ;
#9757=CARTESIAN_POINT ( 'NONE',  ( 85.44302523967576235, 48.29274922941779380, -11.75060226479814318 ) ) ;
#9758=DIRECTION ( 'NONE',  ( -0.8660254037844378194, -0.5000000000000014433, -0.000000000000000000 ) ) ;
#9761=CARTESIAN_POINT ( 'NONE',  ( 81.64018326908548318, 41.60497881960491640, 5.570940999012380601 ) ) ;
#9762=CARTESIAN_POINT ( 'NONE',  ( 88.33748333995926316, 44.07075497373335793, -2.898134731201826852 ) ) ;
#9767=CARTESIAN_POINT ( 'NONE',  ( 76.51423634175225175, 53.18905479164092043, -15.93784919710639691 ) ) ;
#9768=ORIENTED_EDGE ( 'NONE', *, *, #82806, .T. ) ;
#9770=CARTESIAN_POINT ( 'NONE',  ( 87.51647913336857698, 44.56403561216112053, 4.883618514853080406 ) ) ;
#9772=CARTESIAN_POINT ( 'NONE',  ( 11.36960171514096452, 30.65659080271450065, -1.878358725466461243E-16 ) ) ;
#9774=LINE ( 'NONE', #48253, #45224 ) ;
#9776=CARTESIAN_POINT ( 'NONE',  ( 66.45568218898124258, 67.84274271466240691, -6.745522493097580785 ) ) ;
#9777=CARTESIAN_POINT ( 'NONE',  ( 1.830000459568766003, 24.55466486950697202, 1.000260061240931054E-15 ) ) ;
#9790=CARTESIAN_POINT ( 'NONE',  ( 41.95273645663377238, 27.14754757982093381, -5.678558825948276656 ) ) ;
#9794=CARTESIAN_POINT ( 'NONE',  ( 35.39919958817179690, 22.29860640527294535, -2.839279412974138328 ) ) ;
#9797=CARTESIAN_POINT ( 'NONE',  ( 66.04046446033240159, 68.57277501975208622, 1.949611298710725915 ) ) ;
#9802=CARTESIAN_POINT ( 'NONE',  ( 6.007877864960585512, 21.65586893147753855, -7.433330006724137462 ) ) ;
#9804=CARTESIAN_POINT ( 'NONE',  ( 17.52000153575897912, 22.06628583063841020, -9.188101187500006262 ) ) ;
#9806=CARTESIAN_POINT ( 'NONE',  ( 84.63209989742584582, 49.90680382888324118, -13.65945482025744795 ) ) ;
#9809=ORIENTED_EDGE ( 'NONE', *, *, #4460, .T. ) ;
#9810=CARTESIAN_POINT ( 'NONE',  ( 29.85625172820832418, 25.43677371833803136, -10.00000000000000355 ) ) ;
#9813=CARTESIAN_POINT ( 'NONE',  ( 87.87588256303088485, 45.05834245088314560, 6.537532970176366476 ) ) ;
#9817=CARTESIAN_POINT ( 'NONE',  ( 86.10128179547638183, 47.01522930412664181, 10.71950609365847384 ) ) ;
#9818=CARTESIAN_POINT ( 'NONE',  ( 86.02805406347464157, 47.65264056766959300, 10.87896026205523370 ) ) ;
#9819=ORIENTED_EDGE ( 'NONE', *, *, #4205, .F. ) ;
#9820=CARTESIAN_POINT ( 'NONE',  ( 78.12080843744404035, 59.88224619964616835, 16.03904967186319297 ) ) ;
#9824=CARTESIAN_POINT ( 'NONE',  ( 79.18684305567126103, 59.44391592844134919, -16.53590917749602340 ) ) ;
#9825=CARTESIAN_POINT ( 'NONE',  ( 12.38042018312781067, 30.08080186712591697, -3.090169943749475845 ) ) ;
#9842=CARTESIAN_POINT ( 'NONE',  ( 83.70835292455117838, 51.17077017971526232, 14.19597355579030484 ) ) ;
#9845=CARTESIAN_POINT ( 'NONE',  ( 69.13686587061594935, 64.31895405193962745, 11.99662287724232357 ) ) ;
#9853=CARTESIAN_POINT ( 'NONE',  ( 21.45440292344354916, 18.10170272979926764, -7.433330006724141015 ) ) ;
#9861=DIRECTION ( 'NONE',  ( -0.8660254037844377084, -0.5000000000000014433, -0.000000000000000000 ) ) ;
#9863=CARTESIAN_POINT ( 'NONE',  ( 72.02064175744285990, 59.20208988331167888, 15.86477473724754184 ) ) ;
#9866=CARTESIAN_POINT ( 'NONE',  ( 8.323093432028223049, 20.50829794293878905, -10.00000000000000355 ) ) ;
#9872=CARTESIAN_POINT ( 'NONE',  ( 82.11422868418486587, 40.75191158806642022, -0.7887125810678616844 ) ) ;
#9873=CARTESIAN_POINT ( 'NONE',  ( 84.81058727987682744, 50.28540220845615494, 13.39370648373574824 ) ) ;
#9880=VERTEX_POINT ( 'NONE', #38271 ) ;
#9882=CARTESIAN_POINT ( 'NONE',  ( 79.90694551766156906, 47.07889366225261085, -13.03716703668656685 ) ) ;
#9883=CARTESIAN_POINT ( 'NONE',  ( 83.85717419902768199, 43.35873368085128021, 6.682989616040957870 ) ) ;
#9885=CARTESIAN_POINT ( 'NONE',  ( 41.54549712337441747, 24.39040679176986615, -6.890680421881970419E-14 ) ) ;
#9886=CARTESIAN_POINT ( 'NONE',  ( 88.67874521539408761, 45.12822637883663646, 1.911324073694122932E-15 ) ) ;
#9890=CARTESIAN_POINT ( 'NONE',  ( 82.04598463251571161, 43.24397476211455427, 8.160383678059524470 ) ) ;
#9892=ADVANCED_FACE ( 'NONE', ( #92047 ), #69182, .T. ) ;
#9894=CARTESIAN_POINT ( 'NONE',  ( 68.85868628182136320, 64.71584314351879641, -12.20120022179425234 ) ) ;
#9897=CARTESIAN_POINT ( 'NONE',  ( 71.71377818447290053, 68.16592558100862220, -10.55737487113105821 ) ) ;
#9905=CARTESIAN_POINT ( 'NONE',  ( 23.27484393518965788, 15.29860640527292226, -2.839279412974138328 ) ) ;
#9906=CARTESIAN_POINT ( 'NONE',  ( 75.26135223891184012, 66.78369140784673164, 12.92241541316169773 ) ) ;
#9911=CARTESIAN_POINT ( 'NONE',  ( 77.00910850481051284, 63.69207575539577704, -14.97815254220547487 ) ) ;
#9913=DIRECTION ( 'NONE',  ( -0.2925570654631174383, 0.000000000000000000, -0.9562480658530030375 ) ) ;
#9915=CARTESIAN_POINT ( 'NONE',  ( 81.45669997382150029, 55.98862135975877408, -16.04303691645969110 ) ) ;
#9916=ORIENTED_EDGE ( 'NONE', *, *, #22330, .T. ) ;
#9918=CARTESIAN_POINT ( 'NONE',  ( 19.85205661636063112, 27.16454794089041869, -10.00000000000000355 ) ) ;
#9920=ORIENTED_EDGE ( 'NONE', *, *, #18204, .F. ) ;
#9922=CARTESIAN_POINT ( 'NONE',  ( 83.90707806624753573, 51.69617421279772174, -14.41620133319961106 ) ) ;
#9924=CARTESIAN_POINT ( 'NONE',  ( 74.95533196993615377, 53.16522946876935407, -16.03279857048111978 ) ) ;
#9928=CARTESIAN_POINT ( 'NONE',  ( 42.23901261427005949, 30.10170272979930672, -7.433330006724141015 ) ) ;
#9935=CARTESIAN_POINT ( 'NONE',  ( 86.55406513359314147, 47.25665231443431935, -10.69898602647501562 ) ) ;
#9937=CARTESIAN_POINT ( 'NONE',  ( 28.24009562160082609, 16.70852965304480264, 1.583844403245364907 ) ) ;
#9938=CARTESIAN_POINT ( 'NONE',  ( 79.30008114732019919, 51.60973947141255280, -15.28311722500239966 ) ) ;
#9945=CARTESIAN_POINT ( 'NONE',  ( 77.31770070113016402, 49.73547290843352897, -14.99761632544347911 ) ) ;
#9949=CARTESIAN_POINT ( 'NONE',  ( 79.54765903714830699, 55.27048800625036762, 16.06385255412505231 ) ) ;
#9950=( BOUNDED_CURVE ( )  B_SPLINE_CURVE ( 2, ( #3704, #34582, #65482, #84706, #68958, #83207, #67972, #68460, #54237, #8172, #52753, #99880, #22367 ),
 .UNSPECIFIED., .F., .F. ) 
 B_SPLINE_CURVE_WITH_KNOTS ( ( 3, 2, 2, 2, 2, 2, 3 ),
 ( 0.4874999999999999889, 0.4899999999999999911, 0.4949999999999999956, 0.5000000000000000000, 0.5050000000000000044, 0.5100000000000000089, 0.5125000000000000666 ),
 .UNSPECIFIED. ) 
 CURVE ( )  GEOMETRIC_REPRESENTATION_ITEM ( )  RATIONAL_B_SPLINE_CURVE ( ( 0.9755282581475768211, 0.9755282581475768211, 1.000000000000000000, 0.9510565162951535312, 1.000000000000000000, 0.9510565162951535312, 1.000000000000000000, 0.9510565162951535312, 1.000000000000000000, 0.9510565162951535312, 1.000000000000000000, 0.9755282581475761550, 0.9755282581475767101 ) ) 
 REPRESENTATION_ITEM ( '' )  );
#9953=CARTESIAN_POINT ( 'NONE',  ( 25.48331929688331599, 38.21091486745862653, 7.012934429366973338E-14 ) ) ;
#9954=CARTESIAN_POINT ( 'NONE',  ( 70.62624074450191358, 71.35313954103614265, 3.953306911768213361 ) ) ;
#9960=B_SPLINE_CURVE_WITH_KNOTS ( 'NONE', 3,
 ( #93625, #1405, #24193, #32285, #63188, #24686, #94627, #25184, #7482, #30799 ),
 .UNSPECIFIED., .F., .F.,
 ( 4, 2, 2, 2, 4 ),
 ( 0.000000000000000000, 0.0002622400424273497836, 0.0005244800848546995672, 0.0007867201272820493509, 0.001048960169709399134 ),
 .UNSPECIFIED. ) ;
#9962=CARTESIAN_POINT ( 'NONE',  ( 70.65498028500805106, 61.41543102928405062, -14.81213469601333266 ) ) ;
#9964=CARTESIAN_POINT ( 'NONE',  ( 85.74281436412356072, 48.57633205417285893, -12.30481470458759219 ) ) ;
#9970=CARTESIAN_POINT ( 'NONE',  ( 73.05415939173641959, 65.68351150362803992, 12.75436733280234236 ) ) ;
#9972=CARTESIAN_POINT ( 'NONE',  ( 78.30344819242883148, 51.70502438984931359, 15.92195105728979421 ) ) ;
#9978=LINE ( 'NONE', #93086, #65565 ) ;
#9980=EDGE_LOOP ( 'NONE', ( #28608, #77947, #56522 ) ) ;
#9991=CARTESIAN_POINT ( 'NONE',  ( 73.49855677914850105, 61.97002789810530743, -14.76944323329657216 ) ) ;
#9994=CARTESIAN_POINT ( 'NONE',  ( 75.03295173686203157, 65.04298178550190812, -13.86991885877484698 ) ) ;
#9995=CARTESIAN_POINT ( 'NONE',  ( 85.51202090377952914, 48.04672559930133957, 11.47155550240170818 ) ) ;
#9996=CARTESIAN_POINT ( 'NONE',  ( 13.90996860267861024, 31.52903772873356303, -1.583844403245363575 ) ) ;
#10001=CARTESIAN_POINT ( 'NONE',  ( 88.00202013401596446, 44.76312363537992667, -4.611939438784355971 ) ) ;
#10007=CARTESIAN_POINT ( 'NONE',  ( 67.43106664880183132, 66.97720493292270305, 9.028648563732053489 ) ) ;
#10011=CARTESIAN_POINT ( 'NONE',  ( 82.47021907082941539, 53.30441442868470858, -15.33472904691311456 ) ) ;
#10013=ADVANCED_FACE ( 'NONE', ( #76789 ), #52989, .T. ) ;
#10014=CARTESIAN_POINT ( 'NONE',  ( 73.65729962767426287, 69.49757902785614760, 9.740712345197145794 ) ) ;
#10016=CARTESIAN_POINT ( 'NONE',  ( 77.06427544118604089, 63.50113506902185634, -15.44174958657458951 ) ) ;
#10020=CARTESIAN_POINT ( 'NONE',  ( 77.59354443008750479, 52.93461377476350549, -16.27594883185225072 ) ) ;
#10025=CARTESIAN_POINT ( 'NONE',  ( 28.93108252874724684, 32.10171378149919263, 9.188101187500008038 ) ) ;
#10029=CARTESIAN_POINT ( 'NONE',  ( 21.25954720759204974, 17.98920272979926338, 7.433330006724137462 ) ) ;
#10031=CARTESIAN_POINT ( 'NONE',  ( 76.65872121159138430, 63.56238613867309795, 15.33801735844474834 ) ) ;
#10036=CARTESIAN_POINT ( 'NONE',  ( 86.27668453731669729, 47.22199995466520761, 10.82669603042141304 ) ) ;
#10040=CARTESIAN_POINT ( 'NONE',  ( 75.18595658870128773, 53.28276008698350097, 16.02925223909795349 ) ) ;
#10046=CARTESIAN_POINT ( 'NONE',  ( 68.48697530863641703, 68.75015293434431385, -6.119310236332025532 ) ) ;
#10050=CARTESIAN_POINT ( 'NONE',  ( 79.43604583212312775, 46.39531899247212010, -12.74396782343451484 ) ) ;
#10053=ORIENTED_EDGE ( 'NONE', *, *, #37368, .T. ) ;
#10054=CARTESIAN_POINT ( 'NONE',  ( 31.23567208480136514, 20.96004757982091604, -5.678558825948275768 ) ) ;
#10055=CARTESIAN_POINT ( 'NONE',  ( 75.04096107751729505, 66.95220489134599973, -13.17375343603500149 ) ) ;
#10056=CARTESIAN_POINT ( 'NONE',  ( 84.04052627411616072, 48.12394913304956390, -12.17804820212080052 ) ) ;
#10057=ADVANCED_FACE ( 'NONE', ( #69683 ), #39755, .T. ) ;
#10064=CARTESIAN_POINT ( 'NONE',  ( 8.162811221194553823, 28.21091486745858745, -1.111400068045478839E-16 ) ) ;
#10067=CARTESIAN_POINT ( 'NONE',  ( 70.10520353637093649, 71.60267056347754533, -0.2412377010744407302 ) ) ;
#10068=CARTESIAN_POINT ( 'NONE',  ( 70.96429761875693032, 61.15374941679502996, 14.99935025239129871 ) ) ;
#10071=CARTESIAN_POINT ( 'NONE',  ( 77.55707599997003854, 60.86793710643906508, -16.22826185297084578 ) ) ;
#10072=DIRECTION ( 'NONE',  ( 0.1378186779084994706, -0.2387089523694924387, -0.9612616959383186721 ) ) ;
#10081=CARTESIAN_POINT ( 'NONE',  ( 79.90425123310397737, 44.57332524593454082, -11.10618635266240162 ) ) ;
#10085=CARTESIAN_POINT ( 'NONE',  ( 27.25975761432448152, 39.23654200823204263, 1.583844403245397769 ) ) ;
#10086=CARTESIAN_POINT ( 'NONE',  ( 79.97104311170529911, 48.47299295313705159, -13.83239755450518871 ) ) ;
#10092=DIRECTION ( 'NONE',  ( -0.5000000000000015543, 0.8660254037844377084, 0.000000000000000000 ) ) ;
#10093=VERTEX_POINT ( 'NONE', #71209 ) ;
#10095=CARTESIAN_POINT ( 'NONE',  ( 77.55626133878482165, 49.73613333205595666, 14.95107568548285037 ) ) ;
#10097=CARTESIAN_POINT ( 'NONE',  ( 88.24418735786636603, 44.41312371456485408, 4.416884733071428037 ) ) ;
#10104=CARTESIAN_POINT ( 'NONE',  ( 78.36279588851795097, 47.41043415324340771, -13.73196331463247688 ) ) ;
#10110=CARTESIAN_POINT ( 'NONE',  ( 77.98425798866018965, 61.79443237021894930, 16.07418881765925178 ) ) ;
#10118=CARTESIAN_POINT ( 'NONE',  ( 79.64960764401185145, 54.33444549161213644, 16.32474502074725820 ) ) ;
#10120=CARTESIAN_POINT ( 'NONE',  ( 31.15975419450677819, 23.15404122711134960, 8.090169943749479842 ) ) ;
#10128=CARTESIAN_POINT ( 'NONE',  ( 83.00132175467911111, 51.24136005855328335, 14.42644208312803578 ) ) ;
#10130=EDGE_CURVE ( 'NONE', #52745, #8972, #25885, .T. ) ;
#10133=CARTESIAN_POINT ( 'NONE',  ( 32.18369500442691589, 26.78052372038641948, -10.00000000000000355 ) ) ;
#10134=CARTESIAN_POINT ( 'NONE',  ( 72.07700700168975061, 72.29913914755536553, -0.9446506882752414569 ) ) ;
#10140=CARTESIAN_POINT ( 'NONE',  ( 29.52096178950397842, 38.81751292744057480, -6.180339887498951690 ) ) ;
#10144=CARTESIAN_POINT ( 'NONE',  ( 81.15053981873714406, 56.17130680763398942, 16.10758762198818417 ) ) ;
#10145=CARTESIAN_POINT ( 'NONE',  ( 14.64478397084458550, 10.58380873178785642, 6.180339887498953466 ) ) ;
#10148=ADVANCED_FACE ( 'NONE', ( #53967 ), #25078, .T. ) ;
#10149=CARTESIAN_POINT ( 'NONE',  ( 83.90995141641640487, 51.89037297248786729, 14.88406197085303972 ) ) ;
#10152=CARTESIAN_POINT ( 'NONE',  ( 69.61982051209052713, 66.78800749460349095, -10.00191460643801022 ) ) ;
#10159=LINE ( 'NONE', #78061, #24040 ) ;
#10165=CARTESIAN_POINT ( 'NONE',  ( 24.28583178621855865, 34.99752408145591431, 5.678558825948277544 ) ) ;
#10170=CARTESIAN_POINT ( 'NONE',  ( 12.71236424662705566, 15.84335787977761179, 9.188101187500006262 ) ) ;
#10176=CARTESIAN_POINT ( 'NONE',  ( 72.36468543301930367, 71.15458895874081691, -6.079547378801656521 ) ) ;
#10177=CYLINDRICAL_SURFACE ( 'NONE', #69382, 16.60714546451156792 ) ;
#10178=FACE_OUTER_BOUND ( 'NONE', #22012, .T. ) ;
#10188=CARTESIAN_POINT ( 'NONE',  ( 72.60433822694926675, 57.21714546342739283, -16.35209281813967763 ) ) ;
#10189=CARTESIAN_POINT ( 'NONE',  ( 76.63523979702124223, 63.50111620409151669, 15.35509843086873438 ) ) ;
#10199=CARTESIAN_POINT ( 'NONE',  ( 23.84800118292001159, 31.95586893147756058, 7.433330006724141015 ) ) ;
#10201=CARTESIAN_POINT ( 'NONE',  ( 78.14732411849692539, 47.76060378147906960, -13.97190537733660243 ) ) ;
#10204=CARTESIAN_POINT ( 'NONE',  ( 74.35260113823048300, 68.48135296369000002, 11.20560402319359561 ) ) ;
#10209=CARTESIAN_POINT ( 'NONE',  ( 75.01041914018598789, 58.43539866323090592, -15.92242282427785938 ) ) ;
#10211=CARTESIAN_POINT ( 'NONE',  ( 78.36958359800738094, 55.49686521012768026, 16.55473436304751900 ) ) ;
#10212=VERTEX_POINT ( 'NONE', #33189 ) ;
#10220=CARTESIAN_POINT ( 'NONE',  ( 75.78378987240938613, 65.61208117828051911, 13.82073902662707354 ) ) ;
#10224=ORIENTED_EDGE ( 'NONE', *, *, #50258, .T. ) ;
#10226=CARTESIAN_POINT ( 'NONE',  ( 84.54753597202504523, 42.62579540220287555, 3.803055962842035953 ) ) ;
#10229=CARTESIAN_POINT ( 'NONE',  ( 83.57459526254079663, 51.48179996603089137, -14.40656865850368717 ) ) ;
#10231=ORIENTED_EDGE ( 'NONE', *, *, #508, .T. ) ;
#10232=CARTESIAN_POINT ( 'NONE',  ( 80.56382388659234550, 57.17170686835115845, -16.22950384588643402 ) ) ;
#10234=CARTESIAN_POINT ( 'NONE',  ( 72.85283338774588913, 70.95119525769652569, 7.785565881738502725 ) ) ;
#10241=CARTESIAN_POINT ( 'NONE',  ( 72.69493809724967548, 71.16443809380129437, -7.267007365939463170 ) ) ;
#10245=CARTESIAN_POINT ( 'NONE',  ( 71.88059653590643450, 71.08635078533735907, -5.573730649155103301 ) ) ;
#10248=PLANE ( 'NONE',  #41810 ) ;
#10251=( BOUNDED_CURVE ( )  B_SPLINE_CURVE ( 2, ( #17864, #70036, #94880, #87332, #71067, #8257, #9256, #72063, #33554, #77671, #62942, #23434, #54321 ),
 .UNSPECIFIED., .F., .T. ) 
 B_SPLINE_CURVE_WITH_KNOTS ( ( 3, 2, 2, 2, 2, 2, 3 ),
 ( 0.2124999999999999944, 0.2149999999999999967, 0.2200000000000000011, 0.2250000000000000056, 0.2300000000000000100, 0.2349999999999999867, 0.2374999999999999889 ),
 .UNSPECIFIED. ) 
 CURVE ( )  GEOMETRIC_REPRESENTATION_ITEM ( )  RATIONAL_B_SPLINE_CURVE ( ( 0.9755282581475768211, 0.9755282581475768211, 1.000000000000000000, 0.9510565162951535312, 1.000000000000000000, 0.9510565162951535312, 1.000000000000000000, 0.9510565162951535312, 1.000000000000000000, 0.9510565162951535312, 1.000000000000000000, 0.9755282581475768211, 0.9755282581475768211 ) ) 
 REPRESENTATION_ITEM ( '' )  );
#10253=CARTESIAN_POINT ( 'NONE',  ( 81.31123310220682754, 51.67285451222524983, -14.93676299417988318 ) ) ;
#10259=CARTESIAN_POINT ( 'NONE',  ( 22.25607796093117230, 24.80066082961421969, 10.00000000000000533 ) ) ;
#10260=CARTESIAN_POINT ( 'NONE',  ( 68.27244882330454345, 65.69410988500804649, -10.30841495897560023 ) ) ;
#10263=CARTESIAN_POINT ( 'NONE',  ( 74.00705488591727033, 54.85690809062158024, -16.13415776006375424 ) ) ;
#10276=CARTESIAN_POINT ( 'NONE',  ( 34.84050961144773595, 32.06628583063844218, -9.188101187500006262 ) ) ;
#10280=CARTESIAN_POINT ( 'NONE',  ( 28.84929788977513709, 34.84336893147758474, -7.433330006724137462 ) ) ;
#10283=CARTESIAN_POINT ( 'NONE',  ( 80.86506773606531340, 42.95500482456080249, -9.556183558881794937 ) ) ;
#10286=CARTESIAN_POINT ( 'NONE',  ( 8.860943796042899834, 20.51421378149916919, -9.188101187500004485 ) ) ;
#10288=CARTESIAN_POINT ( 'NONE',  ( 14.99289142922413021, 26.84336893147755276, -7.433330006724137462 ) ) ;
#10297=CARTESIAN_POINT ( 'NONE',  ( 87.65336964024139377, 45.10687245489099695, 6.884500160062607677 ) ) ;
#10304=CARTESIAN_POINT ( 'NONE',  ( 85.95939684119618107, 47.60785808554223308, 10.87377621121526339 ) ) ;
#10306=CARTESIAN_POINT ( 'NONE',  ( 77.53002750585342540, 56.25820219453329685, 16.17037978242485607 ) ) ;
#10308=ORIENTED_EDGE ( 'NONE', *, *, #90259, .T. ) ;
#10309=CARTESIAN_POINT ( 'NONE',  ( 78.38752765249786592, 61.22447296964845975, -15.89000806468494531 ) ) ;
#10314=CARTESIAN_POINT ( 'NONE',  ( 21.02495994229494514, 13.10801979619928304, 3.090169943749476733 ) ) ;
#10327=CARTESIAN_POINT ( 'NONE',  ( 80.20857538925844210, 44.21345027839175401, -11.30608575764590107 ) ) ;
#10328=EDGE_LOOP ( 'NONE', ( #4813, #23791, #92118, #38673 ) ) ;
#10335=CARTESIAN_POINT ( 'NONE',  ( 70.17933292656275057, 66.80308542599925659, 10.34396498317840596 ) ) ;
#10341=CARTESIAN_POINT ( 'NONE',  ( 16.26188567080226477, 32.49540643055187417, 3.479690158560446702E-15 ) ) ;
#10346=ORIENTED_EDGE ( 'NONE', *, *, #79852, .T. ) ;
#10356=CARTESIAN_POINT ( 'NONE',  ( 81.62382999622622037, 59.34769798152620268, 0.4414737964294616623 ) ) ;
#10362=CARTESIAN_POINT ( 'NONE',  ( 82.36066395365664050, 40.35653381656560867, -0.9401641086475391873 ) ) ;
#10363=CARTESIAN_POINT ( 'NONE',  ( 84.67479249306344968, 50.56977290030206262, 13.61422284357908197 ) ) ;
#10370=CARTESIAN_POINT ( 'NONE',  ( 79.65783702838581348, 47.13130848700988906, -13.15621609857660523 ) ) ;
#10371=CARTESIAN_POINT ( 'NONE',  ( 82.71995705146288458, 41.94179129365014802, 4.898035795836064743 ) ) ;
#10373=AXIS2_PLACEMENT_3D ( 'NONE', #16530, #91571, #335 ) ;
#10376=CARTESIAN_POINT ( 'NONE',  ( 74.21864607481936105, 68.58553829006309854, -11.54532566021463502 ) ) ;
#10380=CARTESIAN_POINT ( 'NONE',  ( 79.31967116076749846, 59.78699023733837237, -16.51284638439522112 ) ) ;
#10385=FACE_OUTER_BOUND ( 'NONE', #58845, .T. ) ;
#10398=CARTESIAN_POINT ( 'NONE',  ( 13.67041502465407277, 29.93396525600389424, 2.839279412974139660 ) ) ;
#10399=CARTESIAN_POINT ( 'NONE',  ( 75.03253579078814539, 67.12707870640632279, 13.05283704309126414 ) ) ;
#10409=CARTESIAN_POINT ( 'NONE',  ( 81.36199125831662116, 55.41608345602817565, -16.32668456146281244 ) ) ;
#10414=B_SPLINE_CURVE_WITH_KNOTS ( 'NONE', 3,
 ( #91126, #59157, #5493, #90129, #98714, #21691, #28790, #37863, #22186, #97713, #36376, #21204, #52571, #67281, #20703, #35884, #98207, #59670, #51591, #14090, #6494, #90644, #75913, #37372, #53080, #84033, #6980, #14592, #45471, #68772, #99696 ),
 .UNSPECIFIED., .F., .F.,
 ( 4, 3, 3, 3, 3, 3, 3, 3, 3, 3, 4 ),
 ( 0.000000000000000000, 0.1333490885032329043, 0.3007194338854160542, 0.4699862290244992691, 0.5844252810809290599, 0.6686540514502579136, 0.7354980260655432645, 0.8028463152565632477, 0.8633854507757217078, 0.9437142632667381292, 1.000000000000000000 ),
 .UNSPECIFIED. ) ;
#10415=CARTESIAN_POINT ( 'NONE',  ( 80.04281669451169989, 53.86981617844637782, 15.76102994265571411 ) ) ;
#10416=CARTESIAN_POINT ( 'NONE',  ( 83.76063610407190652, 51.49572955327540313, -14.36612422999478866 ) ) ;
#10417=CARTESIAN_POINT ( 'NONE',  ( 70.15559162998948750, 71.15866369468874097, 0.8108420958401643119 ) ) ;
#10419=EDGE_CURVE ( 'NONE', #79111, #86732, #84317, .T. ) ;
#10421=CARTESIAN_POINT ( 'NONE',  ( 41.44395331530407844, 35.87878583063845639, -9.188101187500006262 ) ) ;
#10424=CARTESIAN_POINT ( 'NONE',  ( 77.78993031024410243, 61.70844822385715389, 16.06828208845739780 ) ) ;
#10428=CARTESIAN_POINT ( 'NONE',  ( 78.88256717313477395, 59.65579592159198086, 16.50129574805686161 ) ) ;
#10429=CARTESIAN_POINT ( 'NONE',  ( 76.77731254116881132, 64.09355814141257213, -15.16545583891343263 ) ) ;
#10430=CARTESIAN_POINT ( 'NONE',  ( 87.99887978206298556, 43.75530803335438890, -2.234124107031381534 ) ) ;
#10432=CARTESIAN_POINT ( 'NONE',  ( 84.72693717884534692, 49.96098312850357104, -13.65910992477957819 ) ) ;
#10438=DIRECTION ( 'NONE',  ( 0.5000000000000014433, -0.8660254037844378194, 0.000000000000000000 ) ) ;
#10441=ORIENTED_EDGE ( 'NONE', *, *, #73824, .T. ) ;
#10442=CARTESIAN_POINT ( 'NONE',  ( 74.38298257480929010, 55.99886258023348518, 16.10773052095676405 ) ) ;
#10443=CARTESIAN_POINT ( 'NONE',  ( 77.95436975687957215, 48.11784896437987413, 14.20357318872345331 ) ) ;
#10445=DIRECTION ( 'NONE',  ( -0.3715724127386920705, 0.6435822975543701308, -0.6691306063588670083 ) ) ;
#10447=DIRECTION ( 'NONE',  ( -0.5000000000000082157, 0.8660254037844338226, 0.000000000000000000 ) ) ;
#10449=LINE ( 'NONE', #94576, #83548 ) ;
#10450=CARTESIAN_POINT ( 'NONE',  ( 81.30818518503046732, 58.89441083166271085, 0.000000000000000000 ) ) ;
#10455=CARTESIAN_POINT ( 'NONE',  ( 88.02796755599807454, 43.59779901362369259, -1.172627947537940913E-07 ) ) ;
#10458=CARTESIAN_POINT ( 'NONE',  ( 30.82187231905848535, 18.76426979415091267, 3.090169943749476733 ) ) ;
#10462=CARTESIAN_POINT ( 'NONE',  ( 75.99750771566300500, 65.44421971917601866, -13.95497799904430458 ) ) ;
#10474=DIRECTION ( 'NONE',  ( -0.8503781557569302096, 0.05328141121993809626, -0.5234673661555743207 ) ) ;
#10483=CARTESIAN_POINT ( 'NONE',  ( 72.34523945420380642, 62.27941420626569169, -14.34989103246101827 ) ) ;
#10485=CARTESIAN_POINT ( 'NONE',  ( 73.08007996217260427, 65.63861575768015655, -12.79487007168413015 ) ) ;
#10486=CARTESIAN_POINT ( 'NONE',  ( 85.05511982866016751, 46.74444827917869816, 10.44744734522612717 ) ) ;
#10487=CARTESIAN_POINT ( 'NONE',  ( 80.78918961562681034, 43.20779693872438543, -9.098606657379754381 ) ) ;
#10488=CARTESIAN_POINT ( 'NONE',  ( 67.55525932531482169, 69.43178850908184074, 2.233867015644889431 ) ) ;
#10495=CARTESIAN_POINT ( 'NONE',  ( 74.24029763082349120, 55.47955095029949746, -16.12046342301015756 ) ) ;
#10500=LINE ( 'NONE', #88559, #63731 ) ;
#10502=EDGE_CURVE ( 'NONE', #57260, #55973, #29576, .T. ) ;
#10503=CARTESIAN_POINT ( 'NONE',  ( 77.09103540138860922, 55.43591893971357365, -16.15323720810845742 ) ) ;
#10504=CARTESIAN_POINT ( 'NONE',  ( 79.22212042028705525, 45.73389709458791685, -12.98434876985491115 ) ) ;
#10508=CARTESIAN_POINT ( 'NONE',  ( 73.60600985167290844, 69.76719088550383674, 9.400953274917574376 ) ) ;
#10509=EDGE_CURVE ( 'NONE', #10212, #78334, #45043, .T. ) ;
#10511=CARTESIAN_POINT ( 'NONE',  ( 77.07143086693146472, 63.53409821367920784, -15.43182057973166188 ) ) ;
#10517=CARTESIAN_POINT ( 'NONE',  ( 88.06269261788010283, 43.61796610520789841, 0.05835779599787579291 ) ) ;
#10523=CARTESIAN_POINT ( 'NONE',  ( 37.13125039574066477, 23.29860640527294535, -2.839279412974138328 ) ) ;
#10524=CARTESIAN_POINT ( 'NONE',  ( 82.56061938396526045, 50.68218938071114366, 14.69501007283553307 ) ) ;
#10527=CARTESIAN_POINT ( 'NONE',  ( 13.49720994389718598, 29.83396525600389637, -2.839279412974133887 ) ) ;
#10534=LINE ( 'NONE', #50023, #37268 ) ;
#10540=CARTESIAN_POINT ( 'NONE',  ( 28.28448313147312021, 16.73415679381822230, 1.333680081654574804E-15 ) ) ;
#10543=VERTEX_POINT ( 'NONE', #59959 ) ;
#10545=LINE ( 'NONE', #73347, #19101 ) ;
#10554=CARTESIAN_POINT ( 'NONE',  ( 46.69726203620875538, 27.36477965099643583, 1.583844403245330712 ) ) ;
#10556=CARTESIAN_POINT ( 'NONE',  ( 33.05914333415502426, 24.80170272979928470, 7.433330006724137462 ) ) ;
#10557=CARTESIAN_POINT ( 'NONE',  ( 84.88550499454136400, 50.14668325075617616, -13.29646903481718745 ) ) ;
#10558=CARTESIAN_POINT ( 'NONE',  ( 85.29133164726557936, 47.82314596797873918, -11.37170031403014114 ) ) ;
#10567=CARTESIAN_POINT ( 'NONE',  ( 81.77537817921462704, 55.54508588803495428, -15.95796652904217439 ) ) ;
#10570=CARTESIAN_POINT ( 'NONE',  ( 70.33074575655678018, 61.13420976129943796, 14.85339103883890566 ) ) ;
#10573=CARTESIAN_POINT ( 'NONE',  ( 79.57595289148407858, 59.38824344631919416, 16.55667218292645515 ) ) ;
#10585=CARTESIAN_POINT ( 'NONE',  ( 84.15416455708074750, 41.95829577234375307, -1.425225784223129732 ) ) ;
#10591=DIRECTION ( 'NONE',  ( 0.8660254037844378194, 0.5000000000000016653, 0.000000000000000000 ) ) ;
#10592=VERTEX_POINT ( 'NONE', #91917 ) ;
#10594=CARTESIAN_POINT ( 'NONE',  ( 76.10709454405099450, 64.72268328886903532, -14.35831925167281398 ) ) ;
#10596=CARTESIAN_POINT ( 'NONE',  ( 87.51070308547132015, 44.87157588833125033, -6.586006751413206572 ) ) ;
#10598=CARTESIAN_POINT ( 'NONE',  ( 87.78141208182009336, 44.24254441107329683, 4.709165031671993518 ) ) ;
#10600=CARTESIAN_POINT ( 'NONE',  ( 87.23971111752899787, 44.08784344967020274, -3.737494627976594597 ) ) ;
#10602=CARTESIAN_POINT ( 'NONE',  ( 81.16146148815955996, 46.97546385808738734, 12.48307154572201938 ) ) ;
#10606=FACE_OUTER_BOUND ( 'NONE', #8343, .T. ) ;
#10608=ORIENTED_EDGE ( 'NONE', *, *, #43490, .T. ) ;
#10611=CARTESIAN_POINT ( 'NONE',  ( 83.59213118347814486, 42.01539464043647598, 3.571310749328834522 ) ) ;
#10613=CARTESIAN_POINT ( 'NONE',  ( 83.14954596509920748, 52.21800694492112882, 14.82118944672224714 ) ) ;
#10617=CARTESIAN_POINT ( 'NONE',  ( 36.39373221054007246, 21.41603393254327159, -1.583844403245362020 ) ) ;
#10619=CARTESIAN_POINT ( 'NONE',  ( 74.33967961526438728, 63.91161072895079798, -14.20272303067961950 ) ) ;
#10622=CARTESIAN_POINT ( 'NONE',  ( 69.58400947765115063, 62.48688437104875248, -13.40551765113508331 ) ) ;
#10624=CARTESIAN_POINT ( 'NONE',  ( 34.95497629653712579, 28.38052372038643156, 10.00000000000000533 ) ) ;
#10626=CARTESIAN_POINT ( 'NONE',  ( 81.55388316527243830, 43.41730979745093322, -9.640312318338271069 ) ) ;
#10628=CARTESIAN_POINT ( 'NONE',  ( 71.70264960794062858, 59.22880258761407646, -15.30490172258937953 ) ) ;
#10633=CARTESIAN_POINT ( 'NONE',  ( 81.25623871648237184, 45.26464092063801559, 11.05715119619013187 ) ) ;
#10636=CARTESIAN_POINT ( 'NONE',  ( 87.13739461745468873, 46.26069895958453060, 8.495900850489460865 ) ) ;
#10643=CARTESIAN_POINT ( 'NONE',  ( 30.42216059839860165, 41.65659080271453973, -1.878358725466461243E-16 ) ) ;
#10650=CARTESIAN_POINT ( 'NONE',  ( 84.07138645536940658, 51.57118087273712348, 14.70185406139690976 ) ) ;
#10656=ORIENTED_EDGE ( 'NONE', *, *, #75850, .F. ) ;
#10659=CARTESIAN_POINT ( 'NONE',  ( 67.02216205416458195, 66.98564243900641202, -8.693011569217512502 ) ) ;
#10664=CARTESIAN_POINT ( 'NONE',  ( 70.66235305853896875, 64.93978938733117445, 12.81966862783717964 ) ) ;
#10665=CARTESIAN_POINT ( 'NONE',  ( 27.58754685475307156, 27.87878583063842797, -9.188101187500006262 ) ) ;
#10670=CARTESIAN_POINT ( 'NONE',  ( 15.73863525846626032, 14.80170272979925272, 7.433330006724137462 ) ) ;
#10672=DIRECTION ( 'NONE',  ( -0.03487823687206607903, 0.06041087834084090530, 0.9975640502598237536 ) ) ;
#10674=CARTESIAN_POINT ( 'NONE',  ( 72.19109158906037749, 71.10838548458626462, -5.953967166465981897 ) ) ;
#10677=CARTESIAN_POINT ( 'NONE',  ( 67.86860378221429357, 65.58690806574966814, -10.91583492536020472 ) ) ;
#10684=CARTESIAN_POINT ( 'NONE',  ( 72.04989860578065475, 72.29315785138345518, -3.506402493552649435 ) ) ;
#10685=CARTESIAN_POINT ( 'NONE',  ( 73.11398337492714461, 57.41976801426039856, -15.88230524335126148 ) ) ;
#10686=CARTESIAN_POINT ( 'NONE',  ( 78.21052395450516315, 61.02929962668400066, -15.90929906019731099 ) ) ;
#10693=ORIENTED_EDGE ( 'NONE', *, *, #87886, .T. ) ;
#10696=CARTESIAN_POINT ( 'NONE',  ( 28.38624132378439313, 39.49540643055189548, 3.479690158560446702E-15 ) ) ;
#10698=CARTESIAN_POINT ( 'NONE',  ( 78.22897022588638549, 47.73976331551912011, -14.48630821629448384 ) ) ;
#10701=CARTESIAN_POINT ( 'NONE',  ( 73.91288345017510153, 68.57868192222672121, 11.39134523673512511 ) ) ;
#10707=CARTESIAN_POINT ( 'NONE',  ( 78.29659894437797618, 57.29271133927426263, -16.19830913213783319 ) ) ;
#10710=ORIENTED_EDGE ( 'NONE', *, *, #91820, .T. ) ;
#10725=CARTESIAN_POINT ( 'NONE',  ( 86.56107662385767298, 44.24251769246640720, -5.392801405849540153 ) ) ;
#10730=CARTESIAN_POINT ( 'NONE',  ( 79.49833928707691655, 59.53565285605930768, -16.19549232290340157 ) ) ;
#10733=ORIENTED_EDGE ( 'NONE', *, *, #83221, .T. ) ;
#10734=CARTESIAN_POINT ( 'NONE',  ( 80.27314967653323663, 57.13666510169645107, -16.23447001446601590 ) ) ;
#10744=ADVANCED_FACE ( 'NONE', ( #2186 ), #49276, .T. ) ;
#10745=CARTESIAN_POINT ( 'NONE',  ( 15.75562222995320560, 27.83478043621387599, -8.090169943749479842 ) ) ;
#10753=CARTESIAN_POINT ( 'NONE',  ( 82.15503656874240335, 51.38971310115279323, -14.65386453280463819 ) ) ;
#10755=EDGE_CURVE ( 'NONE', #50031, #77129, #51146, .T. ) ;
#10761=CARTESIAN_POINT ( 'NONE',  ( 18.12000580879176681, 26.16454794089041513, -10.00000000000000355 ) ) ;
#10762=CARTESIAN_POINT ( 'NONE',  ( 85.93449727955278661, 48.41344338607260767, 12.08598331734388509 ) ) ;
#10764=CARTESIAN_POINT ( 'NONE',  ( 72.24659094707693896, 72.05232748221199301, -3.244599947448891797 ) ) ;
#10767=CARTESIAN_POINT ( 'NONE',  ( 73.97864017645115098, 55.44741841079105882, -16.11550171815304111 ) ) ;
#10774=AXIS2_PLACEMENT_3D ( 'NONE', #13457, #83372, #68621 ) ;
#10779=CARTESIAN_POINT ( 'NONE',  ( 40.22068564906490451, 26.14754757982093381, -5.678558825948276656 ) ) ;
#10782=CARTESIAN_POINT ( 'NONE',  ( 35.11595366814305663, 25.98920272979928470, 7.433330006724137462 ) ) ;
#10788=CARTESIAN_POINT ( 'NONE',  ( 3.501222095392049649, 22.99752408145588944, 5.678558825948277544 ) ) ;
#10790=CARTESIAN_POINT ( 'NONE',  ( 13.78045586392592092, 26.14336893147754282, 7.433330006724141015 ) ) ;
#10791=CARTESIAN_POINT ( 'NONE',  ( 72.49386282319785835, 57.57572440859879492, 15.80166580940835885 ) ) ;
#10795=CARTESIAN_POINT ( 'NONE',  ( 84.55537670905214043, 50.62155581810768012, -14.09136642048690291 ) ) ;
#10797=CARTESIAN_POINT ( 'NONE',  ( 87.83899792242847582, 44.00541668311378629, -1.848955303085625390 ) ) ;
#10801=CARTESIAN_POINT ( 'NONE',  ( 66.08271157691945064, 68.62646445644681137, 4.299565650807243067 ) ) ;
#10806=CARTESIAN_POINT ( 'NONE',  ( 86.15223587325151300, 47.11913640227773925, 10.79538652562921541 ) ) ;
#10808=CARTESIAN_POINT ( 'NONE',  ( 76.54141439059615948, 51.80385272469369795, 15.68951548868696300 ) ) ;
#10812=CARTESIAN_POINT ( 'NONE',  ( 78.28735576227695958, 50.40689703484141404, -15.06222486931144111 ) ) ;
#10814=CARTESIAN_POINT ( 'NONE',  ( 21.31189239132533331, 12.70852965304479198, 1.583844403245364907 ) ) ;
#10836=CARTESIAN_POINT ( 'NONE',  ( 41.97168754484824404, 36.18347333012635403, -9.594050593750004907 ) ) ;
#10837=CARTESIAN_POINT ( 'NONE',  ( 26.24098094315136009, 17.01110640527292972, 2.839279412974134775 ) ) ;
#10842=CARTESIAN_POINT ( 'NONE',  ( 85.69563749947228359, 42.25122789774620458, -8.045052972278457832E-08 ) ) ;
#10857=( BOUNDED_CURVE ( )  B_SPLINE_CURVE ( 2, ( #51508, #74839, #13037, #12529, #4413, #59081, #58593, #14012, #83445, #44891, #90052, #66221, #21134 ),
 .UNSPECIFIED., .F., .T. ) 
 B_SPLINE_CURVE_WITH_KNOTS ( ( 3, 2, 2, 2, 2, 2, 3 ),
 ( 0.1125000000000000028, 0.1150000000000000050, 0.1199999999999999956, 0.1250000000000000000, 0.1300000000000000044, 0.1350000000000000089, 0.1375000000000000111 ),
 .UNSPECIFIED. ) 
 CURVE ( )  GEOMETRIC_REPRESENTATION_ITEM ( )  RATIONAL_B_SPLINE_CURVE ( ( 0.9755282581475768211, 0.9755282581475768211, 1.000000000000000000, 0.9510565162951535312, 1.000000000000000000, 0.9510565162951535312, 1.000000000000000000, 0.9510565162951535312, 1.000000000000000000, 0.9510565162951535312, 1.000000000000000000, 0.9755282581475768211, 0.9755282581475768211 ) ) 
 REPRESENTATION_ITEM ( '' )  );
#10864=CARTESIAN_POINT ( 'NONE',  ( 12.22230530498201873, 30.55466486950698624, -1.111400068045478839E-16 ) ) ;
#10881=CARTESIAN_POINT ( 'NONE',  ( 83.93631839880838186, 47.12607340849465487, 11.39547821726712051 ) ) ;
#10887=CARTESIAN_POINT ( 'NONE',  ( 68.70336459149662289, 64.02807437409755664, -12.02912010802727316 ) ) ;
#10895=EDGE_LOOP ( 'NONE', ( #61637, #32246, #11883, #4466 ) ) ;
#10900=CARTESIAN_POINT ( 'NONE',  ( 18.53877768333398990, 26.10171378149918198, 9.188101187500008038 ) ) ;
#10902=CARTESIAN_POINT ( 'NONE',  ( 75.07027850253338386, 67.11046765588916685, 13.07895222455245232 ) ) ;
#10910=VECTOR ( 'NONE', #94141, 1000.000000000000114 ) ;
#10913=CARTESIAN_POINT ( 'NONE',  ( 81.56748776902772136, 55.16552677673315941, -15.91734106113700342 ) ) ;
#10917=VECTOR ( 'NONE', #14864, 1000.000000000000000 ) ;
#10919=CARTESIAN_POINT ( 'NONE',  ( 72.08176305907363712, 72.32341480998664451, 0.8068646397873169285 ) ) ;
#10928=CARTESIAN_POINT ( 'NONE',  ( 7.283862947486897887, 19.90829794293878408, 10.00000000000000355 ) ) ;
#10931=CARTESIAN_POINT ( 'NONE',  ( 77.73453021100772276, 61.59708935479353897, 16.08607222837813566 ) ) ;
#10932=EDGE_CURVE ( 'NONE', #25358, #30622, #12929, .T. ) ;
#10936=CARTESIAN_POINT ( 'NONE',  ( 78.86219776201926379, 59.55369065033507070, 16.50996775951928441 ) ) ;
#10938=CARTESIAN_POINT ( 'NONE',  ( 88.10271290040205372, 43.80081590334129515, -2.139902876137079080 ) ) ;
#10939=DIRECTION ( 'NONE',  ( -0.8660254037844379305, -0.5000000000000014433, -0.000000000000000000 ) ) ;
#10942=CARTESIAN_POINT ( 'NONE',  ( 73.47309087361824709, 69.99741330878467238, -9.625970422713120200 ) ) ;
#10943=CARTESIAN_POINT ( 'NONE',  ( 84.63209989742584582, 49.90680382888324118, -13.65945482025744795 ) ) ;
#10956=CARTESIAN_POINT ( 'NONE',  ( 82.40463100666525520, 40.71042483417762980, 3.199549863589999266 ) ) ;
#10965=CARTESIAN_POINT ( 'NONE',  ( 70.93212201657662774, 61.12454710469379648, -14.47427800527280795 ) ) ;
#10966=B_SPLINE_CURVE_WITH_KNOTS ( 'NONE', 3,
 ( #24197, #93124, #55078, #1905, #94630, #23675, #47486, #17594, #78411, #54567, #8992, #32786, #16092, #70800, #63694, #86554, #1409, #48503, #32290, #25187, #63191, #17086, #56069, #47978 ),
 .UNSPECIFIED., .F., .F.,
 ( 4, 2, 2, 2, 2, 2, 2, 2, 2, 2, 2, 4 ),
 ( 0.000000000000000000, 0.1250000000000144884, 0.2500000000000289768, 0.3750000000000434652, 0.4375000000000391354, 0.5000000000000348610, 0.5625000000000305311, 0.6250000000000262013, 0.6875000000000219824, 0.7500000000000176525, 0.8750000000000087708, 1.000000000000000000 ),
 .UNSPECIFIED. ) ;
#10967=CARTESIAN_POINT ( 'NONE',  ( 45.07042791025775585, 28.94754757982093452, 5.678558825948272215 ) ) ;
#10969=CARTESIAN_POINT ( 'NONE',  ( 85.90518370574052653, 43.58569018707092368, -5.829448724985482500 ) ) ;
#10976=EDGE_CURVE ( 'NONE', #84127, #59353, #14903, .T. ) ;
#10978=CARTESIAN_POINT ( 'NONE',  ( 78.12943550715658603, 47.76092654452022401, 14.52429885557054057 ) ) ;
#10980=EDGE_CURVE ( 'NONE', #40695, #50208, #3926, .T. ) ;
#10981=CARTESIAN_POINT ( 'NONE',  ( 76.31143563843063760, 51.61816296641098489, -15.67522282572066850 ) ) ;
#10985=CARTESIAN_POINT ( 'NONE',  ( 76.01432959614969320, 61.89104940659418475, -15.35760132559815005 ) ) ;
#10987=AXIS2_PLACEMENT_3D ( 'NONE', #28190, #59066, #20610 ) ;
#10996=CARTESIAN_POINT ( 'NONE',  ( 87.80273158879131756, 44.12514266115443462, 2.714529260603524286 ) ) ;
#11002=CARTESIAN_POINT ( 'NONE',  ( 75.45848158068072564, 64.88927211188989475, -14.08658606194572727 ) ) ;
#11005=CARTESIAN_POINT ( 'NONE',  ( 80.96872438510855829, 43.68017817554169113, -9.540616427834850199 ) ) ;
#11011=CARTESIAN_POINT ( 'NONE',  ( 88.11801461435689475, 44.35549720747543745, -4.463913325698415591 ) ) ;
#11013=CYLINDRICAL_SURFACE ( 'NONE', #7561, 16.60714546451156792 ) ;
#11023=CARTESIAN_POINT ( 'NONE',  ( 80.06011714963352688, 53.70964243608271005, -16.15649400312684492 ) ) ;
#11029=CARTESIAN_POINT ( 'NONE',  ( 83.16599801226564637, 42.97050380912442336, -7.691725848249192588 ) ) ;
#11032=CARTESIAN_POINT ( 'NONE',  ( 34.51455378690028652, 28.43085787977765477, -9.188101187500008038 ) ) ;
#11033=CARTESIAN_POINT ( 'NONE',  ( 83.70644011242923455, 48.17923023345559841, -12.88485594781891841 ) ) ;
#11034=CARTESIAN_POINT ( 'NONE',  ( 14.42807667092211865, 8.734156793818204534, -7.779800476318352071E-15 ) ) ;
#11035=EDGE_LOOP ( 'NONE', ( #76855, #93072, #13158, #90200 ) ) ;
#11036=CARTESIAN_POINT ( 'NONE',  ( 21.36958804686389612, 14.19860640527291906, 2.839279412974134775 ) ) ;
#11038=CARTESIAN_POINT ( 'NONE',  ( 75.28650001057751240, 66.67572118895704136, 13.44401380721711270 ) ) ;
#11044=CARTESIAN_POINT ( 'NONE',  ( 72.45903907735083749, 71.58914108862926184, 5.178295322198071204 ) ) ;
#11047=CARTESIAN_POINT ( 'NONE',  ( 19.10612102538523160, 34.52903772873358434, -1.583844403245329602 ) ) ;
#11053=DIRECTION ( 'NONE',  ( 0.4755282581475757664, -0.8236391035463335175, -0.3090169943749448977 ) ) ;
#11059=CARTESIAN_POINT ( 'NONE',  ( 71.96464922262767061, 71.55750601381073750, 5.589292941210044496 ) ) ;
#11067=CARTESIAN_POINT ( 'NONE',  ( 31.37760429443828869, 33.51421378149921537, -9.188101187500004485 ) ) ;
#11069=CARTESIAN_POINT ( 'NONE',  ( 79.14312167556931854, 57.64441083166269664, 0.000000000000000000 ) ) ;
#11077=CARTESIAN_POINT ( 'NONE',  ( 85.44439542427645051, 48.29040533209811059, -11.74811922390697738 ) ) ;
#11084=CARTESIAN_POINT ( 'NONE',  ( 79.58917286194427732, 59.33460254692537461, 16.56081879078485741 ) ) ;
#11089=ORIENTED_EDGE ( 'NONE', *, *, #76838, .T. ) ;
#11092=CARTESIAN_POINT ( 'NONE',  ( 79.93734396971494505, 44.49601230399111529, -11.01925363558071069 ) ) ;
#11103=CARTESIAN_POINT ( 'NONE',  ( 73.67824366217406862, 55.52431661998091528, 16.58293631993679540 ) ) ;
#11108=CARTESIAN_POINT ( 'NONE',  ( 75.79167905567804553, 65.12415201610325255, -14.46789148266619485 ) ) ;
#11111=CARTESIAN_POINT ( 'NONE',  ( 68.98939262229419001, 69.25400323834284677, -5.717648734987297310 ) ) ;
#11113=CARTESIAN_POINT ( 'NONE',  ( 87.58100233665301459, 44.90480556695516867, -6.571228966301012164 ) ) ;
#11115=CARTESIAN_POINT ( 'NONE',  ( 81.29539683296886210, 43.25976067974499273, 9.624898955577574355 ) ) ;
#11121=CARTESIAN_POINT ( 'NONE',  ( 71.55517591705296354, 59.48308490877587928, -15.70938992770603093 ) ) ;
#11128=CARTESIAN_POINT ( 'NONE',  ( 78.28176711274900867, 61.66836085159184933, 15.77706035593199196 ) ) ;
#11129=FACE_OUTER_BOUND ( 'NONE', #2455, .T. ) ;
#11133=VECTOR ( 'NONE', #13188, 1000.000000000000114 ) ;
#11137=CARTESIAN_POINT ( 'NONE',  ( 31.01755306704832194, 42.00034080476293497, -1.878358725466461243E-16 ) ) ;
#11138=CARTESIAN_POINT ( 'NONE',  ( 78.23911696424225681, 47.73527672355887574, 13.93191159841320825 ) ) ;
#11141=B_SPLINE_CURVE_WITH_KNOTS ( 'NONE', 3,
 ( #21509, #43792, #20521, #59983, #68095, #52890, #52394, #66108, #21029, #74238, #83842, #82852, #67596, #74735, #58492, #60476 ),
 .UNSPECIFIED., .F., .F.,
 ( 4, 1, 2, 2, 2, 1, 2, 2, 4 ),
 ( 0.000000000000000000, 0.1250000000000008604, 0.1875000000000018596, 0.2500000000000028311, 0.5000000000000042188, 0.6250000000000045519, 0.6875000000000034417, 0.7500000000000022204, 1.000000000000000000 ),
 .UNSPECIFIED. ) ;
#11142=CARTESIAN_POINT ( 'NONE',  ( 71.85273313970169795, 59.31805131066353454, -15.30413012561420771 ) ) ;
#11149=CARTESIAN_POINT ( 'NONE',  ( 86.58136378248637754, 46.32108903705595537, 9.037364168832199951 ) ) ;
#11150=CARTESIAN_POINT ( 'NONE',  ( 24.22498904768565353, 14.39040679176983062, 1.333680081654574804E-15 ) ) ;
#11152=CARTESIAN_POINT ( 'NONE',  ( 81.94607988216938566, 41.18096579325325024, 5.530507272723311551 ) ) ;
#11158=CARTESIAN_POINT ( 'NONE',  ( 30.83758659773572575, 40.73705186507756082, -3.090169943749475845 ) ) ;
#11164=CARTESIAN_POINT ( 'NONE',  ( 83.38731009417298878, 51.80618739314797949, 14.97569794390972397 ) ) ;
#11179=CARTESIAN_POINT ( 'NONE',  ( 32.96772289237024012, 21.96004757982091959, -5.678558825948276656 ) ) ;
#11180=CARTESIAN_POINT ( 'NONE',  ( 72.96724880819495240, 70.75172224442833624, -7.458605312651823915 ) ) ;
#11184=CARTESIAN_POINT ( 'NONE',  ( 18.60133699236122240, 19.24335787977762990, -9.188101187500008038 ) ) ;
#11187=ORIENTED_EDGE ( 'NONE', *, *, #60172, .F. ) ;
#11188=CARTESIAN_POINT ( 'NONE',  ( 72.06693479607845632, 71.51559350784613400, -5.828149303013867133 ) ) ;
#11191=CARTESIAN_POINT ( 'NONE',  ( 71.42110848219473951, 65.04516533590125960, -13.05791646362531466 ) ) ;
#11192=ORIENTED_EDGE ( 'NONE', *, *, #66881, .F. ) ;
#11201=CARTESIAN_POINT ( 'NONE',  ( 72.26191451101281871, 71.91445694603925176, -5.118044210176695863 ) ) ;
#11202=CARTESIAN_POINT ( 'NONE',  ( 78.09292022067579353, 61.02350456329286033, -15.89647179981830405 ) ) ;
#11206=DIRECTION ( 'NONE',  ( -0.5000000000000013323, 0.8660254037844379305, 0.000000000000000000 ) ) ;
#11211=ORIENTED_EDGE ( 'NONE', *, *, #342, .F. ) ;
#11212=CARTESIAN_POINT ( 'NONE',  ( 31.85034293892215018, 41.49540643055189548, 3.479690158560446702E-15 ) ) ;
#11214=CARTESIAN_POINT ( 'NONE',  ( 78.50112015865835247, 48.01465776021366594, -13.99615223866804570 ) ) ;
#11222=CARTESIAN_POINT ( 'NONE',  ( 80.28198526002465485, 56.49958842488598521, -16.15443186264643316 ) ) ;
#11241=CARTESIAN_POINT ( 'NONE',  ( 86.21802580015948081, 44.21772915329312070, -5.774872143548296144 ) ) ;
#11243=CARTESIAN_POINT ( 'NONE',  ( 78.60735446187599962, 47.91558663937576057, -14.46554739992950189 ) ) ;
#11246=CARTESIAN_POINT ( 'NONE',  ( 76.30616544034060666, 50.97262258187969763, -15.53540872755634439 ) ) ;
#11248=CARTESIAN_POINT ( 'NONE',  ( 80.44110801039052205, 57.53904330600535388, -16.59063950305211677 ) ) ;
#11256=CARTESIAN_POINT ( 'NONE',  ( 67.85514785513115044, 68.63529022595450613, 5.540876512699765222 ) ) ;
#11260=CARTESIAN_POINT ( 'NONE',  ( 19.55501378379531019, 16.45404122711132899, -8.090169943749478065 ) ) ;
#11267=CARTESIAN_POINT ( 'NONE',  ( 17.41189581114303309, 28.79103043416549212, 8.090169943749478065 ) ) ;
#11269=AXIS2_PLACEMENT_3D ( 'NONE', #94150, #18116, #18626 ) ;
#11270=CARTESIAN_POINT ( 'NONE',  ( 66.79965368539949111, 67.34049316045133082, -6.934348251617318049 ) ) ;
#11277=CARTESIAN_POINT ( 'NONE',  ( 21.19599769036394576, 20.43677371833801004, -10.00000000000000355 ) ) ;
#11282=CARTESIAN_POINT ( 'NONE',  ( 73.84183722536076289, 55.07373432386307144, -16.12662324738414910 ) ) ;
#11285=CARTESIAN_POINT ( 'NONE',  ( 75.02164697668396798, 67.17574075851680959, 12.57494967656429985 ) ) ;
#11286=CARTESIAN_POINT ( 'NONE',  ( 26.07214984898741150, 33.79103043416550634, 8.090169943749478065 ) ) ;
#11294=CARTESIAN_POINT ( 'NONE',  ( 30.99092310034283315, 39.93396525600392977, 2.839279412974139660 ) ) ;
#11298=CARTESIAN_POINT ( 'NONE',  ( 30.66313333631613247, 33.10171378149921395, 9.188101187500008038 ) ) ;
#11300=CARTESIAN_POINT ( 'NONE',  ( 25.36820930315042943, 19.81029122506294726, 8.090169943749479842 ) ) ;
#11302=CARTESIAN_POINT ( 'NONE',  ( 80.93613592869992601, 42.95327845849681836, -9.503115154567232992 ) ) ;
#11306=CARTESIAN_POINT ( 'NONE',  ( 6.965323710529800927, 24.99752408145590366, 5.678558825948277544 ) ) ;
#11308=CARTESIAN_POINT ( 'NONE',  ( 21.54279312762077936, 14.29860640527291871, -2.839279412974138328 ) ) ;
#11311=PLANE ( 'NONE',  #20905 ) ;
#11313=CARTESIAN_POINT ( 'NONE',  ( 81.18465792105908463, 42.40984018312481396, 7.627542571750448808 ) ) ;
#11318=DIRECTION ( 'NONE',  ( -0.4924038765061016787, 0.8528685319524424990, -0.1736481776669404342 ) ) ;
#11319=CARTESIAN_POINT ( 'NONE',  ( 87.56358751521999295, 45.50810825807865712, 6.913240104252196261 ) ) ;
#11324=CARTESIAN_POINT ( 'NONE',  ( 86.13530110067358692, 47.09369226531615737, 10.77952153921811096 ) ) ;
#11325=ORIENTED_EDGE ( 'NONE', *, *, #80665, .F. ) ;
#11328=ORIENTED_EDGE ( 'NONE', *, *, #19494, .T. ) ;
#11329=CARTESIAN_POINT ( 'NONE',  ( 69.12672858200174630, 64.33651235087042153, -11.97836756590942997 ) ) ;
#11337=ORIENTED_EDGE ( 'NONE', *, *, #6965, .F. ) ;
#11344=ORIENTED_EDGE ( 'NONE', *, *, #66396, .F. ) ;
#11346=ORIENTED_EDGE ( 'NONE', *, *, #91621, .F. ) ;
#11350=CARTESIAN_POINT ( 'NONE',  ( 70.79402339348382611, 68.13029754943326566, 9.272317926153396783 ) ) ;
#11353=CARTESIAN_POINT ( 'NONE',  ( 87.57621950688576362, 43.92368059598960883, 2.290041065490416194 ) ) ;
#11358=CARTESIAN_POINT ( 'NONE',  ( 29.50362127723248662, 19.96004757982091604, -5.678558825948276656 ) ) ;
#11360=CARTESIAN_POINT ( 'NONE',  ( 77.53640704328023503, 49.75990552807767386, -14.96334311224574165 ) ) ;
#11364=VERTEX_POINT ( 'NONE', #85976 ) ;
#11365=EDGE_CURVE ( 'NONE', #94954, #80395, #62087, .T. ) ;
#11368=EDGE_CURVE ( 'NONE', #35356, #52194, #32702, .T. ) ;
#11369=CARTESIAN_POINT ( 'NONE',  ( 72.04811769650321196, 71.35602353065118564, 5.168332083721268511 ) ) ;
#11377=CARTESIAN_POINT ( 'NONE',  ( 12.62681055351980497, 12.45404122711131656, -8.090169943749478065 ) ) ;
#11382=CARTESIAN_POINT ( 'NONE',  ( 82.53545809363272667, 41.02697948193551269, -1.178820010245875682 ) ) ;
#11388=VERTEX_POINT ( 'NONE', #310 ) ;
#11390=CARTESIAN_POINT ( 'NONE',  ( 66.88838894469625984, 68.52338324295652683, 4.302485449169815013 ) ) ;
#11401=CARTESIAN_POINT ( 'NONE',  ( 69.12006753439638373, 64.33743317121387406, -11.97457433615276123 ) ) ;
#11403=LINE ( 'NONE', #51356, #53187 ) ;
#11413=CARTESIAN_POINT ( 'NONE',  ( 85.22110914792114045, 48.09116874191089153, 12.16284421431235785 ) ) ;
#11415=CARTESIAN_POINT ( 'NONE',  ( 25.38156110457203241, 15.44966523072494624, -2.296566073217252530E-15 ) ) ;
#11416=CARTESIAN_POINT ( 'NONE',  ( 75.25260660042954441, 66.87649888114015084, 12.86011724376103338 ) ) ;
#11417=ADVANCED_FACE ( 'NONE', ( #63602 ), #86469, .T. ) ;
#11423=ORIENTED_EDGE ( 'NONE', *, *, #81877, .T. ) ;
#11428=CARTESIAN_POINT ( 'NONE',  ( 81.62004238798716926, 55.61031524971931361, -16.33394531952002993 ) ) ;
#11434=CARTESIAN_POINT ( 'NONE',  ( 85.24547482218825678, 44.72709687800012546, 7.712155500878341563 ) ) ;
#11436=CARTESIAN_POINT ( 'NONE',  ( 83.88232353660403362, 51.62541775870871419, -14.39191172970312671 ) ) ;
#11437=CARTESIAN_POINT ( 'NONE',  ( 71.66369827319218189, 72.02185750324218816, -1.551229696566573502 ) ) ;
#11441=CARTESIAN_POINT ( 'NONE',  ( 44.74566838383860556, 28.76004757982093807, 5.678558825948272215 ) ) ;
#11444=CARTESIAN_POINT ( 'NONE',  ( 77.84925963432132789, 61.76067837358136359, 16.06420508523131119 ) ) ;
#11446=CARTESIAN_POINT ( 'NONE',  ( 72.06470348997973474, 72.25603645428110156, 1.367373202405273602 ) ) ;
#11447=ORIENTED_EDGE ( 'NONE', *, *, #26867, .T. ) ;
#11448=CARTESIAN_POINT ( 'NONE',  ( 78.75376543412218666, 59.99366791223036444, 16.11417685114693299 ) ) ;
#11452=CARTESIAN_POINT ( 'NONE',  ( 84.55094438110296551, 49.89265462440669552, -13.67900519688966021 ) ) ;
#11456=( BOUNDED_CURVE ( )  B_SPLINE_CURVE ( 2, ( #56217, #25331, #87214, #34433, #64336, #42029, #17749, #48649, #79584, #10145, #41010, #18746, #87714 ),
 .UNSPECIFIED., .F., .T. ) 
 B_SPLINE_CURVE_WITH_KNOTS ( ( 3, 2, 2, 2, 2, 2, 3 ),
 ( 0.06250000000000000000, 0.06500000000000000222, 0.07000000000000000666, 0.07499999999999999722, 0.08000000000000000167, 0.08500000000000000611, 0.08750000000000000833 ),
 .UNSPECIFIED. ) 
 CURVE ( )  GEOMETRIC_REPRESENTATION_ITEM ( )  RATIONAL_B_SPLINE_CURVE ( ( 0.9755282581475768211, 0.9755282581475768211, 1.000000000000000000, 0.9510565162951535312, 1.000000000000000000, 0.9510565162951535312, 1.000000000000000000, 0.9510565162951535312, 1.000000000000000000, 0.9510565162951535312, 1.000000000000000000, 0.9755282581475767101, 0.9755282581475768211 ) ) 
 REPRESENTATION_ITEM ( '' )  );
#11459=VERTEX_POINT ( 'NONE', #25095 ) ;
#11462=CARTESIAN_POINT ( 'NONE',  ( 74.79904262356255629, 57.81733164762822241, 15.98236516859485867 ) ) ;
#11468=CARTESIAN_POINT ( 'NONE',  ( 82.16908567409906539, 40.68835713038597390, 3.666464688308268993 ) ) ;
#11473=CARTESIAN_POINT ( 'NONE',  ( 85.48084685767805979, 42.33396824294695904, -2.482615992588285803 ) ) ;
#11475=EDGE_CURVE ( 'NONE', #121, #35007, #46389, .T. ) ;
#11477=CARTESIAN_POINT ( 'NONE',  ( 88.03957972502300322, 43.60450335154009593, 0.01945071491020158166 ) ) ;
#11478=CARTESIAN_POINT ( 'NONE',  ( 10.98031343905817714, 14.84335787977761001, 9.188101187500006262 ) ) ;
#11479=VERTEX_POINT ( 'NONE', #86973 ) ;
#11481=CARTESIAN_POINT ( 'NONE',  ( 85.45699573997251264, 48.32332763657781527, -12.23527099237750981 ) ) ;
#11490=CARTESIAN_POINT ( 'NONE',  ( 88.11584858642071083, 44.14570234724004649, -1.721659289381729963 ) ) ;
#11493=CARTESIAN_POINT ( 'NONE',  ( 65.83788420375942962, 69.13770088707153150, 0.1877971835443447424 ) ) ;
#11496=B_SPLINE_CURVE_WITH_KNOTS ( 'NONE', 3,
 ( #44413, #67727, #73838, #98651, #44906, #4428, #37310, #8911, #92555, #30722 ),
 .UNSPECIFIED., .F., .F.,
 ( 4, 2, 2, 2, 4 ),
 ( 0.000000000000000000, 0.0002622400424273968922, 0.0005244800848547937844, 0.0007867201272821907308, 0.001048960169709587569 ),
 .UNSPECIFIED. ) ;
#11502=CARTESIAN_POINT ( 'NONE',  ( 88.16334560026523093, 43.89615744693332289, 2.509484348711646273 ) ) ;
#11505=CARTESIAN_POINT ( 'NONE',  ( 75.20678305874149316, 61.44858071201250027, -15.30768782187949029 ) ) ;
#11507=CARTESIAN_POINT ( 'NONE',  ( 72.59318785522671647, 65.75921281613393887, -12.50631930651069723 ) ) ;
#11509=CARTESIAN_POINT ( 'NONE',  ( 80.93651615306337987, 43.67145026278060271, -9.552024319604889513 ) ) ;
#11514=CARTESIAN_POINT ( 'NONE',  ( 88.01192408641850307, 44.27121890238829138, -4.391744778743014166 ) ) ;
#11522=CARTESIAN_POINT ( 'NONE',  ( 75.67111234668428210, 55.92069150990298709, -16.15888377404129628 ) ) ;
#11523=CARTESIAN_POINT ( 'NONE',  ( 79.57426776854913442, 46.24084366570346560, -13.18946159588284139 ) ) ;
#11528=EDGE_CURVE ( 'NONE', #46236, #62365, #7340, .T. ) ;
#11533=CARTESIAN_POINT ( 'NONE',  ( 32.39518414388500389, 34.10171378149921395, 9.188101187500008038 ) ) ;
#11537=CARTESIAN_POINT ( 'NONE',  ( 18.53877768333398990, 26.10171378149918198, 9.188101187500008038 ) ) ;
#11544=CARTESIAN_POINT ( 'NONE',  ( 86.72415995732357885, 47.00718562526229505, 10.33097223407348686 ) ) ;
#11546=CARTESIAN_POINT ( 'NONE',  ( 72.36540186540696595, 71.57331123994032396, 5.085634937608116246 ) ) ;
#11549=CARTESIAN_POINT ( 'NONE',  ( 75.10222324744135847, 53.09139496487031806, 16.49549906635234819 ) ) ;
#11560=CARTESIAN_POINT ( 'NONE',  ( 5.287540158160898507, 21.79103043416546726, 8.090169943749478065 ) ) ;
#11562=CARTESIAN_POINT ( 'NONE',  ( 87.77887691218910504, 44.16646017302762317, -4.484802941535585674 ) ) ;
#11564=CARTESIAN_POINT ( 'NONE',  ( 32.07042461746583939, 33.91421378149920685, 9.188101187500008038 ) ) ;
#11575=CARTESIAN_POINT ( 'NONE',  ( 85.94639921072385391, 48.27664717140825701, 11.96740676232643352 ) ) ;
#11589=CARTESIAN_POINT ( 'NONE',  ( 87.11651898459504650, 46.29685661633757832, -9.218154771921559743 ) ) ;
#11590=EDGE_CURVE ( 'NONE', #33116, #9076, #56993, .T. ) ;
#11592=CARTESIAN_POINT ( 'NONE',  ( 37.75007554933399234, 22.76426979415092333, 3.090169943749476733 ) ) ;
#11596=ORIENTED_EDGE ( 'NONE', *, *, #70963, .T. ) ;
#11604=CARTESIAN_POINT ( 'NONE',  ( 68.91323701008126079, 69.24239215680682946, -5.639282044092864155 ) ) ;
#11606=CARTESIAN_POINT ( 'NONE',  ( 69.48953819294759171, 62.61851694872117235, -13.86937595337403728 ) ) ;
#11612=CARTESIAN_POINT ( 'NONE',  ( 82.16988580781558937, 40.62906898968385860, -3.430093734972964548 ) ) ;
#11615=CARTESIAN_POINT ( 'NONE',  ( 65.88310562893973099, 69.02589174555536999, 1.996831191813060347 ) ) ;
#11619=CARTESIAN_POINT ( 'NONE',  ( 70.42903375700203128, 70.52137667656469944, -4.659989608922488813 ) ) ;
#11621=CARTESIAN_POINT ( 'NONE',  ( 83.39698567699524290, 51.83659370627650276, 14.98600084375454244 ) ) ;
#11623=ADVANCED_FACE ( 'NONE', ( #96055 ), #19537, .T. ) ;
#11626=CARTESIAN_POINT ( 'NONE',  ( 71.55914530767435622, 64.65954455392433431, -12.81547558104803031 ) ) ;
#11628=CARTESIAN_POINT ( 'NONE',  ( 78.86178680068651659, 50.42561631414478285, 15.44278421312068694 ) ) ;
#11629=CARTESIAN_POINT ( 'NONE',  ( 30.83975393042360480, 33.50829794293883168, -10.00000000000000355 ) ) ;
#11633=CARTESIAN_POINT ( 'NONE',  ( 86.67335767502150645, 43.67802127306630666, -3.448278313570464881 ) ) ;
#11639=EDGE_LOOP ( 'NONE', ( #66708, #86996, #68038, #58250 ) ) ;
#11640=CARTESIAN_POINT ( 'NONE',  ( 86.70078377113696888, 46.42938884419434942, 9.090660191201401119 ) ) ;
#11643=CARTESIAN_POINT ( 'NONE',  ( 81.94721816817228444, 41.71691344098891818, 5.409604974753337459 ) ) ;
#11645=CARTESIAN_POINT ( 'NONE',  ( 86.94335770270596697, 46.00923847012510493, 8.969699243401572986 ) ) ;
#11647=CARTESIAN_POINT ( 'NONE',  ( 31.26830227169403997, 36.79103043416551344, 8.090169943749478065 ) ) ;
#11651=CARTESIAN_POINT ( 'NONE',  ( 72.08705432318760131, 67.71326266777748515, -10.59477395882420225 ) ) ;
#11653=CARTESIAN_POINT ( 'NONE',  ( 83.63860429472313740, 52.00081728452853014, 14.99618877770984859 ) ) ;
#11654=EDGE_CURVE ( 'NONE', #99059, #63734, #30315, .T. ) ;
#11657=CARTESIAN_POINT ( 'NONE',  ( 75.40263629470850049, 53.17004129013850644, 16.48570774626835700 ) ) ;
#11658=CARTESIAN_POINT ( 'NONE',  ( 37.49256495613256845, 26.81029122506297568, 8.090169943749479842 ) ) ;
#11659=ORIENTED_EDGE ( 'NONE', *, *, #73090, .T. ) ;
#11661=ORIENTED_EDGE ( 'NONE', *, *, #4696, .F. ) ;
#11670=CARTESIAN_POINT ( 'NONE',  ( 29.31959766232195008, 28.87878583063843152, -9.188101187500006262 ) ) ;
#11674=VECTOR ( 'NONE', #13438, 999.9999999999998863 ) ;
#11675=EDGE_LOOP ( 'NONE', ( #26368, #29342, #92404, #77047 ) ) ;
#11676=CARTESIAN_POINT ( 'NONE',  ( 16.48196734934595398, 24.91421378149918198, 9.188101187500008038 ) ) ;
#11677=CARTESIAN_POINT ( 'NONE',  ( 69.03518170984699509, 64.49507618471645287, 12.45339560606362461 ) ) ;
#11681=CARTESIAN_POINT ( 'NONE',  ( 72.25718139279801733, 71.61371966692031776, -5.855127513239330561 ) ) ;
#11684=ORIENTED_EDGE ( 'NONE', *, *, #80105, .T. ) ;
#11691=ORIENTED_EDGE ( 'NONE', *, *, #88127, .T. ) ;
#11692=CARTESIAN_POINT ( 'NONE',  ( 66.15182308703052172, 68.59394279077463352, -2.211977090278242297 ) ) ;
#11694=CARTESIAN_POINT ( 'NONE',  ( 73.02887634090247104, 57.43239839248311540, -15.87220953312935201 ) ) ;
#11695=CARTESIAN_POINT ( 'NONE',  ( 78.03830882516994905, 61.03761899432888782, -15.88690189282890231 ) ) ;
#11702=CARTESIAN_POINT ( 'NONE',  ( 30.77620441319551503, 35.95586893147757479, 7.433330006724141015 ) ) ;
#11711=CARTESIAN_POINT ( 'NONE',  ( 74.39278055389422661, 58.62799419530674783, -15.82512888129269157 ) ) ;
#11712=CARTESIAN_POINT ( 'NONE',  ( 88.08526958130826756, 44.05723934618831095, -0.5494347720344661123 ) ) ;
#11714=ORIENTED_EDGE ( 'NONE', *, *, #44332, .T. ) ;
#11716=CARTESIAN_POINT ( 'NONE',  ( 68.88217923695410150, 69.54816024699961474, -4.775671802712312619 ) ) ;
#11728=CARTESIAN_POINT ( 'NONE',  ( 87.01675511858377376, 44.28642545908458317, -4.855627809373741499 ) ) ;
#11734=CARTESIAN_POINT ( 'NONE',  ( 80.35060322210587458, 57.11308289743137578, -16.23202674241575849 ) ) ;
#11742=CARTESIAN_POINT ( 'NONE',  ( 69.07022550912036252, 70.00077902694121690, 3.705957357846692446 ) ) ;
#11746=B_SPLINE_SURFACE_WITH_KNOTS ( 'NONE', 3, 1, ( 
 ( #66134, #96084 ),
 ( #58520, #89018 ),
 ( #19569, #87520 ),
 ( #11468, #18051 ),
 ( #27150, #50429 ),
 ( #26642, #35233 ),
 ( #2868, #43320 ),
 ( #74266, #57525 ),
 ( #80897, #97562 ),
 ( #34240, #11952 ),
 ( #42810, #18554 ),
 ( #73743, #42322 ),
 ( #97082, #88005 ),
 ( #4335, #73251 ),
 ( #80386, #88501 ),
 ( #19063, #41827 ),
 ( #3845, #89493 ),
 ( #20052, #50924 ),
 ( #10956, #81874 ),
 ( #49433, #12451 ),
 ( #35734, #41318 ),
 ( #66631, #72262 ),
 ( #72774, #33757 ),
 ( #95598, #3366 ),
 ( #26145, #57023 ),
 ( #21536, #53414 ),
 ( #90485, #29629 ),
 ( #98047, #99045 ),
 ( #82391, #84362 ),
 ( #21057, #37220 ),
 ( #52418, #74760 ) ),
 .UNSPECIFIED., .F., .F., .F.,
 ( 4, 3, 3, 3, 3, 3, 3, 3, 3, 3, 4 ),
 ( 2, 2 ),
 ( 0.000000000000000000, 0.1122669598086752790, 0.2243161639709619903, 0.3396355846219121233, 0.4553962076585190699, 0.5677860799922404000, 0.6749047109689705337, 0.7773884377078417174, 0.8775581155834378810, 0.9782364162378134331, 1.000000000000000000 ),
 ( 0.000000000000000000, 1.000000000000000000 ),
 .UNSPECIFIED. ) ;
#11747=CARTESIAN_POINT ( 'NONE',  ( 22.51478983128357925, 15.12755873383625982, -6.180339887498949025 ) ) ;
#11755=CARTESIAN_POINT ( 'NONE',  ( 25.95703985525452850, 15.39040679176983240, 1.333680081654574804E-15 ) ) ;
#11756=ORIENTED_EDGE ( 'NONE', *, *, #76601, .T. ) ;
#11764=CARTESIAN_POINT ( 'NONE',  ( 13.93250452138409479, 29.81751292744056059, -6.180339887498951690 ) ) ;
#11769=CARTESIAN_POINT ( 'NONE',  ( 74.14735107364549549, 55.49514332839016362, -16.11765820591672949 ) ) ;
#11772=CARTESIAN_POINT ( 'NONE',  ( 76.76222887016557195, 59.42175249350923849, 16.38682359597675742 ) ) ;
#11775=ADVANCED_FACE ( 'NONE', ( #85333 ), #25100, .T. ) ;
#11784=CARTESIAN_POINT ( 'NONE',  ( 80.60685564337630638, 57.64637852931380024, -16.24314337822399779 ) ) ;
#11787=CARTESIAN_POINT ( 'NONE',  ( 34.84050961144773595, 32.06628583063844218, -9.188101187500006262 ) ) ;
#11792=CARTESIAN_POINT ( 'NONE',  ( 38.71056063283548809, 34.30066082961425167, -10.00000000000000533 ) ) ;
#11795=CARTESIAN_POINT ( 'NONE',  ( 9.941082954516854642, 14.24335787977761036, -9.188101187500008038 ) ) ;
#11796=CARTESIAN_POINT ( 'NONE',  ( 71.78242053751056062, 72.53632993589366151, 0.9980050652678106315 ) ) ;
#11797=CARTESIAN_POINT ( 'NONE',  ( 19.96532700332172183, 20.03085787977762422, 9.188101187500006262 ) ) ;
#11803=ORIENTED_EDGE ( 'NONE', *, *, #65619, .F. ) ;
#11807=CARTESIAN_POINT ( 'NONE',  ( 87.77058453035330388, 45.11289234403164983, 6.766180878992238412 ) ) ;
#11817=CARTESIAN_POINT ( 'NONE',  ( 37.75683693788968753, 23.92755873383628895, 6.180339887498953466 ) ) ;
#11820=CARTESIAN_POINT ( 'NONE',  ( 81.29242433156768755, 43.25429275065669543, 9.620330362255517187 ) ) ;
#11833=VERTEX_POINT ( 'NONE', #31453 ) ;
#11835=CARTESIAN_POINT ( 'NONE',  ( 82.99898243690306288, 53.45938235784409898, 15.65150354709845004 ) ) ;
#11836=CARTESIAN_POINT ( 'NONE',  ( 19.05068821614582575, 13.12755873383625271, -6.180339887498949025 ) ) ;
#11841=ORIENTED_EDGE ( 'NONE', *, *, #42360, .F. ) ;
#11842=LINE ( 'NONE', #48331, #7574 ) ;
#11843=CARTESIAN_POINT ( 'NONE',  ( 27.77157046966360809, 18.96004757982091249, -5.678558825948276656 ) ) ;
#11844=EDGE_CURVE ( 'NONE', #51674, #29855, #54747, .T. ) ;
#11856=ORIENTED_EDGE ( 'NONE', *, *, #73160, .T. ) ;
#11866=CARTESIAN_POINT ( 'NONE',  ( 84.74456076088121392, 50.48706963223701649, 13.54072923514545757 ) ) ;
#11872=ORIENTED_EDGE ( 'NONE', *, *, #61273, .F. ) ;
#11873=CARTESIAN_POINT ( 'NONE',  ( 74.32474745866193189, 68.52230083288840490, 11.65590001247776364 ) ) ;
#11883=ORIENTED_EDGE ( 'NONE', *, *, #29502, .F. ) ;
#11884=CARTESIAN_POINT ( 'NONE',  ( 79.13444159074371953, 60.15296345131729083, -16.46386276767551848 ) ) ;
#11888=CARTESIAN_POINT ( 'NONE',  ( 68.79203164621388567, 64.70631446037705814, -12.17797522407645516 ) ) ;
#11892=VECTOR ( 'NONE', #75559, 1000.000000000000114 ) ;
#11895=CARTESIAN_POINT ( 'NONE',  ( 68.82480163077127600, 67.66752897612431639, 8.343174400127590928 ) ) ;
#11897=ORIENTED_EDGE ( 'NONE', *, *, #47156, .T. ) ;
#11902=EDGE_CURVE ( 'NONE', #2005, #89249, #12213, .T. ) ;
#11903=CARTESIAN_POINT ( 'NONE',  ( 17.68238808236222326, 31.18502408145591787, 5.678558825948277544 ) ) ;
#11904=FACE_OUTER_BOUND ( 'NONE', #75285, .T. ) ;
#11908=CARTESIAN_POINT ( 'NONE',  ( 82.04105866126801061, 41.84617809604260685, -5.590206233676478398 ) ) ;
#11909=CARTESIAN_POINT ( 'NONE',  ( 74.89568429962641005, 67.14399892254596125, 12.98700472788359228 ) ) ;
#11916=CARTESIAN_POINT ( 'NONE',  ( 81.59284463765364137, 55.17094835597973912, -15.91583639150689855 ) ) ;
#11920=CARTESIAN_POINT ( 'NONE',  ( 86.46048006423905008, 47.32182001325401188, 10.26516935212321968 ) ) ;
#11921=CARTESIAN_POINT ( 'NONE',  ( 80.37872757669391888, 55.97141553226800426, 16.09280928407363831 ) ) ;
#11923=CARTESIAN_POINT ( 'NONE',  ( 72.09555114463066161, 71.52603334931079360, -5.842164467371243397 ) ) ;
#11927=CARTESIAN_POINT ( 'NONE',  ( 4.135592144620554578, 24.16126292948893450, -6.180339887498951690 ) ) ;
#11934=CARTESIAN_POINT ( 'NONE',  ( 79.40659458863603959, 59.69041580281565018, 16.52608132308844091 ) ) ;
#11937=CARTESIAN_POINT ( 'NONE',  ( 75.30072407401860346, 53.34595582841677697, 16.02892702632065891 ) ) ;
#11940=CARTESIAN_POINT ( 'NONE',  ( 80.23640585404207570, 51.30364936960656763, -15.02180247759152643 ) ) ;
#11944=CARTESIAN_POINT ( 'NONE',  ( 88.23407674691928548, 43.71813397101750098, 0.1961470715255514696 ) ) ;
#11945=ORIENTED_EDGE ( 'NONE', *, *, #42377, .T. ) ;
#11946=CARTESIAN_POINT ( 'NONE',  ( 77.55626133878482165, 49.73613333205595666, 14.95107568548285037 ) ) ;
#11948=CARTESIAN_POINT ( 'NONE',  ( 75.90866741198675527, 63.34674660074826846, 14.83779576734563044 ) ) ;
#11952=CARTESIAN_POINT ( 'NONE',  ( 81.92915189185293912, 41.06609442470161042, 3.489617835449585037 ) ) ;
#11958=CARTESIAN_POINT ( 'NONE',  ( 70.81316579118700361, 61.41551742078693366, -14.85192641767512889 ) ) ;
#11959=CARTESIAN_POINT ( 'NONE',  ( 5.869580825389008716, 26.49540643055185996, 3.479690158560446702E-15 ) ) ;
#11966=ADVANCED_FACE ( 'NONE', ( #10178 ), #41045, .T. ) ;
#11967=CARTESIAN_POINT ( 'NONE',  ( 76.14996942406402525, 65.34647919798338478, -14.05451472204274310 ) ) ;
#11972=CARTESIAN_POINT ( 'NONE',  ( 88.16692178265705593, 43.83444978110026824, -2.116868534317887462 ) ) ;
#11975=CARTESIAN_POINT ( 'NONE',  ( 66.44900687915006188, 68.94146508460354994, 0.02989588888337583669 ) ) ;
#11980=VECTOR ( 'NONE', #24118, 1000.000000000000227 ) ;
#11982=CARTESIAN_POINT ( 'NONE',  ( 78.44203751522360335, 61.21016990572091032, 16.24725970467587999 ) ) ;
#11986=CARTESIAN_POINT ( 'NONE',  ( 88.18856786306730555, 43.91052089632134425, 2.508363019901196367 ) ) ;
#11990=CARTESIAN_POINT ( 'NONE',  ( 75.82478874696548132, 61.23931674123156199, -15.47528407149140861 ) ) ;
#11996=CARTESIAN_POINT ( 'NONE',  ( 80.64679548305885248, 43.26720623737277549, -9.272004999721030316 ) ) ;
#12000=CARTESIAN_POINT ( 'NONE',  ( 87.77744914111154628, 44.40955816724378025, -3.958690154376787174 ) ) ;
#12004=B_SPLINE_CURVE_WITH_KNOTS ( 'NONE', 3,
 ( #28120, #81377, #4845, #81865, #44308, #58994, #51420, #82382, #5820, #36709, #67616, #98544, #11944, #50242, #65444, #56337, #42138, #58334, #64453, #89310, #73070, #72580 ),
 .UNSPECIFIED., .F., .F.,
 ( 4, 3, 3, 3, 3, 3, 3, 4 ),
 ( 0.4976065956401893864, 0.5844252810809384968, 0.6686540514502724575, 0.7354980260655605839, 0.8028463152565796790, 0.8633854507757419139, 0.9437142632667596676, 1.000000000000000000 ),
 .UNSPECIFIED. ) ;
#12008=CARTESIAN_POINT ( 'NONE',  ( 84.74507488503365948, 50.24295689512916141, 13.81875560728438224 ) ) ;
#12011=CARTESIAN_POINT ( 'NONE',  ( 76.44488007030824406, 54.92415880672584194, -16.57738246812632354 ) ) ;
#12023=CARTESIAN_POINT ( 'NONE',  ( 36.24660459446915439, 29.43085787977765833, -9.188101187500008038 ) ) ;
#12027=CARTESIAN_POINT ( 'NONE',  ( 26.89353023359722883, 24.03085787977764198, 9.188101187500006262 ) ) ;
#12036=CARTESIAN_POINT ( 'NONE',  ( 74.76373281376733360, 64.18679306110026062, 14.63261176689765364 ) ) ;
#12040=CARTESIAN_POINT ( 'NONE',  ( 75.25301932441034580, 53.09737962384632937, 16.48714817978221348 ) ) ;
#12043=ORIENTED_EDGE ( 'NONE', *, *, #34396, .T. ) ;
#12045=CARTESIAN_POINT ( 'NONE',  ( 85.12278939449318216, 42.79832675737401360, 3.312954136966923535 ) ) ;
#12051=CARTESIAN_POINT ( 'NONE',  ( 8.399671500380161859, 16.80066082961419482, 10.00000000000000533 ) ) ;
#12052=LINE ( 'NONE', #26250, #16994 ) ;
#12053=CARTESIAN_POINT ( 'NONE',  ( 87.98904372666932261, 44.25610683789894750, -4.385737539232398063 ) ) ;
#12055=CARTESIAN_POINT ( 'NONE',  ( 26.79248755578709762, 33.65586893147757763, -7.433330006724137462 ) ) ;
#12061=CARTESIAN_POINT ( 'NONE',  ( 87.23690874686347740, 46.15778144619924461, -8.941654336830676897 ) ) ;
#12064=CARTESIAN_POINT ( 'NONE',  ( 85.65483554831503454, 48.88356815160276625, -12.11013705813561181 ) ) ;
#12065=CARTESIAN_POINT ( 'NONE',  ( 66.18256082828796139, 68.61784451530441231, -2.171160931695417684 ) ) ;
#12078=CARTESIAN_POINT ( 'NONE',  ( 86.99754070748903700, 45.91539075293407990, -8.140839447248088945 ) ) ;
#12081=CARTESIAN_POINT ( 'NONE',  ( 10.74796456262465050, 21.90829794293879473, 10.00000000000000355 ) ) ;
#12090=CARTESIAN_POINT ( 'NONE',  ( 66.17343954913512505, 68.52301864461630032, -2.711686016849372827 ) ) ;
#12096=CARTESIAN_POINT ( 'NONE',  ( 86.25114834473923509, 43.91001722141434271, -4.889282600613897856 ) ) ;
#12102=DIRECTION ( 'NONE',  ( 0.9133924323370964382, -0.1624253398589829422, -0.3732723851572960494 ) ) ;
#12105=CARTESIAN_POINT ( 'NONE',  ( 82.49322465416763350, 40.88878199599866292, -3.716918875651960441 ) ) ;
#12107=CARTESIAN_POINT ( 'NONE',  ( 80.13153417293931113, 50.66350872248114001, 14.80289417267747965 ) ) ;
#12110=CARTESIAN_POINT ( 'NONE',  ( 77.80736617348490824, 61.72758938687779562, 16.06622420362090153 ) ) ;
#12114=CARTESIAN_POINT ( 'NONE',  ( 69.77890858254123430, 70.63368750135978757, -2.958018195249015658 ) ) ;
#12117=CARTESIAN_POINT ( 'NONE',  ( 42.39820071321547346, 24.28848085856235173, 1.475505719884397138E-15 ) ) ;
#12120=CARTESIAN_POINT ( 'NONE',  ( 81.15576878495137692, 43.19889211345415703, -8.824872785026526500 ) ) ;
#12122=EDGE_CURVE ( 'NONE', #23117, #54050, #15575, .T. ) ;
#12124=CARTESIAN_POINT ( 'NONE',  ( 68.29064676983747972, 69.02907622317006542, 6.494102608087607642 ) ) ;
#12127=CARTESIAN_POINT ( 'NONE',  ( 87.22595043061240005, 46.05622627631750987, 8.811080105847633348 ) ) ;
#12130=CARTESIAN_POINT ( 'NONE',  ( 71.67936538144843439, 72.44724869688445779, -1.358217801655851931 ) ) ;
#12136=CARTESIAN_POINT ( 'NONE',  ( 3.825981621811214151, 23.18502408145589300, 5.678558825948277544 ) ) ;
#12141=EDGE_CURVE ( 'NONE', #25763, #22997, #42004, .T. ) ;
#12143=EDGE_CURVE ( 'NONE', #44579, #83882, #10966, .T. ) ;
#12145=CARTESIAN_POINT ( 'NONE',  ( 74.01413570136905662, 57.15554519978635994, -15.99517262605232659 ) ) ;
#12151=EDGE_LOOP ( 'NONE', ( #35328, #93972, #81868, #47918 ) ) ;
#12155=VERTEX_POINT ( 'NONE', #69292 ) ;
#12159=CARTESIAN_POINT ( 'NONE',  ( 36.80649086932150027, 23.11110640527294535, -2.839279412974138328 ) ) ;
#12160=CARTESIAN_POINT ( 'NONE',  ( 73.04656796621824810, 70.72172819928655940, -7.591179416118629675 ) ) ;
#12164=CARTESIAN_POINT ( 'NONE',  ( 19.48598279363274344, 13.11110640527291693, -2.839279412974138328 ) ) ;
#12165=CARTESIAN_POINT ( 'NONE',  ( 68.70248306966885821, 64.25130556195607312, 12.49291083475091746 ) ) ;
#12168=ORIENTED_EDGE ( 'NONE', *, *, #49617, .T. ) ;
#12179=CARTESIAN_POINT ( 'NONE',  ( 66.07625507003409382, 68.50412252646739830, -2.501755903184967433 ) ) ;
#12182=CARTESIAN_POINT ( 'NONE',  ( 78.34332907769417886, 61.12495998885079018, -15.90539878443391864 ) ) ;
#12193=CARTESIAN_POINT ( 'NONE',  ( 35.31080938399455249, 26.10170272979929607, -7.433330006724141015 ) ) ;
#12195=CARTESIAN_POINT ( 'NONE',  ( 75.31302016003080269, 66.58151914953994321, -13.09053389059541139 ) ) ;
#12203=CARTESIAN_POINT ( 'NONE',  ( 70.10178725980775027, 64.18715254517744029, -12.51786991059252685 ) ) ;
#12205=CARTESIAN_POINT ( 'NONE',  ( 86.19918046091518704, 42.54196271365974980, 0.6765657524371224696 ) ) ;
#12213=B_SPLINE_CURVE_WITH_KNOTS ( 'NONE', 3,
 ( #86725, #39043, #78080, #7668, #22863, #1075, #85734, #8173, #16263, #15753, #69954, #38045, #46659, #68959, #99881, #77060 ),
 .UNSPECIFIED., .F., .F.,
 ( 4, 1, 2, 2, 2, 1, 2, 2, 4 ),
 ( 0.000000000000000000, 0.1250000000000006661, 0.1875000000000009714, 0.2500000000000012768, 0.5000000000000007772, 0.6250000000000001110, 0.6875000000000006661, 0.7500000000000012212, 1.000000000000000000 ),
 .UNSPECIFIED. ) ;
#12228=CARTESIAN_POINT ( 'NONE',  ( 75.48702785388739755, 65.17841116432670390, 13.95333018839138006 ) ) ;
#12238=CARTESIAN_POINT ( 'NONE',  ( 68.34215885236082499, 69.21295319673539836, 4.808519653334967892 ) ) ;
#12242=CARTESIAN_POINT ( 'NONE',  ( 23.34564182995783455, 13.28848085856231442, 1.475505719884397138E-15 ) ) ;
#12244=CARTESIAN_POINT ( 'NONE',  ( 81.84662774497913063, 41.65891706340769218, 5.409804292327541120 ) ) ;
#12251=LINE ( 'NONE', #65929, #20817 ) ;
#12257=CARTESIAN_POINT ( 'NONE',  ( 83.55156767614275282, 41.73934938018408047, 4.529189728718444385 ) ) ;
#12258=CARTESIAN_POINT ( 'NONE',  ( 24.48230016887698568, 13.94473085651392452, 1.475505719884397138E-15 ) ) ;
#12259=CARTESIAN_POINT ( 'NONE',  ( 85.85757975920050455, 48.54684933318403495, 12.22929488966399880 ) ) ;
#12263=CARTESIAN_POINT ( 'NONE',  ( 74.09797824419197809, 55.64112326900559680, -16.58847249929255341 ) ) ;
#12266=ADVANCED_FACE ( 'NONE', ( #13013 ), #52472, .T. ) ;
#12276=CARTESIAN_POINT ( 'NONE',  ( 35.16646543599519248, 35.70171378149922248, -9.188101187500004485 ) ) ;
#12277=CARTESIAN_POINT ( 'NONE',  ( 20.54487693938818538, 27.56454794089042082, 10.00000000000000355 ) ) ;
#12283=EDGE_CURVE ( 'NONE', #2731, #63769, #21110, .T. ) ;
#12284=CARTESIAN_POINT ( 'NONE',  ( 16.32921660555538423, 21.37878583063840310, 9.188101187500006262 ) ) ;
#12285=CARTESIAN_POINT ( 'NONE',  ( 71.76139268086218692, 72.52520824035063640, 0.9833505332507315178 ) ) ;
#12286=CARTESIAN_POINT ( 'NONE',  ( 82.42561518943209364, 53.83419803862933861, 15.85509184085860745 ) ) ;
#12291=CARTESIAN_POINT ( 'NONE',  ( 18.51072855673551487, 34.18528772668518201, -1.583844403245363575 ) ) ;
#12292=CARTESIAN_POINT ( 'NONE',  ( 74.94754896363279784, 53.48443655244039263, -16.53883777380878684 ) ) ;
#12297=CARTESIAN_POINT ( 'NONE',  ( 68.70570789778643928, 70.27148567445367178, -0.5708798829847213652 ) ) ;
#12299=CARTESIAN_POINT ( 'NONE',  ( 66.43537002243755296, 68.65414004482329347, 4.832212937122434049 ) ) ;
#12300=CARTESIAN_POINT ( 'NONE',  ( 87.10115137904760729, 45.28340438443852634, 6.995308688534726649 ) ) ;
#12307=CARTESIAN_POINT ( 'NONE',  ( 80.53198101875031512, 57.77087603849956565, 16.24514743536724026 ) ) ;
#12310=CARTESIAN_POINT ( 'NONE',  ( 87.65912690667771301, 45.19743498868427167, -6.201137598350706881 ) ) ;
#12315=CARTESIAN_POINT ( 'NONE',  ( 73.65586519493432149, 59.54601760613143568, 15.54039508984885565 ) ) ;
#12320=CARTESIAN_POINT ( 'NONE',  ( 75.25170673533752108, 66.73598490943447814, 12.94887977284632896 ) ) ;
#12321=VECTOR ( 'NONE', #60423, 1000.000000000000114 ) ;
#12326=LINE ( 'NONE', #71643, #64218 ) ;
#12334=CARTESIAN_POINT ( 'NONE',  ( 80.48057461997055384, 55.60742216994913889, -16.06452287015007840 ) ) ;
#12369=CARTESIAN_POINT ( 'NONE',  ( 74.45055738859878147, 68.30939989315471905, -11.41140116448488051 ) ) ;
#12370=CARTESIAN_POINT ( 'NONE',  ( 74.23286061265172009, 64.97622957471450889, 14.08197172241813888 ) ) ;
#12375=CARTESIAN_POINT ( 'NONE',  ( 67.00187114335926708, 67.08813303282481399, 8.529924657355552498 ) ) ;
#12378=ORIENTED_EDGE ( 'NONE', *, *, #15660, .T. ) ;
#12388=CARTESIAN_POINT ( 'NONE',  ( 71.72631157091053922, 72.05082354862287275, -1.633393872038913175 ) ) ;
#12391=CARTESIAN_POINT ( 'NONE',  ( 72.52093223241688236, 57.39944909060013600, 16.31544603362117485 ) ) ;
#12392=CARTESIAN_POINT ( 'NONE',  ( 69.57879208480075306, 68.94139417373898482, 7.052474478442530170 ) ) ;
#12396=CARTESIAN_POINT ( 'NONE',  ( 82.28662647995521695, 41.83953847820645677, 6.586483578078058621 ) ) ;
#12398=CARTESIAN_POINT ( 'NONE',  ( 18.31869600479030424, 33.68290643055186706, 3.479690158560446702E-15 ) ) ;
#12404=CARTESIAN_POINT ( 'NONE',  ( 11.67130034620459256, 30.23654200823201776, 1.583844403245363353 ) ) ;
#12409=CARTESIAN_POINT ( 'NONE',  ( 82.12550757349835351, 41.17588303117550907, -3.464665208087097437 ) ) ;
#12413=CARTESIAN_POINT ( 'NONE',  ( 68.69386498186378276, 66.37052439002927429, 9.851853166250990057 ) ) ;
#12415=CARTESIAN_POINT ( 'NONE',  ( 71.88106639363309114, 72.58558382077731608, 1.103795272596851174 ) ) ;
#12416=CARTESIAN_POINT ( 'NONE',  ( 83.70208412440790369, 42.60878222363336931, 5.172964853322376655 ) ) ;
#12421=CARTESIAN_POINT ( 'NONE',  ( 10.37514450368026786, 11.15404122711131407, 8.090169943749479842 ) ) ;
#12422=LINE ( 'NONE', #75219, #44874 ) ;
#12439=CARTESIAN_POINT ( 'NONE',  ( 81.45273407654831033, 41.92911449342699370, -7.602784365630077978 ) ) ;
#12445=CARTESIAN_POINT ( 'NONE',  ( 76.90683638624993534, 49.81317808655190049, 15.10818565773490008 ) ) ;
#12447=CARTESIAN_POINT ( 'NONE',  ( 75.95776633494669738, 63.62874501809822902, 14.74263889421621698 ) ) ;
#12451=CARTESIAN_POINT ( 'NONE',  ( 82.18687726816486361, 41.15680977039290411, 3.242629060634906857 ) ) ;
#12454=CYLINDRICAL_SURFACE ( 'NONE', #56583, 10.00000000000001066 ) ;
#12455=CARTESIAN_POINT ( 'NONE',  ( 22.27692774695706035, 28.56454794089042082, 10.00000000000000355 ) ) ;
#12460=CARTESIAN_POINT ( 'NONE',  ( 12.55777956335723644, 9.111106405272902720, -2.839279412974138328 ) ) ;
#12468=CARTESIAN_POINT ( 'NONE',  ( 76.24546156567440391, 64.85285070271640961, -14.33378511211777706 ) ) ;
#12474=CARTESIAN_POINT ( 'NONE',  ( 84.31620252596033538, 42.01387254285906891, 1.014253996708007088 ) ) ;
#12478=CARTESIAN_POINT ( 'NONE',  ( 65.98821791718346219, 68.67660198893013046, -0.1386984857929180193 ) ) ;
#12479=ORIENTED_EDGE ( 'NONE', *, *, #17236, .F. ) ;
#12485=CARTESIAN_POINT ( 'NONE',  ( 81.40384678758614712, 44.82616229828595777, -10.53103118534553850 ) ) ;
#12487=CARTESIAN_POINT ( 'NONE',  ( 1.396987757676521058, 24.30466486950695071, 1.224646799147354045E-15 ) ) ;
#12488=CARTESIAN_POINT ( 'NONE',  ( 88.42823867725131493, 44.01048851461693090, 2.280060627005664919 ) ) ;
#12491=ORIENTED_EDGE ( 'NONE', *, *, #38803, .F. ) ;
#12493=CARTESIAN_POINT ( 'NONE',  ( 80.17588645533830061, 58.12694466101720536, 16.26593623338475680 ) ) ;
#12494=CARTESIAN_POINT ( 'NONE',  ( 85.73351810911900373, 48.76173041439603395, -12.45270611261531180 ) ) ;
#12497=CARTESIAN_POINT ( 'NONE',  ( 81.03047946496111820, 43.68561371680597460, -9.505511175303684723 ) ) ;
#12501=CARTESIAN_POINT ( 'NONE',  ( 87.84569706029115821, 44.18597558567909545, -4.425511980624551533 ) ) ;
#12503=CARTESIAN_POINT ( 'NONE',  ( 78.42722165381930211, 53.22649076314601047, 15.78604470347753264 ) ) ;
#12504=CARTESIAN_POINT ( 'NONE',  ( 75.92491905781218975, 51.44142931567759547, 15.68752148852608741 ) ) ;
#12508=CARTESIAN_POINT ( 'NONE',  ( 84.17379491356786048, 50.54589666422514682, 13.76883155557667138 ) ) ;
#12515=CARTESIAN_POINT ( 'NONE',  ( 10.26584248093601737, 14.43085787977761036, -9.188101187500008038 ) ) ;
#12519=CARTESIAN_POINT ( 'NONE',  ( 86.30629612394095318, 43.10717986221388998, -0.8733839489286622237 ) ) ;
#12524=CARTESIAN_POINT ( 'NONE',  ( 32.31339950491288704, 36.84336893147758474, -7.433330006724137462 ) ) ;
#12527=CARTESIAN_POINT ( 'NONE',  ( 25.24326406500046360, 20.28920272979927475, -7.433330006724141015 ) ) ;
#12529=CARTESIAN_POINT ( 'NONE',  ( 7.350711452622367581, 26.01751292744054567, 6.180339887498949913 ) ) ;
#12532=CARTESIAN_POINT ( 'NONE',  ( 70.99214533039287289, 61.07251846123117645, 14.51118677859261119 ) ) ;
#12538=CARTESIAN_POINT ( 'NONE',  ( 75.32443696912777398, 53.39185654545678972, 16.03229517472230370 ) ) ;
#12545=CARTESIAN_POINT ( 'NONE',  ( 83.77213608728635563, 41.72335732820068444, 1.354266426187002992 ) ) ;
#12546=ADVANCED_FACE ( 'NONE', ( #47362 ), #1664, .T. ) ;
#12549=ORIENTED_EDGE ( 'NONE', *, *, #48077, .F. ) ;
#12550=CARTESIAN_POINT ( 'NONE',  ( 72.01291228344958029, 71.60916324447191528, 5.531298035833710713 ) ) ;
#12556=CARTESIAN_POINT ( 'NONE',  ( 26.01788259378743362, 35.99752408145593563, 5.678558825948276656 ) ) ;
#12557=CARTESIAN_POINT ( 'NONE',  ( 74.51118135615443805, 60.14921420329969948, -15.52886586986496376 ) ) ;
#12564=CARTESIAN_POINT ( 'NONE',  ( 68.10490905690869567, 65.76241361189985923, 10.87691428392215620 ) ) ;
#12566=CARTESIAN_POINT ( 'NONE',  ( 85.71893696364587356, 48.44430998916941178, -11.74445541149036742 ) ) ;
#12569=CARTESIAN_POINT ( 'NONE',  ( 82.08088010363431408, 40.77644816011592610, 1.343812065088729302 ) ) ;
#12579=ORIENTED_EDGE ( 'NONE', *, *, #87804, .F. ) ;
#12583=CARTESIAN_POINT ( 'NONE',  ( 86.94972120171313179, 45.89256597715363739, -8.147647120779746288 ) ) ;
#12584=ADVANCED_FACE ( 'NONE', ( #10385 ), #86642, .T. ) ;
#12591=EDGE_LOOP ( 'NONE', ( #89873, #86239, #13935, #47455 ) ) ;
#12600=CARTESIAN_POINT ( 'NONE',  ( 82.08766997739726889, 44.26091490527264938, 9.509083040982000412 ) ) ;
#12605=VECTOR ( 'NONE', #7316, 1000.000000000000000 ) ;
#12608=CARTESIAN_POINT ( 'NONE',  ( 26.55243232390424879, 15.73415679381822585, 1.333680081654574804E-15 ) ) ;
#12613=CARTESIAN_POINT ( 'NONE',  ( 76.45572749640669485, 51.64231386250387601, -16.15369532800221108 ) ) ;
#12615=LINE ( 'NONE', #82548, #38124 ) ;
#12616=CARTESIAN_POINT ( 'NONE',  ( 78.90549422596571105, 46.47045305960070039, 12.99985401326298984 ) ) ;
#12623=CARTESIAN_POINT ( 'NONE',  ( 68.23939761155092754, 69.98628890222548193, -0.9983377936462706215 ) ) ;
#12625=CARTESIAN_POINT ( 'NONE',  ( 78.14015596324891533, 47.79605781560270117, 14.53813849190288465 ) ) ;
#12626=CARTESIAN_POINT ( 'NONE',  ( 38.08795742478228163, 27.15404122711136381, 8.090169943749479842 ) ) ;
#12627=CARTESIAN_POINT ( 'NONE',  ( 80.33315281163550026, 55.86497812776784855, -16.47487610438770034 ) ) ;
#12629=CARTESIAN_POINT ( 'NONE',  ( 82.28582548923134254, 54.25481651909717584, 15.63115421305295527 ) ) ;
#12635=AXIS2_PLACEMENT_3D ( 'NONE', #96526, #28072, #27096 ) ;
#12636=CARTESIAN_POINT ( 'NONE',  ( 87.04534585051717954, 46.05262481000475105, 8.948764308993935046 ) ) ;
#12638=CARTESIAN_POINT ( 'NONE',  ( 71.49023828022640714, 72.34911387847559183, -1.236132173619994168 ) ) ;
#12645=CARTESIAN_POINT ( 'NONE',  ( 7.993722094130166766, 16.56628583063838533, 9.188101187500006262 ) ) ;
#12651=CARTESIAN_POINT ( 'NONE',  ( 68.05640523449149271, 67.83844799063044206, -7.344562446520097154 ) ) ;
#12654=CARTESIAN_POINT ( 'NONE',  ( 81.90096821949344985, 41.09411741666988149, 3.667264625812675316 ) ) ;
#12655=AXIS2_PLACEMENT_3D ( 'NONE', #8793, #93936, #84339 ) ;
#12657=CARTESIAN_POINT ( 'NONE',  ( 75.45929019331548204, 53.24617608301296201, 16.49036319738879897 ) ) ;
#12661=ORIENTED_EDGE ( 'NONE', *, *, #19172, .F. ) ;
#12665=CARTESIAN_POINT ( 'NONE',  ( 67.43033157395939270, 67.25313052952390080, -8.647980512837968092 ) ) ;
#12670=CARTESIAN_POINT ( 'NONE',  ( 27.40352323984253502, 36.79752408145593279, -5.678558825948271327 ) ) ;
#12674=EDGE_LOOP ( 'NONE', ( #56646, #1607, #10308, #6173 ) ) ;
#12675=CARTESIAN_POINT ( 'NONE',  ( 12.93608109523609073, 25.65586893147755276, -7.433330006724137462 ) ) ;
#12676=CARTESIAN_POINT ( 'NONE',  ( 30.57965140047823738, 19.78380873178787880, -6.180339887498949025 ) ) ;
#12679=EDGE_CURVE ( 'NONE', #85413, #9557, #2545, .T. ) ;
#12686=EDGE_LOOP ( 'NONE', ( #97066, #34494, #3005, #18329 ) ) ;
#12691=VERTEX_POINT ( 'NONE', #1033 ) ;
#12692=CARTESIAN_POINT ( 'NONE',  ( 66.53067542137131340, 68.81138069514842925, -2.220520527782671838 ) ) ;
#12694=CARTESIAN_POINT ( 'NONE',  ( 81.86683804372771078, 55.45883585039843666, 16.28524382593451136 ) ) ;
#12695=CARTESIAN_POINT ( 'NONE',  ( 78.18406947592188772, 61.66846224198985027, -16.12704840749690050 ) ) ;
#12702=EDGE_LOOP ( 'NONE', ( #62731, #572, #9434, #74564 ) ) ;
#12703=EDGE_CURVE ( 'NONE', #77668, #20229, #23240, .T. ) ;
#12711=CARTESIAN_POINT ( 'NONE',  ( 87.74082335983182190, 45.11567895962654973, 6.804767787324432327 ) ) ;
#12712=EDGE_LOOP ( 'NONE', ( #28042, #21080, #9687, #66885 ) ) ;
#12714=CARTESIAN_POINT ( 'NONE',  ( 66.43194084327845417, 68.18590565871475917, 4.517642387139569671 ) ) ;
#12715=CARTESIAN_POINT ( 'NONE',  ( 87.29803824456323014, 43.36679595344801896, 2.358950023001834317 ) ) ;
#12724=VECTOR ( 'NONE', #10072, 1000.000000000000114 ) ;
#12729=AXIS2_PLACEMENT_3D ( 'NONE', #53275, #23360, #62865 ) ;
#12733=CARTESIAN_POINT ( 'NONE',  ( 80.84437787308391421, 44.34192801377794524, -10.37496191005612900 ) ) ;
#12734=CARTESIAN_POINT ( 'NONE',  ( 73.85816664754916872, 67.07998314229074310, -12.61123796580315570 ) ) ;
#12737=CARTESIAN_POINT ( 'NONE',  ( 74.66991520905840218, 60.53581785384168512, 15.47673426609052960 ) ) ;
#12740=CARTESIAN_POINT ( 'NONE',  ( 77.49042508736837931, 60.78651308045809998, 15.85568622532634819 ) ) ;
#12743=CARTESIAN_POINT ( 'NONE',  ( 72.56743321539229896, 71.30517223960133322, -6.002003212711099600 ) ) ;
#12745=CARTESIAN_POINT ( 'NONE',  ( 73.64963185817160252, 69.30855129028742567, -9.977530012273353677 ) ) ;
#12752=CARTESIAN_POINT ( 'NONE',  ( 14.02357142238433063, 26.83478043621387243, -8.090169943749479842 ) ) ;
#12755=CARTESIAN_POINT ( 'NONE',  ( 15.68640692011977222, 32.55466486950700045, -1.111400068045478839E-16 ) ) ;
#12757=CARTESIAN_POINT ( 'NONE',  ( 72.21898876619836471, 72.04774665458343463, -3.189688383038575381 ) ) ;
#12760=ORIENTED_EDGE ( 'NONE', *, *, #84398, .F. ) ;
#12765=CARTESIAN_POINT ( 'NONE',  ( 82.66777534753497036, 40.88273136530058594, 3.288167606880417981 ) ) ;
#12766=CARTESIAN_POINT ( 'NONE',  ( 29.67845259158361415, 16.94473085651393163, 1.475505719884397138E-15 ) ) ;
#12767=CARTESIAN_POINT ( 'NONE',  ( 85.48805828002734586, 48.64268271054365300, 12.46980397201070900 ) ) ;
#12783=CARTESIAN_POINT ( 'NONE',  ( 34.04545031248176912, 37.84336893147759184, -7.433330006724137462 ) ) ;
#12786=VECTOR ( 'NONE', #17473, 1000.000000000000114 ) ;
#12791=AXIS2_PLACEMENT_3D ( 'NONE', #53570, #68277, #60162 ) ;
#12792=CARTESIAN_POINT ( 'NONE',  ( 16.86928618479236164, 18.24335787977762990, -9.188101187500008038 ) ) ;
#12793=CARTESIAN_POINT ( 'NONE',  ( 71.71444459471547361, 72.49928141732986830, 0.9658765412761121105 ) ) ;
#12794=CARTESIAN_POINT ( 'NONE',  ( 82.40504737207831454, 54.25064673307860375, 15.61126503404915233 ) ) ;
#12799=CARTESIAN_POINT ( 'NONE',  ( 18.71323094475359738, 33.73705186507753950, -3.090169943749475845 ) ) ;
#12801=EDGE_CURVE ( 'NONE', #50534, #98353, #57569, .T. ) ;
#12802=ORIENTED_EDGE ( 'NONE', *, *, #72641, .F. ) ;
#12809=ORIENTED_EDGE ( 'NONE', *, *, #62765, .T. ) ;
#12816=CARTESIAN_POINT ( 'NONE',  ( 88.41107184461979784, 44.00353577411875960, -2.298891457252526749 ) ) ;
#12817=CARTESIAN_POINT ( 'NONE',  ( 80.56456852273207403, 57.68474611512090178, 16.59351620786970827 ) ) ;
#12820=CARTESIAN_POINT ( 'NONE',  ( 87.60616923137877166, 45.13511946215697890, -6.138091206483382578 ) ) ;
#12821=CARTESIAN_POINT ( 'NONE',  ( 88.49445028879968334, 43.86712364161932243, -9.307608808691473302E-08 ) ) ;
#12822=CARTESIAN_POINT ( 'NONE',  ( 80.67567036563099236, 43.43790138286748714, 9.454380761424062030 ) ) ;
#12825=CARTESIAN_POINT ( 'NONE',  ( 74.01533384933624404, 61.07494375654813723, 15.18702621176734446 ) ) ;
#12827=EDGE_LOOP ( 'NONE', ( #11661, #76386, #17974, #34984 ) ) ;
#12839=CARTESIAN_POINT ( 'NONE',  ( 83.01487341893997041, 53.35419878647658720, 15.61608225115200810 ) ) ;
#12853=CARTESIAN_POINT ( 'NONE',  ( 70.92937966038938669, 67.01461546877725084, 10.61286113055345304 ) ) ;
#12855=CARTESIAN_POINT ( 'NONE',  ( 83.91622664933946396, 41.67106969241695680, 3.569253368665360249 ) ) ;
#12856=FACE_OUTER_BOUND ( 'NONE', #93709, .T. ) ;
#12861=CARTESIAN_POINT ( 'NONE',  ( 85.76883949360097859, 47.60599329228222842, 11.49143109850623823 ) ) ;
#12867=AXIS2_PLACEMENT_3D ( 'NONE', #76068, #99355, #78429 ) ;
#12872=CARTESIAN_POINT ( 'NONE',  ( 82.62131884904979984, 40.84117856601688601, 3.225010313909428383 ) ) ;
#12876=CARTESIAN_POINT ( 'NONE',  ( 73.01042618992920552, 69.46801108043791828, 9.349659332454741900 ) ) ;
#12880=FACE_OUTER_BOUND ( 'NONE', #50551, .T. ) ;
#12892=B_SPLINE_CURVE_WITH_KNOTS ( 'NONE', 3,
 ( #51999, #98625, #83936, #44878, #29206, #4919, #60571, #52988, #82463, #52485 ),
 .UNSPECIFIED., .F., .F.,
 ( 4, 2, 2, 2, 4 ),
 ( 0.000000000000000000, 0.0002622400424273360143, 0.0005244800848546720285, 0.0007867201272820080428, 0.001048960169709344057 ),
 .UNSPECIFIED. ) ;
#12893=CARTESIAN_POINT ( 'NONE',  ( 7.727700963378506316, 20.16454794089039382, -10.00000000000000355 ) ) ;
#12895=CARTESIAN_POINT ( 'NONE',  ( 71.69771586823793541, 58.77412815006911728, -15.43371067787085416 ) ) ;
#12896=CARTESIAN_POINT ( 'NONE',  ( 73.62250635243425734, 69.55784274833358438, 10.23584637956793131 ) ) ;
#12900=CARTESIAN_POINT ( 'NONE',  ( 71.44251307236943660, 71.49647877896676107, 3.603793749803205770 ) ) ;
#12902=VERTEX_POINT ( 'NONE', #26333 ) ;
#12906=CARTESIAN_POINT ( 'NONE',  ( 29.91980124543643171, 22.98920272979927759, 7.433330006724137462 ) ) ;
#12908=CARTESIAN_POINT ( 'NONE',  ( 83.52018940653934465, 51.62319858702418429, -14.86581989589152819 ) ) ;
#12913=VERTEX_POINT ( 'NONE', #72953 ) ;
#12917=DIRECTION ( 'NONE',  ( -0.8660254037844379305, -0.5000000000000014433, -0.000000000000000000 ) ) ;
#12920=CARTESIAN_POINT ( 'NONE',  ( 70.70503195363177440, 69.91188268790216398, 6.471540178100598339 ) ) ;
#12923=CARTESIAN_POINT ( 'NONE',  ( 84.39397012298853440, 43.45927479173952435, 6.252015531843233553 ) ) ;
#12927=CARTESIAN_POINT ( 'NONE',  ( 68.07503851180729271, 69.33559177987039845, 4.005160369666961984 ) ) ;
#12929=( BOUNDED_CURVE ( )  B_SPLINE_CURVE ( 2, ( #92292, #46120, #84685, #29945, #70441, #92777, #30941, #14746, #62323, #77561, #84200, #61827, #23832 ),
 .UNSPECIFIED., .F., .T. ) 
 B_SPLINE_CURVE_WITH_KNOTS ( ( 3, 2, 2, 2, 2, 2, 3 ),
 ( 0.7375000000000000444, 0.7399999999999999911, 0.7449999999999999956, 0.7500000000000000000, 0.7550000000000000044, 0.7600000000000000089, 0.7625000000000000666 ),
 .UNSPECIFIED. ) 
 CURVE ( )  GEOMETRIC_REPRESENTATION_ITEM ( )  RATIONAL_B_SPLINE_CURVE ( ( 0.9755282581475767101, 0.9755282581475772652, 1.000000000000000000, 0.9510565162951535312, 1.000000000000000000, 0.9510565162951535312, 1.000000000000000000, 0.9510565162951535312, 1.000000000000000000, 0.9510565162951535312, 1.000000000000000000, 0.9755282581475761550, 0.9755282581475767101 ) ) 
 REPRESENTATION_ITEM ( '' )  );
#12931=CARTESIAN_POINT ( 'NONE',  ( 15.05724179552094277, 20.64441083166259716, -10.00000000000000533 ) ) ;
#12936=CARTESIAN_POINT ( 'NONE',  ( 86.50330892798304205, 47.09883604031134752, -10.56546389670382169 ) ) ;
#12953=CARTESIAN_POINT ( 'NONE',  ( 80.88463073246907697, 48.08410267114198433, 13.33332236086108580 ) ) ;
#12964=CARTESIAN_POINT ( 'NONE',  ( 72.26211198664731228, 68.26187575085410231, -10.17965940589137830 ) ) ;
#12967=CARTESIAN_POINT ( 'NONE',  ( 76.78200948252425917, 60.31104682374800774, 15.82330234246767731 ) ) ;
#12968=CARTESIAN_POINT ( 'NONE',  ( 12.27453364332850505, 12.80170272979924739, 7.433330006724137462 ) ) ;
#12985=CARTESIAN_POINT ( 'NONE',  ( 66.04689650495228648, 69.25707841837410683, 0.2683665952402904398 ) ) ;
#12994=CARTESIAN_POINT ( 'NONE',  ( 87.85678018468817640, 44.16677905111681923, 2.775409157791113746 ) ) ;
#13000=CARTESIAN_POINT ( 'NONE',  ( 85.70478682239833290, 48.82600918481677610, -12.04570940814934410 ) ) ;
#13003=CARTESIAN_POINT ( 'NONE',  ( 84.75487950562418860, 47.73074732454571745, 11.57677916824878750 ) ) ;
#13010=CARTESIAN_POINT ( 'NONE',  ( 78.93634411335234802, 55.84994475496723254, 16.12935936599136966 ) ) ;
#13013=FACE_OUTER_BOUND ( 'NONE', #72216, .T. ) ;
#13016=CARTESIAN_POINT ( 'NONE',  ( 84.15878383405946295, 50.51712059312899328, 13.75732096714377128 ) ) ;
#13024=CARTESIAN_POINT ( 'NONE',  ( 6.852252633650415703, 22.14336893147753571, 7.433330006724141015 ) ) ;
#13028=CARTESIAN_POINT ( 'NONE',  ( 82.95114570043003255, 42.01829743365728831, -4.711341735647942564 ) ) ;
#13032=CARTESIAN_POINT ( 'NONE',  ( 34.04545031248176912, 37.84336893147759184, -7.433330006724137462 ) ) ;
#13034=CARTESIAN_POINT ( 'NONE',  ( 86.46048006423905008, 47.32182001325401188, 10.26516935212321968 ) ) ;
#13035=EDGE_LOOP ( 'NONE', ( #31391, #18954, #69585, #96311 ) ) ;
#13036=CARTESIAN_POINT ( 'NONE',  ( 17.33597792084844258, 30.98502408145592213, -5.678558825948271327 ) ) ;
#13037=CARTESIAN_POINT ( 'NONE',  ( 6.762080372528353145, 26.83705186507751961, 3.090169943749475401 ) ) ;
#13042=CARTESIAN_POINT ( 'NONE',  ( 70.99702552970684621, 61.08644655966345738, 14.50662264333758955 ) ) ;
#13048=CARTESIAN_POINT ( 'NONE',  ( 88.30335668473479416, 44.31564768512615160, -2.101522154600196757 ) ) ;
#13053=CARTESIAN_POINT ( 'NONE',  ( 84.60109600385015938, 42.34421550614859342, 2.521655685731596819 ) ) ;
#13061=CARTESIAN_POINT ( 'NONE',  ( 88.19817206715259772, 44.49282453600611831, -4.737833512016792703 ) ) ;
#13064=CARTESIAN_POINT ( 'NONE',  ( 34.84170590957603508, 35.51421378149921537, -9.188101187500004485 ) ) ;
#13065=CARTESIAN_POINT ( 'NONE',  ( 76.87832059550045471, 59.35088420047541291, -15.98204322003894973 ) ) ;
#13070=CARTESIAN_POINT ( 'NONE',  ( 67.00187114335926708, 67.08813303282481399, 8.529924657355548945 ) ) ;
#13074=CARTESIAN_POINT ( 'NONE',  ( 79.11723855630626190, 59.11194703662724237, -16.21433712332713029 ) ) ;
#13075=CARTESIAN_POINT ( 'NONE',  ( 82.13265554904860721, 40.82714603808517495, 1.567016277279669412 ) ) ;
#13077=CARTESIAN_POINT ( 'NONE',  ( 76.83812372118222811, 63.31165668814058023, -15.46182035231785079 ) ) ;
#13080=EDGE_LOOP ( 'NONE', ( #63896, #55019, #97428, #54159, #97201, #49040, #32426, #9591 ) ) ;
#13089=CARTESIAN_POINT ( 'NONE',  ( 66.97748580466556234, 68.05911003901715617, 6.908000617270682042 ) ) ;
#13091=ORIENTED_EDGE ( 'NONE', *, *, #79614, .F. ) ;
#13094=B_SPLINE_CURVE_WITH_KNOTS ( 'NONE', 3,
 ( #43171, #73608, #35090, #57390, #41687, #65994, #65008, #95951, #96947, #27513, #51279, #88364, #12821 ),
 .UNSPECIFIED., .F., .F.,
 ( 4, 3, 3, 3, 4 ),
 ( 0.000000000000000000, 0.1333490885032349305, 0.3007194338854379256, 0.4699862290245218621, 0.4976065956401893864 ),
 .UNSPECIFIED. ) ;
#13099=ADVANCED_FACE ( 'NONE', ( #20889 ), #87493, .T. ) ;
#13102=CARTESIAN_POINT ( 'NONE',  ( 69.58015593410982547, 62.56871313314800176, -13.92720401298870314 ) ) ;
#13103=CARTESIAN_POINT ( 'NONE',  ( 71.88281838930642209, 59.56282477439597045, -15.74156321294393024 ) ) ;
#13104=EDGE_LOOP ( 'NONE', ( #26260, #81765, #40737, #42428 ) ) ;
#13114=CARTESIAN_POINT ( 'NONE',  ( 79.58915790851577299, 48.58846474191479814, 14.00006715458789408 ) ) ;
#13115=CARTESIAN_POINT ( 'NONE',  ( 68.72531525883097459, 70.03068556548458901, -2.698007717796147009 ) ) ;
#13118=CARTESIAN_POINT ( 'NONE',  ( 77.65745049418580948, 61.93790999624750526, 15.64425804037917977 ) ) ;
#13123=B_SPLINE_CURVE_WITH_KNOTS ( 'NONE', 3,
 ( #25948, #19362, #95882, #18347, #50222, #88291, #56822, #87805, #11256, #41615, #49240, #42119, #51207, #73052, #12238, #4628, #57319, #4121, #81176, #49724, #80175, #11742, #73538, #35015, #65915, #66422, #19840, #27440, #50711, #81665, #43098, #97352, #97842, #5128, #36508, #44096, #28411, #14218, #52202, #45595, #29911, #67412, #44594, #51735, #76525, #98840 ),
 .UNSPECIFIED., .F., .F.,
 ( 4, 1, 1, 1, 2, 2, 1, 1, 1, 2, 2, 1, 1, 2, 2, 1, 1, 2, 2, 1, 1, 2, 2, 1, 2, 2, 1, 2, 2, 4 ),
 ( 0.000000000000000000, 0.06249999999998591405, 0.09374999999997879474, 0.1093749999999743955, 0.1171874999999721056, 0.1249999999999698158, 0.1874999999999572009, 0.2187499999999528988, 0.2343749999999486244, 0.2421874999999465150, 0.2499999999999444333, 0.3124999999999362177, 0.3437499999999322209, 0.3593749999999303335, 0.3749999999999283906, 0.4374999999999171774, 0.4687499999999125144, 0.4843749999999111822, 0.4999999999999098499, 0.5624999999999139577, 0.5937499999999159561, 0.6093749999999177325, 0.6249999999999195088, 0.6874999999999310552, 0.7187499999999377165, 0.7499999999999442668, 0.8124999999999570344, 0.8437499999999632516, 0.8749999999999695799, 1.000000000000000000 ),
 .UNSPECIFIED. ) ;
#13127=CARTESIAN_POINT ( 'NONE',  ( 78.70150085959764397, 59.83202584994826623, 16.12694553795978081 ) ) ;
#13129=CARTESIAN_POINT ( 'NONE',  ( 84.14312167556933275, 48.98415679381830756, 0.000000000000000000 ) ) ;
#13135=CARTESIAN_POINT ( 'NONE',  ( 76.68698272566328455, 51.55172097108391682, -15.61692696388005253 ) ) ;
#13137=CARTESIAN_POINT ( 'NONE',  ( 71.50396643458246615, 72.35543200887750004, -1.254608710098219060 ) ) ;
#13142=CARTESIAN_POINT ( 'NONE',  ( 38.90461549961826648, 38.16454794089044356, -10.00000000000000355 ) ) ;
#13144=CARTESIAN_POINT ( 'NONE',  ( 74.83655476910678317, 53.51806293180211327, 16.54630480343736210 ) ) ;
#13146=CARTESIAN_POINT ( 'NONE',  ( 73.27736499958758998, 63.96510177322678459, 13.82219565750662937 ) ) ;
#13147=CARTESIAN_POINT ( 'NONE',  ( 67.15772368909350121, 67.74692886573922124, -6.548511843863573212 ) ) ;
#13148=EDGE_CURVE ( 'NONE', #3917, #82089, #22938, .T. ) ;
#13152=FACE_OUTER_BOUND ( 'NONE', #53976, .T. ) ;
#13158=ORIENTED_EDGE ( 'NONE', *, *, #27655, .F. ) ;
#13159=EDGE_CURVE ( 'NONE', #68463, #76483, #13511, .T. ) ;
#13166=CARTESIAN_POINT ( 'NONE',  ( 79.18000070754021635, 45.80091866078065976, -13.04680284947386681 ) ) ;
#13167=CARTESIAN_POINT ( 'NONE',  ( 71.84864803011454626, 61.11459157905925110, 15.23051327526690990 ) ) ;
#13168=CARTESIAN_POINT ( 'NONE',  ( 35.44910642356613550, 21.26216523072496045, -2.296566073217252530E-15 ) ) ;
#13172=EDGE_LOOP ( 'NONE', ( #23606, #33904, #89932, #28744 ) ) ;
#13173=CARTESIAN_POINT ( 'NONE',  ( 19.08967936351193373, 31.99752408145592497, 5.678558825948276656 ) ) ;
#13174=CARTESIAN_POINT ( 'NONE',  ( 76.49863583581506532, 63.42625474237735261, 14.98000607567798070 ) ) ;
#13175=CARTESIAN_POINT ( 'NONE',  ( 70.23435920221514550, 70.16979271778447469, -5.338967590826342757 ) ) ;
#13176=CARTESIAN_POINT ( 'NONE',  ( 11.78502771447809394, 29.73705186507753240, -3.090169943749475845 ) ) ;
#13186=CARTESIAN_POINT ( 'NONE',  ( 66.08197961146748867, 68.50086866870223901, -2.540402597524118455 ) ) ;
#13188=DIRECTION ( 'NONE',  ( -0.8660254037844378194, -0.5000000000000014433, -0.000000000000000000 ) ) ;
#13200=CARTESIAN_POINT ( 'NONE',  ( 75.14783087284527596, 67.02178724657008502, -12.71884470538153877 ) ) ;
#13207=( BOUNDED_CURVE ( )  B_SPLINE_CURVE ( 2, ( #8069, #63257, #94198, #71377, #40932, #1966, #25254, #85615, #87135, #93698, #31839, #79506, #963 ),
 .UNSPECIFIED., .F., .T. ) 
 B_SPLINE_CURVE_WITH_KNOTS ( ( 3, 2, 2, 2, 2, 2, 3 ),
 ( 0.8375000000000000222, 0.8399999999999999689, 0.8449999999999999734, 0.8499999999999999778, 0.8549999999999999822, 0.8599999999999999867, 0.8625000000000000444 ),
 .UNSPECIFIED. ) 
 CURVE ( )  GEOMETRIC_REPRESENTATION_ITEM ( )  RATIONAL_B_SPLINE_CURVE ( ( 0.9755282581475767101, 0.9755282581475772652, 1.000000000000000000, 0.9510565162951535312, 1.000000000000000000, 0.9510565162951535312, 1.000000000000000000, 0.9510565162951535312, 1.000000000000000000, 0.9510565162951535312, 1.000000000000000000, 0.9755282581475761550, 0.9755282581475767101 ) ) 
 REPRESENTATION_ITEM ( '' )  );
#13208=CARTESIAN_POINT ( 'NONE',  ( 71.38275130371390276, 63.94649258510062850, -13.17855260962158326 ) ) ;
#13212=ORIENTED_EDGE ( 'NONE', *, *, #26317, .T. ) ;
#13214=CARTESIAN_POINT ( 'NONE',  ( 76.05516770966454487, 51.24013347110783201, -16.11765975597679912 ) ) ;
#13216=CARTESIAN_POINT ( 'NONE',  ( 80.67108465943677231, 56.43556366967433746, 16.52050149510320765 ) ) ;
#13218=ADVANCED_FACE ( 'NONE', ( #40239 ), #71685, .T. ) ;
#13228=CARTESIAN_POINT ( 'NONE',  ( 88.02868988710136477, 43.76708177457258842, -2.199075477856099692 ) ) ;
#13229=( BOUNDED_CURVE ( )  B_SPLINE_CURVE ( 2, ( #39134, #24950, #30566, #15850, #84799, #23950, #40139, #47253, #660, #69052, #85831, #99983, #61452 ),
 .UNSPECIFIED., .F., .T. ) 
 B_SPLINE_CURVE_WITH_KNOTS ( ( 3, 2, 2, 2, 2, 2, 3 ),
 ( 0.1875000000000000000, 0.1900000000000000022, 0.1950000000000000067, 0.2000000000000000111, 0.2049999999999999878, 0.2099999999999999922, 0.2124999999999999944 ),
 .UNSPECIFIED. ) 
 CURVE ( )  GEOMETRIC_REPRESENTATION_ITEM ( )  RATIONAL_B_SPLINE_CURVE ( ( 0.9755282581475768211, 0.9755282581475768211, 1.000000000000000000, 0.9510565162951535312, 1.000000000000000000, 0.9510565162951535312, 1.000000000000000000, 0.9510565162951535312, 1.000000000000000000, 0.9510565162951535312, 1.000000000000000000, 0.9755282581475768211, 0.9755282581475768211 ) ) 
 REPRESENTATION_ITEM ( '' )  );
#13230=CARTESIAN_POINT ( 'NONE',  ( 72.97386446981147401, 70.68132344495337804, 8.316175787459503255 ) ) ;
#13238=CARTESIAN_POINT ( 'NONE',  ( 81.12147712725017357, 52.00152150211298618, 15.09009577504130029 ) ) ;
#13240=EDGE_CURVE ( 'NONE', #47570, #34846, #48373, .T. ) ;
#13246=CARTESIAN_POINT ( 'NONE',  ( 26.31557204471864253, 27.14441083166262203, 10.00000000000000533 ) ) ;
#13250=CARTESIAN_POINT ( 'NONE',  ( 69.62482084542597249, 69.32845382139950630, -7.406819698113993766 ) ) ;
#13255=ORIENTED_EDGE ( 'NONE', *, *, #98161, .T. ) ;
#13256=CARTESIAN_POINT ( 'NONE',  ( 66.83852597929605110, 67.59941986568811956, -6.474490792332534994 ) ) ;
#13260=CARTESIAN_POINT ( 'NONE',  ( 25.74102936209481385, 30.56454794089042437, 10.00000000000000355 ) ) ;
#13261=CARTESIAN_POINT ( 'NONE',  ( 85.56872147382391347, 49.01729895498410627, 12.25953038224546887 ) ) ;
#13264=DIRECTION ( 'NONE',  ( -0.5242119900219301964, 0.000000000000000000, -0.8515878049369001168 ) ) ;
#13276=CARTESIAN_POINT ( 'NONE',  ( 79.25902298712658478, 59.95016084666949752, 16.14518600951581817 ) ) ;
#13277=CARTESIAN_POINT ( 'NONE',  ( 39.01788588657935719, 31.03085787977765975, 9.188101187500006262 ) ) ;
#13285=CARTESIAN_POINT ( 'NONE',  ( 19.48598279363274344, 13.11110640527291693, -2.839279412974138328 ) ) ;
#13287=CARTESIAN_POINT ( 'NONE',  ( 82.74741872462533365, 53.81327073439516084, 15.79824936317409900 ) ) ;
#13295=CARTESIAN_POINT ( 'NONE',  ( 81.35504097469424778, 42.12982285155051443, 8.020547866998608555 ) ) ;
#13303=ORIENTED_EDGE ( 'NONE', *, *, #55887, .F. ) ;
#13310=CARTESIAN_POINT ( 'NONE',  ( 80.56202954020665175, 57.53823600680944139, 16.23110421993948549 ) ) ;
#13325=CARTESIAN_POINT ( 'NONE',  ( 82.71332607344807286, 50.53308841156612630, -14.58498437345447662 ) ) ;
#13333=CARTESIAN_POINT ( 'NONE',  ( 81.20168625321292666, 55.28033247127913796, -15.96862711004452784 ) ) ;
#13337=CARTESIAN_POINT ( 'NONE',  ( 67.27771118422515428, 66.58732564224565920, 8.551707608175874498 ) ) ;
#13339=CARTESIAN_POINT ( 'NONE',  ( 85.51384538016034753, 42.26407845341874747, 2.123067372083550897 ) ) ;
#13342=CARTESIAN_POINT ( 'NONE',  ( 71.05835085023741726, 67.33870905001845131, 10.36604878428025955 ) ) ;
#13344=CARTESIAN_POINT ( 'NONE',  ( 79.36339018020615299, 45.77489031751736093, 12.95595637456517046 ) ) ;
#13357=CARTESIAN_POINT ( 'NONE',  ( 84.54558420127669649, 50.65463084595457843, 13.70779263677913562 ) ) ;
#13365=CARTESIAN_POINT ( 'NONE',  ( 70.60363933684126891, 71.39732000281048840, -0.9291670929876240104 ) ) ;
#13367=CARTESIAN_POINT ( 'NONE',  ( 76.12823843484866870, 51.15411698274154162, 16.08981265264790750 ) ) ;
#13368=CARTESIAN_POINT ( 'NONE',  ( 81.73250340314956475, 41.47603874751758468, -5.132177573234927515 ) ) ;
#13378=CARTESIAN_POINT ( 'NONE',  ( 4.856824484202590497, 25.73705186507751819, -3.090169943749475845 ) ) ;
#13381=CARTESIAN_POINT ( 'NONE',  ( 73.63650596374165502, 69.59800771093053129, 10.20034856658873323 ) ) ;
#13385=CARTESIAN_POINT ( 'NONE',  ( 69.32567463353416315, 68.52802923855151107, 7.491982181575302491 ) ) ;
#13386=CARTESIAN_POINT ( 'NONE',  ( 66.31646558143364700, 68.08799829551760752, -4.617347279476426536 ) ) ;
#13389=CARTESIAN_POINT ( 'NONE',  ( 79.76359975193354046, 44.98417069036879923, 11.54310746654911846 ) ) ;
#13392=CARTESIAN_POINT ( 'NONE',  ( 83.84382548910321020, 44.36689950846875519, 9.171174898895673167 ) ) ;
#13394=CARTESIAN_POINT ( 'NONE',  ( 28.84566271970979301, 17.44966523072494979, -2.296566073217252530E-15 ) ) ;
#13396=CARTESIAN_POINT ( 'NONE',  ( 83.78311978599397492, 51.75050911116664309, -14.85521894841905599 ) ) ;
#13409=CARTESIAN_POINT ( 'NONE',  ( 70.25375250786443360, 69.20215222833037672, 7.266984090244938521 ) ) ;
#13421=CARTESIAN_POINT ( 'NONE',  ( 11.06379537489605625, 28.16126292948893806, -6.180339887498951690 ) ) ;
#13423=VERTEX_POINT ( 'NONE', #90777 ) ;
#13425=CARTESIAN_POINT ( 'NONE',  ( 86.44808582675112518, 47.03435218195901513, -10.53111747673477794 ) ) ;
#13438=DIRECTION ( 'NONE',  ( 0.2347357813929421555, -0.4065742997269585213, 0.8829475928589297640 ) ) ;
#13439=CARTESIAN_POINT ( 'NONE',  ( 81.35748880148535989, 42.22347387491733883, -7.155507324468844743 ) ) ;
#13440=B_SPLINE_SURFACE_WITH_KNOTS ( 'NONE', 3, 1, ( 
 ( #41513, #88687 ),
 ( #50124, #10134 ),
 ( #64835, #3061 ),
 ( #57211, #17216 ),
 ( #9652, #48122 ),
 ( #2546, #33429 ),
 ( #64326, #27821 ),
 ( #74449, #13626 ),
 ( #37398, #44498 ),
 ( #5519, #58697 ),
 ( #67308, #52106 ),
 ( #5029, #89672 ),
 ( #28307, #14119 ),
 ( #83554, #6522 ),
 ( #73930, #90670 ),
 ( #36402, #20232 ),
 ( #44999, #21227 ),
 ( #35416, #98742 ),
 ( #75945, #83053 ),
 ( #4516, #66323 ),
 ( #12130, #21714 ),
 ( #43510, #98235 ),
 ( #74936, #75429 ),
 ( #97740, #82574 ),
 ( #67819, #68303 ),
 ( #27333, #28820 ),
 ( #59704, #58215 ),
 ( #89193, #60188 ),
 ( #13137, #36906 ),
 ( #12638, #91149 ),
 ( #6013, #51620 ) ),
 .UNSPECIFIED., .F., .F., .F.,
 ( 4, 3, 3, 3, 3, 3, 3, 3, 3, 3, 4 ),
 ( 2, 2 ),
 ( 0.000000000000000000, 0.1333490885032380391, 0.3007194338854225490, 0.4699862290244999907, 0.5844252810809225096, 0.6686540514502540278, 0.7354980260655328284, 0.8028463152565535887, 0.8633854507757017238, 0.9437142632667037123, 1.000000000000000000 ),
 ( 0.000000000000000000, 1.000000000000000000 ),
 .UNSPECIFIED. ) ;
#13441=ORIENTED_EDGE ( 'NONE', *, *, #57812, .T. ) ;
#13452=EDGE_CURVE ( 'NONE', #85116, #3917, #83664, .T. ) ;
#13454=CARTESIAN_POINT ( 'NONE',  ( 73.67429767784587114, 67.97956927692818851, -11.30367013265376563 ) ) ;
#13457=CARTESIAN_POINT ( 'NONE',  ( 81.30818518503046732, 58.89441083166271085, 0.000000000000000000 ) ) ;
#13458=CARTESIAN_POINT ( 'NONE',  ( 6.244247187202517146, 25.64646525600388216, -2.839279412974133887 ) ) ;
#13477=CARTESIAN_POINT ( 'NONE',  ( 86.05489758235616193, 44.63495567976185185, -6.775695627399047183 ) ) ;
#13480=CARTESIAN_POINT ( 'NONE',  ( 75.96128792555467157, 65.56719406519354720, 13.89537262461679212 ) ) ;
#13488=CARTESIAN_POINT ( 'NONE',  ( 69.10717603675902865, 66.30743475805610387, -10.20864196604519769 ) ) ;
#13490=CARTESIAN_POINT ( 'NONE',  ( 85.78101276405163844, 42.88643024831080908, 1.820988380798113537 ) ) ;
#13492=CARTESIAN_POINT ( 'NONE',  ( 83.66738886159650690, 44.95173633656256129, 9.291185867263966003 ) ) ;
#13499=CARTESIAN_POINT ( 'NONE',  ( 78.01941338035848617, 51.47862715311421056, 15.42328866796606235 ) ) ;
#13506=CARTESIAN_POINT ( 'NONE',  ( 84.68103419341217375, 50.25510846593720515, 13.84703097836258934 ) ) ;
#13511=( BOUNDED_CURVE ( )  B_SPLINE_CURVE ( 2, ( #54950, #8856, #17457, #39724, #70654, #1777, #32150, #25566, #55431, #32656, #63556, #72180, #1266 ),
 .UNSPECIFIED., .F., .T. ) 
 B_SPLINE_CURVE_WITH_KNOTS ( ( 3, 2, 2, 2, 2, 2, 3 ),
 ( 0.6125000000000000444, 0.6149999999999999911, 0.6199999999999999956, 0.6250000000000000000, 0.6300000000000000044, 0.6350000000000000089, 0.6375000000000000666 ),
 .UNSPECIFIED. ) 
 CURVE ( )  GEOMETRIC_REPRESENTATION_ITEM ( )  RATIONAL_B_SPLINE_CURVE ( ( 0.9755282581475767101, 0.9755282581475772652, 1.000000000000000000, 0.9510565162951535312, 1.000000000000000000, 0.9510565162951535312, 1.000000000000000000, 0.9510565162951535312, 1.000000000000000000, 0.9510565162951535312, 1.000000000000000000, 0.9755282581475761550, 0.9755282581475767101 ) ) 
 REPRESENTATION_ITEM ( '' )  );
#13512=ADVANCED_FACE ( 'NONE', ( #98846 ), #93682, .T. ) ;
#13515=CARTESIAN_POINT ( 'NONE',  ( 5.120201826081539842, 21.14336893147752861, 7.433330006724141015 ) ) ;
#13522=CARTESIAN_POINT ( 'NONE',  ( 37.43858582280105907, 33.56628583063844218, 9.188101187500006262 ) ) ;
#13524=FACE_BOUND ( 'NONE', #85588, .T. ) ;
#13526=CARTESIAN_POINT ( 'NONE',  ( 24.12224894148702248, 22.43085787977763701, -9.188101187500008038 ) ) ;
#13527=CARTESIAN_POINT ( 'NONE',  ( 36.34934470066777834, 21.39040679176985194, 1.333680081654574804E-15 ) ) ;
#13530=VERTEX_POINT ( 'NONE', #21819 ) ;
#13531=CARTESIAN_POINT ( 'NONE',  ( 70.90699100671335486, 61.04309739204857266, 15.03109142694147948 ) ) ;
#13533=CARTESIAN_POINT ( 'NONE',  ( 73.16956295238907160, 57.33411781477383329, 16.38320611710937058 ) ) ;
#13539=CARTESIAN_POINT ( 'NONE',  ( 83.70225478178599587, 46.26040777977714669, -11.35289932219425602 ) ) ;
#13547=B_SPLINE_CURVE_WITH_KNOTS ( 'NONE', 3,
 ( #55767, #88260, #56283, #3136, #48714, #16794, #79645, #10211, #49692, #24400, #34020, #63895, #86255, #87282, #9203, #48196 ),
 .UNSPECIFIED., .F., .F.,
 ( 4, 1, 2, 2, 2, 1, 2, 2, 4 ),
 ( 0.000000000000000000, 0.1250000000000055234, 0.1875000000000074385, 0.2500000000000093814, 0.5000000000000118794, 0.6250000000000117684, 0.6875000000000107692, 0.7500000000000096589, 1.000000000000000000 ),
 .UNSPECIFIED. ) ;
#13549=CARTESIAN_POINT ( 'NONE',  ( 88.17106782721933200, 44.41923492627702075, -4.565543248975949098 ) ) ;
#13552=CARTESIAN_POINT ( 'NONE',  ( 37.65389587561886486, 30.24335787977765833, -9.188101187500008038 ) ) ;
#13553=CARTESIAN_POINT ( 'NONE',  ( 80.12724894187661562, 44.72419067623221167, 11.12292608744810529 ) ) ;
#13554=CARTESIAN_POINT ( 'NONE',  ( 72.09806618716604021, 60.83808587311448690, -14.86418196441615258 ) ) ;
#13557=ORIENTED_EDGE ( 'NONE', *, *, #95300, .T. ) ;
#13560=CARTESIAN_POINT ( 'NONE',  ( 87.04122873496829982, 46.31593380912286761, -9.298662157179395038 ) ) ;
#13566=CARTESIAN_POINT ( 'NONE',  ( 74.65094944003260480, 60.90640990763624529, -15.37438762173259121 ) ) ;
#13569=CARTESIAN_POINT ( 'NONE',  ( 77.08262651433446422, 63.62497865693946153, -15.40261155718560815 ) ) ;
#13571=CARTESIAN_POINT ( 'NONE',  ( 78.86410592861936664, 59.57720046317054852, 16.50785913320112996 ) ) ;
#13576=CARTESIAN_POINT ( 'NONE',  ( 74.22019797964286170, 68.67351823779483766, -11.46693203622143820 ) ) ;
#13579=CARTESIAN_POINT ( 'NONE',  ( 68.45576418072165836, 69.87261364207513736, 4.691110543634933627 ) ) ;
#13580=CARTESIAN_POINT ( 'NONE',  ( 74.15525029152222203, 55.50479885125673718, -16.11756190328145166 ) ) ;
#13589=CARTESIAN_POINT ( 'NONE',  ( 69.89140086045073019, 62.80215112504183850, -13.32307909001956858 ) ) ;
#13594=CARTESIAN_POINT ( 'NONE',  ( 82.34676179634530513, 41.29334736454898547, -3.425696165949260852 ) ) ;
#13603=CARTESIAN_POINT ( 'NONE',  ( 69.81478986972626899, 70.37643060760527192, -3.960572301807858242 ) ) ;
#13613=CARTESIAN_POINT ( 'NONE',  ( 73.47309087361824709, 69.99741330878467238, -9.625970422713120200 ) ) ;
#13615=( LENGTH_UNIT ( ) NAMED_UNIT ( * ) SI_UNIT ( .MILLI., .METRE. ) );
#13618=CARTESIAN_POINT ( 'NONE',  ( 85.49318370521093868, 48.99722645306706426, -12.73116331006621316 ) ) ;
#13619=CARTESIAN_POINT ( 'NONE',  ( 72.24711563986207352, 72.09099709781209242, 3.122935046306669626 ) ) ;
#13626=CARTESIAN_POINT ( 'NONE',  ( 72.13656828596906223, 72.31233833605649863, -1.326438232958793595 ) ) ;
#13628=CARTESIAN_POINT ( 'NONE',  ( 14.85459438965255607, 31.68290643055186706, 3.479690158560446702E-15 ) ) ;
#13631=CARTESIAN_POINT ( 'NONE',  ( 35.06352437372437691, 42.01751292744058475, 6.180339887498949913 ) ) ;
#13633=CARTESIAN_POINT ( 'NONE',  ( 76.50778254745674190, 62.49071378302044621, 15.67075087195867944 ) ) ;
#13635=CARTESIAN_POINT ( 'NONE',  ( 72.66072155841338542, 61.62800837470290816, 14.69956871679224442 ) ) ;
#13649=ORIENTED_EDGE ( 'NONE', *, *, #59652, .F. ) ;
#13652=CARTESIAN_POINT ( 'NONE',  ( 79.17880889709233827, 46.03054149826856190, -13.20140403770785831 ) ) ;
#13658=ORIENTED_EDGE ( 'NONE', *, *, #24862, .T. ) ;
#13659=CARTESIAN_POINT ( 'NONE',  ( 26.13094010387951371, 20.80170272979927049, 7.433330006724137462 ) ) ;
#13660=CARTESIAN_POINT ( 'NONE',  ( 22.17733255989135088, 35.73705186507754661, -3.090169943749475845 ) ) ;
#13661=CARTESIAN_POINT ( 'NONE',  ( 72.13796995798945488, 70.29191212227198093, -7.425297919149587145 ) ) ;
#13662=CARTESIAN_POINT ( 'NONE',  ( 75.07870222088888568, 67.13256391452974015, -13.06718628923150582 ) ) ;
#13670=CARTESIAN_POINT ( 'NONE',  ( 66.32409466995383696, 68.70548013689253253, -2.129162495935091659 ) ) ;
#13672=CARTESIAN_POINT ( 'NONE',  ( 85.93470712620026575, 48.23248545518190866, 11.93606436224419909 ) ) ;
#13677=VERTEX_POINT ( 'NONE', #53468 ) ;
#13680=ORIENTED_EDGE ( 'NONE', *, *, #21060, .F. ) ;
#13684=CARTESIAN_POINT ( 'NONE',  ( 76.27744555259825177, 65.02376616331082460, 14.64893924750894350 ) ) ;
#13690=CARTESIAN_POINT ( 'NONE',  ( 70.68522907938090327, 64.69131028183736021, 12.41109312486960015 ) ) ;
#13691=CARTESIAN_POINT ( 'NONE',  ( 87.39560864876780499, 44.96555158233555716, 6.898727475461879699 ) ) ;
#13695=CARTESIAN_POINT ( 'NONE',  ( 66.24778991220809132, 68.20621754481172161, 4.138286745133333611 ) ) ;
#13698=CARTESIAN_POINT ( 'NONE',  ( 71.93062239541285408, 69.86009586726821396, -7.857747555887292457 ) ) ;
#13699=CARTESIAN_POINT ( 'NONE',  ( 76.16520121882301453, 51.58665863457357403, -16.17654979223751610 ) ) ;
#13706=CARTESIAN_POINT ( 'NONE',  ( 88.24418735786636603, 44.41312371456485408, 4.416884733071428926 ) ) ;
#13707=CARTESIAN_POINT ( 'NONE',  ( 85.20344164368778195, 43.30853108818458708, 4.813148867806795295 ) ) ;
#13708=CARTESIAN_POINT ( 'NONE',  ( 88.01315147845571119, 43.76068472133272280, -2.215761827693341957 ) ) ;
#13712=CARTESIAN_POINT ( 'NONE',  ( 75.95696686559092825, 52.20348117277876554, 15.83814512776487327 ) ) ;
#13715=CARTESIAN_POINT ( 'NONE',  ( 81.18177496026471829, 52.29543988957072997, 15.18084038034863248 ) ) ;
#13716=CARTESIAN_POINT ( 'NONE',  ( 73.70115868159994932, 69.61480312196140119, -9.646229744283855823 ) ) ;
#13722=CARTESIAN_POINT ( 'NONE',  ( 20.95177465265983585, 30.83478043621388665, -8.090169943749479842 ) ) ;
#13731=CARTESIAN_POINT ( 'NONE',  ( 72.93368834549268342, 70.33274728410245302, -8.126413671899975100 ) ) ;
#13734=CARTESIAN_POINT ( 'NONE',  ( 27.53097578467762219, 16.86426979415090699, -3.090169943749474069 ) ) ;
#13735=CARTESIAN_POINT ( 'NONE',  ( 85.66185486794186943, 48.65504738537000406, 12.40237352552430750 ) ) ;
#13737=CARTESIAN_POINT ( 'NONE',  ( 71.98986200492696241, 72.23686350399877654, -3.591898176886850980 ) ) ;
#13745=CARTESIAN_POINT ( 'NONE',  ( 81.84820468759039613, 41.18211169042432829, 5.670485032956731786 ) ) ;
#13750=CARTESIAN_POINT ( 'NONE',  ( 33.27084535048209091, 40.18502408145594273, 5.678558825948277544 ) ) ;
#13758=CARTESIAN_POINT ( 'NONE',  ( 20.49695707787433463, 14.76004757982089188, 5.678558825948272215 ) ) ;
#13761=CARTESIAN_POINT ( 'NONE',  ( 71.40405452044859658, 59.30247739756921987, 15.73691996190138731 ) ) ;
#13767=CARTESIAN_POINT ( 'NONE',  ( 88.15969727192141647, 44.33042168331400745, 2.709744954521523308 ) ) ;
#13771=CARTESIAN_POINT ( 'NONE',  ( 82.69197927684081151, 40.54452889128955206, 0.8884936269468197700 ) ) ;
#13779=VERTEX_POINT ( 'NONE', #24074 ) ;
#13781=CARTESIAN_POINT ( 'NONE',  ( 80.15404930735284950, 58.24487849859600885, -16.60713908503101521 ) ) ;
#13782=CARTESIAN_POINT ( 'NONE',  ( 80.24454609401104221, 57.41156006636176556, -16.59009416930489422 ) ) ;
#13797=CARTESIAN_POINT ( 'NONE',  ( 31.60618414714233637, 41.18080186712595747, 3.090169943749475401 ) ) ;
#13800=ORIENTED_EDGE ( 'NONE', *, *, #46624, .F. ) ;
#13802=CARTESIAN_POINT ( 'NONE',  ( 82.53565421717173933, 50.59536920694240791, -14.66185160561549594 ) ) ;
#13810=CARTESIAN_POINT ( 'NONE',  ( 72.28945313610159928, 58.55580128780883342, -15.58200032445072125 ) ) ;
#13819=CARTESIAN_POINT ( 'NONE',  ( 79.41195711930690493, 53.07626158231409619, -15.66850831761463070 ) ) ;
#13820=EDGE_CURVE ( 'NONE', #22997, #25763, #24814, .T. ) ;
#13822=CARTESIAN_POINT ( 'NONE',  ( 79.49951204047911801, 46.37032438487754149, 12.70281872619212393 ) ) ;
#13825=CARTESIAN_POINT ( 'NONE',  ( 83.66603977373949874, 52.22634557578435732, -14.68915192515179235 ) ) ;
#13841=ORIENTED_EDGE ( 'NONE', *, *, #77873, .F. ) ;
#13844=CARTESIAN_POINT ( 'NONE',  ( 81.89485588203808675, 55.22971306509118250, 16.24120679747552032 ) ) ;
#13845=EDGE_CURVE ( 'NONE', #70075, #27651, #28995, .T. ) ;
#13848=DIRECTION ( 'NONE',  ( 0.5000000000000014433, -0.8660254037844378194, 0.000000000000000000 ) ) ;
#13851=CARTESIAN_POINT ( 'NONE',  ( 68.74436278108203169, 64.70250930642976073, -12.15889933130203637 ) ) ;
#13859=CARTESIAN_POINT ( 'NONE',  ( 5.272250483539712818, 24.81751292744053927, -6.180339887498951690 ) ) ;
#13861=CARTESIAN_POINT ( 'NONE',  ( 71.79142014069363142, 59.57573540338584195, -15.72233485351718230 ) ) ;
#13862=LINE ( 'NONE', #52851, #36169 ) ;
#13867=CARTESIAN_POINT ( 'NONE',  ( 67.79725476218452229, 65.71048819351143777, 10.00598338191753101 ) ) ;
#13868=CARTESIAN_POINT ( 'NONE',  ( 66.07327459268398684, 68.54940412191220389, -4.524685454579428168 ) ) ;
#13869=ORIENTED_EDGE ( 'NONE', *, *, #98665, .T. ) ;
#13874=CARTESIAN_POINT ( 'NONE',  ( 23.65314546706850862, 31.84336893147757408, -7.433330006724137462 ) ) ;
#13876=CARTESIAN_POINT ( 'NONE',  ( 83.70956241415673560, 51.66838590121233210, -14.83800726304596118 ) ) ;
#13878=CARTESIAN_POINT ( 'NONE',  ( 88.11819866784119881, 43.86870363832048270, 2.501606352371071651 ) ) ;
#13879=CARTESIAN_POINT ( 'NONE',  ( 75.10353227920388974, 67.08955699197328215, 13.10598502456514503 ) ) ;
#13880=CARTESIAN_POINT ( 'NONE',  ( 68.58822102335196291, 64.27314873672484907, 12.42572437470450986 ) ) ;
#13888=CARTESIAN_POINT ( 'NONE',  ( 80.20857538925844210, 44.21345027839175401, -11.30608575764590107 ) ) ;
#13892=CARTESIAN_POINT ( 'NONE',  ( 71.65793835465373718, 72.08874482037508358, 0.6792430321896046896 ) ) ;
#13900=CARTESIAN_POINT ( 'NONE',  ( 13.13113612116928763, 15.78052372038639106, -10.00000000000000355 ) ) ;
#13908=EDGE_CURVE ( 'NONE', #41583, #78218, #30355, .T. ) ;
#13909=CARTESIAN_POINT ( 'NONE',  ( 30.67947171958994090, 41.21091486745863364, -1.111400068045478839E-16 ) ) ;
#13911=B_SPLINE_CURVE_WITH_KNOTS ( 'NONE', 3,
 ( #39851, #62664, #47475, #70784, #55558, #25696, #9495, #11873, #86051, #55066, #32275, #43233, #48489, #74174, #1395, #50347, #24677, #4246, #25176, #56576, #79430, #71804, #94122, #93616, #88932, #40858, #24184, #78399, #63178, #19491, #2401 ),
 .UNSPECIFIED., .F., .F.,
 ( 4, 3, 3, 3, 3, 3, 3, 3, 3, 3, 4 ),
 ( 0.000000000000000000, 0.1333490885032357076, 0.3007194338854359827, 0.4699862290245028773, 0.5844252810809169585, 0.6686540514502661292, 0.7354980260655498148, 0.8028463152565713523, 0.8633854507757302565, 0.9437142632667330222, 1.000000000000000000 ),
 .UNSPECIFIED. ) ;
#13918=CARTESIAN_POINT ( 'NONE',  ( 73.07600783879472317, 69.60248043393922046, -9.824339152688605026 ) ) ;
#13920=CARTESIAN_POINT ( 'NONE',  ( 81.23681747614864435, 42.40944431637972656, -7.576782141913678714 ) ) ;
#13927=CARTESIAN_POINT ( 'NONE',  ( 73.76584831522593788, 68.38082682530667000, 11.49424229391076402 ) ) ;
#13929=CARTESIAN_POINT ( 'NONE',  ( 70.43095659816272303, 71.06107982962434733, 2.817390920827290923 ) ) ;
#13933=CARTESIAN_POINT ( 'NONE',  ( 70.10515995482631979, 68.44220587271549050, -8.343978931046503789 ) ) ;
#13935=ORIENTED_EDGE ( 'NONE', *, *, #31039, .T. ) ;
#13936=CARTESIAN_POINT ( 'NONE',  ( 66.06214068257196459, 68.71579393632853794, -0.4716098740908659659 ) ) ;
#13937=CARTESIAN_POINT ( 'NONE',  ( 16.86928618479236164, 18.24335787977762990, -9.188101187500008038 ) ) ;
#13955=CARTESIAN_POINT ( 'NONE',  ( 71.25860280237223776, 63.33879986367642090, -13.50434263417577263 ) ) ;
#13958=ADVANCED_FACE ( 'NONE', ( #1549 ), #55210, .T. ) ;
#13966=CARTESIAN_POINT ( 'NONE',  ( 76.27744555259825177, 65.02376616331082460, 14.64893924750894705 ) ) ;
#13968=ORIENTED_EDGE ( 'NONE', *, *, #90314, .F. ) ;
#13973=DIRECTION ( 'NONE',  ( -0.8660254037844377084, -0.5000000000000014433, -0.000000000000000000 ) ) ;
#13975=VECTOR ( 'NONE', #48368, 1000.000000000000000 ) ;
#13978=CARTESIAN_POINT ( 'NONE',  ( 81.04961468568201610, 43.68546784643918812, -9.492462169003026418 ) ) ;
#13982=CARTESIAN_POINT ( 'NONE',  ( 87.82209769797702847, 44.43170261543946964, -3.947207905613685952 ) ) ;
#13984=CARTESIAN_POINT ( 'NONE',  ( 79.42866338260434134, 59.50128377535573776, 16.18467811310512872 ) ) ;
#13986=CARTESIAN_POINT ( 'NONE',  ( 80.24139587601152357, 53.52586694347819929, -15.66200724048011672 ) ) ;
#13987=CARTESIAN_POINT ( 'NONE',  ( 66.10228174255657052, 68.64626758096548542, 4.271897712742705799 ) ) ;
#13990=CARTESIAN_POINT ( 'NONE',  ( 84.54066908761240029, 50.65850875116926488, 13.71172019562601285 ) ) ;
#13998=CARTESIAN_POINT ( 'NONE',  ( 13.25720545158990937, 8.449665230724928477, -2.296566073217252530E-15 ) ) ;
#14002=CARTESIAN_POINT ( 'NONE',  ( 82.60090280491364467, 41.94575979494328521, -5.057853582627321209 ) ) ;
#14007=CARTESIAN_POINT ( 'NONE',  ( 32.92443518896833154, 39.98502408145595410, -5.678558825948271327 ) ) ;
#14011=CARTESIAN_POINT ( 'NONE',  ( 18.31869600479030424, 33.68290643055186706, 3.479690158560446702E-15 ) ) ;
#14012=CARTESIAN_POINT ( 'NONE',  ( 13.57497413706089517, 16.03677371833800436, 10.00000000000000533 ) ) ;
#14017=CARTESIAN_POINT ( 'NONE',  ( 70.39311885314104700, 61.02709512477209586, 14.38506243159549314 ) ) ;
#14018=CARTESIAN_POINT ( 'NONE',  ( 75.96213316711562413, 65.70078031631311433, -14.22672748915905316 ) ) ;
#14019=CARTESIAN_POINT ( 'NONE',  ( 73.57796644695659438, 59.01413344347207612, 16.12674309221841895 ) ) ;
#14023=EDGE_LOOP ( 'NONE', ( #78630, #22964, #77161, #16147 ) ) ;
#14030=CARTESIAN_POINT ( 'NONE',  ( 86.46015012553586132, 47.50298594968677435, -10.46242490754989518 ) ) ;
#14036=CARTESIAN_POINT ( 'NONE',  ( 37.26657704017246431, 36.91421378149922816, 9.188101187500008038 ) ) ;
#14041=CARTESIAN_POINT ( 'NONE',  ( 87.66480641278828045, 45.41976245752641006, 6.618816385381215639 ) ) ;
#14051=CARTESIAN_POINT ( 'NONE',  ( 68.96685452785939674, 69.33442928595859200, 6.693821423866975984 ) ) ;
#14052=CARTESIAN_POINT ( 'NONE',  ( 75.29281472599660674, 60.68631827055407513, -15.54484235153014282 ) ) ;
#14055=CARTESIAN_POINT ( 'NONE',  ( 77.21485428481166480, 62.97229237163904969, -15.28182260264458492 ) ) ;
#14060=CARTESIAN_POINT ( 'NONE',  ( 37.18115723113500337, 22.26216523072496400, -2.296566073217252530E-15 ) ) ;
#14067=CARTESIAN_POINT ( 'NONE',  ( 19.46394688279507079, 19.43677371833800649, -10.00000000000000355 ) ) ;
#14068=VERTEX_POINT ( 'NONE', #76906 ) ;
#14072=CARTESIAN_POINT ( 'NONE',  ( 79.14312167556931854, 57.64441083166269664, 0.000000000000000000 ) ) ;
#14074=FACE_OUTER_BOUND ( 'NONE', #37086, .T. ) ;
#14080=CARTESIAN_POINT ( 'NONE',  ( 69.99892673467476811, 62.80419320708934094, -13.35911945385968735 ) ) ;
#14083=AXIS2_PLACEMENT_3D ( 'NONE', #37443, #76950, #98285 ) ;
#14090=CARTESIAN_POINT ( 'NONE',  ( 71.83801353683954005, 72.23051172126305630, 3.257724734605890848 ) ) ;
#14091=CARTESIAN_POINT ( 'NONE',  ( 84.24093560737047426, 44.97564044950197371, 8.884023765932731465 ) ) ;
#14094=( BOUNDED_CURVE ( )  B_SPLINE_CURVE ( 2, ( #67681, #98611, #92996, #94010, #79324, #31648, #31154, #24066, #55940, #762, #46347, #94510, #54959 ),
 .UNSPECIFIED., .F., .T. ) 
 B_SPLINE_CURVE_WITH_KNOTS ( ( 3, 2, 2, 2, 2, 2, 3 ),
 ( 0.7875000000000000888, 0.7900000000000000355, 0.7950000000000000400, 0.8000000000000000444, 0.8050000000000000488, 0.8100000000000000533, 0.8125000000000000000 ),
 .UNSPECIFIED. ) 
 CURVE ( )  GEOMETRIC_REPRESENTATION_ITEM ( )  RATIONAL_B_SPLINE_CURVE ( ( 0.9755282581475767101, 0.9755282581475772652, 1.000000000000000000, 0.9510565162951535312, 1.000000000000000000, 0.9510565162951535312, 1.000000000000000000, 0.9510565162951535312, 1.000000000000000000, 0.9510565162951535312, 1.000000000000000000, 0.9755282581475768211, 0.9755282581475768211 ) ) 
 REPRESENTATION_ITEM ( '' )  );
#14095=CARTESIAN_POINT ( 'NONE',  ( 70.54765706325409269, 60.82528431242337064, -15.03543891230351370 ) ) ;
#14096=CARTESIAN_POINT ( 'NONE',  ( 72.40063605961431392, 70.75631031022656714, -6.847773698889723981 ) ) ;
#14102=B_SPLINE_CURVE_WITH_KNOTS ( 'NONE', 3,
 ( #84920, #69178, #83430, #68179, #68676, #54454, #8390, #52984, #100108, #53477 ),
 .UNSPECIFIED., .F., .F.,
 ( 4, 2, 2, 2, 4 ),
 ( 0.000000000000000000, 0.0002622400424273382911, 0.0005244800848546765822, 0.0007867201272820148732, 0.001048960169709353164 ),
 .UNSPECIFIED. ) ;
#14106=CARTESIAN_POINT ( 'NONE',  ( 73.27146650943220152, 69.63413511619549467, -9.919440617956860606 ) ) ;
#14109=CARTESIAN_POINT ( 'NONE',  ( 68.55513178119723250, 64.39780669069259034, 11.67030924314737206 ) ) ;
#14110=CARTESIAN_POINT ( 'NONE',  ( 82.55167669771859096, 54.18190009503562266, 15.56852171010267938 ) ) ;
#14111=CARTESIAN_POINT ( 'NONE',  ( 72.04296851029907600, 72.03750459758265379, 2.856970073737167048 ) ) ;
#14117=CARTESIAN_POINT ( 'NONE',  ( 81.27790830334583916, 42.47193573065089822, -7.638390500584347542 ) ) ;
#14118=CARTESIAN_POINT ( 'NONE',  ( 80.61857449287080613, 50.42422421458247328, -14.58301214530503387 ) ) ;
#14119=CARTESIAN_POINT ( 'NONE',  ( 72.04541054607656747, 72.23942076927355060, -1.584012611844705765 ) ) ;
#14121=CARTESIAN_POINT ( 'NONE',  ( 28.84566271970979301, 17.44966523072495335, -2.296566073217252530E-15 ) ) ;
#14124=CARTESIAN_POINT ( 'NONE',  ( 45.26690985970349601, 25.94473085651396005, 1.475505719884397138E-15 ) ) ;
#14140=DIRECTION ( 'NONE',  ( -0.9646071681523451513, 0.2636911283094546254, 0.000000000000000000 ) ) ;
#14143=CARTESIAN_POINT ( 'NONE',  ( 79.15998105033318666, 45.86243901705208259, -13.09633689766342890 ) ) ;
#14145=CARTESIAN_POINT ( 'NONE',  ( 84.00344187778067351, 41.31840900968617802, 1.163504541493592948 ) ) ;
#14151=CARTESIAN_POINT ( 'NONE',  ( 23.96105869301208813, 16.76004757982089899, 5.678558825948272215 ) ) ;
#14158=EDGE_CURVE ( 'NONE', #79592, #9076, #32569, .T. ) ;
#14162=CARTESIAN_POINT ( 'NONE',  ( 73.02433024948126672, 69.66517378990661769, 9.714162469163332148 ) ) ;
#14164=CARTESIAN_POINT ( 'NONE',  ( 67.41069134358542669, 70.04696837240071261, -4.305487806446024446E-08 ) ) ;
#14170=EDGE_CURVE ( 'NONE', #93753, #14510, #91813, .T. ) ;
#14179=AXIS2_PLACEMENT_3D ( 'NONE', #80388, #25652, #10447 ) ;
#14182=B_SPLINE_CURVE_WITH_KNOTS ( 'NONE', 3,
 ( #64774, #17156, #11084, #10573, #64262, #48054, #40447, #41448, #26766, #86129, #1970, #16659, #2999, #33888, #47553, #9067, #70873, #63261, #94202, #24757, #58637, #4973, #90097, #51554, #20666, #36848, #65748, #52055, #98681, #13571, #5462 ),
 .UNSPECIFIED., .F., .F.,
 ( 4, 3, 3, 3, 3, 3, 3, 3, 3, 3, 4 ),
 ( 0.000000000000000000, 0.1333490885032346807, 0.3007194338854402571, 0.4699862290245250818, 0.5844252810809306142, 0.6686540514502837818, 0.7354980260655518132, 0.8028463152565542549, 0.8633854507757066088, 0.9437142632667097075, 1.000000000000000000 ),
 .UNSPECIFIED. ) ;
#14185=CARTESIAN_POINT ( 'NONE',  ( 66.45490466085416870, 67.84821477620812402, 6.733515886304859421 ) ) ;
#14188=CARTESIAN_POINT ( 'NONE',  ( 81.40581815559377787, 55.82057330830384956, 16.38440887150438385 ) ) ;
#14190=CARTESIAN_POINT ( 'NONE',  ( 71.50375327671149250, 66.90100933989515397, 11.02690240348687212 ) ) ;
#14203=VERTEX_POINT ( 'NONE', #80970 ) ;
#14207=CARTESIAN_POINT ( 'NONE',  ( 73.06720963123042623, 70.70023934857047720, 7.647115370324644168 ) ) ;
#14208=CARTESIAN_POINT ( 'NONE',  ( 69.98405410183003994, 67.38768254928731949, -9.599236973523137095 ) ) ;
#14211=CARTESIAN_POINT ( 'NONE',  ( 72.46615884746773872, 71.21309588215865460, -6.079728238972058385 ) ) ;
#14213=CARTESIAN_POINT ( 'NONE',  ( 80.92950541471338965, 51.12517857173720159, 14.80259026963665470 ) ) ;
#14214=CARTESIAN_POINT ( 'NONE',  ( 73.59632604377750908, 69.25558887711068223, -10.00338666068682691 ) ) ;
#14217=B_SPLINE_CURVE_WITH_KNOTS ( 'NONE', 3,
 ( #25718, #33300, #66569, #97495, #44250, #89906, #87584, #18109, #90421, #20994 ),
 .UNSPECIFIED., .F., .F.,
 ( 4, 2, 2, 2, 4 ),
 ( 0.000000000000000000, 0.2500000000000000000, 0.5000000000000000000, 0.7500000000000000000, 1.000000000000000000 ),
 .UNSPECIFIED. ) ;
#14218=CARTESIAN_POINT ( 'NONE',  ( 70.77025480411006697, 71.48656028203394897, 1.095472859252403897 ) ) ;
#14226=CARTESIAN_POINT ( 'NONE',  ( 20.44744908501035852, 27.50829794293881037, -10.00000000000000355 ) ) ;
#14227=DIRECTION ( 'NONE',  ( 0.8660254037844399289, 0.4999999999999977240, -0.000000000000000000 ) ) ;
#14231=CARTESIAN_POINT ( 'NONE',  ( 72.30698315258602804, 72.02217937971185791, -3.539662339715687889 ) ) ;
#14237=CARTESIAN_POINT ( 'NONE',  ( 72.78592982716214976, 70.27025758361958196, -8.090204238294326444 ) ) ;
#14240=CARTESIAN_POINT ( 'NONE',  ( 31.96529204653334588, 20.58380873178789017, 6.180339887498953466 ) ) ;
#14241=CARTESIAN_POINT ( 'NONE',  ( 85.12553491092469926, 49.00280835124235779, 12.44658997562346769 ) ) ;
#14243=CARTESIAN_POINT ( 'NONE',  ( 72.06167755366938366, 71.78506459024572450, -3.928121392008132151 ) ) ;
#14245=B_SPLINE_SURFACE_WITH_KNOTS ( 'NONE', 3, 1, ( 
 ( #21295, #59254 ),
 ( #58765, #29389 ),
 ( #59769, #52169 ),
 ( #98302, #67886 ),
 ( #5580, #28892 ),
 ( #6081, #66387 ),
 ( #5092, #97316 ),
 ( #35973, #20802 ),
 ( #89735, #51695 ),
 ( #43060, #76012 ),
 ( #74003, #4589 ),
 ( #66875, #36974 ),
 ( #20297, #83118 ),
 ( #6590, #44561 ),
 ( #60258, #21777 ),
 ( #52666, #83621 ),
 ( #14188, #37463 ),
 ( #78494, #92232 ),
 ( #15157, #85631 ),
 ( #39448, #479 ),
 ( #93206, #99790 ),
 ( #23762, #93718 ),
 ( #39950, #16176 ),
 ( #38960, #32374 ),
 ( #84616, #91715 ),
 ( #1491, #85112 ),
 ( #30379, #86142 ),
 ( #61262, #7572 ),
 ( #22783, #24279 ),
 ( #53660, #100293 ),
 ( #70369, #76493 ) ),
 .UNSPECIFIED., .F., .F., .F.,
 ( 4, 3, 3, 3, 3, 3, 3, 3, 3, 3, 4 ),
 ( 2, 2 ),
 ( 0.000000000000000000, 0.1333490885032341255, 0.3007194338854348725, 0.4699862290245032659, 0.5844252810809253962, 0.6686540514502775645, 0.7354980260655532565, 0.8028463152565672445, 0.8633854507757174890, 0.9437142632667334663, 1.000000000000000000 ),
 ( 0.000000000000000000, 1.000000000000000000 ),
 .UNSPECIFIED. ) ;
#14253=CARTESIAN_POINT ( 'NONE',  ( 71.24258803893445702, 70.28559471200580333, -7.340107459681124880 ) ) ;
#14255=CARTESIAN_POINT ( 'NONE',  ( 36.29711636232130445, 39.14336893147758900, 7.433330006724141015 ) ) ;
#14260=CARTESIAN_POINT ( 'NONE',  ( 21.59269996301512862, 13.26216523072493914, -2.296566073217252530E-15 ) ) ;
#14261=CARTESIAN_POINT ( 'NONE',  ( 14.99119413235835729, 10.78380873178785571, -6.180339887498949025 ) ) ;
#14262=CARTESIAN_POINT ( 'NONE',  ( 71.49559693922878978, 59.13754170620860862, 15.79921231626542699 ) ) ;
#14264=ORIENTED_EDGE ( 'NONE', *, *, #13845, .T. ) ;
#14267=CARTESIAN_POINT ( 'NONE',  ( 88.00349997577261263, 44.64923112938744509, 4.253506518527974123 ) ) ;
#14268=CARTESIAN_POINT ( 'NONE',  ( 81.60392558426443088, 42.57997742557506626, 7.507547604040053280 ) ) ;
#14269=ORIENTED_EDGE ( 'NONE', *, *, #26875, .T. ) ;
#14271=CARTESIAN_POINT ( 'NONE',  ( 82.32225094544060084, 40.36431351492650776, 1.323353720485960672 ) ) ;
#14272=CARTESIAN_POINT ( 'NONE',  ( 76.95450487289042485, 63.82793267849404373, 14.93104742799489593 ) ) ;
#14281=CARTESIAN_POINT ( 'NONE',  ( 71.74963559588888984, 69.27730147043639874, 9.283338642638904403 ) ) ;
#14284=B_SPLINE_CURVE_WITH_KNOTS ( 'NONE', 3,
 ( #48246, #79191, #18356, #55812, #3175, #9767, #57828, #24936, #17861, #25962, #42130, #49249, #34060, #19373, #71563, #3658, #26455, #2659, #1665, #56331, #87327, #33551, #40627, #96379, #81187, #63940, #48759, #32548, #72058, #64951, #79691, #10253, #95405, #95895, #49740, #10753, #41629, #26943, #80693, #63447, #72571, #73062, #57330, #88303, #94382, #18858 ),
 .UNSPECIFIED., .F., .F.,
 ( 4, 1, 1, 1, 2, 2, 1, 1, 1, 2, 2, 1, 1, 2, 2, 1, 1, 2, 2, 1, 1, 2, 2, 1, 2, 2, 1, 2, 2, 4 ),
 ( 0.000000000000000000, 0.06250000000002038647, 0.09375000000003029521, 0.1093750000000349165, 0.1171875000000369843, 0.1250000000000390521, 0.1875000000000338896, 0.2187500000000316136, 0.2343750000000324463, 0.2421875000000331679, 0.2500000000000338618, 0.3125000000000286438, 0.3437500000000238698, 0.3593750000000215383, 0.3750000000000191513, 0.4375000000000183187, 0.4687500000000181521, 0.4843750000000158762, 0.5000000000000135447, 0.5625000000000096589, 0.5937500000000056621, 0.6093750000000056621, 0.6250000000000056621, 0.6875000000000015543, 0.7187499999999994449, 0.7499999999999972244, 0.8124999999999938938, 0.8437499999999943379, 0.8749999999999947820, 1.000000000000000000 ),
 .UNSPECIFIED. ) ;
#14285=ORIENTED_EDGE ( 'NONE', *, *, #83999, .F. ) ;
#14286=CARTESIAN_POINT ( 'NONE',  ( 87.60166352820709790, 45.45111633860030054, -6.741156191458166802 ) ) ;
#14291=EDGE_LOOP ( 'NONE', ( #1446, #34230, #47266, #22383 ) ) ;
#14298=VERTEX_POINT ( 'NONE', #11034 ) ;
#14301=CARTESIAN_POINT ( 'NONE',  ( 83.61215227093727265, 52.34510252200112035, 14.76249278255550657 ) ) ;
#14316=CARTESIAN_POINT ( 'NONE',  ( 66.97123670830937670, 67.01180370489193194, 8.614194428613410892 ) ) ;
#14322=CARTESIAN_POINT ( 'NONE',  ( 72.15493168869993212, 69.90749124128198844, 8.044790318638545656 ) ) ;
#14327=CARTESIAN_POINT ( 'NONE',  ( 69.54903494467576763, 65.01932103406771546, -11.65098723592027063 ) ) ;
#14332=FACE_OUTER_BOUND ( 'NONE', #92038, .T. ) ;
#14348=CARTESIAN_POINT ( 'NONE',  ( 81.76046516772940720, 41.68411953923578039, -5.589761987555794676 ) ) ;
#14350=DIRECTION ( 'NONE',  ( -0.8660254037844378194, -0.5000000000000014433, -0.000000000000000000 ) ) ;
#14354=EDGE_LOOP ( 'NONE', ( #88705, #96598, #55475, #19963 ) ) ;
#14356=CARTESIAN_POINT ( 'NONE',  ( 79.25252407528779486, 59.49743072449277292, -16.53464936128684926 ) ) ;
#14357=AXIS2_PLACEMENT_3D ( 'NONE', #80187, #17339, #2160 ) ;
#14362=CARTESIAN_POINT ( 'NONE',  ( 15.40662013169548672, 9.864269794150882120, -3.090169943749474069 ) ) ;
#14366=CARTESIAN_POINT ( 'NONE',  ( 73.10017469210082197, 69.78597432261236122, 9.621008654245756020 ) ) ;
#14370=CARTESIAN_POINT ( 'NONE',  ( 73.13476967714909449, 57.39438153525127007, 15.88807208273859395 ) ) ;
#14372=CARTESIAN_POINT ( 'NONE',  ( 66.43183815540312764, 68.23408033485772251, -4.371383677469295570 ) ) ;
#14380=CARTESIAN_POINT ( 'NONE',  ( 21.92109465949963720, 30.84336893147756697, -7.433330006724137462 ) ) ;
#14382=DIRECTION ( 'NONE',  ( -0.4493970231495795775, 0.7783784768652820540, -0.4383711467890876734 ) ) ;
#14384=CARTESIAN_POINT ( 'NONE',  ( 70.98241741224116197, 71.33924828472395063, 4.661226392503834859 ) ) ;
#14386=CARTESIAN_POINT ( 'NONE',  ( 68.75657388079734744, 64.08238207491497462, 12.00962459721684894 ) ) ;
#14392=CARTESIAN_POINT ( 'NONE',  ( 7.993722094130166766, 16.56628583063838533, 9.188101187500006262 ) ) ;
#14394=ORIENTED_EDGE ( 'NONE', *, *, #93100, .F. ) ;
#14397=ADVANCED_FACE ( 'NONE', ( #45392, #44392, #21131, #28708, #99620, #29217, #7390, #84441, #76322, #60084, #6897, #21614, #69191, #59586, #67202, #52494, #13524, #90562, #44887 ), #6414, .T. ) ;
#14406=CARTESIAN_POINT ( 'NONE',  ( 9.331744567327184825, 27.16126292948893806, -6.180339887498951690 ) ) ;
#14407=CARTESIAN_POINT ( 'NONE',  ( 72.52317797754714945, 70.67061044535299175, 7.191400705033394125 ) ) ;
#14410=CARTESIAN_POINT ( 'NONE',  ( 86.13879346367242817, 46.95025718893441535, -10.63009676298478823 ) ) ;
#14411=CARTESIAN_POINT ( 'NONE',  ( 86.74128215123107566, 44.99823344504448386, -6.819724595823730695 ) ) ;
#14412=ORIENTED_EDGE ( 'NONE', *, *, #51965, .T. ) ;
#14415=CARTESIAN_POINT ( 'NONE',  ( 79.24569797405095528, 59.88260215966532485, -16.14197575274306828 ) ) ;
#14418=CARTESIAN_POINT ( 'NONE',  ( 69.85710753323976974, 62.58612235388682876, 13.43716744926057061 ) ) ;
#14424=CARTESIAN_POINT ( 'NONE',  ( 81.38143055733745257, 42.03490022094371170, -7.845107503210293487 ) ) ;
#14429=CARTESIAN_POINT ( 'NONE',  ( 80.69421300080995252, 47.47854041208089626, 13.01832096680326600 ) ) ;
#14437=CARTESIAN_POINT ( 'NONE',  ( 69.58285789709184144, 68.44046384883969836, -7.877954211123528339 ) ) ;
#14439=CARTESIAN_POINT ( 'NONE',  ( 77.04509665064642832, 61.98795237192920382, 15.49868876593534495 ) ) ;
#14440=CARTESIAN_POINT ( 'NONE',  ( 13.45569633750675465, 25.95586893147754282, 7.433330006724141015 ) ) ;
#14442=CARTESIAN_POINT ( 'NONE',  ( 80.47095457055254997, 57.75622231085856129, 16.59751886879109151 ) ) ;
#14443=VECTOR ( 'NONE', #21793, 1000.000000000000114 ) ;
#14445=ORIENTED_EDGE ( 'NONE', *, *, #81125, .F. ) ;
#14449=CARTESIAN_POINT ( 'NONE',  ( 77.38344707992527560, 49.10671604805792612, -15.27628165681131200 ) ) ;
#14456=B_SPLINE_CURVE_WITH_KNOTS ( 'NONE', 3,
 ( #78815, #16492, #54469, #23578, #53975, #30705, #55474 ),
 .UNSPECIFIED., .F., .F.,
 ( 4, 2, 1, 4 ),
 ( 0.7443881330833320709, 0.8082910998124995805, 0.8721940665416672012, 1.000000000000000000 ),
 .UNSPECIFIED. ) ;
#14459=CARTESIAN_POINT ( 'NONE',  ( 82.87527646796823433, 53.57285545580594999, -15.34456322816472706 ) ) ;
#14462=CARTESIAN_POINT ( 'NONE',  ( 72.11017239049232330, 72.33233329575897130, 0.8941507534055238571 ) ) ;
#14472=ADVANCED_FACE ( 'NONE', ( #52008 ), #83947, .T. ) ;
#14473=CARTESIAN_POINT ( 'NONE',  ( 81.39417835958199987, 46.77585984559194543, -12.26216018662527318 ) ) ;
#14474=CARTESIAN_POINT ( 'NONE',  ( 85.68543549478557964, 42.81554016910153848, 1.675580183874652018 ) ) ;
#14476=CARTESIAN_POINT ( 'NONE',  ( 83.29938471922254450, 44.25013702680151795, 8.630921364687216268 ) ) ;
#14481=CARTESIAN_POINT ( 'NONE',  ( 65.81099121317393497, 68.96265426817872424, 2.147452934379848521 ) ) ;
#14483=DIRECTION ( 'NONE',  ( -0.1378186779084930869, 0.2387089523694814197, -0.9612616959383223358 ) ) ;
#14484=B_SPLINE_CURVE_WITH_KNOTS ( 'NONE', 3,
 ( #68892, #30402, #99819, #31887, #61295, #7601, #85145, #45590, #69893, #91242 ),
 .UNSPECIFIED., .F., .F.,
 ( 4, 2, 2, 2, 4 ),
 ( 0.000000000000000000, 0.2500000000000000000, 0.5000000000000000000, 0.7500000000000000000, 1.000000000000000000 ),
 .UNSPECIFIED. ) ;
#14490=EDGE_CURVE ( 'NONE', #87546, #3917, #85739, .T. ) ;
#14502=CARTESIAN_POINT ( 'NONE',  ( 66.07943095046397275, 68.55699243926717656, 2.188521597562036902 ) ) ;
#14503=CARTESIAN_POINT ( 'NONE',  ( 82.89325122283835867, 42.00608085941690462, -4.768917158401198009 ) ) ;
#14507=CARTESIAN_POINT ( 'NONE',  ( 42.04415689841856363, 29.98920272979930246, 7.433330006724137462 ) ) ;
#14510=VERTEX_POINT ( 'NONE', #32190 ) ;
#14511=CARTESIAN_POINT ( 'NONE',  ( 25.90481151690805106, 33.14336893147756768, 7.433330006724141015 ) ) ;
#14519=CARTESIAN_POINT ( 'NONE',  ( 70.86521028213462614, 60.91151414948516418, 14.54696446430460810 ) ) ;
#14520=CARTESIAN_POINT ( 'NONE',  ( 76.03824915322937272, 65.38513206480712370, -14.40956150002899783 ) ) ;
#14527=CARTESIAN_POINT ( 'NONE',  ( 73.46598367719339251, 69.88918780369783690, 9.751349427452053575 ) ) ;
#14533=FACE_OUTER_BOUND ( 'NONE', #48826, .T. ) ;
#14534=EDGE_CURVE ( 'NONE', #71177, #36219, #14456, .T. ) ;
#14539=EDGE_CURVE ( 'NONE', #34466, #4961, #46895, .T. ) ;
#14540=CARTESIAN_POINT ( 'NONE',  ( 35.45274159363147959, 38.65586893147759184, -7.433330006724137462 ) ) ;
#14541=CARTESIAN_POINT ( 'NONE',  ( 81.59924320624311633, 55.92250459863397083, -16.38315390958105411 ) ) ;
#14545=CARTESIAN_POINT ( 'NONE',  ( 71.21219703145997926, 63.67509445150784586, -13.83477564754000788 ) ) ;
#14551=CARTESIAN_POINT ( 'NONE',  ( 87.15508732983295204, 45.91009000376428872, -8.663677684674611967 ) ) ;
#14552=FACE_OUTER_BOUND ( 'NONE', #46879, .T. ) ;
#14555=CARTESIAN_POINT ( 'NONE',  ( 70.16456968396876448, 70.84923341515788309, 4.730100017123507250 ) ) ;
#14559=CARTESIAN_POINT ( 'NONE',  ( 77.08113471857714671, 63.57880127914461355, -15.41835532793242791 ) ) ;
#14564=CARTESIAN_POINT ( 'NONE',  ( 39.38594668318775405, 31.24335787977766188, -9.188101187500008038 ) ) ;
#14568=B_SPLINE_CURVE_WITH_KNOTS ( 'NONE', 3,
 ( #46430, #38339, #75380, #52547, #99172, #53052, #60139, #5963, #13576, #44946, #83499, #36856, #22662, #84008, #54029, #30760, #53544, #45444, #69743, #37840, #91099, #21667, #30255, #61140, #67766, #76378, #77359, #84984, #6951, #44447, #75889 ),
 .UNSPECIFIED., .F., .F.,
 ( 4, 3, 3, 3, 3, 3, 3, 3, 3, 3, 4 ),
 ( 0.000000000000000000, 0.1333490885032349860, 0.3007194338854367599, 0.4699862290245074292, 0.5844252810809225096, 0.6686540514502804511, 0.7354980260655492597, 0.8028463152565746830, 0.8633854507757233732, 0.9437142632667367970, 1.000000000000000000 ),
 .UNSPECIFIED. ) ;
#14569=CARTESIAN_POINT ( 'NONE',  ( 86.92574391271591594, 45.77938117786232652, -8.666101563913320760 ) ) ;
#14570=LINE ( 'NONE', #84011, #78747 ) ;
#14578=ORIENTED_EDGE ( 'NONE', *, *, #20011, .T. ) ;
#14579=CYLINDRICAL_SURFACE ( 'NONE', #74268, 10.00000000000001066 ) ;
#14582=CARTESIAN_POINT ( 'NONE',  ( 69.55679667848153258, 71.27692851584133393, -0.5916159062426952220 ) ) ;
#14584=CARTESIAN_POINT ( 'NONE',  ( 69.72818323148324282, 63.14936655818974032, -13.63905201428613090 ) ) ;
#14588=CARTESIAN_POINT ( 'NONE',  ( 73.17451026478642007, 68.08244569788803346, 10.88860031406959727 ) ) ;
#14589=CARTESIAN_POINT ( 'NONE',  ( 82.62224726316846102, 40.93996069151095440, -3.627884205396067596 ) ) ;
#14592=CARTESIAN_POINT ( 'NONE',  ( 71.66453512356649469, 72.11062924793525042, 3.341973230705638898 ) ) ;
#14593=CARTESIAN_POINT ( 'NONE',  ( 84.87297731598476958, 46.29707946066870505, 10.07320804996537689 ) ) ;
#14597=CARTESIAN_POINT ( 'NONE',  ( 82.66575685400569284, 54.08976349579732812, -15.88644314918171574 ) ) ;
#14605=CARTESIAN_POINT ( 'NONE',  ( 65.72708745793390506, 69.07493967346769637, -0.1118595723326069880 ) ) ;
#14608=CARTESIAN_POINT ( 'NONE',  ( 81.35748880148537410, 42.22347387491733173, -7.155507324468848296 ) ) ;
#14610=CARTESIAN_POINT ( 'NONE',  ( 39.30595310148520838, 34.64441083166263979, -10.00000000000000533 ) ) ;
#14613=LINE ( 'NONE', #84546, #67321 ) ;
#14614=ADVANCED_FACE ( 'NONE', ( #79349 ), #17860, .T. ) ;
#14618=CARTESIAN_POINT ( 'NONE',  ( 80.07311184616966671, 50.58256448429610685, -14.76394167379344857 ) ) ;
#14621=CARTESIAN_POINT ( 'NONE',  ( 21.69737781089059681, 21.03085787977762777, 9.188101187500006262 ) ) ;
#14624=CARTESIAN_POINT ( 'NONE',  ( 10.31635424878816742, 24.14336893147753926, 7.433330006724141015 ) ) ;
#14626=CARTESIAN_POINT ( 'NONE',  ( 76.92864961180355010, 63.84291323147403574, 14.92053277014489687 ) ) ;
#14637=CARTESIAN_POINT ( 'NONE',  ( 77.07931261141762036, 49.50410267394570951, 15.47847711487539257 ) ) ;
#14642=ORIENTED_EDGE ( 'NONE', *, *, #97048, .T. ) ;
#14651=CARTESIAN_POINT ( 'NONE',  ( 22.22900788544320605, 15.76004757982089544, 5.678558825948272215 ) ) ;
#14652=CARTESIAN_POINT ( 'NONE',  ( 68.77081067755379706, 69.84697089389068481, -3.678078207114283238 ) ) ;
#14659=AXIS2_PLACEMENT_3D ( 'NONE', #62915, #3154, #41099 ) ;
#14663=CARTESIAN_POINT ( 'NONE',  ( 68.11396990062021928, 66.09066184282977474, -10.54551009860708355 ) ) ;
#14675=ORIENTED_EDGE ( 'NONE', *, *, #14170, .F. ) ;
#14677=VERTEX_POINT ( 'NONE', #91418 ) ;
#14679=CARTESIAN_POINT ( 'NONE',  ( 66.43852593890612468, 67.87665097547890980, 6.658925527579347303 ) ) ;
#14683=CARTESIAN_POINT ( 'NONE',  ( 67.81833433099461672, 65.48244593839081062, 10.25897341332929003 ) ) ;
#14689=EDGE_CURVE ( 'NONE', #86588, #7077, #86052, .T. ) ;
#14690=CARTESIAN_POINT ( 'NONE',  ( 76.22774175637606220, 51.62333717891167595, -16.17666187944767486 ) ) ;
#14691=PLANE ( 'NONE',  #22310 ) ;
#14695=VERTEX_POINT ( 'NONE', #9399 ) ;
#14696=CARTESIAN_POINT ( 'NONE',  ( 88.25652195435415592, 44.39905568574920380, 4.349260828767086196 ) ) ;
#14700=CARTESIAN_POINT ( 'NONE',  ( 79.52159056500875067, 59.38160983241339608, -16.21114012547523231 ) ) ;
#14701=CARTESIAN_POINT ( 'NONE',  ( 69.02655799626819544, 67.42939723981996281, -8.834294664151611798 ) ) ;
#14706=CARTESIAN_POINT ( 'NONE',  ( 80.83664057472495301, 50.73597435593438831, 14.66433228262979327 ) ) ;
#14707=CARTESIAN_POINT ( 'NONE',  ( 73.34422642274553539, 69.17188908751711551, -9.931122192565558393 ) ) ;
#14709=ADVANCED_FACE ( 'NONE', ( #7908 ), #38783, .T. ) ;
#14714=FACE_BOUND ( 'NONE', #10895, .T. ) ;
#14716=CARTESIAN_POINT ( 'NONE',  ( 28.54179425266445591, 16.28848085856231975, 1.475505719884397138E-15 ) ) ;
#14719=CARTESIAN_POINT ( 'NONE',  ( 16.01772687902244741, 32.18080186712592905, 3.090169943749475401 ) ) ;
#14727=CARTESIAN_POINT ( 'NONE',  ( 66.46588474414394909, 67.86938339201618930, -6.704488035472810914 ) ) ;
#14728=CARTESIAN_POINT ( 'NONE',  ( 73.11028533216558856, 70.59594333518880660, -7.866013523829703757 ) ) ;
#14732=CARTESIAN_POINT ( 'NONE',  ( 24.34009904141853653, 32.79103043416549923, 8.090169943749478065 ) ) ;
#14733=CARTESIAN_POINT ( 'NONE',  ( 84.12761100671502845, 42.09295748728150954, -2.591167056789191125 ) ) ;
#14745=CARTESIAN_POINT ( 'NONE',  ( 73.27328646083023500, 70.16270934360544231, -9.274526489422589393 ) ) ;
#14746=CARTESIAN_POINT ( 'NONE',  ( 30.83975393042360835, 33.50829794293883168, -10.00000000000000355 ) ) ;
#14747=CARTESIAN_POINT ( 'NONE',  ( 36.01387044229257128, 42.83396525600393545, -2.839279412974133887 ) ) ;
#14750=DIRECTION ( 'NONE',  ( -0.8660254037844379305, -0.5000000000000014433, -0.000000000000000000 ) ) ;
#14753=CARTESIAN_POINT ( 'NONE',  ( 18.36860284018464995, 32.64646525600389992, -2.839279412974133887 ) ) ;
#14755=CARTESIAN_POINT ( 'NONE',  ( 71.40405452044859658, 59.30247739756921987, 15.23691996167968910 ) ) ;
#14757=EDGE_LOOP ( 'NONE', ( #29867, #53360, #89007, #11659, #56206, #27423 ) ) ;
#14760=CARTESIAN_POINT ( 'NONE',  ( 75.18500952680872729, 53.63335195952274148, -16.53975160506809772 ) ) ;
#14761=CARTESIAN_POINT ( 'NONE',  ( 81.54911411804300769, 41.98910540586440021, 7.610088923344967782 ) ) ;
#14762=DIRECTION ( 'NONE',  ( 0.5242119900219298634, 0.000000000000000000, 0.8515878049369003389 ) ) ;
#14763=ORIENTED_EDGE ( 'NONE', *, *, #32108, .F. ) ;
#14765=CARTESIAN_POINT ( 'NONE',  ( 72.39511741677974044, 71.78066914166659274, -5.650358525013035482 ) ) ;
#14775=CARTESIAN_POINT ( 'NONE',  ( 28.02677306626161879, 24.38052372038642091, 10.00000000000000533 ) ) ;
#14777=CARTESIAN_POINT ( 'NONE',  ( 65.92723761088207368, 68.94945291059251247, -2.624861928015910895 ) ) ;
#14785=ORIENTED_EDGE ( 'NONE', *, *, #96460, .T. ) ;
#14791=CARTESIAN_POINT ( 'NONE',  ( 78.52645726747817889, 47.93368687526088934, -14.49719720932383638 ) ) ;
#14795=CARTESIAN_POINT ( 'NONE',  ( 72.55458512285707684, 59.16573985917453626, -15.46293891684866040 ) ) ;
#14803=CARTESIAN_POINT ( 'NONE',  ( 69.12388524367867149, 65.75570191728738223, 10.77047642910910952 ) ) ;
#14805=CARTESIAN_POINT ( 'NONE',  ( 67.12926300868817009, 66.68692061479262634, 8.295177568791400446 ) ) ;
#14807=CARTESIAN_POINT ( 'NONE',  ( 78.18799119024448885, 47.74668810756791970, 13.95283994106731207 ) ) ;
#14810=CARTESIAN_POINT ( 'NONE',  ( 79.10982015350863605, 53.18341928809535091, -15.72547263405508744 ) ) ;
#14812=CARTESIAN_POINT ( 'NONE',  ( 78.98931672906337553, 46.17816290900251630, 12.77312729586772555 ) ) ;
#14819=CARTESIAN_POINT ( 'NONE',  ( 72.58296766565817393, 71.54644804895973209, 5.445337812415410816 ) ) ;
#14828=ORIENTED_EDGE ( 'NONE', *, *, #61593, .T. ) ;
#14833=FACE_BOUND ( 'NONE', #65518, .T. ) ;
#14836=CARTESIAN_POINT ( 'NONE',  ( 84.14312167556933275, 48.98415679381830756, 0.000000000000000000 ) ) ;
#14838=CARTESIAN_POINT ( 'NONE',  ( 68.53315363119618553, 64.54459275260778384, -12.18798101231200448 ) ) ;
#14842=ORIENTED_EDGE ( 'NONE', *, *, #85523, .T. ) ;
#14843=EDGE_CURVE ( 'NONE', #52194, #50951, #4777, .T. ) ;
#14845=CARTESIAN_POINT ( 'NONE',  ( 79.60268825639580825, 47.69515478760800420, -14.06140264647798510 ) ) ;
#14847=CARTESIAN_POINT ( 'NONE',  ( 2.709347677296586987, 25.65659080271448644, -1.878358725466461243E-16 ) ) ;
#14850=CARTESIAN_POINT ( 'NONE',  ( 73.19096742874920380, 69.77356361390103245, 9.106933955064157260 ) ) ;
#14854=CARTESIAN_POINT ( 'NONE',  ( 74.25393038840245197, 55.45593832152543712, 16.12141555578006091 ) ) ;
#14855=CARTESIAN_POINT ( 'NONE',  ( 69.03518170984699509, 64.49507618471645287, 12.45339560606362461 ) ) ;
#14861=CARTESIAN_POINT ( 'NONE',  ( 33.82173346387272517, 28.03085787977764909, 9.188101187500006262 ) ) ;
#14864=DIRECTION ( 'NONE',  ( -0.2033683215378938036, 0.3522442655536374700, -0.9135454576426059736 ) ) ;
#14867=CARTESIAN_POINT ( 'NONE',  ( 68.99533790586593796, 64.15022810885204763, 12.06270211734473463 ) ) ;
#14869=CARTESIAN_POINT ( 'NONE',  ( 75.36487073175837281, 53.53173320265494084, -16.04382577248123809 ) ) ;
#14871=CARTESIAN_POINT ( 'NONE',  ( 73.37932691289753961, 66.58465441985281075, -12.76502462501827395 ) ) ;
#14880=CARTESIAN_POINT ( 'NONE',  ( 67.32333946482658860, 68.49528494984309646, 5.140773697818922017 ) ) ;
#14885=VERTEX_POINT ( 'NONE', #49396 ) ;
#14887=CARTESIAN_POINT ( 'NONE',  ( 71.24177335598133709, 70.40240055988557799, 7.130317524929912665 ) ) ;
#14895=CARTESIAN_POINT ( 'NONE',  ( 69.40688464331348939, 62.76167709611338097, 13.18428418677036795 ) ) ;
#14903=B_SPLINE_CURVE_WITH_KNOTS ( 'NONE', 3,
 ( #41411, #91782, #22348, #18641, #19649, #82481, #43906, #88092, #73339, #33852, #64737, #80980, #11044, #4419, #41921, #11546, #50026, #58599, #49520, #72857, #2960, #96663, #26234, #3446 ),
 .UNSPECIFIED., .F., .F.,
 ( 4, 2, 2, 2, 2, 2, 2, 2, 2, 2, 2, 4 ),
 ( 0.000000000000000000, 0.1250000000000058009, 0.2500000000000116018, 0.3750000000000174305, 0.4375000000000157097, 0.5000000000000139888, 0.5625000000000122125, 0.6250000000000104361, 0.6875000000000086597, 0.7500000000000068834, 0.8750000000000035527, 1.000000000000000000 ),
 .UNSPECIFIED. ) ;
#14905=CARTESIAN_POINT ( 'NONE',  ( 80.99519602156757969, 48.45934176588340847, 13.51949272217580500 ) ) ;
#14907=CARTESIAN_POINT ( 'NONE',  ( 69.29937091505746594, 69.83787342855333691, 4.724315302973998598 ) ) ;
#14914=CARTESIAN_POINT ( 'NONE',  ( 68.37595286067593747, 68.37058859125058063, -6.769880321061123141 ) ) ;
#14916=CARTESIAN_POINT ( 'NONE',  ( 13.17245041747802148, 29.64646525600389637, -2.839279412974133887 ) ) ;
#14919=CYLINDRICAL_SURFACE ( 'NONE', #8832, 10.00000000000001066 ) ;
#14924=CARTESIAN_POINT ( 'NONE',  ( 82.79116273540778081, 45.87476224633662980, -10.81090643298098897 ) ) ;
#14929=CARTESIAN_POINT ( 'NONE',  ( 72.21059398248078764, 63.10797502098981937, -13.93913043402019447 ) ) ;
#14935=CARTESIAN_POINT ( 'NONE',  ( 86.48597344569623147, 44.64948832258973255, -6.340490538666154308 ) ) ;
#14936=CARTESIAN_POINT ( 'NONE',  ( 72.82183928371372872, 70.95611737677427300, 7.748181657111714138 ) ) ;
#14938=CARTESIAN_POINT ( 'NONE',  ( 76.20595068776574976, 65.19451524589622693, 14.14378227490007056 ) ) ;
#14941=ORIENTED_EDGE ( 'NONE', *, *, #87572, .F. ) ;
#14944=CARTESIAN_POINT ( 'NONE',  ( 67.37294101383669442, 67.25214370961325017, -8.602411162679397094 ) ) ;
#14945=CARTESIAN_POINT ( 'NONE',  ( 85.87487879953339132, 42.95715103324309325, 1.964983386555947842 ) ) ;
#14947=( BOUNDED_CURVE ( )  B_SPLINE_CURVE ( 2, ( #74144, #74649, #21420, #82274, #43707, #67008, #97933, #28508, #59389, #90365, #52306, #44692, #90869 ),
 .UNSPECIFIED., .F., .T. ) 
 B_SPLINE_CURVE_WITH_KNOTS ( ( 3, 2, 2, 2, 2, 2, 3 ),
 ( 0.7875000000000000888, 0.7900000000000000355, 0.7950000000000000400, 0.8000000000000000444, 0.8050000000000000488, 0.8100000000000000533, 0.8125000000000000000 ),
 .UNSPECIFIED. ) 
 CURVE ( )  GEOMETRIC_REPRESENTATION_ITEM ( )  RATIONAL_B_SPLINE_CURVE ( ( 0.9755282581475767101, 0.9755282581475772652, 1.000000000000000000, 0.9510565162951535312, 1.000000000000000000, 0.9510565162951535312, 1.000000000000000000, 0.9510565162951535312, 1.000000000000000000, 0.9510565162951535312, 1.000000000000000000, 0.9755282581475768211, 0.9755282581475768211 ) ) 
 REPRESENTATION_ITEM ( '' )  );
#14961=CARTESIAN_POINT ( 'NONE',  ( 68.90560621877193626, 63.79076715805909004, -12.30144644517787711 ) ) ;
#14963=CARTESIAN_POINT ( 'NONE',  ( 82.83468505418072425, 48.81772959092904784, 13.64447714929874067 ) ) ;
#14964=CARTESIAN_POINT ( 'NONE',  ( 70.98683038387876820, 61.11472152276905234, -14.49225651734632692 ) ) ;
#14965=CARTESIAN_POINT ( 'NONE',  ( 73.21854134910928735, 68.38249955197431973, 11.21855355596820480 ) ) ;
#14968=CARTESIAN_POINT ( 'NONE',  ( 72.06470348997973474, 72.25603645428110156, 1.367373202405273602 ) ) ;
#14975=CARTESIAN_POINT ( 'NONE',  ( 14.33134397731654630, 13.98920272979924917, 7.433330006724137462 ) ) ;
#14976=CARTESIAN_POINT ( 'NONE',  ( 77.18523492127140173, 59.47428895107222502, -16.40887739104300991 ) ) ;
#14984=CARTESIAN_POINT ( 'NONE',  ( 36.18707552304946518, 42.93396525600392977, 2.839279412974139660 ) ) ;
#14988=CARTESIAN_POINT ( 'NONE',  ( 28.23826220571969969, 31.70171378149920471, -9.188101187500004485 ) ) ;
#14999=CARTESIAN_POINT ( 'NONE',  ( 73.03785937943386841, 69.69865149502336976, 9.683281169778272357 ) ) ;
#15000=CARTESIAN_POINT ( 'NONE',  ( 33.10965510200716722, 34.51421378149920827, -9.188101187500004485 ) ) ;
#15003=CARTESIAN_POINT ( 'NONE',  ( 87.27998730159347929, 43.91877473756031947, 2.943096442281895264 ) ) ;
#15011=CARTESIAN_POINT ( 'NONE',  ( 81.49256741308062146, 59.57505144466710334, 0.05226423163382182269 ) ) ;
#15012=CARTESIAN_POINT ( 'NONE',  ( 81.30975366074838462, 56.24313983998633404, -16.44754541364716971 ) ) ;
#15013=EDGE_CURVE ( 'NONE', #44296, #22415, #26106, .T. ) ;
#15021=DIRECTION ( 'NONE',  ( 0.8845109580947929651, -0.1124011590738235450, 0.4527762631246172731 ) ) ;
#15025=CARTESIAN_POINT ( 'NONE',  ( 77.10851993703164453, 59.99585613907493098, -15.93770053271873621 ) ) ;
#15026=CARTESIAN_POINT ( 'NONE',  ( 82.42863484518792916, 40.95299279291557326, 1.014380864406314808 ) ) ;
#15029=CARTESIAN_POINT ( 'NONE',  ( 77.05758262809833070, 63.67252911167651774, -14.99652361060851646 ) ) ;
#15032=VERTEX_POINT ( 'NONE', #96537 ) ;
#15034=CARTESIAN_POINT ( 'NONE',  ( 35.45274159363147959, 38.65586893147759184, -7.433330006724137462 ) ) ;
#15041=DIRECTION ( 'NONE',  ( 0.000000000000000000, 0.6788029332000655724, -0.7343204871709539949 ) ) ;
#15044=CARTESIAN_POINT ( 'NONE',  ( 13.35896364390118052, 31.21091486745859811, -1.111400068045478839E-16 ) ) ;
#15049=LINE ( 'NONE', #89269, #55849 ) ;
#15062=B_SPLINE_SURFACE_WITH_KNOTS ( 'NONE', 3, 1, ( 
 ( #89912, #91399 ),
 ( #5280, #59951 ),
 ( #52359, #90426 ),
 ( #74701, #36159 ),
 ( #28564, #35672 ),
 ( #83307, #84308 ),
 ( #67063, #97986 ),
 ( #68557, #37163 ),
 ( #28068, #13386 ),
 ( #20492, #91908 ),
 ( #13868, #44748 ),
 ( #52857, #68062 ),
 ( #21964, #82332 ),
 ( #51363, #76193 ),
 ( #98985, #83808 ),
 ( #29569, #60444 ),
 ( #22464, #14372 ),
 ( #45258, #6768 ),
 ( #37646, #99483 ),
 ( #30058, #1169 ),
 ( #17354, #69559 ),
 ( #8269, #15340 ),
 ( #55828, #46235 ),
 ( #63461, #46758 ),
 ( #92403, #62435 ),
 ( #71079, #7761 ),
 ( #165, #76665 ),
 ( #86822, #70047 ),
 ( #77160, #1680 ),
 ( #38655, #92891 ),
 ( #77686, #8760 ) ),
 .UNSPECIFIED., .F., .F., .F.,
 ( 4, 3, 3, 3, 3, 3, 3, 3, 3, 3, 4 ),
 ( 2, 2 ),
 ( 0.000000000000000000, 0.1122669598086808440, 0.2243161639709783939, 0.3396355846219274444, 0.4553962076585297836, 0.5677860799922560542, 0.6749047109689785273, 0.7773884377078629226, 0.8775581155834549785, 0.9782364162378116568, 1.000000000000000000 ),
 ( 0.000000000000000000, 1.000000000000000000 ),
 .UNSPECIFIED. ) ;
#15063=CARTESIAN_POINT ( 'NONE',  ( 72.35643307556982506, 65.56020265574198902, 12.51768452229861772 ) ) ;
#15065=CARTESIAN_POINT ( 'NONE',  ( 82.07581200760314744, 41.13792279056817591, -3.429577836730589802 ) ) ;
#15071=EDGE_CURVE ( 'NONE', #68127, #14885, #20369, .T. ) ;
#15073=CARTESIAN_POINT ( 'NONE',  ( 73.92817530304030527, 65.74941589806995523, -13.53337586798867065 ) ) ;
#15082=CARTESIAN_POINT ( 'NONE',  ( 73.24862708662814725, 69.62355710376385787, -9.916407523326116191 ) ) ;
#15083=CARTESIAN_POINT ( 'NONE',  ( 75.88740524811866806, 51.50386128526941576, 15.70536156696038965 ) ) ;
#15088=CARTESIAN_POINT ( 'NONE',  ( 71.74723311883084875, 72.17470677413867008, 3.272391839458893781 ) ) ;
#15096=CARTESIAN_POINT ( 'NONE',  ( 24.28581821943125263, 16.94754757982089544, 5.678558825948272215 ) ) ;
#15099=CARTESIAN_POINT ( 'NONE',  ( 13.18987451683679524, 19.56628583063839244, 9.188101187500006262 ) ) ;
#15102=CARTESIAN_POINT ( 'NONE',  ( 75.58789875694216676, 56.96802034365616407, 16.56515463127572119 ) ) ;
#15104=CARTESIAN_POINT ( 'NONE',  ( 72.81957114983744361, 62.23005867720106465, 14.49872350333313697 ) ) ;
#15106=CARTESIAN_POINT ( 'NONE',  ( 79.13150298882169409, 55.44825781748590288, -16.08240833089401534 ) ) ;
#15111=CARTESIAN_POINT ( 'NONE',  ( 76.91885953472434778, 49.85770563519495369, 15.12061930091973849 ) ) ;
#15119=CARTESIAN_POINT ( 'NONE',  ( 79.09330386122300638, 46.17864056469723977, -12.73155772710657452 ) ) ;
#15122=EDGE_LOOP ( 'NONE', ( #95573, #82669, #4592, #37798 ) ) ;
#15123=CARTESIAN_POINT ( 'NONE',  ( 24.30746885452586525, 16.96004757982090183, -5.678558825948275768 ) ) ;
#15124=CARTESIAN_POINT ( 'NONE',  ( 75.59055352145890083, 57.67694070126884753, 16.07306487193169531 ) ) ;
#15130=ORIENTED_EDGE ( 'NONE', *, *, #84448, .T. ) ;
#15133=CARTESIAN_POINT ( 'NONE',  ( 67.70227059457259600, 65.68093037200397077, -10.72427208149578881 ) ) ;
#15151=ORIENTED_EDGE ( 'NONE', *, *, #68316, .F. ) ;
#15153=CARTESIAN_POINT ( 'NONE',  ( 67.06310037049678385, 67.63674953590368943, 6.653793825411979945 ) ) ;
#15155=EDGE_CURVE ( 'NONE', #90942, #83096, #76208, .T. ) ;
#15156=CARTESIAN_POINT ( 'NONE',  ( 82.20453289287176801, 41.97260302554307287, -6.936896895868616575 ) ) ;
#15157=CARTESIAN_POINT ( 'NONE',  ( 81.35074466249913883, 55.80872010294902452, 16.38725056492407361 ) ) ;
#15163=CARTESIAN_POINT ( 'NONE',  ( 24.82038151633537026, 14.73415679381822230, 1.333680081654574804E-15 ) ) ;
#15166=CARTESIAN_POINT ( 'NONE',  ( 76.09110705058404278, 51.50373584443451591, -16.16844731949881719 ) ) ;
#15172=CARTESIAN_POINT ( 'NONE',  ( 84.75572546936606955, 43.74292620480390781, -6.422790150011197241 ) ) ;
#15176=CARTESIAN_POINT ( 'NONE',  ( 72.65255621578388912, 70.92891038547531934, 7.631180297043458793 ) ) ;
#15178=CARTESIAN_POINT ( 'NONE',  ( 72.23816834301878487, 67.09684945540639944, -11.28492405425373768 ) ) ;
#15184=CARTESIAN_POINT ( 'NONE',  ( 81.39610991623023040, 53.46539056111136290, 15.50635795318955701 ) ) ;
#15185=CARTESIAN_POINT ( 'NONE',  ( 84.06604358195920668, 51.46910565605918464, 14.65639964578790888 ) ) ;
#15193=CARTESIAN_POINT ( 'NONE',  ( 82.47021907082941539, 53.30441442868470858, -15.33472904691311456 ) ) ;
#15195=CARTESIAN_POINT ( 'NONE',  ( 73.90603277580463271, 55.10673587672410889, 16.60184368115057651 ) ) ;
#15198=CARTESIAN_POINT ( 'NONE',  ( 23.71749583336532297, 25.64441083166261492, -10.00000000000000533 ) ) ;
#15206=B_SPLINE_CURVE_WITH_KNOTS ( 'NONE', 3,
 ( #98994, #60959, #99492, #38146, #61462, #21007, #59454, #52866, #83817, #76676 ),
 .UNSPECIFIED., .F., .F.,
 ( 4, 2, 2, 2, 4 ),
 ( 0.000000000000000000, 0.2500000000000000000, 0.5000000000000000000, 0.7500000000000000000, 1.000000000000000000 ),
 .UNSPECIFIED. ) ;
#15208=CARTESIAN_POINT ( 'NONE',  ( 72.44129552685038220, 70.67501955208014408, -7.848061272651219333 ) ) ;
#15213=CARTESIAN_POINT ( 'NONE',  ( 26.07214984898741150, 33.79103043416550634, 8.090169943749478065 ) ) ;
#15216=PLANE ( 'NONE',  #52303 ) ;
#15221=CARTESIAN_POINT ( 'NONE',  ( 34.14357333472769085, 43.21091486745863364, 7.012934429366973338E-14 ) ) ;
#15224=CARTESIAN_POINT ( 'NONE',  ( 66.93805147409950962, 68.00539448811831278, 6.966594628907381903 ) ) ;
#15225=ADVANCED_FACE ( 'NONE', ( #7271 ), #88701, .T. ) ;
#15234=CARTESIAN_POINT ( 'NONE',  ( 18.13223351794271565, 28.65586893147756342, -7.433330006724137462 ) ) ;
#15240=CARTESIAN_POINT ( 'NONE',  ( 81.62555094951984813, 42.60298488570899877, 7.525266644112702075 ) ) ;
#15242=ORIENTED_EDGE ( 'NONE', *, *, #95173, .F. ) ;
#15245=CARTESIAN_POINT ( 'NONE',  ( 71.12243608386381766, 71.25991561840170618, -3.643341247755859325 ) ) ;
#15246=CARTESIAN_POINT ( 'NONE',  ( 76.93391092271131981, 63.83843569504302451, 14.92315812435476019 ) ) ;
#15252=ORIENTED_EDGE ( 'NONE', *, *, #19172, .T. ) ;
#15254=CARTESIAN_POINT ( 'NONE',  ( 81.91486247953744737, 58.84361493377822683, 0.3596699001693273168 ) ) ;
#15255=CARTESIAN_POINT ( 'NONE',  ( 80.01151941643857413, 58.12832627190487500, 16.26807764006944979 ) ) ;
#15264=CARTESIAN_POINT ( 'NONE',  ( 74.60601093365112035, 63.68499727765737362, 14.35797525815900144 ) ) ;
#15269=EDGE_CURVE ( 'NONE', #89471, #13779, #44989, .T. ) ;
#15271=CARTESIAN_POINT ( 'NONE',  ( 34.29273532275193759, 21.92755873383628185, 6.180339887498953466 ) ) ;
#15273=CARTESIAN_POINT ( 'NONE',  ( 83.14160737058271877, 52.20232750492525753, 14.81664504224666778 ) ) ;
#15274=VERTEX_POINT ( 'NONE', #53587 ) ;
#15277=CARTESIAN_POINT ( 'NONE',  ( 86.95487931624934674, 46.48160929640930306, 8.961892044152525827 ) ) ;
#15278=CARTESIAN_POINT ( 'NONE',  ( 82.07407170904370730, 42.67750543218616599, -7.226825756593194150 ) ) ;
#15288=CARTESIAN_POINT ( 'NONE',  ( 74.01371779070863965, 64.71087909724029430, -13.67405404575846184 ) ) ;
#15289=CARTESIAN_POINT ( 'NONE',  ( 77.96593341510595110, 47.91059554715139512, 14.09972309609993424 ) ) ;
#15292=CARTESIAN_POINT ( 'NONE',  ( 82.87719117936363489, 41.29838300305157617, -1.984818766237280485 ) ) ;
#15293=CARTESIAN_POINT ( 'NONE',  ( 87.37223321024185907, 44.84069173413745091, -6.683519980512460101 ) ) ;
#15294=CARTESIAN_POINT ( 'NONE',  ( 78.92186904685135573, 46.24801581213586132, 12.84669794032027212 ) ) ;
#15296=CARTESIAN_POINT ( 'NONE',  ( 83.61754957953866096, 52.24592005514148951, -14.70745080183155906 ) ) ;
#15301=CARTESIAN_POINT ( 'NONE',  ( 72.50318959249285911, 71.67715071215087619, 6.033079537162486794 ) ) ;
#15310=CARTESIAN_POINT ( 'NONE',  ( 68.56611454130262473, 66.34273538077306398, -9.815413640989422817 ) ) ;
#15312=CARTESIAN_POINT ( 'NONE',  ( 71.88285097721950478, 66.11705595339820718, 11.91407432373335240 ) ) ;
#15313=CARTESIAN_POINT ( 'NONE',  ( 74.40645258968876874, 67.99769933107435804, -11.66855138296962480 ) ) ;
#15318=VECTOR ( 'NONE', #36728, 1000.000000000000114 ) ;
#15320=LINE ( 'NONE', #70030, #33761 ) ;
#15322=CARTESIAN_POINT ( 'NONE',  ( 42.57599984984017993, 32.78052372038644791, -10.00000000000000355 ) ) ;
#15323=ORIENTED_EDGE ( 'NONE', *, *, #66396, .T. ) ;
#15331=CARTESIAN_POINT ( 'NONE',  ( 8.736352098677466316, 26.81751292744054638, -6.180339887498951690 ) ) ;
#15334=CARTESIAN_POINT ( 'NONE',  ( 73.07852875935716952, 69.76346136681742394, 9.633212380859575319 ) ) ;
#15338=CARTESIAN_POINT ( 'NONE',  ( 73.03390162335675484, 57.22514805668252080, 15.90373071166581020 ) ) ;
#15340=CARTESIAN_POINT ( 'NONE',  ( 66.58138301798484804, 68.33132062184148481, -4.336431400097447764 ) ) ;
#15345=CARTESIAN_POINT ( 'NONE',  ( 23.88951478931043937, 35.83396525600391413, -2.839279412974133887 ) ) ;
#15349=CARTESIAN_POINT ( 'NONE',  ( 88.18856786306730555, 43.91052089632135136, 2.508363019901202140 ) ) ;
#15351=CARTESIAN_POINT ( 'NONE',  ( 68.68990518416599400, 64.09702660386993500, 11.96895164568068104 ) ) ;
#15353=CARTESIAN_POINT ( 'NONE',  ( 80.40629399489428408, 48.06278861952080916, 14.00309965006242230 ) ) ;
#15354=CARTESIAN_POINT ( 'NONE',  ( 0.000000000000000000, 0.000000000000000000, 0.000000000000000000 ) ) ;
#15357=CARTESIAN_POINT ( 'NONE',  ( 13.89351337401799391, 10.94754757982088123, 5.678558825948272215 ) ) ;
#15360=AXIS2_PLACEMENT_3D ( 'NONE', #96940, #42668, #27506 ) ;
#15364=LINE ( 'NONE', #38162, #55271 ) ;
#15371=VERTEX_POINT ( 'NONE', #77914 ) ;
#15373=CARTESIAN_POINT ( 'NONE',  ( 23.52344096658254102, 21.78052372038640883, -10.00000000000000355 ) ) ;
#15375=EDGE_LOOP ( 'NONE', ( #17623, #22369, #68101, #82286 ) ) ;
#15377=CARTESIAN_POINT ( 'NONE',  ( 79.48567122603782309, 59.58331865380349512, -16.19020142938439477 ) ) ;
#15378=CARTESIAN_POINT ( 'NONE',  ( 8.320926099340340443, 27.73705186507752174, -3.090169943749475845 ) ) ;
#15380=CARTESIAN_POINT ( 'NONE',  ( 69.57577311412531174, 62.66348738126951901, 13.87209483570389779 ) ) ;
#15390=ORIENTED_EDGE ( 'NONE', *, *, #63166, .F. ) ;
#15391=CARTESIAN_POINT ( 'NONE',  ( 72.80832253034486712, 58.87847187791489745, 15.58086070995311978 ) ) ;
#15395=CARTESIAN_POINT ( 'NONE',  ( 69.98230802859291089, 70.60635815750532629, 3.580953781081825493 ) ) ;
#15398=CARTESIAN_POINT ( 'NONE',  ( 82.75467282439718986, 47.54992309942269912, 12.26659463265117900 ) ) ;
#15404=CARTESIAN_POINT ( 'NONE',  ( 82.65530164897143095, 54.02391170524479946, -15.49949047637507782 ) ) ;
#15405=CARTESIAN_POINT ( 'NONE',  ( 78.32669662580138947, 55.90372456675076762, -16.57385434309017924 ) ) ;
#15406=CARTESIAN_POINT ( 'NONE',  ( 17.03285546273658113, 12.76004757982088655, 5.678558825948272215 ) ) ;
#15408=CARTESIAN_POINT ( 'NONE',  ( 80.74762043199122274, 57.32811249769932971, 16.57232535949600916 ) ) ;
#15413=CARTESIAN_POINT ( 'NONE',  ( 45.05398624838444022, 26.41603393254328935, -1.583844403245362020 ) ) ;
#15414=CARTESIAN_POINT ( 'NONE',  ( 80.30437888069963037, 44.85419571244045045, 11.14874347110982988 ) ) ;
#15415=CARTESIAN_POINT ( 'NONE',  ( 67.80205187238352948, 65.98368644125179117, -10.46800807810757483 ) ) ;
#15424=CARTESIAN_POINT ( 'NONE',  ( 82.66995253617540129, 53.27399894339424691, -15.29269040213952913 ) ) ;
#15427=CARTESIAN_POINT ( 'NONE',  ( 72.67799729538583620, 70.93760247754363490, 7.641220802698788894 ) ) ;
#15436=CARTESIAN_POINT ( 'NONE',  ( 85.74869351040513266, 46.00941097376583855, -9.208016345952161785 ) ) ;
#15439=CARTESIAN_POINT ( 'NONE',  ( 82.78295361368475369, 43.37803873317465531, 7.757655889806053473 ) ) ;
#15443=DIRECTION ( 'NONE',  ( 0.000000000000000000, -0.4385670422228087340, -0.8986984752829710876 ) ) ;
#15445=DIRECTION ( 'NONE',  ( 0.5000000000000014433, -0.8660254037844378194, 0.000000000000000000 ) ) ;
#15453=CARTESIAN_POINT ( 'NONE',  ( 82.64400278703348590, 48.09335400213094402, 13.25860807430423272 ) ) ;
#15458=CARTESIAN_POINT ( 'NONE',  ( 69.22118451730979416, 69.17181481221663830, 6.156610956507596377 ) ) ;
#15463=CARTESIAN_POINT ( 'NONE',  ( 74.30578394237890905, 58.31684474416242381, 16.33455613536389350 ) ) ;
#15466=EDGE_CURVE ( 'NONE', #18179, #29839, #64196, .T. ) ;
#15468=CARTESIAN_POINT ( 'NONE',  ( 16.65397613197454518, 21.56628583063840310, 9.188101187500006262 ) ) ;
#15471=CARTESIAN_POINT ( 'NONE',  ( 66.49460505587296666, 68.77342561816206512, 2.322209999061914498 ) ) ;
#15475=CARTESIAN_POINT ( 'NONE',  ( 77.32817876982271343, 63.13942984521013813, 15.61058464551962288 ) ) ;
#15477=CARTESIAN_POINT ( 'NONE',  ( 35.32779635548150310, 39.13478043621390867, 8.090169943749478065 ) ) ;
#15481=CARTESIAN_POINT ( 'NONE',  ( 28.93108252874724684, 32.10171378149919974, 9.188101187500008038 ) ) ;
#15494=CARTESIAN_POINT ( 'NONE',  ( 30.49295849316677831, 39.64646525600392835, -2.839279412974133887 ) ) ;
#15495=ORIENTED_EDGE ( 'NONE', *, *, #73942, .F. ) ;
#15499=CARTESIAN_POINT ( 'NONE',  ( 86.51873334781436142, 47.12553361672021879, -10.58414027450333528 ) ) ;
#15501=CARTESIAN_POINT ( 'NONE',  ( 85.04850917506151120, 49.90949791588273143, 13.51477744872044262 ) ) ;
#15503=CARTESIAN_POINT ( 'NONE',  ( 88.41177868068123757, 44.08414425260226466, -2.750064808092239410 ) ) ;
#15505=DIRECTION ( 'NONE',  ( 0.8660254037844380415, 0.5000000000000012212, 0.000000000000000000 ) ) ;
#15506=CARTESIAN_POINT ( 'NONE',  ( 81.44563236102617054, 56.14986361120382696, -16.42609089136781009 ) ) ;
#15507=CARTESIAN_POINT ( 'NONE',  ( 71.40858655494352547, 63.62864610033815183, -13.92573448899003274 ) ) ;
#15519=CARTESIAN_POINT ( 'NONE',  ( 82.80834019656774103, 40.61763827593378551, 0.9796441576777050741 ) ) ;
#15521=EDGE_CURVE ( 'NONE', #73618, #43232, #10500, .T. ) ;
#15526=CARTESIAN_POINT ( 'NONE',  ( 43.56148901884012048, 27.01110640527296169, 2.839279412974134775 ) ) ;
#15528=ORIENTED_EDGE ( 'NONE', *, *, #46843, .F. ) ;
#15530=CARTESIAN_POINT ( 'NONE',  ( 86.84459937989694822, 45.86515160798009560, -8.194834137214424885 ) ) ;
#15531=CARTESIAN_POINT ( 'NONE',  ( 74.77113966951148427, 63.06429047545149302, -14.66048351875234523 ) ) ;
#15534=CARTESIAN_POINT ( 'NONE',  ( 72.46461309515387939, 63.44911742965013701, 13.84624394093605027 ) ) ;
#15535=CARTESIAN_POINT ( 'NONE',  ( 66.77752810875767864, 68.40544692769400115, 4.459354299965320401 ) ) ;
#15537=ORIENTED_EDGE ( 'NONE', *, *, #24439, .T. ) ;
#15538=CARTESIAN_POINT ( 'NONE',  ( 29.80052344588228408, 32.90829794293883026, 10.00000000000000355 ) ) ;
#15539=( BOUNDED_CURVE ( )  B_SPLINE_CURVE ( 2, ( #87162, #49576, #80529, #49091, #3506, #55659, #95236, #72415, #33907, #65281, #96222, #64795, #94721 ),
 .UNSPECIFIED., .F., .T. ) 
 B_SPLINE_CURVE_WITH_KNOTS ( ( 3, 2, 2, 2, 2, 2, 3 ),
 ( 0.5875000000000000222, 0.5899999999999999689, 0.5949999999999999734, 0.5999999999999999778, 0.6049999999999999822, 0.6099999999999999867, 0.6125000000000000444 ),
 .UNSPECIFIED. ) 
 CURVE ( )  GEOMETRIC_REPRESENTATION_ITEM ( )  RATIONAL_B_SPLINE_CURVE ( ( 0.9755282581475767101, 0.9755282581475772652, 1.000000000000000000, 0.9510565162951535312, 1.000000000000000000, 0.9510565162951535312, 1.000000000000000000, 0.9510565162951535312, 1.000000000000000000, 0.9510565162951535312, 1.000000000000000000, 0.9755282581475761550, 0.9755282581475767101 ) ) 
 REPRESENTATION_ITEM ( '' )  );
#15542=FACE_OUTER_BOUND ( 'NONE', #7173, .T. ) ;
#15544=FACE_OUTER_BOUND ( 'NONE', #20807, .T. ) ;
#15549=DIRECTION ( 'NONE',  ( 0.7235470741700457120, 0.1663964660674585594, 0.6699192843471722947 ) ) ;
#15550=CARTESIAN_POINT ( 'NONE',  ( 69.62688595351798426, 63.12627229902661696, -13.61770258999189309 ) ) ;
#15560=CARTESIAN_POINT ( 'NONE',  ( 83.37188637347107090, 43.51478601198282803, 7.417674380252161193 ) ) ;
#15562=CARTESIAN_POINT ( 'NONE',  ( 73.97124227054526102, 68.60621492378263042, 10.89700218101527085 ) ) ;
#15564=CARTESIAN_POINT ( 'NONE',  ( 82.66149664020484522, 53.53843108144140928, -15.73363621927586742 ) ) ;
#15566=CARTESIAN_POINT ( 'NONE',  ( 67.16503064337793205, 66.61400111815741809, 8.426382589595288408 ) ) ;
#15575=LINE ( 'NONE', #31285, #84145 ) ;
#15576=CARTESIAN_POINT ( 'NONE',  ( 73.09452573934707686, 69.60050248057373778, -9.839270276345128963 ) ) ;
#15589=CARTESIAN_POINT ( 'NONE',  ( 88.53016884517781193, 43.88792164385783678, -0.09627500500477706447 ) ) ;
#15590=CARTESIAN_POINT ( 'NONE',  ( 4.654322096184512425, 26.18528772668515714, -1.583844403245363575 ) ) ;
#15594=CARTESIAN_POINT ( 'NONE',  ( 30.20304716546516133, 19.29860640527293469, -2.839279412974138328 ) ) ;
#15597=CARTESIAN_POINT ( 'NONE',  ( 16.58301002715608519, 15.28920272979925876, -7.433330006724141015 ) ) ;
#15599=CARTESIAN_POINT ( 'NONE',  ( 77.22913030991912819, 63.42231615505745879, 15.12051831926749834 ) ) ;
#15600=CARTESIAN_POINT ( 'NONE',  ( 74.14312167556930433, 66.30466486950707861, 1.224646799147354045E-15 ) ) ;
#15606=CARTESIAN_POINT ( 'NONE',  ( 77.04458465457972238, 56.18878383020774692, -16.16646171855996172 ) ) ;
#15607=CARTESIAN_POINT ( 'NONE',  ( 87.65828818788342858, 45.19712344130779513, -6.201442590288507972 ) ) ;
#15612=CARTESIAN_POINT ( 'NONE',  ( 77.32596066893822240, 49.50693989401381856, 14.91615350571074927 ) ) ;
#15617=CARTESIAN_POINT ( 'NONE',  ( 70.66454081066896720, 68.90461880718730470, -8.132011908148811585 ) ) ;
#15618=EDGE_LOOP ( 'NONE', ( #32380, #66362, #40554, #3637 ) ) ;
#15625=CARTESIAN_POINT ( 'NONE',  ( 28.45357225853751260, 28.37878583063842441, 9.188101187500006262 ) ) ;
#15626=CARTESIAN_POINT ( 'NONE',  ( 75.76995552607449724, 58.63049212716732228, 15.98588464947494892 ) ) ;
#15630=EDGE_CURVE ( 'NONE', #59206, #98946, #84458, .T. ) ;
#15637=CARTESIAN_POINT ( 'NONE',  ( 67.83068094623702393, 65.48536241154209847, 10.26294962280224965 ) ) ;
#15648=VERTEX_POINT ( 'NONE', #25586 ) ;
#15659=CARTESIAN_POINT ( 'NONE',  ( 66.78892157389906004, 67.90037632253439881, 7.001642916364290592 ) ) ;
#15660=EDGE_CURVE ( 'NONE', #65907, #50908, #91619, .T. ) ;
#15663=B_SPLINE_SURFACE_WITH_KNOTS ( 'NONE', 3, 1, ( 
 ( #94438, #94940 ),
 ( #24992, #8802 ),
 ( #25504, #17919 ),
 ( #18925, #88367 ),
 ( #41183, #72120 ),
 ( #64509, #33612 ),
 ( #56889, #49799 ),
 ( #41690, #18419 ),
 ( #49309, #72633 ),
 ( #34117, #95954 ),
 ( #26515, #57392 ),
 ( #39670, #70598 ),
 ( #32088, #93945 ),
 ( #20920, #81737 ),
 ( #66493, #12822 ),
 ( #74116, #3719 ),
 ( #98413, #74625 ),
 ( #19437, #43173 ),
 ( #89837, #80761 ),
 ( #59877, #51280 ),
 ( #90844, #44173 ),
 ( #82249, #27515 ),
 ( #5198, #66982 ),
 ( #36577, #4710 ),
 ( #27989, #27011 ),
 ( #19915, #59365 ),
 ( #67483, #50786 ),
 ( #35596, #96444 ),
 ( #57895, #97420 ),
 ( #11820, #73609 ),
 ( #82745, #58385 ) ),
 .UNSPECIFIED., .F., .F., .F.,
 ( 4, 3, 3, 3, 3, 3, 3, 3, 3, 3, 4 ),
 ( 2, 2 ),
 ( 0.000000000000000000, 0.1122669598086764586, 0.2243161639709642108, 0.3396355846219141217, 0.4553962076585162944, 0.5677860799922443968, 0.6749047109689607638, 0.7773884377078399410, 0.8775581155834293323, 0.9782364162377974459, 1.000000000000000000 ),
 ( 0.000000000000000000, 1.000000000000000000 ),
 .UNSPECIFIED. ) ;
#15665=CARTESIAN_POINT ( 'NONE',  ( 84.38804523167981131, 47.38734847442095344, -11.44389121885481764 ) ) ;
#15666=CARTESIAN_POINT ( 'NONE',  ( 70.39359452487714464, 63.86253493995260300, 12.85482810418176491 ) ) ;
#15670=CARTESIAN_POINT ( 'NONE',  ( 15.64201941024748521, 32.52903772873357724, -1.583844403245363575 ) ) ;
#15674=CARTESIAN_POINT ( 'NONE',  ( 75.96213316711562413, 65.70078031631311433, -14.22672748915905316 ) ) ;
#15682=CARTESIAN_POINT ( 'NONE',  ( 82.07714787726266081, 43.65997060240250249, -8.726277158289674318 ) ) ;
#15687=CARTESIAN_POINT ( 'NONE',  ( 72.60199962089298253, 70.74354872798666349, 7.145580164668644763 ) ) ;
#15688=CARTESIAN_POINT ( 'NONE',  ( 67.90243728005769697, 67.41594138055857854, -7.898924796095583289 ) ) ;
#15693=CARTESIAN_POINT ( 'NONE',  ( 83.67218728734262356, 52.30219252426102372, 14.72955347366556111 ) ) ;
#15700=CARTESIAN_POINT ( 'NONE',  ( 73.60243789457724972, 55.52622633506491212, 16.10732509438123827 ) ) ;
#15703=CARTESIAN_POINT ( 'NONE',  ( 29.75882387383049377, 25.38052372038642091, 10.00000000000000533 ) ) ;
#15715=CARTESIAN_POINT ( 'NONE',  ( 76.95483076014906487, 63.96668203270510134, -15.25269828761453894 ) ) ;
#15718=CARTESIAN_POINT ( 'NONE',  ( 34.28597393419622819, 20.76426979415091978, 3.090169943749476733 ) ) ;
#15723=CARTESIAN_POINT ( 'NONE',  ( 83.57010898113827579, 45.17450624426406591, 10.33823738828239591 ) ) ;
#15731=CARTESIAN_POINT ( 'NONE',  ( 72.51946054628301397, 70.67701989327741785, -7.917356521280773940 ) ) ;
#15734=CYLINDRICAL_SURFACE ( 'NONE', #95264, 10.00000000000001066 ) ;
#15737=CARTESIAN_POINT ( 'NONE',  ( 22.06543860749898300, 21.24335787977763346, -9.188101187500008038 ) ) ;
#15739=CARTESIAN_POINT ( 'NONE',  ( 71.42966913292450215, 59.23173737558743568, 15.76165678759474886 ) ) ;
#15743=CARTESIAN_POINT ( 'NONE',  ( 14.52619969316804394, 14.10170272979925699, -7.433330006724141015 ) ) ;
#15744=CARTESIAN_POINT ( 'NONE',  ( 75.29051265121657366, 53.62752787197079130, -16.53442706284598174 ) ) ;
#15746=CARTESIAN_POINT ( 'NONE',  ( 81.55469672513726209, 42.53656836688637810, 7.482253779589008502 ) ) ;
#15747=EDGE_CURVE ( 'NONE', #25763, #29087, #2287, .T. ) ;
#15753=CARTESIAN_POINT ( 'NONE',  ( 85.95899798769401912, 43.49248111663925442, 5.533741676130133236 ) ) ;
#15759=CARTESIAN_POINT ( 'NONE',  ( 85.51332262388091010, 42.92838935012721180, -2.942937653912271578 ) ) ;
#15763=CARTESIAN_POINT ( 'NONE',  ( 72.84093999285123289, 56.97456911661188883, -16.40692799644482847 ) ) ;
#15773=ORIENTED_EDGE ( 'NONE', *, *, #26322, .T. ) ;
#15774=CARTESIAN_POINT ( 'NONE',  ( 26.79248755578709762, 33.65586893147757763, -7.433330006724137462 ) ) ;
#15775=DIRECTION ( 'NONE',  ( -0.8660254037844379305, -0.5000000000000014433, -0.000000000000000000 ) ) ;
#15794=VECTOR ( 'NONE', #67800, 1000.000000000000114 ) ;
#15795=CARTESIAN_POINT ( 'NONE',  ( 70.45330330358065396, 68.59310515512933648, 8.429446140656228437 ) ) ;
#15797=CARTESIAN_POINT ( 'NONE',  ( 67.52858891722985391, 67.09395499530575080, 8.947318060521286753 ) ) ;
#15798=CARTESIAN_POINT ( 'NONE',  ( 68.53194582573554783, 65.67665921644565685, -10.48464730244969800 ) ) ;
#15799=CARTESIAN_POINT ( 'NONE',  ( 78.40134077247404321, 47.78707627181417905, 13.91009550459359900 ) ) ;
#15804=CARTESIAN_POINT ( 'NONE',  ( 69.55597381272447421, 63.29032634764875098, 12.91558643708738252 ) ) ;
#15805=CARTESIAN_POINT ( 'NONE',  ( 87.40678246761487458, 44.84425702272720571, -6.651126967624185760 ) ) ;
#15807=DIRECTION ( 'NONE',  ( -0.8660254037844379305, -0.5000000000000014433, -0.000000000000000000 ) ) ;
#15808=CARTESIAN_POINT ( 'NONE',  ( 83.91859562547405460, 51.78473283747415934, -14.45112324054444564 ) ) ;
#15811=CARTESIAN_POINT ( 'NONE',  ( 72.13858704899024588, 72.77662068827325470, 2.033788753608857291E-15 ) ) ;
#15813=CARTESIAN_POINT ( 'NONE',  ( 72.03640812230088386, 71.62847206889918539, 5.517176230632446554 ) ) ;
#15817=AXIS2_PLACEMENT_3D ( 'NONE', #54123, #38935, #77468 ) ;
#15820=CARTESIAN_POINT ( 'NONE',  ( 82.80564809338142140, 40.64392876451551473, -1.326136484204850197 ) ) ;
#15822=CONICAL_SURFACE ( 'NONE', #14179, 10.00000000000000711, 0.7853981633974608245 ) ;
#15823=CARTESIAN_POINT ( 'NONE',  ( 85.67146519243034675, 48.43225591334719837, -12.22341872913518301 ) ) ;
#15825=CARTESIAN_POINT ( 'NONE',  ( 71.81168878175323300, 65.89568737772486884, 12.05079262845972998 ) ) ;
#15826=CARTESIAN_POINT ( 'NONE',  ( 88.06671310400491848, 44.64817415083963681, -4.178514498757152751 ) ) ;
#15832=VECTOR ( 'NONE', #81546, 1000.000000000000114 ) ;
#15838=CARTESIAN_POINT ( 'NONE',  ( 88.02404992778008364, 44.67257770573197462, 4.293538178122671134 ) ) ;
#15840=CARTESIAN_POINT ( 'NONE',  ( 9.637550907572093095, 29.65659080271449710, -1.878358725466461243E-16 ) ) ;
#15843=CARTESIAN_POINT ( 'NONE',  ( 73.20446552614963309, 69.86374744967437778, 9.599577609524185817 ) ) ;
#15847=CARTESIAN_POINT ( 'NONE',  ( 73.16956295240451880, 57.33411781474711688, 16.38320611732891408 ) ) ;
#15850=CARTESIAN_POINT ( 'NONE',  ( 17.31863740857695078, 12.12755873383625271, -6.180339887498949025 ) ) ;
#15852=ORIENTED_EDGE ( 'NONE', *, *, #62897, .T. ) ;
#15858=CARTESIAN_POINT ( 'NONE',  ( 33.49394369984602804, 21.19860640527294038, 2.839279412974134775 ) ) ;
#15862=CARTESIAN_POINT ( 'NONE',  ( 70.81858580497740263, 71.13538289942123072, 4.973410337506771306 ) ) ;
#15863=CARTESIAN_POINT ( 'NONE',  ( 66.52957814384430435, 68.80191156052306667, 2.274549643663521969 ) ) ;
#15869=CARTESIAN_POINT ( 'NONE',  ( 17.70402515066951565, 13.14754757982089117, -5.678558825948275768 ) ) ;
#15872=CARTESIAN_POINT ( 'NONE',  ( 88.29045754653738243, 44.33610290606567617, -2.255006784116474261 ) ) ;
#15873=CARTESIAN_POINT ( 'NONE',  ( 71.55389639452418749, 72.40420208557205228, 1.000837480472114294 ) ) ;
#15883=CARTESIAN_POINT ( 'NONE',  ( 72.91019467649705632, 70.83288342014805039, 7.292254455461825380 ) ) ;
#15885=CARTESIAN_POINT ( 'NONE',  ( 19.21972384509095733, 29.83478043621388309, -8.090169943749479842 ) ) ;
#15886=CARTESIAN_POINT ( 'NONE',  ( 81.87732929995556219, 45.42932287087572973, -10.88775556568189629 ) ) ;
#15889=CARTESIAN_POINT ( 'NONE',  ( 79.29973261757049841, 59.57579620614539806, -16.53044932756548846 ) ) ;
#15892=CARTESIAN_POINT ( 'NONE',  ( 14.26779446008844587, 16.43677371833800294, -10.00000000000000355 ) ) ;
#15893=CARTESIAN_POINT ( 'NONE',  ( 85.37820560265511460, 47.12669036677656464, -11.24746114250747553 ) ) ;
#15894=CARTESIAN_POINT ( 'NONE',  ( 69.95523204132881290, 62.90150226506938225, 13.86126985482015961 ) ) ;
#15900=B_SPLINE_SURFACE_WITH_KNOTS ( 'NONE', 3, 1, ( 
 ( #91029, #35789 ),
 ( #73800, #27205 ),
 ( #21113, #59059 ),
 ( #43379, #75808 ),
 ( #44376, #29198 ),
 ( #34783, #83424 ),
 ( #97140, #74818 ),
 ( #51991, #89075 ),
 ( #50483, #35290 ),
 ( #90543, #4906 ),
 ( #27709, #89549 ),
 ( #21593, #13990 ),
 ( #12008, #5889 ),
 ( #82930, #74323 ),
 ( #13506, #52476 ),
 ( #75308, #58092 ),
 ( #66197, #65684 ),
 ( #59567, #66686 ),
 ( #44869, #96640 ),
 ( #36779, #67687 ),
 ( #58576, #19625 ),
 ( #98616, #81438 ),
 ( #42866, #90030 ),
 ( #4391, #97619 ),
 ( #20111, #50980 ),
 ( #81932, #12508 ),
 ( #20604, #13016 ),
 ( #43876, #5398 ),
 ( #36282, #67181 ),
 ( #98105, #28687 ),
 ( #22580, #93516 ) ),
 .UNSPECIFIED., .F., .F., .F.,
 ( 4, 3, 3, 3, 3, 3, 3, 3, 3, 3, 4 ),
 ( 2, 2 ),
 ( 0.000000000000000000, 0.1333490885032312667, 0.3007194338854344284, 0.4699862290245184759, 0.5844252810809397181, 0.6686540514502811172, 0.7354980260655615831, 0.8028463152565572525, 0.8633854507757208196, 0.9437142632667274711, 1.000000000000000000 ),
 ( 0.000000000000000000, 1.000000000000000000 ),
 .UNSPECIFIED. ) ;
#15902=EDGE_CURVE ( 'NONE', #89249, #36835, #34886, .T. ) ;
#15905=CARTESIAN_POINT ( 'NONE',  ( 74.55670760492021998, 66.78977310388269473, 12.65506860017463175 ) ) ;
#15911=CARTESIAN_POINT ( 'NONE',  ( 82.57448465555356165, 47.03648843181296257, 11.94445601533793422 ) ) ;
#15918=CARTESIAN_POINT ( 'NONE',  ( 14.66813190280496570, 26.65586893147755276, -7.433330006724137462 ) ) ;
#15921=CARTESIAN_POINT ( 'NONE',  ( 80.02165461388095480, 57.57226732806288538, 16.59957571444259017 ) ) ;
#15928=CARTESIAN_POINT ( 'NONE',  ( 68.04067724501535963, 66.09559063115733579, -10.49573481652158335 ) ) ;
#15939=CARTESIAN_POINT ( 'NONE',  ( 82.47990923055493795, 40.99821503651507015, -1.212878302331509728 ) ) ;
#15944=CARTESIAN_POINT ( 'NONE',  ( 72.42968441479126795, 70.75204143367579945, 7.711333220305022884 ) ) ;
#15946=CARTESIAN_POINT ( 'NONE',  ( 75.69465226566293836, 65.43705427022661070, 14.28313312794709589 ) ) ;
#15955=AXIS2_PLACEMENT_3D ( 'NONE', #20006, #12917, #74721 ) ;
#15960=FACE_OUTER_BOUND ( 'NONE', #45661, .T. ) ;
#15971=CARTESIAN_POINT ( 'NONE',  ( 72.46146760938286491, 66.06259922122619344, 12.76239748237539473 ) ) ;
#15972=CARTESIAN_POINT ( 'NONE',  ( 74.05623475345210238, 67.87786276047000911, -11.59565021290446651 ) ) ;
#15975=CARTESIAN_POINT ( 'NONE',  ( 71.06456094586361871, 71.36015830129700532, 3.098779000439031428 ) ) ;
#15980=EDGE_CURVE ( 'NONE', #94954, #43596, #71164, .T. ) ;
#15983=EDGE_CURVE ( 'NONE', #39764, #30496, #51573, .T. ) ;
#15985=CARTESIAN_POINT ( 'NONE',  ( 10.20631340951632104, 27.93396525600388713, 2.839279412974139660 ) ) ;
#15988=CARTESIAN_POINT ( 'NONE',  ( 12.48001537019352369, 22.90829794293879473, 10.00000000000000355 ) ) ;
#15994=CARTESIAN_POINT ( 'NONE',  ( 82.06353261700769508, 41.00057011406286733, -2.892018250819532454 ) ) ;
#15995=CARTESIAN_POINT ( 'NONE',  ( 38.43992769770077444, 34.14441083166263979, 10.00000000000000533 ) ) ;
#15997=ORIENTED_EDGE ( 'NONE', *, *, #28444, .T. ) ;
#15999=CARTESIAN_POINT ( 'NONE',  ( 70.99925208767550089, 64.35626315177518109, -13.34609736598558172 ) ) ;
#16000=CARTESIAN_POINT ( 'NONE',  ( 80.93303655709135569, 47.13181478245343925, 13.26053224286359544 ) ) ;
#16002=CARTESIAN_POINT ( 'NONE',  ( 86.10128179547638183, 47.01522930412664181, 10.71950609365847384 ) ) ;
#16004=DIRECTION ( 'NONE',  ( -0.8660254037844378194, -0.5000000000000014433, -0.000000000000000000 ) ) ;
#16006=VERTEX_POINT ( 'NONE', #63712 ) ;
#16010=CARTESIAN_POINT ( 'NONE',  ( 44.10936046141049616, 26.26216523072498887, -2.296566073217252530E-15 ) ) ;
#16015=VERTEX_POINT ( 'NONE', #47998 ) ;
#16016=AXIS2_PLACEMENT_3D ( 'NONE', #25709, #64703, #78412 ) ;
#16017=CARTESIAN_POINT ( 'NONE',  ( 86.22341231051544241, 46.94107917315361078, -10.56950783746433764 ) ) ;
#16020=CARTESIAN_POINT ( 'NONE',  ( 80.44297273216874089, 44.73620253192707708, -11.65665792466250039 ) ) ;
#16023=CARTESIAN_POINT ( 'NONE',  ( 44.74566838383860556, 28.76004757982093807, 5.678558825948272215 ) ) ;
#16025=ORIENTED_EDGE ( 'NONE', *, *, #70870, .F. ) ;
#16028=CARTESIAN_POINT ( 'NONE',  ( 77.13982593033820478, 49.36145032405385535, -14.90501067692936310 ) ) ;
#16032=CARTESIAN_POINT ( 'NONE',  ( 78.40326579531324569, 49.68334333693088212, 14.77346682042102621 ) ) ;
#16038=CARTESIAN_POINT ( 'NONE',  ( 79.25874806327021815, 46.14125615598921115, 12.64021366946045433 ) ) ;
#16049=VECTOR ( 'NONE', #14382, 1000.000000000000227 ) ;
#16054=CARTESIAN_POINT ( 'NONE',  ( 71.76582198392000578, 60.80067951720612029, 14.81518451064557063 ) ) ;
#16056=CARTESIAN_POINT ( 'NONE',  ( 78.54814453918285722, 52.73914818458334963, 16.14325216142513497 ) ) ;
#16073=CARTESIAN_POINT ( 'NONE',  ( 71.98782200592057734, 64.37985811868047392, 13.14021211575542836 ) ) ;
#16080=CARTESIAN_POINT ( 'NONE',  ( 74.40269252765078534, 68.37285155744012854, 11.32427007268841912 ) ) ;
#16081=CARTESIAN_POINT ( 'NONE',  ( 71.39461857329790462, 71.57943448657258045, -3.153141937835415742 ) ) ;
#16082=CARTESIAN_POINT ( 'NONE',  ( 67.87888135928258748, 66.79448504996196334, -9.615113643841004532 ) ) ;
#16084=PLANE ( 'NONE',  #662 ) ;
#16090=CARTESIAN_POINT ( 'NONE',  ( 78.47204957586916407, 57.63415352787896495, 16.22432601261093765 ) ) ;
#16091=CARTESIAN_POINT ( 'NONE',  ( 84.85515811532782493, 50.28810280189843240, -13.38803942659112423 ) ) ;
#16092=CARTESIAN_POINT ( 'NONE',  ( 78.00383892016681386, 61.98526604297752129, 15.67820829689503270 ) ) ;
#16093=CARTESIAN_POINT ( 'NONE',  ( 73.38763933171604492, 69.17329012685399903, -9.958834189398086068 ) ) ;
#16094=CARTESIAN_POINT ( 'NONE',  ( 75.91040063343092470, 51.47081534094227351, 15.69546924919345088 ) ) ;
#16108=CARTESIAN_POINT ( 'NONE',  ( 88.25809008468522165, 43.73205518618092214, 0.2003341539982116393 ) ) ;
#16111=PLANE ( 'NONE',  #12867 ) ;
#16112=CARTESIAN_POINT ( 'NONE',  ( 77.07877823284091789, 49.44627466125040627, 15.45926714762989995 ) ) ;
#16115=CARTESIAN_POINT ( 'NONE',  ( 23.51484842749693627, 36.68290643055188838, 3.479690158560446702E-15 ) ) ;
#16117=CARTESIAN_POINT ( 'NONE',  ( 82.21566304485764931, 47.23221333006363665, -12.24838049750184865 ) ) ;
#16118=CARTESIAN_POINT ( 'NONE',  ( 12.64980493759981250, 22.70171378149918340, -9.188101187500004485 ) ) ;
#16120=CARTESIAN_POINT ( 'NONE',  ( 77.05907617643467233, 63.75643696445189335, 14.97702801636213543 ) ) ;
#16125=CARTESIAN_POINT ( 'NONE',  ( 80.56811894275233499, 54.89951299323676182, -15.91924062418832087 ) ) ;
#16130=CARTESIAN_POINT ( 'NONE',  ( 77.26634761542135266, 49.24219256474607676, 15.35008689065183418 ) ) ;
#16131=CARTESIAN_POINT ( 'NONE',  ( 82.09463905232223624, 54.09232422927597383, 15.61698559803690145 ) ) ;
#16135=CARTESIAN_POINT ( 'NONE',  ( 69.28962944736927909, 68.84243576899710604, -6.877947330648720659 ) ) ;
#16139=CARTESIAN_POINT ( 'NONE',  ( 79.55352191442486287, 46.24377923495724474, -13.19933309463437432 ) ) ;
#16143=CARTESIAN_POINT ( 'NONE',  ( 33.16918417342686354, 21.01110640527294038, 2.839279412974134775 ) ) ;
#16144=CARTESIAN_POINT ( 'NONE',  ( 79.74329520344379318, 44.92144841624061513, 11.49897470811640332 ) ) ;
#16146=CARTESIAN_POINT ( 'NONE',  ( 75.05448840609841454, 66.98218832618682939, -13.15900604923073658 ) ) ;
#16147=ORIENTED_EDGE ( 'NONE', *, *, #31701, .F. ) ;
#16148=CARTESIAN_POINT ( 'NONE',  ( 41.60633307851366425, 35.97253583063844928, -10.00000000000000533 ) ) ;
#16151=ORIENTED_EDGE ( 'NONE', *, *, #51623, .T. ) ;
#16154=CARTESIAN_POINT ( 'NONE',  ( 67.77450396239858321, 65.65200295091629812, 10.05452136947112329 ) ) ;
#16155=CARTESIAN_POINT ( 'NONE',  ( 68.10039974585599509, 65.18542567973285884, -10.72853162865224341 ) ) ;
#16156=CARTESIAN_POINT ( 'NONE',  ( 81.42484531195619013, 55.17584661510441890, -15.93226465548353410 ) ) ;
#16165=EDGE_LOOP ( 'NONE', ( #5958, #28491, #54778, #100295 ) ) ;
#16167=CARTESIAN_POINT ( 'NONE',  ( 78.18465668123985779, 61.71620641638569538, -16.11691968629958183 ) ) ;
#16168=EDGE_CURVE ( 'NONE', #94179, #89471, #94345, .T. ) ;
#16169=ORIENTED_EDGE ( 'NONE', *, *, #50258, .F. ) ;
#16171=ORIENTED_EDGE ( 'NONE', *, *, #37885, .F. ) ;
#16173=CARTESIAN_POINT ( 'NONE',  ( 80.09120749856195687, 44.41673742825525295, -10.86461196121643979 ) ) ;
#16176=CARTESIAN_POINT ( 'NONE',  ( 81.04919588797569929, 56.11257561189316334, 16.10755627670017276 ) ) ;
#16188=CARTESIAN_POINT ( 'NONE',  ( 76.45843591644145931, 51.61599511231165138, -15.65747087338039556 ) ) ;
#16189=CARTESIAN_POINT ( 'NONE',  ( 76.24945506196253575, 64.85903190964545217, -14.33188622986231842 ) ) ;
#16212=FACE_BOUND ( 'NONE', #64423, .T. ) ;
#16215=CARTESIAN_POINT ( 'NONE',  ( 32.56068451518306262, 20.92755873383627829, 6.180339887498953466 ) ) ;
#16220=LINE ( 'NONE', #86183, #7626 ) ;
#16226=EDGE_CURVE ( 'NONE', #63171, #81636, #23739, .T. ) ;
#16231=CARTESIAN_POINT ( 'NONE',  ( 24.34009904141853653, 32.79103043416549923, 8.090169943749478065 ) ) ;
#16232=CARTESIAN_POINT ( 'NONE',  ( 34.35958382788741261, 28.03677371833804699, 10.00000000000000533 ) ) ;
#16233=CARTESIAN_POINT ( 'NONE',  ( 85.71989473008328275, 42.74111325103400105, -0.5968306828680215448 ) ) ;
#16235=CARTESIAN_POINT ( 'NONE',  ( 84.48912213214688904, 47.60039072597393073, 12.10431667099950559 ) ) ;
#16239=CARTESIAN_POINT ( 'NONE',  ( 72.88390603025270309, 66.33307502503427600, -12.19624667911425853 ) ) ;
#16242=CARTESIAN_POINT ( 'NONE',  ( 72.81630190666361102, 70.85884106002269789, -7.900673142507896429 ) ) ;
#16246=CARTESIAN_POINT ( 'NONE',  ( 67.27399870575082730, 66.42956969496371755, -8.768125640873389415 ) ) ;
#16248=DIRECTION ( 'NONE',  ( -0.2359789242578323731, -0.9717581732643756354, 0.000000000000000000 ) ) ;
#16251=CARTESIAN_POINT ( 'NONE',  ( 20.33338779993010803, 20.24335787977762990, -9.188101187500008038 ) ) ;
#16254=ORIENTED_EDGE ( 'NONE', *, *, #84044, .T. ) ;
#16256=CARTESIAN_POINT ( 'NONE',  ( 11.67313376208572961, 15.24335787977761569, -9.188101187500008038 ) ) ;
#16257=CARTESIAN_POINT ( 'NONE',  ( 76.98116725474599775, 58.55206284898313385, -16.09923721801287755 ) ) ;
#16258=CARTESIAN_POINT ( 'NONE',  ( 71.95319803722021845, 72.64445964553972601, -0.8526933041427806614 ) ) ;
#16260=CARTESIAN_POINT ( 'NONE',  ( 82.81737761406506593, 40.62361263874299055, 0.9906565629087065172 ) ) ;
#16261=CARTESIAN_POINT ( 'NONE',  ( 72.48661302258760486, 71.52526770760660213, -5.337229783571237007 ) ) ;
#16262=CARTESIAN_POINT ( 'NONE',  ( 85.41264917886874741, 49.08844855121448347, 12.38516025679438748 ) ) ;
#16263=CARTESIAN_POINT ( 'NONE',  ( 85.68486538673562336, 43.15900242217779237, 5.076191362464745893 ) ) ;
#16267=CARTESIAN_POINT ( 'NONE',  ( 84.22353192663439359, 42.61057292944220620, -4.410993892459540433 ) ) ;
#16268=ORIENTED_EDGE ( 'NONE', *, *, #23012, .F. ) ;
#16270=CARTESIAN_POINT ( 'NONE',  ( 71.85441816053061359, 72.14404838950795806, -3.648524940272755757 ) ) ;
#16271=CARTESIAN_POINT ( 'NONE',  ( 80.12977496600375105, 58.13812068622525686, 16.26683105399684237 ) ) ;
#16279=CARTESIAN_POINT ( 'NONE',  ( 82.81737761406506593, 40.62361263874299055, 0.9906565629087087377 ) ) ;
#16280=EDGE_LOOP ( 'NONE', ( #29778, #11803, #8452, #10733 ) ) ;
#16281=CARTESIAN_POINT ( 'NONE',  ( 22.20737081713591010, 33.79752408145593279, -5.678558825948271327 ) ) ;
#16286=EDGE_LOOP ( 'NONE', ( #21432, #74517, #22618, #14675 ) ) ;
#16291=VERTEX_POINT ( 'NONE', #63086 ) ;
#16292=ORIENTED_EDGE ( 'NONE', *, *, #58622, .T. ) ;
#16298=LINE ( 'NONE', #62379, #76058 ) ;
#16302=B_SPLINE_CURVE_WITH_KNOTS ( 'NONE', 3,
 ( #63512, #15905, #31099, #70098, #93955, #9317, #46286, #84851, #86878, #40191, #71639, #39183, #2233, #61505, #92454, #53892, #16408, #8810, #71132, #55882, #55388, #78728, #39678, #94450, #32098, #70606, #7818, #708, #77215, #1735, #85356, #1219, #63010, #23492, #32615, #86375, #16904, #25005, #77733, #47303, #8319, #31592, #15391, #17410, #48320, #62486 ),
 .UNSPECIFIED., .F., .F.,
 ( 4, 1, 2, 2, 1, 2, 2, 1, 1, 2, 2, 1, 1, 2, 2, 1, 1, 2, 2, 1, 1, 1, 2, 2, 1, 1, 1, 2, 2, 4 ),
 ( 0.000000000000000000, 0.06250000000001654232, 0.09375000000002257916, 0.1250000000000286160, 0.1875000000000436595, 0.2187500000000511813, 0.2500000000000586753, 0.3125000000000699441, 0.3437500000000737188, 0.3593750000000733302, 0.3750000000000729972, 0.4375000000000655032, 0.4687500000000641154, 0.4843750000000648370, 0.5000000000000656142, 0.5625000000000563993, 0.5937500000000521805, 0.6093750000000500711, 0.6250000000000478506, 0.6875000000000371925, 0.7187500000000308642, 0.7343750000000281997, 0.7421875000000267564, 0.7500000000000254241, 0.8125000000000149880, 0.8437500000000102141, 0.8593750000000084377, 0.8671875000000078826, 0.8750000000000074385, 1.000000000000000000 ),
 .UNSPECIFIED. ) ;
#16304=CARTESIAN_POINT ( 'NONE',  ( 70.14042535710315462, 67.96861681286139856, 9.010985477280877731 ) ) ;
#16305=CARTESIAN_POINT ( 'NONE',  ( 82.15890019083936124, 42.36938956976207749, -7.663980805570597354 ) ) ;
#16308=CARTESIAN_POINT ( 'NONE',  ( 78.56257306381201033, 47.97152266697279543, 13.95721769279705171 ) ) ;
#16321=ORIENTED_EDGE ( 'NONE', *, *, #96781, .T. ) ;
#16323=CARTESIAN_POINT ( 'NONE',  ( 72.31970296779593355, 71.55818645699302749, 5.058004163053099411 ) ) ;
#16327=CARTESIAN_POINT ( 'NONE',  ( 88.05624235485146301, 44.55787864911079765, -5.145732200269208079 ) ) ;
#16333=CARTESIAN_POINT ( 'NONE',  ( 70.50184245679560036, 61.65203380429616686, 14.13751713409887323 ) ) ;
#16348=CARTESIAN_POINT ( 'NONE',  ( 88.05313862314940820, 44.74715133896623342, 4.488002289119355837 ) ) ;
#16350=CARTESIAN_POINT ( 'NONE',  ( 9.964077338596862177, 24.49103043416547365, -8.090169943749479842 ) ) ;
#16353=CARTESIAN_POINT ( 'NONE',  ( 72.25139993921258963, 72.08772000594029805, 3.145145327714725880 ) ) ;
#16368=CARTESIAN_POINT ( 'NONE',  ( 29.97031301328857467, 32.70171378149920827, -9.188101187500004485 ) ) ;
#16373=CARTESIAN_POINT ( 'NONE',  ( 65.98930969947784320, 69.00056210431527859, 2.540950622023999461 ) ) ;
#16374=ORIENTED_EDGE ( 'NONE', *, *, #55451, .T. ) ;
#16379=CARTESIAN_POINT ( 'NONE',  ( 10.59179830548347745, 18.06628583063839599, -9.188101187500006262 ) ) ;
#16381=CARTESIAN_POINT ( 'NONE',  ( 88.28100378030374884, 44.27701181192854563, -1.950484388336117814 ) ) ;
#16391=CARTESIAN_POINT ( 'NONE',  ( 73.02574606114626476, 70.77724550349999788, 7.489232062110982469 ) ) ;
#16393=CARTESIAN_POINT ( 'NONE',  ( 17.41845772768865075, 33.55466486950699334, -1.111400068045478839E-16 ) ) ;
#16394=DIRECTION ( 'NONE',  ( -0.8660254037844378194, -0.5000000000000014433, -0.000000000000000000 ) ) ;
#16395=ORIENTED_EDGE ( 'NONE', *, *, #62765, .F. ) ;
#16396=CARTESIAN_POINT ( 'NONE',  ( 68.75007899452677407, 64.17077260193588018, -11.93723544003106696 ) ) ;
#16397=LINE ( 'NONE', #55376, #41083 ) ;
#16399=CARTESIAN_POINT ( 'NONE',  ( 84.89575725111018301, 47.24063678070221783, -11.59919686242552217 ) ) ;
#16400=CARTESIAN_POINT ( 'NONE',  ( 69.61300338435667356, 62.66305564137741868, 13.88455583225131917 ) ) ;
#16404=CARTESIAN_POINT ( 'NONE',  ( 31.86369474034375671, 37.13478043621390157, 8.090169943749478065 ) ) ;
#16405=ORIENTED_EDGE ( 'NONE', *, *, #38607, .T. ) ;
#16408=CARTESIAN_POINT ( 'NONE',  ( 73.92771649931930256, 63.77271023027558527, 14.14211124488107174 ) ) ;
#16417=CARTESIAN_POINT ( 'NONE',  ( 82.64074333392795779, 53.51963485226765016, -15.73164264726942640 ) ) ;
#16421=CARTESIAN_POINT ( 'NONE',  ( 26.03951966209473312, 17.96004757982090538, -5.678558825948276656 ) ) ;
#16430=CARTESIAN_POINT ( 'NONE',  ( 84.83256327216713544, 45.63739360033983417, -9.320991929122717679 ) ) ;
#16441=CARTESIAN_POINT ( 'NONE',  ( 82.12886798991216608, 40.75801620276044446, -0.7528608118565335294 ) ) ;
#16451=CARTESIAN_POINT ( 'NONE',  ( 84.56802347276283172, 46.19559949517749686, -10.17660803681333626 ) ) ;
#16452=CARTESIAN_POINT ( 'NONE',  ( 85.04462449185939477, 45.37010230792124332, 8.864637975708317796 ) ) ;
#16456=CARTESIAN_POINT ( 'NONE',  ( 74.42329672017201858, 68.02203094029241015, -11.65569731704910694 ) ) ;
#16470=EDGE_CURVE ( 'NONE', #85165, #29132, #22696, .T. ) ;
#16474=CARTESIAN_POINT ( 'NONE',  ( 80.44215978124604760, 58.39441083166273216, 0.000000000000000000 ) ) ;
#16475=CARTESIAN_POINT ( 'NONE',  ( 69.84036666288623962, 69.98366574888289904, 5.148563393720963610 ) ) ;
#16477=PLANE ( 'NONE',  #25313 ) ;
#16483=CARTESIAN_POINT ( 'NONE',  ( 11.45782370926791849, 18.56628583063839244, 9.188101187500006262 ) ) ;
#16492=CARTESIAN_POINT ( 'NONE',  ( 67.28077729273597640, 69.97196434288713363, 0.1681859604356396032 ) ) ;
#16493=VERTEX_POINT ( 'NONE', #30073 ) ;
#16497=CARTESIAN_POINT ( 'NONE',  ( 82.18936110093612513, 52.64993106124108380, 15.54926669311582188 ) ) ;
#16500=CARTESIAN_POINT ( 'NONE',  ( 75.91502559367474134, 65.16891969575354437, -14.48077610374784996 ) ) ;
#16502=DIRECTION ( 'NONE',  ( -0.4330127018922203530, 0.7500000000000046629, 0.4999999999999919509 ) ) ;
#16503=CARTESIAN_POINT ( 'NONE',  ( 74.94245617315240793, 53.14056109367614056, -16.50934518181217925 ) ) ;
#16507=CARTESIAN_POINT ( 'NONE',  ( 32.39821438149254362, 40.74646525600392977, 2.839279412974139660 ) ) ;
#16508=ORIENTED_EDGE ( 'NONE', *, *, #69063, .F. ) ;
#16509=CARTESIAN_POINT ( 'NONE',  ( 78.44787846840736734, 61.26446607870955319, 16.23792605971962999 ) ) ;
#16514=CARTESIAN_POINT ( 'NONE',  ( 86.30773806088525646, 46.95517243064260526, -10.53307507464019821 ) ) ;
#16517=CARTESIAN_POINT ( 'NONE',  ( 88.36930832042526163, 44.08004549128393990, -2.853748190838125254 ) ) ;
#16519=CARTESIAN_POINT ( 'NONE',  ( 79.36263291408793918, 45.67866562566761957, -12.88899626193393821 ) ) ;
#16522=EDGE_LOOP ( 'NONE', ( #24736, #14578, #49050, #97638 ) ) ;
#16525=CARTESIAN_POINT ( 'NONE',  ( 77.24698020313218194, 49.64373807359542212, -15.49284761250392428 ) ) ;
#16527=CARTESIAN_POINT ( 'NONE',  ( 86.97822204926990253, 45.79386009709899952, -8.643660422075560845 ) ) ;
#16528=CARTESIAN_POINT ( 'NONE',  ( 78.57569412390834884, 50.34383551948430835, 14.98634759621179136 ) ) ;
#16530=CARTESIAN_POINT ( 'NONE',  ( 80.87517248313827167, 58.64441083166272506, 0.000000000000000000 ) ) ;
#16534=CARTESIAN_POINT ( 'NONE',  ( 82.30540685579956062, 40.88228610481488801, 1.021405830961136685 ) ) ;
#16536=CARTESIAN_POINT ( 'NONE',  ( 76.94978126365660387, 62.92300403630901684, -15.24643684403981858 ) ) ;
#16542=CARTESIAN_POINT ( 'NONE',  ( 39.98734656443052415, 28.80170272979929535, 7.433330006724137462 ) ) ;
#16551=CARTESIAN_POINT ( 'NONE',  ( 80.95762699323942968, 43.02477363226272189, 9.576251469719451848 ) ) ;
#16558=DIRECTION ( 'NONE',  ( -0.4755282581475737680, 0.8236391035463299648, -0.3090169943749573878 ) ) ;
#16560=ORIENTED_EDGE ( 'NONE', *, *, #11590, .F. ) ;
#16563=CARTESIAN_POINT ( 'NONE',  ( 81.22979812886450190, 55.45288652294036780, -16.34461090620093771 ) ) ;
#16566=CARTESIAN_POINT ( 'NONE',  ( 70.18948356013267187, 71.57821204930945669, -1.478097172221414013 ) ) ;
#16574=CARTESIAN_POINT ( 'NONE',  ( 87.86584501647516277, 43.90525888894924833, 0.3790033701962610135 ) ) ;
#16578=CARTESIAN_POINT ( 'NONE',  ( 73.99564936472528132, 68.61382277044870648, 10.90295599471779120 ) ) ;
#16579=CARTESIAN_POINT ( 'NONE',  ( 69.97271289134489791, 71.02073340580969329, -1.163651360304144511 ) ) ;
#16584=CARTESIAN_POINT ( 'NONE',  ( 67.16256804578091533, 66.80979783321161847, 8.146902435796070208 ) ) ;
#16588=VECTOR ( 'NONE', #85261, 1000.000000000000114 ) ;
#16602=CARTESIAN_POINT ( 'NONE',  ( 88.23407674691928548, 43.71813397101750098, 0.1961470715255511643 ) ) ;
#16604=CARTESIAN_POINT ( 'NONE',  ( 71.92536400468701174, 72.18844424196340981, -3.635291937859653544 ) ) ;
#16605=CARTESIAN_POINT ( 'NONE',  ( 70.98065340298427373, 71.07006770911269200, -5.392052274046765348 ) ) ;
#16609=CARTESIAN_POINT ( 'NONE',  ( 24.26418115112394602, 34.98502408145593279, -5.678558825948271327 ) ) ;
#16612=CARTESIAN_POINT ( 'NONE',  ( 17.70402515066951565, 13.14754757982089295, -5.678558825948276656 ) ) ;
#16617=CARTESIAN_POINT ( 'NONE',  ( 69.53570971148970159, 62.57802854026397910, -13.90760378158714161 ) ) ;
#16619=CARTESIAN_POINT ( 'NONE',  ( 75.82058630256133824, 56.59402139164659218, -16.13716463214695906 ) ) ;
#16620=CARTESIAN_POINT ( 'NONE',  ( 87.65075002439434115, 44.95127668719692338, -6.583683359477274344 ) ) ;
#16624=ORIENTED_EDGE ( 'NONE', *, *, #30604, .T. ) ;
#16625=CARTESIAN_POINT ( 'NONE',  ( 77.42326786333445909, 49.55262521988469615, 14.91231252120838846 ) ) ;
#16630=CARTESIAN_POINT ( 'NONE',  ( 73.50461245277466560, 72.41059528448880656, 0.000000000000000000 ) ) ;
#16634=CARTESIAN_POINT ( 'NONE',  ( 72.49672817265226854, 71.70303783552662935, 5.966909785267804800 ) ) ;
#16639=CARTESIAN_POINT ( 'NONE',  ( 29.31959766232195008, 28.87878583063843152, -9.188101187500006262 ) ) ;
#16641=CARTESIAN_POINT ( 'NONE',  ( 74.94692089407369906, 66.84572622250873053, -13.20830831734917865 ) ) ;
#16642=CARTESIAN_POINT ( 'NONE',  ( 77.54361356138011274, 49.75803992512373952, -14.96129575302290249 ) ) ;
#16645=LINE ( 'NONE', #33874, #17420 ) ;
#16650=CARTESIAN_POINT ( 'NONE',  ( 67.77223724734612631, 65.62443007439019027, 10.08236501146177311 ) ) ;
#16651=CARTESIAN_POINT ( 'NONE',  ( 68.23134756035658199, 65.67744778407723061, -10.30070688804788759 ) ) ;
#16654=CARTESIAN_POINT ( 'NONE',  ( 70.79254675561878685, 71.95096862338711219, -1.204795362960673355 ) ) ;
#16659=CARTESIAN_POINT ( 'NONE',  ( 79.27109561811333549, 59.78567773455861811, 16.51039248270449278 ) ) ;
#16663=CARTESIAN_POINT ( 'NONE',  ( 77.96041703586088545, 62.15569039082562597, -15.98643159653562940 ) ) ;
#16664=ORIENTED_EDGE ( 'NONE', *, *, #98727, .F. ) ;
#16668=CARTESIAN_POINT ( 'NONE',  ( 79.90085239356115210, 44.63345658378899117, -11.16155600664863812 ) ) ;
#16673=CARTESIAN_POINT ( 'NONE',  ( 85.74833574201379349, 47.06672189974739950, -10.43935527095086613 ) ) ;
#16686=CARTESIAN_POINT ( 'NONE',  ( 75.84116199970137018, 65.13315491392486933, -14.47742810051069284 ) ) ;
#16689=CARTESIAN_POINT ( 'NONE',  ( 88.00526762198180108, 44.79707723138842113, 4.734962078095950488 ) ) ;
#16696=CARTESIAN_POINT ( 'NONE',  ( 72.52401626864599393, 70.66912915067958068, 7.194662573583692655 ) ) ;
#16701=CARTESIAN_POINT ( 'NONE',  ( 86.22410369846130607, 45.53897050033827298, 8.200890175624763856 ) ) ;
#16704=CARTESIAN_POINT ( 'NONE',  ( 68.11396990072299218, 66.09066184265174115, -10.54551009852403709 ) ) ;
#16705=ORIENTED_EDGE ( 'NONE', *, *, #88378, .T. ) ;
#16710=DIRECTION ( 'NONE',  ( -0.8660254037844379305, -0.5000000000000014433, -0.000000000000000000 ) ) ;
#16712=CARTESIAN_POINT ( 'NONE',  ( 25.26661199696083671, 36.36126292948895866, 6.180339887498949913 ) ) ;
#16715=FACE_OUTER_BOUND ( 'NONE', #27527, .T. ) ;
#16719=CARTESIAN_POINT ( 'NONE',  ( 82.88857619529979104, 50.60347501890201016, 14.14623256037462795 ) ) ;
#16725=CARTESIAN_POINT ( 'NONE',  ( 81.83010596707761408, 41.21765235792337734, 5.778278449264639960 ) ) ;
#16729=CARTESIAN_POINT ( 'NONE',  ( 25.64143417502910083, 37.73705186507756082, -3.090169943749475845 ) ) ;
#16730=CARTESIAN_POINT ( 'NONE',  ( 85.14475835685283300, 42.48365458255290150, -1.347915880835522717 ) ) ;
#16735=CARTESIAN_POINT ( 'NONE',  ( 73.16956295238907160, 57.33411781477383329, 16.38320611710937058 ) ) ;
#16739=CARTESIAN_POINT ( 'NONE',  ( 73.88098677858248209, 66.09861445257523371, -12.79634476329270498 ) ) ;
#16746=CARTESIAN_POINT ( 'NONE',  ( 67.06380573374150345, 66.82000881363511269, -8.954971976866424654 ) ) ;
#16750=CARTESIAN_POINT ( 'NONE',  ( 24.83671989960918935, 22.84335787977763488, 9.188101187500006262 ) ) ;
#16755=LINE ( 'NONE', #23345, #48437 ) ;
#16756=CARTESIAN_POINT ( 'NONE',  ( 71.50396643458246615, 72.35543200887750004, -1.254608710098219060 ) ) ;
#16759=CARTESIAN_POINT ( 'NONE',  ( 69.36456772554703321, 70.60618739324945636, -1.417523587071017444 ) ) ;
#16764=DIRECTION ( 'NONE',  ( -0.8660254037844377084, -0.5000000000000014433, -0.000000000000000000 ) ) ;
#16765=CARTESIAN_POINT ( 'NONE',  ( 85.07154897650163150, 42.80747891370868530, -3.465323602608772369 ) ) ;
#16767=CARTESIAN_POINT ( 'NONE',  ( 45.56060369728960069, 26.70852965304483106, 1.583844403245330712 ) ) ;
#16768=CARTESIAN_POINT ( 'NONE',  ( 71.71105958810139214, 72.07721142573539908, -3.586786881503329472 ) ) ;
#16770=CARTESIAN_POINT ( 'NONE',  ( 2.966658798487924908, 25.21091486745858035, 1.000260061240931054E-15 ) ) ;
#16777=DIRECTION ( 'NONE',  ( -0.4851478631379979034, 0.8403007481384877631, 0.2419218955996582654 ) ) ;
#16778=ORIENTED_EDGE ( 'NONE', *, *, #13820, .T. ) ;
#16779=CARTESIAN_POINT ( 'NONE',  ( 32.62131273085646654, 21.76004757982090965, 5.678558825948272215 ) ) ;
#16782=CARTESIAN_POINT ( 'NONE',  ( 72.44129552685039641, 70.67501955208014408, -7.848061272651214004 ) ) ;
#16785=CARTESIAN_POINT ( 'NONE',  ( 74.41008358870023187, 68.25813196090381041, 11.92500230979622522 ) ) ;
#16786=CARTESIAN_POINT ( 'NONE',  ( 29.77967365985639248, 29.14441083166262203, 10.00000000000000533 ) ) ;
#16794=CARTESIAN_POINT ( 'NONE',  ( 78.63295798250021562, 57.35503737189328177, 16.60795452140541784 ) ) ;
#16804=CARTESIAN_POINT ( 'NONE',  ( 76.05941642030330740, 65.49204198467158733, 13.96074477642770084 ) ) ;
#16810=CARTESIAN_POINT ( 'NONE',  ( 70.32594426133741194, 65.43690866019677799, 11.69452207246081876 ) ) ;
#16813=CARTESIAN_POINT ( 'NONE',  ( 83.80447776121599190, 52.10292630681441040, -14.99896445683751622 ) ) ;
#16817=CARTESIAN_POINT ( 'NONE',  ( 82.93853206040887471, 44.70350428498475281, -9.452842870200390379 ) ) ;
#16826=CARTESIAN_POINT ( 'NONE',  ( 78.02123370085931242, 59.86933949065961968, -16.42544237888153447 ) ) ;
#16828=CARTESIAN_POINT ( 'NONE',  ( 72.21531847787744596, 67.13642658987301104, 11.23760059196915861 ) ) ;
#16831=CARTESIAN_POINT ( 'NONE',  ( 70.03535249260973217, 70.71478112856975429, -3.280756518793910281 ) ) ;
#16837=CARTESIAN_POINT ( 'NONE',  ( 3.562051267137642085, 25.55466486950697558, -1.111400068045478839E-16 ) ) ;
#16843=CARTESIAN_POINT ( 'NONE',  ( 17.73189607522619937, 18.43677371833801359, -10.00000000000000355 ) ) ;
#16846=CARTESIAN_POINT ( 'NONE',  ( 72.14138414250713538, 72.07495387501906237, 2.939176625790155928 ) ) ;
#16847=CARTESIAN_POINT ( 'NONE',  ( 12.65163835348095489, 7.708529653044779550, 1.583844403245363130 ) ) ;
#16861=CARTESIAN_POINT ( 'NONE',  ( 27.35361640444819287, 37.83396525600391413, -2.839279412974133887 ) ) ;
#16869=CARTESIAN_POINT ( 'NONE',  ( 65.82177962144463379, 68.97126114446055567, 2.130094581049046365 ) ) ;
#16874=CARTESIAN_POINT ( 'NONE',  ( 12.50787272796288896, 10.14754757982088051, -5.678558825948275768 ) ) ;
#16883=VERTEX_POINT ( 'NONE', #33276 ) ;
#16891=CARTESIAN_POINT ( 'NONE',  ( 79.01889296114715933, 59.41967273037257513, -16.52995258344894580 ) ) ;
#16904=CARTESIAN_POINT ( 'NONE',  ( 73.05277295987646369, 59.90981557475946317, 15.36185477374104025 ) ) ;
#16909=CARTESIAN_POINT ( 'NONE',  ( 81.89930626873778863, 42.21375885382296644, 7.647715624843494098 ) ) ;
#16913=CARTESIAN_POINT ( 'NONE',  ( 82.59012279121988342, 53.49374897786832150, -15.73261944071848895 ) ) ;
#16918=CARTESIAN_POINT ( 'NONE',  ( 22.66683848874176022, 18.80170272979926693, 7.433330006724137462 ) ) ;
#16932=CARTESIAN_POINT ( 'NONE',  ( 74.76064909570828831, 66.79516745633125652, -13.17056974000816005 ) ) ;
#16936=VECTOR ( 'NONE', #67498, 1000.000000000000114 ) ;
#16937=CARTESIAN_POINT ( 'NONE',  ( 82.18541192110650684, 40.82295230248577411, -1.158419095661346487 ) ) ;
#16938=CARTESIAN_POINT ( 'NONE',  ( 6.981765372403105907, 27.52903772873354882, -1.583844403245363575 ) ) ;
#16941=CARTESIAN_POINT ( 'NONE',  ( 75.92188977558036811, 65.58667241883225074, 13.87414006683291134 ) ) ;
#16947=CARTESIAN_POINT ( 'NONE',  ( 68.08257952738715346, 69.66255777483917200, 2.615794919781196715 ) ) ;
#16953=ORIENTED_EDGE ( 'NONE', *, *, #20309, .T. ) ;
#16954=FACE_OUTER_BOUND ( 'NONE', #11675, .T. ) ;
#16957=EDGE_CURVE ( 'NONE', #7306, #39570, #6883, .T. ) ;
#16959=CARTESIAN_POINT ( 'NONE',  ( 80.62770670945103291, 57.26257946240811236, -16.23162490972527294 ) ) ;
#16974=CARTESIAN_POINT ( 'NONE',  ( 12.04840505635704417, 25.14336893147754282, 7.433330006724141015 ) ) ;
#16975=DIRECTION ( 'NONE',  ( -0.2033683215378938036, 0.3522442655536374700, -0.9135454576426059736 ) ) ;
#16981=CARTESIAN_POINT ( 'NONE',  ( 22.68382546022871438, 31.83478043621389020, -8.090169943749479842 ) ) ;
#16993=CARTESIAN_POINT ( 'NONE',  ( 86.01243404335103548, 46.72055381764010917, 10.47010224649849164 ) ) ;
#16994=VECTOR ( 'NONE', #58615, 1000.000000000000114 ) ;
#16998=ORIENTED_EDGE ( 'NONE', *, *, #50830, .F. ) ;
#17001=CARTESIAN_POINT ( 'NONE',  ( 32.50825522076439000, 36.95586893147758190, 7.433330006724141015 ) ) ;
#17006=CARTESIAN_POINT ( 'NONE',  ( 80.20857538925844210, 44.21345027839176112, -11.30608575764589752 ) ) ;
#17008=CARTESIAN_POINT ( 'NONE',  ( 86.15665200708443194, 46.94614013873178493, -10.61509939557873139 ) ) ;
#17011=CARTESIAN_POINT ( 'NONE',  ( 86.31635269648819531, 44.43553455137352870, -7.074382444400770353 ) ) ;
#17013=CARTESIAN_POINT ( 'NONE',  ( 40.57792791151964451, 35.37878583063844218, 9.188101187500006262 ) ) ;
#17016=ORIENTED_EDGE ( 'NONE', *, *, #4821, .F. ) ;
#17017=B_SPLINE_CURVE_WITH_KNOTS ( 'NONE', 3,
 ( #58107, #50498, #1924, #25208, #40395, #25731, #94653, #18121, #95674, #49023, #79956, #10524, #41399, #2948, #18630, #20124 ),
 .UNSPECIFIED., .F., .F.,
 ( 4, 1, 2, 2, 2, 1, 2, 2, 4 ),
 ( 0.000000000000000000, 0.1249999999999992506, 0.1874999999999986122, 0.2499999999999979461, 0.4999999999999965028, 0.6249999999999962252, 0.6874999999999970024, 0.7499999999999976685, 1.000000000000000000 ),
 .UNSPECIFIED. ) ;
#17020=CARTESIAN_POINT ( 'NONE',  ( 77.18032279635316684, 49.61715883235847002, -14.98457440409997332 ) ) ;
#17024=( BOUNDED_CURVE ( )  B_SPLINE_CURVE ( 2, ( #21376, #75581, #31948, #25764, #95192, #85728, #57127, #78075, #39039, #8661, #65727, #10554, #41429 ),
 .UNSPECIFIED., .F., .T. ) 
 B_SPLINE_CURVE_WITH_KNOTS ( ( 3, 2, 2, 2, 2, 2, 3 ),
 ( 0.9625000000000000222, 0.9649999999999999689, 0.9699999999999999734, 0.9749999999999999778, 0.9799999999999999822, 0.9849999999999999867, 0.9875000000000000444 ),
 .UNSPECIFIED. ) 
 CURVE ( )  GEOMETRIC_REPRESENTATION_ITEM ( )  RATIONAL_B_SPLINE_CURVE ( ( 0.9755282581475767101, 0.9755282581475772652, 1.000000000000000000, 0.9510565162951535312, 1.000000000000000000, 0.9510565162951535312, 1.000000000000000000, 0.9510565162951535312, 1.000000000000000000, 0.9510565162951535312, 1.000000000000000000, 0.9755282581475761550, 0.9755282581475767101 ) ) 
 REPRESENTATION_ITEM ( '' )  );
#17030=CARTESIAN_POINT ( 'NONE',  ( 82.36756280691109566, 40.91737819406999677, 1.008661990617413462 ) ) ;
#17033=ADVANCED_FACE ( 'NONE', ( #5872 ), #51973, .T. ) ;
#17048=CARTESIAN_POINT ( 'NONE',  ( 81.26123305391610074, 43.19691626584125999, 9.572390852610855205 ) ) ;
#17049=CARTESIAN_POINT ( 'NONE',  ( 79.41556488834493166, 57.64893992652134358, 16.61893195969238946 ) ) ;
#17060=DIRECTION ( 'NONE',  ( -0.8660254037844377084, -0.5000000000000014433, -0.000000000000000000 ) ) ;
#17075=CARTESIAN_POINT ( 'NONE',  ( 74.23458728405026363, 68.58752153053315226, 11.05172902932885748 ) ) ;
#17076=CARTESIAN_POINT ( 'NONE',  ( 71.73760591565927314, 71.67260046175982779, -3.632057051425773953 ) ) ;
#17080=CARTESIAN_POINT ( 'NONE',  ( 88.11938802471243548, 44.55983648551643483, -5.053413235213819021 ) ) ;
#17084=CARTESIAN_POINT ( 'NONE',  ( 78.56874099464104688, 58.44545352437597785, 16.21180999836897385 ) ) ;
#17085=CARTESIAN_POINT ( 'NONE',  ( 84.75937136884553524, 50.43455760676256006, -13.50133169173267156 ) ) ;
#17086=CARTESIAN_POINT ( 'NONE',  ( 77.60916036496431047, 61.86143054388973184, 15.65520624218167889 ) ) ;
#17088=CARTESIAN_POINT ( 'NONE',  ( 76.38456361472545098, 51.42163124864198664, 15.62351987089070526 ) ) ;
#17093=CARTESIAN_POINT ( 'NONE',  ( 71.63103492117564031, 72.07843208848032646, 3.395715836721240777 ) ) ;
#17097=DIRECTION ( 'NONE',  ( -0.5295078238379060664, -0.5024823063053051042, -0.6834712842135700628 ) ) ;
#17099=B_SPLINE_CURVE_WITH_KNOTS ( 'NONE', 3,
 ( #27891, #36479, #67383, #43067, #21301, #58286, #42090, #90744, #20811, #73507 ),
 .UNSPECIFIED., .F., .F.,
 ( 4, 2, 2, 2, 4 ),
 ( 0.000000000000000000, 0.0002622400424273466394, 0.0005244800848546932789, 0.0007867201272820399183, 0.001048960169709386558 ),
 .UNSPECIFIED. ) ;
#17100=CARTESIAN_POINT ( 'NONE',  ( 13.87707171214468715, 8.416033932543234286, -1.583844403245364241 ) ) ;
#17105=CARTESIAN_POINT ( 'NONE',  ( 30.57771352727866443, 18.44966523072495335, -2.296566073217252530E-15 ) ) ;
#17108=CARTESIAN_POINT ( 'NONE',  ( 16.80672687576512203, 25.10171378149917842, 9.188101187500008038 ) ) ;
#17119=CARTESIAN_POINT ( 'NONE',  ( 87.55613534105700069, 44.89236293052572790, -6.575074172489557611 ) ) ;
#17121=DIRECTION ( 'NONE',  ( -0.4972609476841356457, 0.8612812260087758798, 0.1045284632676436315 ) ) ;
#17124=CARTESIAN_POINT ( 'NONE',  ( 77.71494937802162895, 49.45066113300357102, 15.33194528869553785 ) ) ;
#17128=LINE ( 'NONE', #87106, #27186 ) ;
#17130=ORIENTED_EDGE ( 'NONE', *, *, #7896, .T. ) ;
#17133=CARTESIAN_POINT ( 'NONE',  ( 79.56052108471259032, 46.24302599146017911, -13.19616287432493706 ) ) ;
#17137=CARTESIAN_POINT ( 'NONE',  ( 22.71735025659390317, 28.51421378149919406, -9.188101187500004485 ) ) ;
#17139=CARTESIAN_POINT ( 'NONE',  ( 74.92223598134691542, 66.83043205548884202, -13.20899543911388108 ) ) ;
#17140=CARTESIAN_POINT ( 'NONE',  ( 81.06846199619322135, 48.85856745326930906, -13.70439893166367362 ) ) ;
#17144=AXIS2_PLACEMENT_3D ( 'NONE', #68538, #98472, #37628 ) ;
#17148=CARTESIAN_POINT ( 'NONE',  ( 67.65092628909327743, 65.77671196984043434, 10.59442795868019260 ) ) ;
#17150=CARTESIAN_POINT ( 'NONE',  ( 81.54778536404420208, 55.93674090176426716, -16.03022157117148794 ) ) ;
#17155=CARTESIAN_POINT ( 'NONE',  ( 73.74570213160561138, 62.19087806175586053, -15.23723686604174077 ) ) ;
#17156=CARTESIAN_POINT ( 'NONE',  ( 79.59476633789469702, 59.27799801817308634, 16.56459525109985975 ) ) ;
#17160=CARTESIAN_POINT ( 'NONE',  ( 77.82180247422382990, 61.41261899432889493, -16.13690189282890941 ) ) ;
#17164=CARTESIAN_POINT ( 'NONE',  ( 80.01671443575703790, 44.39865788142935088, -11.57581203907570000 ) ) ;
#17169=CARTESIAN_POINT ( 'NONE',  ( 85.35902799246794359, 47.15769306684208573, -10.74235809367880456 ) ) ;
#17172=ORIENTED_EDGE ( 'NONE', *, *, #57167, .F. ) ;
#17179=CARTESIAN_POINT ( 'NONE',  ( 87.90883736606430432, 44.33697863951398688, 4.769790285073533198 ) ) ;
#17182=CARTESIAN_POINT ( 'NONE',  ( 84.04835165962728638, 43.69724715580328933, -7.079821572537318808 ) ) ;
#17183=CARTESIAN_POINT ( 'NONE',  ( 32.41152252715882298, 42.21091486745863364, 7.012934429366973338E-14 ) ) ;
#17193=CARTESIAN_POINT ( 'NONE',  ( 85.39402269659207434, 44.11278400351730511, 6.509279094370365115 ) ) ;
#17195=CARTESIAN_POINT ( 'NONE',  ( 78.20977235749720080, 61.70939135586247204, 16.12143617465002521 ) ) ;
#17201=CARTESIAN_POINT ( 'NONE',  ( 72.67881136679183385, 64.39378700367657871, -13.40573345294599328 ) ) ;
#17203=CARTESIAN_POINT ( 'NONE',  ( 73.87064539096938631, 55.12372134487154796, 16.60095896530753379 ) ) ;
#17205=CARTESIAN_POINT ( 'NONE',  ( 29.10770312285472627, 32.50829794293882458, -10.00000000000000355 ) ) ;
#17211=CARTESIAN_POINT ( 'NONE',  ( 82.83348971583357923, 50.32886766858683103, 14.01852798243808529 ) ) ;
#17214=CARTESIAN_POINT ( 'NONE',  ( 35.25707387162091067, 20.75978393459166327, -1.583844403245362020 ) ) ;
#17216=CARTESIAN_POINT ( 'NONE',  ( 72.11276354278739120, 72.31486658476875107, -1.049745372677822530 ) ) ;
#17219=CARTESIAN_POINT ( 'NONE',  ( 36.28012939083434674, 26.11029122506296929, -8.090169943749478065 ) ) ;
#17223=CARTESIAN_POINT ( 'NONE',  ( 73.42854352997271405, 67.10243356698696005, 12.40008471655043820 ) ) ;
#17224=CARTESIAN_POINT ( 'NONE',  ( 81.33751392502985311, 42.06992806637205717, 7.942293151799421302 ) ) ;
#17226=CARTESIAN_POINT ( 'NONE',  ( 83.39698567699524290, 51.83659370627650986, 14.98600084375454067 ) ) ;
#17230=CARTESIAN_POINT ( 'NONE',  ( 70.73742561589182287, 66.68555088280790244, -10.79243469196173599 ) ) ;
#17236=EDGE_CURVE ( 'NONE', #62754, #77470, #47771, .T. ) ;
#17246=CARTESIAN_POINT ( 'NONE',  ( 25.14222138719033595, 29.91421378149919974, 9.188101187500008038 ) ) ;
#17253=CARTESIAN_POINT ( 'NONE',  ( 13.91516400911260298, 10.96004757982088584, -5.678558825948275768 ) ) ;
#17254=CARTESIAN_POINT ( 'NONE',  ( 72.14092658844184314, 60.15097928497420554, -15.11828870562148097 ) ) ;
#17256=B_SPLINE_CURVE_WITH_KNOTS ( 'NONE', 3,
 ( #9689, #47154, #41552, #71485 ),
 .UNSPECIFIED., .F., .F.,
 ( 4, 4 ),
 ( 0.8920974736355009593, 1.000000000000000000 ),
 .UNSPECIFIED. ) ;
#17257=ORIENTED_EDGE ( 'NONE', *, *, #56694, .F. ) ;
#17261=CARTESIAN_POINT ( 'NONE',  ( 85.39213576672661077, 49.09213582878910387, 12.39711816105355169 ) ) ;
#17266=B_SPLINE_CURVE_WITH_KNOTS ( 'NONE', 3,
 ( #80014, #977, #87149, #79521, #33371, #54653, #25268, #64274, #93716, #94212 ),
 .UNSPECIFIED., .F., .F.,
 ( 4, 2, 2, 2, 4 ),
 ( 0.000000000000000000, 0.2500000000000000000, 0.5000000000000000000, 0.7500000000000000000, 1.000000000000000000 ),
 .UNSPECIFIED. ) ;
#17272=CARTESIAN_POINT ( 'NONE',  ( 72.58983975722236437, 57.29650192470587911, -16.33847390063895944 ) ) ;
#17281=CARTESIAN_POINT ( 'NONE',  ( 27.91350267930052809, 31.51421378149921182, -9.188101187500004485 ) ) ;
#17283=CARTESIAN_POINT ( 'NONE',  ( 78.54833788481614931, 48.00718989679155158, -13.97922736711163871 ) ) ;
#17285=CARTESIAN_POINT ( 'NONE',  ( 73.96424987833113107, 68.60250435897062005, 10.89670188853132160 ) ) ;
#17286=CARTESIAN_POINT ( 'NONE',  ( 32.89180500207565672, 24.15404122711135670, 8.090169943749479842 ) ) ;
#17291=CARTESIAN_POINT ( 'NONE',  ( 79.44531977136954026, 56.84425820487384584, -16.19431182515960543 ) ) ;
#17292=CARTESIAN_POINT ( 'NONE',  ( 85.51659574944204678, 43.18010505494499540, -3.869227498884009186 ) ) ;
#17297=CARTESIAN_POINT ( 'NONE',  ( 68.99060303605790523, 69.57119366415392392, -4.889576104870550388 ) ) ;
#17302=ADVANCED_FACE ( 'NONE', ( #91885 ), #6746, .T. ) ;
#17304=CARTESIAN_POINT ( 'NONE',  ( 82.65630208547716506, 42.40614048910975242, -7.237031299700372955 ) ) ;
#17305=CARTESIAN_POINT ( 'NONE',  ( 76.20785806305732990, 65.13882236753694599, 14.17010354976770081 ) ) ;
#17311=CARTESIAN_POINT ( 'NONE',  ( 70.44136121614442914, 65.74669562498131370, 11.49719858076791112 ) ) ;
#17314=CARTESIAN_POINT ( 'NONE',  ( 83.82065378329919270, 51.84410121092205515, -14.88618515114630370 ) ) ;
#17317=CARTESIAN_POINT ( 'NONE',  ( 80.31827234370541646, 57.12191670730477000, -16.23302104177161098 ) ) ;
#17319=CARTESIAN_POINT ( 'NONE',  ( 71.97624815057693581, 71.57072644777218784, 5.573434703584700500 ) ) ;
#17328=CARTESIAN_POINT ( 'NONE',  ( 72.21962075016683968, 61.93018538591146438, -14.97888511395804301 ) ) ;
#17330=B_SPLINE_SURFACE_WITH_KNOTS ( 'NONE', 3, 1, ( 
 ( #48877, #86930 ),
 ( #85408, #39234 ),
 ( #25570, #79812 ),
 ( #71184, #24555 ),
 ( #9364, #32659 ),
 ( #1269, #56459 ),
 ( #55434, #40243 ),
 ( #63559, #756 ),
 ( #86424, #87450 ),
 ( #33161, #93499 ),
 ( #10376, #63061 ),
 ( #32154, #17983 ),
 ( #94498, #24059 ),
 ( #23541, #31640 ),
 ( #25056, #16456 ),
 ( #64066, #48370 ),
 ( #62540, #79318 ),
 ( #40743, #78275 ),
 ( #54953, #85932 ),
 ( #95010, #41246 ),
 ( #263, #46860 ),
 ( #92988, #47353 ),
 ( #8859, #39726 ),
 ( #96505, #27073 ),
 ( #66061, #41753 ),
 ( #65557, #34657 ),
 ( #4254, #57450 ),
 ( #28050, #33676 ),
 ( #50354, #19972 ),
 ( #72699, #82312 ),
 ( #97485, #97011 ) ),
 .UNSPECIFIED., .F., .F., .F.,
 ( 4, 3, 3, 3, 3, 3, 3, 3, 3, 3, 4 ),
 ( 2, 2 ),
 ( 0.000000000000000000, 0.1333490885032349860, 0.3007194338854367599, 0.4699862290245074292, 0.5844252810809225096, 0.6686540514502804511, 0.7354980260655492597, 0.8028463152565746830, 0.8633854507757233732, 0.9437142632667367970, 1.000000000000000000 ),
 ( 0.000000000000000000, 1.000000000000000000 ),
 .UNSPECIFIED. ) ;
#17331=CARTESIAN_POINT ( 'NONE',  ( 69.26427230429020199, 70.44614424028236499, -2.306916011527871291 ) ) ;
#17339=DIRECTION ( 'NONE',  ( -0.8660254037844379305, -0.5000000000000014433, -0.000000000000000000 ) ) ;
#17342=CARTESIAN_POINT ( 'NONE',  ( 87.56439764236804990, 44.61845377809836322, 4.962693721234261446 ) ) ;
#17344=CARTESIAN_POINT ( 'NONE',  ( 12.21574338843640284, 25.79103043416548147, 8.090169943749478065 ) ) ;
#17348=CARTESIAN_POINT ( 'NONE',  ( 72.28971570511666300, 72.05020073419474613, 3.372523219123622518 ) ) ;
#17351=CARTESIAN_POINT ( 'NONE',  ( 4.135592144620554578, 24.16126292948893450, -6.180339887498951690 ) ) ;
#17354=CARTESIAN_POINT ( 'NONE',  ( 66.30020840643021529, 68.74685235891840307, -4.316186131942656878 ) ) ;
#17362=CARTESIAN_POINT ( 'NONE',  ( 39.09967052555147404, 28.28920272979929962, -7.433330006724141015 ) ) ;
#17367=CARTESIAN_POINT ( 'NONE',  ( 25.79477067763620468, 36.93396525600391556, 2.839279412974139660 ) ) ;
#17371=CARTESIAN_POINT ( 'NONE',  ( 65.84382221999611318, 68.94682728932481552, 2.365708372102203860 ) ) ;
#17375=CARTESIAN_POINT ( 'NONE',  ( 9.553764119070452310, 20.91421378149917132, 9.188101187500008038 ) ) ;
#17377=CARTESIAN_POINT ( 'NONE',  ( 10.20631340951632104, 27.93396525600388713, 2.839279412974139660 ) ) ;
#17384=CARTESIAN_POINT ( 'NONE',  ( 87.89265348834460667, 45.03651295921147835, 6.473805411810640287 ) ) ;
#17387=ORIENTED_EDGE ( 'NONE', *, *, #90014, .F. ) ;
#17389=CARTESIAN_POINT ( 'NONE',  ( 86.47451081130098771, 47.36193104714216418, 10.30071581693739624 ) ) ;
#17391=CARTESIAN_POINT ( 'NONE',  ( 77.39735829247300103, 55.57776196096627785, 16.14182346449976180 ) ) ;
#17394=CARTESIAN_POINT ( 'NONE',  ( 78.12740563502775615, 61.81406844543894863, -15.72119867135329407 ) ) ;
#17395=CARTESIAN_POINT ( 'NONE',  ( 79.28344036561787789, 59.07624401938414138, -16.22551900837544281 ) ) ;
#17397=CARTESIAN_POINT ( 'NONE',  ( 18.32728854387591255, 18.78052372038640172, -10.00000000000000355 ) ) ;
#17410=CARTESIAN_POINT ( 'NONE',  ( 72.70390389555041111, 58.44164253163238243, 15.66496257417437654 ) ) ;
#17412=CARTESIAN_POINT ( 'NONE',  ( 88.42017002704760387, 43.92753743058676008, 1.721442031696316599 ) ) ;
#17414=CARTESIAN_POINT ( 'NONE',  ( 83.30833261233810560, 49.39214575607078217, 13.32215296955395623 ) ) ;
#17418=CARTESIAN_POINT ( 'NONE',  ( 82.47021907082940118, 53.30441442868471569, -15.33472904691312699 ) ) ;
#17420=VECTOR ( 'NONE', #47539, 1000.000000000000114 ) ;
#17423=CARTESIAN_POINT ( 'NONE',  ( 14.90450122504689823, 30.64646525600389637, -2.839279412974133887 ) ) ;
#17429=AXIS2_PLACEMENT_3D ( 'NONE', #94706, #32868, #63774 ) ;
#17442=CARTESIAN_POINT ( 'NONE',  ( 75.05448840609841454, 66.98218832618681517, -13.15900604923073480 ) ) ;
#17444=EDGE_CURVE ( 'NONE', #25006, #98353, #79180, .T. ) ;
#17447=CARTESIAN_POINT ( 'NONE',  ( 82.59121451996566066, 40.53000206385964788, -1.428901709462959468 ) ) ;
#17451=CARTESIAN_POINT ( 'NONE',  ( 75.58531661750802755, 65.25623013732912625, 14.34312269817976571 ) ) ;
#17456=DIRECTION ( 'NONE',  ( -0.8660254037844379305, -0.5000000000000014433, -0.000000000000000000 ) ) ;
#17457=CARTESIAN_POINT ( 'NONE',  ( 22.94593010929795085, 36.18080186712593616, 3.090169943749475401 ) ) ;
#17466=CARTESIAN_POINT ( 'NONE',  ( 83.13189617009490462, 45.21769814841992030, 9.926785792809118547 ) ) ;
#17468=VECTOR ( 'NONE', #55799, 1000.000000000000114 ) ;
#17471=CARTESIAN_POINT ( 'NONE',  ( 68.69421868117841257, 64.67178190514665914, -12.16033057019549801 ) ) ;
#17473=DIRECTION ( 'NONE',  ( -0.8660254037844378194, -0.5000000000000014433, -0.000000000000000000 ) ) ;
#17481=B_SPLINE_CURVE_WITH_KNOTS ( 'NONE', 3,
 ( #28356, #20782, #82622, #44041, #74981, #36451, #88234, #85093, #38440, #52643, #75991, #14164 ),
 .UNSPECIFIED., .F., .F.,
 ( 4, 2, 2, 2, 2, 4 ),
 ( 0.000000000000000000, 0.1860970332708319352, 0.2791455499062492351, 0.3721940665416665350, 0.5582910998124992474, 0.7443881330833320709 ),
 .UNSPECIFIED. ) ;
#17484=CARTESIAN_POINT ( 'NONE',  ( 23.64951029700315743, 14.44966523072494624, -2.296566073217252530E-15 ) ) ;
#17485=CARTESIAN_POINT ( 'NONE',  ( 75.27726335905293809, 66.87231400452490959, 13.31561030640130916 ) ) ;
#17487=CARTESIAN_POINT ( 'NONE',  ( 78.33954679865345838, 57.47496213173443635, -16.60598043669875068 ) ) ;
#17495=CARTESIAN_POINT ( 'NONE',  ( 82.05544088639145173, 41.12520979201238447, -3.426473099821476964 ) ) ;
#17500=CARTESIAN_POINT ( 'NONE',  ( 17.39660613652184296, 31.81751292744056059, -6.180339887498951690 ) ) ;
#17503=CARTESIAN_POINT ( 'NONE',  ( 84.90716433703735788, 44.17344321180959099, 8.036067867235411555 ) ) ;
#17510=CARTESIAN_POINT ( 'NONE',  ( 39.71190250773520347, 34.87878583063844928, -9.188101187500006262 ) ) ;
#17512=ORIENTED_EDGE ( 'NONE', *, *, #76595, .T. ) ;
#17517=CARTESIAN_POINT ( 'NONE',  ( 79.53039288183295241, 59.52037319582147035, 16.54552321433124007 ) ) ;
#17519=CARTESIAN_POINT ( 'NONE',  ( 83.99043920266019825, 44.44647294453730524, -9.181167553117798974 ) ) ;
#17520=CARTESIAN_POINT ( 'NONE',  ( 75.64058981421790406, 52.75146229252735708, -15.94971674686773611 ) ) ;
#17521=CARTESIAN_POINT ( 'NONE',  ( 84.78071699792324978, 50.02262005461608396, -13.67739062443489750 ) ) ;
#17527=CARTESIAN_POINT ( 'NONE',  ( 77.14781257410808735, 49.36774166773431460, -15.41843211982917339 ) ) ;
#17529=CARTESIAN_POINT ( 'NONE',  ( 74.46907260258244321, 56.36757137110866722, 16.09080421635434632 ) ) ;
#17530=CARTESIAN_POINT ( 'NONE',  ( 78.49844428082862180, 50.04128099798806772, 14.89165427517412077 ) ) ;
#17543=CARTESIAN_POINT ( 'NONE',  ( 75.92249805096321325, 55.87144976864329493, 16.14995706910994500 ) ) ;
#17544=CARTESIAN_POINT ( 'NONE',  ( 38.63056705113294953, 37.70171378149921537, -9.188101187500004485 ) ) ;
#17546=VERTEX_POINT ( 'NONE', #85805 ) ;
#17547=EDGE_CURVE ( 'NONE', #86867, #11833, #57467, .T. ) ;
#17549=DIRECTION ( 'NONE',  ( -0.9646071681523453734, 0.2636911283094537373, 0.000000000000000000 ) ) ;
#17556=CARTESIAN_POINT ( 'NONE',  ( 70.74512962697180285, 71.93581810439270896, 1.182017065394330935 ) ) ;
#17564=EDGE_LOOP ( 'NONE', ( #6324, #601, #55047, #88397 ) ) ;
#17574=ORIENTED_EDGE ( 'NONE', *, *, #56421, .T. ) ;
#17586=CARTESIAN_POINT ( 'NONE',  ( 69.18172419252286431, 70.58912176915313808, -0.05407004869426973448 ) ) ;
#17590=CARTESIAN_POINT ( 'NONE',  ( 87.91732953454810229, 44.48954743135376333, -3.956250123475848923 ) ) ;
#17593=CARTESIAN_POINT ( 'NONE',  ( 78.70150085959764397, 59.83202584994826623, 16.12694553795978081 ) ) ;
#17594=CARTESIAN_POINT ( 'NONE',  ( 78.14496974547672892, 61.87975766354972507, 15.71822119279614149 ) ) ;
#17595=CARTESIAN_POINT ( 'NONE',  ( 67.00187114335926708, 67.08813303282481399, 8.529924657355552498 ) ) ;
#17596=CARTESIAN_POINT ( 'NONE',  ( 76.61485521235918839, 51.34506894449801706, 16.06955735627100879 ) ) ;
#17604=CARTESIAN_POINT ( 'NONE',  ( 73.46598367719339251, 69.88918780369783690, 9.751349427452053575 ) ) ;
#17611=CARTESIAN_POINT ( 'NONE',  ( 88.33319108017924748, 44.17511578188309329, 0.3281601038862981268 ) ) ;
#17615=LINE ( 'NONE', #79952, #67872 ) ;
#17620=CARTESIAN_POINT ( 'NONE',  ( 24.77416059058194264, 29.70171378149920471, -9.188101187500004485 ) ) ;
#17623=ORIENTED_EDGE ( 'NONE', *, *, #78688, .T. ) ;
#17624=CARTESIAN_POINT ( 'NONE',  ( 21.77916244986271366, 18.28920272979926764, -7.433330006724141015 ) ) ;
#17626=LINE ( 'NONE', #11038, #41618 ) ;
#17629=CARTESIAN_POINT ( 'NONE',  ( 74.23220016013017641, 67.58394823275320107, 11.88963712537928963 ) ) ;
#17635=CARTESIAN_POINT ( 'NONE',  ( 87.49549730082159726, 45.05290463331818529, -6.101382655908043517 ) ) ;
#17639=CARTESIAN_POINT ( 'NONE',  ( 75.15133516359631471, 53.27350175670123633, 16.03037545075837755 ) ) ;
#17641=CARTESIAN_POINT ( 'NONE',  ( 82.15897249015579007, 54.19038615186607188, 15.63353333787036092 ) ) ;
#17646=VERTEX_POINT ( 'NONE', #97844 ) ;
#17654=CARTESIAN_POINT ( 'NONE',  ( 30.88926192328758802, 20.76004757982090609, 5.678558825948272215 ) ) ;
#17655=CARTESIAN_POINT ( 'NONE',  ( 79.98196094458992889, 44.41873343662761897, 11.61139898969204332 ) ) ;
#17656=CARTESIAN_POINT ( 'NONE',  ( 74.91863663735624357, 66.38413888100485849, -13.07019282884168554 ) ) ;
#17661=ORIENTED_EDGE ( 'NONE', *, *, #30024, .F. ) ;
#17663=CARTESIAN_POINT ( 'NONE',  ( 67.74658028437072232, 65.68527340592420671, 10.74595957982673333 ) ) ;
#17667=CARTESIAN_POINT ( 'NONE',  ( 70.62151858337061583, 71.87035307724539734, -0.9651809227819526660 ) ) ;
#17675=CARTESIAN_POINT ( 'NONE',  ( 78.04364300777291419, 61.42399649461658129, -16.16113552180852508 ) ) ;
#17676=ORIENTED_EDGE ( 'NONE', *, *, #56017, .T. ) ;
#17680=CARTESIAN_POINT ( 'NONE',  ( 80.04842081486408745, 44.52432947382052220, -11.67065558011785598 ) ) ;
#17681=DIRECTION ( 'NONE',  ( 0.3037402332698194707, 0.8935232438716381731, 0.3306933373297694656 ) ) ;
#17683=CARTESIAN_POINT ( 'NONE',  ( 84.28420018112215928, 42.01594207371087464, -1.269366431083392754 ) ) ;
#17684=CARTESIAN_POINT ( 'NONE',  ( 80.77687203815185057, 48.27074620053196696, -13.47869067257540188 ) ) ;
#17693=B_SPLINE_CURVE_WITH_KNOTS ( 'NONE', 3,
 ( #55801, #1142, #16826, #71552, #64437, #93878, #47714, #40114, #86794, #33028, #48749, #47226, #17328, #94867, #25428, #70525 ),
 .UNSPECIFIED., .F., .F.,
 ( 4, 1, 2, 2, 2, 1, 2, 2, 4 ),
 ( 0.000000000000000000, 0.1250000000000061340, 0.1875000000000072442, 0.2500000000000083822, 0.5000000000000089928, 0.6250000000000093259, 0.6875000000000095479, 0.7500000000000096589, 1.000000000000000000 ),
 .UNSPECIFIED. ) ;
#17694=CARTESIAN_POINT ( 'NONE',  ( 75.63268008801898645, 65.14737934564519151, -14.41129995628931404 ) ) ;
#17695=CARTESIAN_POINT ( 'NONE',  ( 69.36794925685066460, 69.30658466222585901, -6.105352991895093062 ) ) ;
#17697=CARTESIAN_POINT ( 'NONE',  ( 88.03035862218379748, 44.39407565500617636, 4.731894665149350310 ) ) ;
#17699=ORIENTED_EDGE ( 'NONE', *, *, #84758, .F. ) ;
#17701=CARTESIAN_POINT ( 'NONE',  ( 80.52615818510180645, 45.35857030409034252, 11.48786613706528570 ) ) ;
#17703=CARTESIAN_POINT ( 'NONE',  ( 81.05763270389509501, 43.67158023151814916, 9.470390458390101074 ) ) ;
#17704=CARTESIAN_POINT ( 'NONE',  ( 71.62823836921063503, 58.95366258879743526, -15.87062632715016974 ) ) ;
#17706=CARTESIAN_POINT ( 'NONE',  ( 72.62284165280777870, 70.75758632292105688, 7.142220272083244836 ) ) ;
#17707=ADVANCED_FACE ( 'NONE', ( #52702, #67413, #37501, #68408, #99336, #14714, #76529, #69903, #85154, #516, #85675, #63309, #94251, #8617, #62803, #23802, #71427, #1018, #16212, #86670 ), #39484, .T. ) ;
#17709=ORIENTED_EDGE ( 'NONE', *, *, #91274, .F. ) ;
#17713=CARTESIAN_POINT ( 'NONE',  ( 84.25055062944881001, 42.67738571844763129, 4.568100458215928583 ) ) ;
#17722=CARTESIAN_POINT ( 'NONE',  ( 74.25007963244678422, 55.44098039740443085, 16.12168607022720579 ) ) ;
#17725=CARTESIAN_POINT ( 'NONE',  ( 34.88136640284594847, 21.10801979619931146, 3.090169943749476733 ) ) ;
#17734=CARTESIAN_POINT ( 'NONE',  ( 81.89275847971933331, 46.90471798235346057, 12.15198961269920730 ) ) ;
#17737=ADVANCED_FACE ( 'NONE', ( #47105 ), #40466, .T. ) ;
#17740=CARTESIAN_POINT ( 'NONE',  ( 82.06978721653376851, 41.21810153943793864, 5.445615563582272500 ) ) ;
#17744=CARTESIAN_POINT ( 'NONE',  ( 42.35759689194659927, 26.58380873178790793, 6.180339887498953466 ) ) ;
#17749=CARTESIAN_POINT ( 'NONE',  ( 10.13172230794903683, 17.80066082961419838, 10.00000000000000533 ) ) ;
#17752=CARTESIAN_POINT ( 'NONE',  ( 84.06109941699628507, 51.61974178474098096, 14.72645736870185473 ) ) ;
#17754=CARTESIAN_POINT ( 'NONE',  ( 69.72700409348841788, 66.78052502340607077, -10.07945174565168678 ) ) ;
#17762=CARTESIAN_POINT ( 'NONE',  ( 72.97386446981147401, 70.68132344495336383, 8.316175787459508584 ) ) ;
#17763=EDGE_LOOP ( 'NONE', ( #89620, #20544, #452, #11423 ) ) ;
#17768=CARTESIAN_POINT ( 'NONE',  ( 20.47532000956703513, 32.79752408145593279, -5.678558825948271327 ) ) ;
#17773=CARTESIAN_POINT ( 'NONE',  ( 8.259543914800127951, 22.95586893147753571, 7.433330006724141015 ) ) ;
#17775=CARTESIAN_POINT ( 'NONE',  ( 76.93060788005539052, 58.57154978847167826, -16.09350835567875748 ) ) ;
#17776=CARTESIAN_POINT ( 'NONE',  ( 71.84099513407564075, 72.54812194311107021, -1.276242074083207001 ) ) ;
#17781=CARTESIAN_POINT ( 'NONE',  ( 74.91675901630549106, 64.03713867913845093, -14.74143563292419934 ) ) ;
#17790=CARTESIAN_POINT ( 'NONE',  ( 72.63229333555629808, 57.14188050215015835, -16.36598023500532051 ) ) ;
#17791=CARTESIAN_POINT ( 'NONE',  ( 76.95477351241487440, 63.69079797318030955, 15.35326628456841824 ) ) ;
#17800=CARTESIAN_POINT ( 'NONE',  ( 25.85549604718420014, 26.87878583063842797, -9.188101187500006262 ) ) ;
#17801=LINE ( 'NONE', #18302, #3475 ) ;
#17802=CARTESIAN_POINT ( 'NONE',  ( 70.24096790410676761, 70.63068755123174469, -5.460583647663642459 ) ) ;
#17804=CARTESIAN_POINT ( 'NONE',  ( 73.77733668265750566, 68.41783923479601981, 10.96675506585084925 ) ) ;
#17808=CARTESIAN_POINT ( 'NONE',  ( 87.83187315495058556, 45.09740525803776023, 6.666720864128775403 ) ) ;
#17809=B_SPLINE_CURVE_WITH_KNOTS ( 'NONE', 3,
 ( #783, #53968, #45865, #37289, #14502, #77812, #68184, #23076, #15471, #69184 ),
 .UNSPECIFIED., .F., .F.,
 ( 4, 2, 2, 2, 4 ),
 ( 0.000000000000000000, 0.2500000000000000000, 0.5000000000000000000, 0.7500000000000000000, 1.000000000000000000 ),
 .UNSPECIFIED. ) ;
#17810=VERTEX_POINT ( 'NONE', #44988 ) ;
#17811=CARTESIAN_POINT ( 'NONE',  ( 80.74481995453727734, 56.30375985177428078, -16.12179401971438608 ) ) ;
#17823=CARTESIAN_POINT ( 'NONE',  ( 75.80739212458533416, 65.61160923183801685, 13.82794609268849406 ) ) ;
#17829=CARTESIAN_POINT ( 'NONE',  ( 83.10371324467729437, 41.41193507237026949, 1.792060051283224098 ) ) ;
#17831=EDGE_CURVE ( 'NONE', #17546, #50031, #75931, .T. ) ;
#17833=EDGE_CURVE ( 'NONE', #34456, #42933, #90080, .T. ) ;
#17834=CARTESIAN_POINT ( 'NONE',  ( 83.74452895351211623, 51.49425885220755816, -14.36953079076762663 ) ) ;
#17837=CARTESIAN_POINT ( 'NONE',  ( 80.51438793199335464, 57.80134815862462005, -16.24637616362180026 ) ) ;
#17838=CARTESIAN_POINT ( 'NONE',  ( 71.90384105138682003, 72.23694104886283185, 0.5914362187818961170 ) ) ;
#17839=CARTESIAN_POINT ( 'NONE',  ( 72.51358964696871112, 70.84733833069179809, 7.633428234268393453 ) ) ;
#17844=AXIS2_PLACEMENT_3D ( 'NONE', #38235, #63057, #76286 ) ;
#17848=CARTESIAN_POINT ( 'NONE',  ( 85.63146384662782395, 48.39429698310328121, -12.21155806772682340 ) ) ;
#17850=CARTESIAN_POINT ( 'NONE',  ( 68.04992555225376805, 69.88878367761962807, -0.7546937224205583217 ) ) ;
#17860=B_SPLINE_SURFACE_WITH_KNOTS ( 'NONE', 3, 1, ( 
 ( #296, #9915 ),
 ( #85447, #77819 ),
 ( #8401, #72221 ),
 ( #3324, #2826 ),
 ( #49398, #48908 ),
 ( #73706, #35188 ),
 ( #25607, #80856 ),
 ( #57994, #88975 ),
 ( #33715, #88464 ),
 ( #42280, #56983 ),
 ( #73214, #34690 ),
 ( #49898, #3809 ),
 ( #34205, #64607 ),
 ( #11428, #87968 ),
 ( #4288, #19530 ),
 ( #81834, #72734 ),
 ( #79843, #56494 ),
 ( #41788, #26108 ),
 ( #87481, #43277 ),
 ( #18016, #26606 ),
 ( #65591, #95562 ),
 ( #89451, #96048 ),
 ( #66096, #11916 ),
 ( #19025, #10913 ),
 ( #65095, #96539 ),
 ( #10409, #41279 ),
 ( #18512, #20007 ),
 ( #80345, #27110 ),
 ( #50886, #50390 ),
 ( #81342, #42772 ),
 ( #97044, #27612 ) ),
 .UNSPECIFIED., .F., .F., .F.,
 ( 4, 3, 3, 3, 3, 3, 3, 3, 3, 3, 4 ),
 ( 2, 2 ),
 ( 0.000000000000000000, 0.1333490885032332374, 0.3007194338854220494, 0.4699862290245090390, 0.5844252810809320575, 0.6686540514502788968, 0.7354980260655487045, 0.8028463152565534777, 0.8633854507757111607, 0.9437142632667073761, 1.000000000000000000 ),
 ( 0.000000000000000000, 1.000000000000000000 ),
 .UNSPECIFIED. ) ;
#17861=CARTESIAN_POINT ( 'NONE',  ( 76.82765370740766286, 53.09445422599739572, -15.90143384433676665 ) ) ;
#17864=CARTESIAN_POINT ( 'NONE',  ( 9.894862028763428796, 29.21091486745858745, -1.111400068045478839E-16 ) ) ;
#17867=CARTESIAN_POINT ( 'NONE',  ( 16.56575413784759121, 33.65659080271450421, -1.878358725466461243E-16 ) ) ;
#17871=CARTESIAN_POINT ( 'NONE',  ( 72.27349450330626723, 72.00028387666623075, 3.519045224867114907 ) ) ;
#17883=CARTESIAN_POINT ( 'NONE',  ( 38.69009612255265296, 24.19860640527295104, 2.839279412974134775 ) ) ;
#17887=CARTESIAN_POINT ( 'NONE',  ( 31.37640799630998956, 30.06628583063843507, -9.188101187500006262 ) ) ;
#17890=CARTESIAN_POINT ( 'NONE',  ( 65.86133180236033979, 68.95061956165834260, 2.403325992957665580 ) ) ;
#17891=VERTEX_POINT ( 'NONE', #74924 ) ;
#17892=CARTESIAN_POINT ( 'NONE',  ( 37.17256469204939151, 37.16454794089045066, -10.00000000000000355 ) ) ;
#17894=( NAMED_UNIT ( * ) PLANE_ANGLE_UNIT ( ) SI_UNIT ( $, .RADIAN. ) );
#17896=CARTESIAN_POINT ( 'NONE',  ( 12.27453364332850505, 12.80170272979924739, 7.433330006724137462 ) ) ;
#17898=CARTESIAN_POINT ( 'NONE',  ( 12.13982549814181411, 27.98502408145591502, -5.678558825948271327 ) ) ;
#17900=CARTESIAN_POINT ( 'NONE',  ( 84.42663183290279960, 49.91580812419739743, -13.73522929182741059 ) ) ;
#17901=CARTESIAN_POINT ( 'NONE',  ( 88.12055419386514643, 44.14876995426037354, -1.724036421897656934 ) ) ;
#17903=CARTESIAN_POINT ( 'NONE',  ( 73.43762515466688967, 73.52662068827324049, 2.033788753608857291E-15 ) ) ;
#17906=CARTESIAN_POINT ( 'NONE',  ( 87.18667961818120204, 45.38743208957181707, 7.099644388500629510 ) ) ;
#17911=CARTESIAN_POINT ( 'NONE',  ( 85.85796257688252808, 47.46348540752531875, 10.78667950937928310 ) ) ;
#17912=ORIENTED_EDGE ( 'NONE', *, *, #87657, .T. ) ;
#17913=CARTESIAN_POINT ( 'NONE',  ( 77.99241281452712826, 58.97741566620933895, 16.11859265156807552 ) ) ;
#17915=ORIENTED_EDGE ( 'NONE', *, *, #51314, .F. ) ;
#17916=CARTESIAN_POINT ( 'NONE',  ( 27.81076257310190769, 39.55466486950702176, 7.012934429366973338E-14 ) ) ;
#17917=CARTESIAN_POINT ( 'NONE',  ( 78.92023586790456591, 59.45316570216662910, -16.52216786098998824 ) ) ;
#17918=CARTESIAN_POINT ( 'NONE',  ( 80.20807540180908290, 48.38748433693235285, -14.23851719010586336 ) ) ;
#17919=CARTESIAN_POINT ( 'NONE',  ( 80.48839377771611225, 43.63089982895380103, 9.811837369924520047 ) ) ;
#17924=CARTESIAN_POINT ( 'NONE',  ( 30.46276441966746873, 39.36126292948897998, 6.180339887498949913 ) ) ;
#17927=CARTESIAN_POINT ( 'NONE',  ( 33.58045587329145576, 41.16126292948898424, -6.180339887498951690 ) ) ;
#17939=CARTESIAN_POINT ( 'NONE',  ( 69.31776955885030134, 64.77206886784115625, 11.72538624431390630 ) ) ;
#17941=CARTESIAN_POINT ( 'NONE',  ( 82.56662147140762897, 53.48431740468424778, -15.73383048919865423 ) ) ;
#17942=CARTESIAN_POINT ( 'NONE',  ( 77.36600796148924530, 49.13692148722834929, -14.77749963168140113 ) ) ;
#17943=ORIENTED_EDGE ( 'NONE', *, *, #46843, .T. ) ;
#17945=CARTESIAN_POINT ( 'NONE',  ( 21.37261828447143586, 20.84335787977763133, 9.188101187500006262 ) ) ;
#17952=CARTESIAN_POINT ( 'NONE',  ( 81.46828529536601593, 52.31631583627443405, -15.16276159314715066 ) ) ;
#17953=CARTESIAN_POINT ( 'NONE',  ( 86.67826574493778935, 45.56729948127456709, 8.573571648110831944 ) ) ;
#17954=FACE_OUTER_BOUND ( 'NONE', #5780, .T. ) ;
#17956=ADVANCED_FACE ( 'NONE', ( #36391 ), #5017, .T. ) ;
#17959=CARTESIAN_POINT ( 'NONE',  ( 79.14312167556931854, 57.64441083166269664, 0.000000000000000000 ) ) ;
#17962=CARTESIAN_POINT ( 'NONE',  ( 5.249714564834229158, 26.52903772873355237, -1.583844403245363575 ) ) ;
#17966=ADVANCED_FACE ( 'NONE', ( #86066 ), #2499, .T. ) ;
#17969=FACE_OUTER_BOUND ( 'NONE', #65510, .T. ) ;
#17974=ORIENTED_EDGE ( 'NONE', *, *, #8614, .T. ) ;
#17978=CARTESIAN_POINT ( 'NONE',  ( 67.90496466116340457, 69.50686951990996931, 2.866334304769667884 ) ) ;
#17983=CARTESIAN_POINT ( 'NONE',  ( 74.46210375232622880, 68.11509597928741755, -11.59312039134510819 ) ) ;
#17986=ORIENTED_EDGE ( 'NONE', *, *, #31199, .F. ) ;
#17987=CARTESIAN_POINT ( 'NONE',  ( 84.48565599034226636, 48.85800685522642794, 12.55231365627821916 ) ) ;
#18004=CARTESIAN_POINT ( 'NONE',  ( 24.63222838094502265, 17.14754757982090894, -5.678558825948276656 ) ) ;
#18005=CARTESIAN_POINT ( 'NONE',  ( 75.11766928578728653, 67.11905233721752495, 12.65062760071900705 ) ) ;
#18016=CARTESIAN_POINT ( 'NONE',  ( 81.52014092374062670, 55.46057516179622837, -16.31907950184206513 ) ) ;
#18018=CARTESIAN_POINT ( 'NONE',  ( 70.11864118459847361, 65.88152597758180207, -11.84054788745243414 ) ) ;
#18021=CARTESIAN_POINT ( 'NONE',  ( 71.94719849994382344, 72.57089041204895352, 1.653882010069164021 ) ) ;
#18024=CARTESIAN_POINT ( 'NONE',  ( 70.62781635888518394, 71.46971406967139728, 0.07536961296809761846 ) ) ;
#18028=CARTESIAN_POINT ( 'NONE',  ( 41.62797693021462209, 26.96004757982093381, -5.678558825948276656 ) ) ;
#18036=CARTESIAN_POINT ( 'NONE',  ( 78.86410592861936664, 59.57720046317054852, 16.50785913320113352 ) ) ;
#18038=CARTESIAN_POINT ( 'NONE',  ( 88.21629111658447187, 43.86250281267856366, -2.113840622537501268 ) ) ;
#18039=CARTESIAN_POINT ( 'NONE',  ( 81.33978991279256832, 50.93462248752911137, -14.65978185948963386 ) ) ;
#18043=VERTEX_POINT ( 'NONE', #25189 ) ;
#18046=CARTESIAN_POINT ( 'NONE',  ( 69.61542750552385428, 62.56132062511078828, -13.94275833699888700 ) ) ;
#18048=CARTESIAN_POINT ( 'NONE',  ( 88.36883182482389998, 44.19992593570371042, 0.005427499793692280861 ) ) ;
#18049=CARTESIAN_POINT ( 'NONE',  ( 78.93730744513115383, 51.88019286357000226, 15.41741368655081246 ) ) ;
#18051=CARTESIAN_POINT ( 'NONE',  ( 81.92045520014677606, 41.11899774358128923, 3.718728919965262225 ) ) ;
#18061=ORIENTED_EDGE ( 'NONE', *, *, #94144, .T. ) ;
#18062=CARTESIAN_POINT ( 'NONE',  ( 25.72017957606892580, 26.80066082961422680, 10.00000000000000533 ) ) ;
#18071=CARTESIAN_POINT ( 'NONE',  ( 78.14015596333129565, 47.79605781546002419, 14.53813849205122466 ) ) ;
#18083=CARTESIAN_POINT ( 'NONE',  ( 79.14312167556931854, 57.64441083166269664, 0.000000000000000000 ) ) ;
#18088=ORIENTED_EDGE ( 'NONE', *, *, #70149, .F. ) ;
#18089=CARTESIAN_POINT ( 'NONE',  ( 71.09431784387571440, 62.57662900256345750, -13.84435817819633385 ) ) ;
#18093=CARTESIAN_POINT ( 'NONE',  ( 80.72890526444484749, 43.21432171413569989, -9.149766045926375213 ) ) ;
#18094=CARTESIAN_POINT ( 'NONE',  ( 69.09200187819043038, 70.53478952123415979, 0.07191778000971091322 ) ) ;
#18096=CARTESIAN_POINT ( 'NONE',  ( 87.93867815554295930, 44.50532786965745657, -3.967150898595685593 ) ) ;
#18099=CARTESIAN_POINT ( 'NONE',  ( 78.68575686975825079, 59.63804999145194330, 16.14434349017544434 ) ) ;
#18107=CARTESIAN_POINT ( 'NONE',  ( 78.15040261416261558, 55.05491506378064059, -16.09679860028264287 ) ) ;
#18109=CARTESIAN_POINT ( 'NONE',  ( 66.63175369249636049, 68.36105297849150020, -4.334338317156124276 ) ) ;
#18116=DIRECTION ( 'NONE',  ( 0.2837547813814357833, 0.9281390619545413223, -0.2409172175609659572 ) ) ;
#18120=CARTESIAN_POINT ( 'NONE',  ( 31.19238438139944947, 38.98502408145593989, -5.678558825948271327 ) ) ;
#18121=CARTESIAN_POINT ( 'NONE',  ( 81.89326088175978668, 48.07889234901487896, 13.52455100267233234 ) ) ;
#18122=CARTESIAN_POINT ( 'NONE',  ( 84.58903325794560146, 46.78888499796955358, -10.74999075493416356 ) ) ;
#18124=CARTESIAN_POINT ( 'NONE',  ( 21.69737781089059681, 21.03085787977762777, 9.188101187500006262 ) ) ;
#18134=CARTESIAN_POINT ( 'NONE',  ( 87.58584962094528237, 45.11644481794071737, -6.124215339656664980 ) ) ;
#18137=CARTESIAN_POINT ( 'NONE',  ( 74.72358351985596414, 53.61584409156186126, 16.08411429754375277 ) ) ;
#18138=ORIENTED_EDGE ( 'NONE', *, *, #22512, .T. ) ;
#18139=CARTESIAN_POINT ( 'NONE',  ( 82.07917488340794421, 54.03863367488002467, 15.60468158849540998 ) ) ;
#18143=EDGE_CURVE ( 'NONE', #57886, #33116, #32177, .T. ) ;
#18145=EDGE_LOOP ( 'NONE', ( #20571, #24275, #26289, #2210 ) ) ;
#18148=CARTESIAN_POINT ( 'NONE',  ( 72.05417303993513656, 71.64307123591491688, 5.506498905688411050 ) ) ;
#18152=CARTESIAN_POINT ( 'NONE',  ( 31.98863997849372254, 36.65586893147758474, -7.433330006724137462 ) ) ;
#18153=CARTESIAN_POINT ( 'NONE',  ( 79.83020946089156666, 44.72169397376073618, 11.27752533527092282 ) ) ;
#18154=CARTESIAN_POINT ( 'NONE',  ( 84.83002093244189723, 50.29676582423640241, -13.82165720535206788 ) ) ;
#18172=ORIENTED_EDGE ( 'NONE', *, *, #44241, .F. ) ;
#18179=VERTEX_POINT ( 'NONE', #94386 ) ;
#18180=EDGE_CURVE ( 'NONE', #58645, #5821, #10251, .T. ) ;
#18181=CARTESIAN_POINT ( 'NONE',  ( 12.69602586335324190, 7.734156793818200981, -2.889640176918245968E-15 ) ) ;
#18186=CARTESIAN_POINT ( 'NONE',  ( 27.21537010445218741, 39.21091486745862653, 7.012934429366973338E-14 ) ) ;
#18197=CARTESIAN_POINT ( 'NONE',  ( 76.05882932919557504, 64.70680307606549775, -14.35248828871676174 ) ) ;
#18201=CARTESIAN_POINT ( 'NONE',  ( 88.22177397292790602, 44.42207723138842113, 4.484962078095955818 ) ) ;
#18204=EDGE_CURVE ( 'NONE', #65871, #22415, #91431, .T. ) ;
#18206=CARTESIAN_POINT ( 'NONE',  ( 82.18503486167877270, 40.60955881824741454, -3.312051805122440129 ) ) ;
#18215=CARTESIAN_POINT ( 'NONE',  ( 84.94422939829060226, 43.49408491451843162, 5.705947650134866933 ) ) ;
#18217=CARTESIAN_POINT ( 'NONE',  ( 77.92147852599414648, 62.01641577372943459, 15.66086047352921540 ) ) ;
#18225=CARTESIAN_POINT ( 'NONE',  ( 30.46276441966746518, 39.36126292948897998, 6.180339887498949913 ) ) ;
#18228=CARTESIAN_POINT ( 'NONE',  ( 71.85869513609316073, 58.67586711399008692, -15.48493562761569287 ) ) ;
#18229=CARTESIAN_POINT ( 'NONE',  ( 82.87443698061515818, 43.21958489367609957, -7.413545511274116429 ) ) ;
#18234=CARTESIAN_POINT ( 'NONE',  ( 82.77577997019196232, 50.05166863141886324, 13.88734606986174924 ) ) ;
#18236=CARTESIAN_POINT ( 'NONE',  ( 86.80989918712758424, 45.87808919071956382, 8.896275332294523608 ) ) ;
#18244=CARTESIAN_POINT ( 'NONE',  ( 22.01921768174555893, 36.21091486745860522, -1.111400068045478839E-16 ) ) ;
#18245=CARTESIAN_POINT ( 'NONE',  ( 41.80280824456575317, 23.94473085651394939, 1.475505719884397138E-15 ) ) ;
#18248=DIRECTION ( 'NONE',  ( -0.4851478631379979034, 0.8403007481384877631, 0.2419218955996582654 ) ) ;
#18250=CARTESIAN_POINT ( 'NONE',  ( 87.16825469001011584, 46.28910860497907009, -8.521112165214120182 ) ) ;
#18252=CARTESIAN_POINT ( 'NONE',  ( 83.43050110256683638, 51.89332412091457059, 15.00139857044201896 ) ) ;
#18262=CARTESIAN_POINT ( 'NONE',  ( 67.25222559693544611, 66.46721440497699973, -8.699209683962450868 ) ) ;
#18263=VERTEX_POINT ( 'NONE', #87802 ) ;
#18269=CARTESIAN_POINT ( 'NONE',  ( 22.71735025659390317, 28.51421378149919406, -9.188101187500004485 ) ) ;
#18274=CARTESIAN_POINT ( 'NONE',  ( 10.08301516415377641, 26.79752408145591147, -5.678558825948271327 ) ) ;
#18275=CARTESIAN_POINT ( 'NONE',  ( 90.04477061917849312, 44.76220097505219542, 0.000000000000000000 ) ) ;
#18277=LINE ( 'NONE', #49172, #39174 ) ;
#18281=CARTESIAN_POINT ( 'NONE',  ( 85.51452730306243666, 49.05009231135860404, 12.30971062534492866 ) ) ;
#18284=CARTESIAN_POINT ( 'NONE',  ( 69.36019124367645361, 65.42472516583706010, -11.87354268267799995 ) ) ;
#18291=CARTESIAN_POINT ( 'NONE',  ( 41.88317952681261858, 32.38052372038644933, 10.00000000000000533 ) ) ;
#18293=CARTESIAN_POINT ( 'NONE',  ( 70.57990371369005800, 71.55749465124115716, -3.025387803121589059 ) ) ;
#18294=CARTESIAN_POINT ( 'NONE',  ( 78.23407395591094371, 61.03864688087466561, -15.91017056289256715 ) ) ;
#18295=DIRECTION ( 'NONE',  ( 0.8660254037844379305, 0.5000000000000014433, 0.000000000000000000 ) ) ;
#18301=CARTESIAN_POINT ( 'NONE',  ( 36.24780089259745353, 32.87878583063844218, -9.188101187500006262 ) ) ;
#18302=CARTESIAN_POINT ( 'NONE',  ( 75.15191903148871688, 52.97183600646508239, -16.48001256418180915 ) ) ;
#18305=CARTESIAN_POINT ( 'NONE',  ( 74.39896838111268096, 68.39356553035000275, 11.30479640254015195 ) ) ;
#18310=EDGE_CURVE ( 'NONE', #88281, #18732, #76670, .T. ) ;
#18311=CARTESIAN_POINT ( 'NONE',  ( 74.31767992295678482, 58.65107630571846187, -15.81261070485675369 ) ) ;
#18313=ORIENTED_EDGE ( 'NONE', *, *, #93191, .T. ) ;
#18323=CARTESIAN_POINT ( 'NONE',  ( 86.62177255451531721, 43.12972632285899266, -3.134764161692230822 ) ) ;
#18329=ORIENTED_EDGE ( 'NONE', *, *, #30590, .T. ) ;
#18330=CARTESIAN_POINT ( 'NONE',  ( 87.63170318219837895, 44.36446170533411504, -4.079950490519347106 ) ) ;
#18331=CARTESIAN_POINT ( 'NONE',  ( 84.62393343236645649, 42.70031028179986521, 3.917025725994074836 ) ) ;
#18336=CARTESIAN_POINT ( 'NONE',  ( 73.93202095776594263, 57.04871283604670396, 16.01142866964926270 ) ) ;
#18339=CARTESIAN_POINT ( 'NONE',  ( 80.58432042439230258, 57.19069178250910568, -16.22979220026185487 ) ) ;
#18347=CARTESIAN_POINT ( 'NONE',  ( 67.58366560447741733, 68.29344612013603921, 5.947104913347712518 ) ) ;
#18356=CARTESIAN_POINT ( 'NONE',  ( 75.89861163282604650, 53.37371604803925607, -16.00187665499177925 ) ) ;
#18358=ADVANCED_FACE ( 'NONE', ( #92260 ), #41293, .T. ) ;
#18362=CARTESIAN_POINT ( 'NONE',  ( 26.21435097644586776, 14.94473085651392630, 1.475505719884397138E-15 ) ) ;
#18363=CARTESIAN_POINT ( 'NONE',  ( 85.94639921072385391, 48.27664717140825701, 11.96740676232643352 ) ) ;
#18364=CARTESIAN_POINT ( 'NONE',  ( 65.84416302801280096, 69.14091760660781461, 0.2185777033355933430 ) ) ;
#18367=CARTESIAN_POINT ( 'NONE',  ( 72.17372541499028671, 72.08331884783481769, 2.982055604231361290 ) ) ;
#18368=CARTESIAN_POINT ( 'NONE',  ( 7.263013161461002731, 16.14441083166258295, 10.00000000000000533 ) ) ;
#18373=DIRECTION ( 'NONE',  ( -0.3613624741150709974, -0.7937185950816926239, 0.4893137583626469000 ) ) ;
#18379=CARTESIAN_POINT ( 'NONE',  ( 36.57256041901661803, 33.06628583063844928, -9.188101187500006262 ) ) ;
#18382=CARTESIAN_POINT ( 'NONE',  ( 32.72297390791170812, 40.93396525600392977, 2.839279412974139660 ) ) ;
#18386=CARTESIAN_POINT ( 'NONE',  ( 80.81105205787801538, 42.98178676852656821, -9.627323360252351137 ) ) ;
#18389=CARTESIAN_POINT ( 'NONE',  ( 4.512196379633642174, 24.64646525600387861, -2.839279412974133887 ) ) ;
#18391=CARTESIAN_POINT ( 'NONE',  ( 15.78795072819010770, 21.06628583063840665, -9.188101187500006262 ) ) ;
#18395=CARTESIAN_POINT ( 'NONE',  ( 84.68046352546232924, 50.54697168049320055, -14.01127729920333742 ) ) ;
#18398=ADVANCED_FACE ( 'NONE', ( #63803 ), #94715, .T. ) ;
#18402=CARTESIAN_POINT ( 'NONE',  ( 66.05014806366969538, 68.57571539968135710, 4.401547170603885561 ) ) ;
#18404=CARTESIAN_POINT ( 'NONE',  ( 87.34055741008818075, 44.89555582937398981, 6.825810004488436888 ) ) ;
#18410=AXIS2_PLACEMENT_3D ( 'NONE', #79069, #40006, #86192 ) ;
#18411=CARTESIAN_POINT ( 'NONE',  ( 86.25117823697901542, 47.20812847272011226, 10.82755581481952056 ) ) ;
#18413=CARTESIAN_POINT ( 'NONE',  ( 78.15957118868782061, 60.17571743070642043, 16.00619919759238741 ) ) ;
#18416=CARTESIAN_POINT ( 'NONE',  ( 78.36990314024963311, 61.17320995784978521, -15.89858940129926523 ) ) ;
#18419=CARTESIAN_POINT ( 'NONE',  ( 80.50336155508412617, 43.50879043608720309, 9.659109878193110177 ) ) ;
#18423=CARTESIAN_POINT ( 'NONE',  ( 74.22445535223697277, 61.98362111549793241, 14.93260878751794074 ) ) ;
#18434=EDGE_CURVE ( 'NONE', #20280, #92014, #93626, .T. ) ;
#18435=CARTESIAN_POINT ( 'NONE',  ( 81.87359138893998534, 41.32955797152819599, 5.976920566253460798 ) ) ;
#18438=CARTESIAN_POINT ( 'NONE',  ( 69.54656231429063951, 65.32963776451991578, 11.37142180160457094 ) ) ;
#18444=CARTESIAN_POINT ( 'NONE',  ( 24.50893013558248157, 16.01110640527292261, 2.839279412974134775 ) ) ;
#18446=CARTESIAN_POINT ( 'NONE',  ( 77.56105267982387375, 49.72783448593992262, -15.46007777837396979 ) ) ;
#18455=CARTESIAN_POINT ( 'NONE',  ( 79.11275361919636850, 46.11146926017930525, 13.27945046512232707 ) ) ;
#18457=CARTESIAN_POINT ( 'NONE',  ( 71.71614068478815796, 59.03149745595231934, 15.86337787674895594 ) ) ;
#18459=CYLINDRICAL_SURFACE ( 'NONE', #76903, 10.00000000000001066 ) ;
#18465=CARTESIAN_POINT ( 'NONE',  ( 85.29362735876655677, 48.41412782346650800, 12.38048700662147716 ) ) ;
#18470=ORIENTED_EDGE ( 'NONE', *, *, #42284, .T. ) ;
#18473=CARTESIAN_POINT ( 'NONE',  ( 88.27284635163252347, 44.14049577968297200, 0.4518384918358809288 ) ) ;
#18474=CARTESIAN_POINT ( 'NONE',  ( 84.24943540987109714, 43.94360214673953635, 7.356120964585859845 ) ) ;
#18478=CARTESIAN_POINT ( 'NONE',  ( 81.30975366074838462, 56.24313983998633404, -16.44754541364716971 ) ) ;
#18484=CARTESIAN_POINT ( 'NONE',  ( 83.03935637480527987, 45.02721014752604844, 9.768256401072576978 ) ) ;
#18485=VECTOR ( 'NONE', #73726, 999.9999999999998863 ) ;
#18488=CARTESIAN_POINT ( 'NONE',  ( 68.57734787275012422, 64.58769200091258256, -12.17370147371886624 ) ) ;
#18492=CARTESIAN_POINT ( 'NONE',  ( 68.54821950050275348, 68.31194209259709282, -8.033256955384258546 ) ) ;
#18497=B_SPLINE_CURVE_WITH_KNOTS ( 'NONE', 3,
 ( #40499, #95273, #57698, #71431, #88178, #11138, #33936, #18724, #50113, #80057 ),
 .UNSPECIFIED., .F., .F.,
 ( 4, 2, 2, 2, 4 ),
 ( 0.000000000000000000, 0.2500000000000000000, 0.5000000000000000000, 0.7500000000000000000, 1.000000000000000000 ),
 .UNSPECIFIED. ) ;
#18501=CARTESIAN_POINT ( 'NONE',  ( 13.12254358208367400, 30.68290643055187061, 3.479690158560446702E-15 ) ) ;
#18512=CARTESIAN_POINT ( 'NONE',  ( 81.32801083308449108, 55.42016325551186640, -16.33050219934855463 ) ) ;
#18519=CARTESIAN_POINT ( 'NONE',  ( 79.75097749241258782, 52.41140398045773452, 15.43538078857268836 ) ) ;
#18522=CARTESIAN_POINT ( 'NONE',  ( 68.68909986782581711, 64.16576715805911135, -12.55144644517788777 ) ) ;
#18527=CARTESIAN_POINT ( 'NONE',  ( 12.12248498587032586, 9.127558733836243832, -6.180339887498949025 ) ) ;
#18530=CARTESIAN_POINT ( 'NONE',  ( 78.08661669030729513, 61.77574478846858597, 16.09152831843414333 ) ) ;
#18538=CARTESIAN_POINT ( 'NONE',  ( 78.44491574804551703, 51.88413252454667912, -15.48821912003990242 ) ) ;
#18542=( BOUNDED_CURVE ( )  B_SPLINE_CURVE ( 2, ( #24381, #47662, #40561, #46670, #32968, #55253, #16770 ),
 .UNSPECIFIED., .F., .T. ) 
 B_SPLINE_CURVE_WITH_KNOTS ( ( 3, 2, 2, 3 ),
 ( 0.000000000000000000, 0.005000000000000000104, 0.01000000000000000021, 0.01250000000000000243 ),
 .UNSPECIFIED. ) 
 CURVE ( )  GEOMETRIC_REPRESENTATION_ITEM ( )  RATIONAL_B_SPLINE_CURVE ( ( 1.000000000000000000, 0.9510565162951535312, 1.000000000000000000, 0.9510565162951535312, 1.000000000000000000, 0.9755282581475768211, 0.9755282581475768211 ) ) 
 REPRESENTATION_ITEM ( '' )  );
#18545=ORIENTED_EDGE ( 'NONE', *, *, #82701, .F. ) ;
#18554=CARTESIAN_POINT ( 'NONE',  ( 81.94191999987826591, 41.06410402935708248, 3.451294334475704773 ) ) ;
#18555=CARTESIAN_POINT ( 'NONE',  ( 80.78918961562681034, 43.20779693872438543, -9.098606657379765039 ) ) ;
#18559=DIRECTION ( 'NONE',  ( -0.5000000000000013323, 0.8660254037844379305, 0.000000000000000000 ) ) ;
#18562=ORIENTED_EDGE ( 'NONE', *, *, #9633, .T. ) ;
#18563=CARTESIAN_POINT ( 'NONE',  ( 70.89704694694920306, 61.12483521587895297, -14.46529911291810855 ) ) ;
#18564=CARTESIAN_POINT ( 'NONE',  ( 2.780145572064765425, 23.64646525600387506, -2.839279412974133887 ) ) ;
#18577=CARTESIAN_POINT ( 'NONE',  ( 76.43353238120225512, 51.64775962558189804, -16.15746030387889576 ) ) ;
#18590=CARTESIAN_POINT ( 'NONE',  ( 87.83461099834376284, 44.15040118474664865, 2.754765003853551164 ) ) ;
#18593=CARTESIAN_POINT ( 'NONE',  ( 71.16465123163835926, 62.56096922933172522, -13.87416499188189967 ) ) ;
#18597=CARTESIAN_POINT ( 'NONE',  ( 80.62296282160744454, 43.30841819719253039, -9.338142585044177935 ) ) ;
#18603=CARTESIAN_POINT ( 'NONE',  ( 88.01665444240776992, 44.57641488075346814, -4.048309816952348150 ) ) ;
#18612=DIRECTION ( 'NONE',  ( 0.3715724127386967335, -0.6435822975543782354, -0.6691306063588567943 ) ) ;
#18614=CARTESIAN_POINT ( 'NONE',  ( 80.66989203997422919, 54.07632877718189945, -15.76682839205882303 ) ) ;
#18617=CARTESIAN_POINT ( 'NONE',  ( 73.28147120125912295, 69.89235501152899133, 9.618937042358501444 ) ) ;
#18624=CARTESIAN_POINT ( 'NONE',  ( 80.58959146898024528, 51.98427572625367787, -15.62881256032639143 ) ) ;
#18626=DIRECTION ( 'NONE',  ( -0.9563064286990887730, 0.2923662333936572488, 0.000000000000000000 ) ) ;
#18629=CARTESIAN_POINT ( 'NONE',  ( 29.80674373534435162, 38.18502408145592852, 5.678558825948276656 ) ) ;
#18630=CARTESIAN_POINT ( 'NONE',  ( 82.91284324307122233, 52.55272390429983176, 15.38138080693978260 ) ) ;
#18632=VERTEX_POINT ( 'NONE', #38878 ) ;
#18638=ORIENTED_EDGE ( 'NONE', *, *, #68695, .F. ) ;
#18641=CARTESIAN_POINT ( 'NONE',  ( 72.60378163331358792, 71.48865662481082950, 5.602150642661395175 ) ) ;
#18644=CARTESIAN_POINT ( 'NONE',  ( 23.71749583336532297, 25.64441083166261492, -10.00000000000000533 ) ) ;
#18655=CARTESIAN_POINT ( 'NONE',  ( 72.14394712234364704, 71.70061920742823247, 5.492383471420779095 ) ) ;
#18661=CARTESIAN_POINT ( 'NONE',  ( 34.18979426048111492, 28.24335787977765477, -9.188101187500008038 ) ) ;
#18662=CARTESIAN_POINT ( 'NONE',  ( 79.85636374066935161, 49.16479052345632539, -14.19701399251250606 ) ) ;
#18681=EDGE_LOOP ( 'NONE', ( #16268, #90010, #5450, #96790 ) ) ;
#18682=CARTESIAN_POINT ( 'NONE',  ( 80.27473767918105807, 44.94266210147404195, -11.24373657056636411 ) ) ;
#18684=CARTESIAN_POINT ( 'NONE',  ( 84.89659611704327347, 42.30984424720800519, -0.5111085200278608909 ) ) ;
#18694=CARTESIAN_POINT ( 'NONE',  ( 75.97482311634344398, 65.22733265193998875, -14.46914695647701343 ) ) ;
#18697=CARTESIAN_POINT ( 'NONE',  ( 72.57805760592546562, 69.29498314558189520, -9.228818816694399629 ) ) ;
#18699=CARTESIAN_POINT ( 'NONE',  ( 87.69076027921141758, 45.30224151825790813, -7.205911438339954955 ) ) ;
#18700=DIRECTION ( 'NONE',  ( -0.03487823687206607903, 0.06041087834084090530, 0.9975640502598237536 ) ) ;
#18704=CARTESIAN_POINT ( 'NONE',  ( 80.84499876707492660, 46.13620846899319616, 11.98265363283131890 ) ) ;
#18705=CARTESIAN_POINT ( 'NONE',  ( 82.17821026166568288, 40.61471803336392128, -3.350310559445664360 ) ) ;
#18708=DIRECTION ( 'NONE',  ( -6.123233995736783292E-17, 1.060575238724905929E-16, 1.000000000000000000 ) ) ;
#18713=CARTESIAN_POINT ( 'NONE',  ( 86.03120134746475856, 45.16028859492116254, 7.773040122391054574 ) ) ;
#18714=CARTESIAN_POINT ( 'NONE',  ( 17.67616779290014861, 25.90829794293880184, 10.00000000000000355 ) ) ;
#18715=CARTESIAN_POINT ( 'NONE',  ( 83.13520543127567919, 52.15262426605144697, 14.79738518802720115 ) ) ;
#18717=ADVANCED_FACE ( 'NONE', ( #86549 ), #71555, .T. ) ;
#18719=CARTESIAN_POINT ( 'NONE',  ( 27.21537010445218741, 39.21091486745862653, 7.012934429366973338E-14 ) ) ;
#18720=CARTESIAN_POINT ( 'NONE',  ( 73.74022686020369122, 64.09745181038972817, -13.92561685800006011 ) ) ;
#18721=CARTESIAN_POINT ( 'NONE',  ( 74.23720666048474470, 55.39997257812912324, 16.12237831225943907 ) ) ;
#18723=CARTESIAN_POINT ( 'NONE',  ( 38.60757266705294910, 27.45404122711136452, -8.090169943749478065 ) ) ;
#18724=CARTESIAN_POINT ( 'NONE',  ( 78.48263164489894450, 47.83473025059171135, 13.91046930105468959 ) ) ;
#18727=CARTESIAN_POINT ( 'NONE',  ( 87.37773417632490691, 43.73256146576093073, 3.884381177787582740 ) ) ;
#18732=VERTEX_POINT ( 'NONE', #19618 ) ;
#18733=CARTESIAN_POINT ( 'NONE',  ( 87.11349487006071968, 46.19076519147613169, 8.411924245371462661 ) ) ;
#18736=CARTESIAN_POINT ( 'NONE',  ( 81.85284180441837520, 41.66615176753711580, 5.418929497052564770 ) ) ;
#18740=CARTESIAN_POINT ( 'NONE',  ( 35.44051388448051654, 36.16454794089042935, -10.00000000000000355 ) ) ;
#18746=CARTESIAN_POINT ( 'NONE',  ( 15.52034749996898633, 9.364779650996391425, 1.583844403245360466 ) ) ;
#18747=ADVANCED_FACE ( 'NONE', ( #50476 ), #42858, .T. ) ;
#18749=CARTESIAN_POINT ( 'NONE',  ( 86.84557476849437307, 45.86349151742059860, -8.191698938791937223 ) ) ;
#18750=CARTESIAN_POINT ( 'NONE',  ( 83.85749844460281111, 51.92724282576335781, 14.91256361652489915 ) ) ;
#18753=CYLINDRICAL_SURFACE ( 'NONE', #74948, 16.60714546451156792 ) ;
#18761=VERTEX_POINT ( 'NONE', #51477 ) ;
#18766=CARTESIAN_POINT ( 'NONE',  ( 20.10065364775352847, 33.64646525600390703, -2.839279412974133887 ) ) ;
#18768=CARTESIAN_POINT ( 'NONE',  ( 86.43474555478655930, 47.06867616905372387, -10.03419037324795049 ) ) ;
#18771=CARTESIAN_POINT ( 'NONE',  ( 20.84336723938811176, 14.96004757982089828, -5.678558825948275768 ) ) ;
#18787=CARTESIAN_POINT ( 'NONE',  ( 66.17343954913513926, 68.52301864461628611, -2.711686016849376379 ) ) ;
#18789=CARTESIAN_POINT ( 'NONE',  ( 72.94747645884849874, 57.63385081541922972, -16.31741162060431805 ) ) ;
#18790=CARTESIAN_POINT ( 'NONE',  ( 78.12678986096226197, 61.01961664896378323, -15.90133184208619710 ) ) ;
#18797=CARTESIAN_POINT ( 'NONE',  ( 36.63328578856461348, 23.01110640527294748, 2.839279412974134775 ) ) ;
#18799=CARTESIAN_POINT ( 'NONE',  ( 68.00890493122102498, 70.09522272019684408, -2.916841246453294456 ) ) ;
#18801=CARTESIAN_POINT ( 'NONE',  ( 73.76584831522593788, 68.38082682530667000, 11.49424229391077290 ) ) ;
#18807=CARTESIAN_POINT ( 'NONE',  ( 74.70131395912255812, 58.53265795774088076, -15.87551583097357799 ) ) ;
#18811=CARTESIAN_POINT ( 'NONE',  ( 67.35737046155603025, 69.12142928160184852, -3.136879690473392213 ) ) ;
#18812=FACE_OUTER_BOUND ( 'NONE', #48323, .T. ) ;
#18817=DIRECTION ( 'NONE',  ( 0.2551196190400365493, 0.9669094993746139011, 0.000000000000000000 ) ) ;
#18820=ORIENTED_EDGE ( 'NONE', *, *, #42814, .T. ) ;
#18823=EDGE_LOOP ( 'NONE', ( #1308, #71280, #11089, #25274 ) ) ;
#18825=CARTESIAN_POINT ( 'NONE',  ( 82.88002151971222986, 44.20230398355771229, -8.882486828932147915 ) ) ;
#18832=CARTESIAN_POINT ( 'NONE',  ( 82.35975313173908319, 41.41624149291902057, 5.521678208619409389 ) ) ;
#18835=CARTESIAN_POINT ( 'NONE',  ( 80.48346613340457623, 57.68579040447578166, -16.59506630531065241 ) ) ;
#18836=( BOUNDED_CURVE ( )  B_SPLINE_CURVE ( 2, ( #31736, #47448, #78377, #8958, #63656, #15538, #9469, #25150, #40339, #63154, #46438, #84503, #70249 ),
 .UNSPECIFIED., .F., .T. ) 
 B_SPLINE_CURVE_WITH_KNOTS ( ( 3, 2, 2, 2, 2, 2, 3 ),
 ( 0.7125000000000000222, 0.7149999999999999689, 0.7199999999999999734, 0.7249999999999999778, 0.7299999999999999822, 0.7349999999999999867, 0.7375000000000000444 ),
 .UNSPECIFIED. ) 
 CURVE ( )  GEOMETRIC_REPRESENTATION_ITEM ( )  RATIONAL_B_SPLINE_CURVE ( ( 0.9755282581475767101, 0.9755282581475772652, 1.000000000000000000, 0.9510565162951535312, 1.000000000000000000, 0.9510565162951535312, 1.000000000000000000, 0.9510565162951535312, 1.000000000000000000, 0.9510565162951535312, 1.000000000000000000, 0.9755282581475761550, 0.9755282581475767101 ) ) 
 REPRESENTATION_ITEM ( '' )  );
#18839=DIRECTION ( 'NONE',  ( -0.8660254037844377084, -0.5000000000000014433, -0.000000000000000000 ) ) ;
#18850=CARTESIAN_POINT ( 'NONE',  ( 22.75701074986381656, 14.10801979619928659, 3.090169943749476733 ) ) ;
#18851=ADVANCED_FACE ( 'NONE', ( #7359 ), #53456, .T. ) ;
#18858=CARTESIAN_POINT ( 'NONE',  ( 84.60735463175657856, 50.53152741511170376, -13.60229262012000184 ) ) ;
#18866=CARTESIAN_POINT ( 'NONE',  ( 22.92804849793282784, 21.43677371833801715, -10.00000000000000355 ) ) ;
#18871=CARTESIAN_POINT ( 'NONE',  ( 74.13238489426800015, 55.63346398866154630, -16.58957000666680059 ) ) ;
#18885=CARTESIAN_POINT ( 'NONE',  ( 40.83172133312034191, 29.28920272979929962, -7.433330006724141015 ) ) ;
#18888=CARTESIAN_POINT ( 'NONE',  ( 36.24660459446916150, 29.43085787977765833, -9.188101187500008038 ) ) ;
#18891=ADVANCED_FACE ( 'NONE', ( #60550 ), #10248, .F. ) ;
#18896=CARTESIAN_POINT ( 'NONE',  ( 9.248262631489305718, 13.84335787977760823, 9.188101187500006262 ) ) ;
#18898=CARTESIAN_POINT ( 'NONE',  ( 14.38185574516869458, 23.70171378149918340, -9.188101187500004485 ) ) ;
#18911=CARTESIAN_POINT ( 'NONE',  ( 66.51592627583551121, 68.71315881233805101, 4.796467218963683443 ) ) ;
#18912=CARTESIAN_POINT ( 'NONE',  ( 87.70668618551661666, 45.11329565042247935, 6.837976445409220894 ) ) ;
#18913=ORIENTED_EDGE ( 'NONE', *, *, #70133, .T. ) ;
#18917=CARTESIAN_POINT ( 'NONE',  ( 86.47115166784590201, 47.25330420953332577, 10.74459335058070941 ) ) ;
#18919=CARTESIAN_POINT ( 'NONE',  ( 76.75404550250510738, 52.66510328405545494, 15.83505843469623287 ) ) ;
#18921=ORIENTED_EDGE ( 'NONE', *, *, #95869, .F. ) ;
#18922=CARTESIAN_POINT ( 'NONE',  ( 68.96058394729804775, 64.32740065508541250, -11.90885421820057921 ) ) ;
#18923=CARTESIAN_POINT ( 'NONE',  ( 77.66333127137711756, 50.58589379260305918, -15.22707563559156263 ) ) ;
#18925=CARTESIAN_POINT ( 'NONE',  ( 80.72327543658212790, 43.19257391986853634, 9.937540063720549099 ) ) ;
#18938=DIRECTION ( 'NONE',  ( -0.4996954135095461047, 0.8654978445076770832, -0.03489949670251103753 ) ) ;
#18942=CARTESIAN_POINT ( 'NONE',  ( 69.87185781331436374, 66.10011063722555491, 10.85240889336124859 ) ) ;
#18948=CARTESIAN_POINT ( 'NONE',  ( 29.70508255828911004, 19.01110640527293327, 2.839279412974134775 ) ) ;
#18954=ORIENTED_EDGE ( 'NONE', *, *, #72190, .F. ) ;
#18967=B_SPLINE_CURVE_WITH_KNOTS ( 'NONE', 3,
 ( #38922, #8049, #86104, #63737 ),
 .UNSPECIFIED., .F., .F.,
 ( 4, 4 ),
 ( 0.9262915356181703475, 1.000000000000000000 ),
 .UNSPECIFIED. ) ;
#18974=CARTESIAN_POINT ( 'NONE',  ( 22.16837966976980567, 14.92755873383626053, 6.180339887498953466 ) ) ;
#18983=CARTESIAN_POINT ( 'NONE',  ( 67.54335693373008098, 69.17532794797624263, 3.376759353522594154 ) ) ;
#18984=EDGE_CURVE ( 'NONE', #1813, #57272, #93110, .T. ) ;
#18993=CARTESIAN_POINT ( 'NONE',  ( 84.65781438197950592, 49.52625469906533340, 12.95988928232620374 ) ) ;
#18997=CARTESIAN_POINT ( 'NONE',  ( 68.82519319127361257, 64.71339118656145217, -12.18766638205895347 ) ) ;
#18999=CARTESIAN_POINT ( 'NONE',  ( 79.90666100684894957, 48.61584110152371352, 14.44201039220772564 ) ) ;
#19010=CARTESIAN_POINT ( 'NONE',  ( 83.19757352214881507, 43.20952170335151266, 8.047085336822298984 ) ) ;
#19012=CARTESIAN_POINT ( 'NONE',  ( 17.84595736030643920, 25.70171378149918340, -9.188101187500004485 ) ) ;
#19013=CARTESIAN_POINT ( 'NONE',  ( 77.76098460965452830, 59.25386675525071922, -16.47652547104713250 ) ) ;
#19015=CARTESIAN_POINT ( 'NONE',  ( 81.95854183835243134, 41.81427719307645674, -5.625612379983921052 ) ) ;
#19018=CARTESIAN_POINT ( 'NONE',  ( 18.77112655976752009, 19.03677371833801502, 10.00000000000000533 ) ) ;
#19025=CARTESIAN_POINT ( 'NONE',  ( 81.42054145595460568, 55.42004525696071937, -16.32184955832448381 ) ) ;
#19026=ORIENTED_EDGE ( 'NONE', *, *, #54057, .T. ) ;
#19027=CARTESIAN_POINT ( 'NONE',  ( 76.08964319905662421, 64.37085305084526965, -14.90483801509815542 ) ) ;
#19031=CARTESIAN_POINT ( 'NONE',  ( 77.53799973678586355, 49.68283126470399225, 14.93564267158908443 ) ) ;
#19034=DIRECTION ( 'NONE',  ( 0.000000000000000000, -0.6788029332000657945, 0.7343204871709537729 ) ) ;
#19039=CARTESIAN_POINT ( 'NONE',  ( 9.015913755055775525, 20.90829794293878763, 10.00000000000000355 ) ) ;
#19046=CARTESIAN_POINT ( 'NONE',  ( 79.19335676987149952, 59.81345803429233143, 16.50342877771833017 ) ) ;
#19050=CARTESIAN_POINT ( 'NONE',  ( 77.51795247811750755, 52.17589778563348801, -15.67370978287279470 ) ) ;
#19054=ORIENTED_EDGE ( 'NONE', *, *, #51709, .T. ) ;
#19057=CARTESIAN_POINT ( 'NONE',  ( 77.23008513726504987, 49.48297111420801286, 14.92774319911447733 ) ) ;
#19059=CARTESIAN_POINT ( 'NONE',  ( 74.81619755463081844, 57.89461443497145154, 15.97444856423281934 ) ) ;
#19063=CARTESIAN_POINT ( 'NONE',  ( 82.31202062023011479, 40.66771258265164590, 3.246634729999704483 ) ) ;
#19070=CARTESIAN_POINT ( 'NONE',  ( 71.38870771651419034, 68.37070112333339011, -9.453314934521086954 ) ) ;
#19073=CARTESIAN_POINT ( 'NONE',  ( 70.55696984825441120, 61.37392526597871267, -14.80549934020668701 ) ) ;
#19074=CARTESIAN_POINT ( 'NONE',  ( 10.54248283575963008, 11.80170272979924206, 7.433330006724137462 ) ) ;
#19077=ORIENTED_EDGE ( 'NONE', *, *, #64872, .T. ) ;
#19079=CARTESIAN_POINT ( 'NONE',  ( 78.17464201438049543, 47.84695061245597003, -14.00636085769150974 ) ) ;
#19082=CARTESIAN_POINT ( 'NONE',  ( 78.50967049263377362, 51.05820285709072692, -15.70993305931173545 ) ) ;
#19084=CARTESIAN_POINT ( 'NONE',  ( 87.51937303406259616, 45.11776172068187662, 6.154781583138794865 ) ) ;
#19085=CARTESIAN_POINT ( 'NONE',  ( 88.13797031347935729, 44.16014372656159281, -1.732870377860791677 ) ) ;
#19088=CARTESIAN_POINT ( 'NONE',  ( 66.10733050139633349, 69.29219150952910411, 0.2566142034190574961 ) ) ;
#19095=AXIS2_PLACEMENT_3D ( 'NONE', #28776, #82022, #3981 ) ;
#19098=FACE_OUTER_BOUND ( 'NONE', #73377, .T. ) ;
#19100=ORIENTED_EDGE ( 'NONE', *, *, #46651, .F. ) ;
#19101=VECTOR ( 'NONE', #86593, 1000.000000000000114 ) ;
#19102=CARTESIAN_POINT ( 'NONE',  ( 74.62258251110877438, 61.63511669430710782, -15.13440849647893494 ) ) ;
#19103=CARTESIAN_POINT ( 'NONE',  ( 79.94597790610303889, 58.10291136569557580, 16.26832645005858424 ) ) ;
#19104=EDGE_CURVE ( 'NONE', #20250, #75378, #56204, .T. ) ;
#19109=CARTESIAN_POINT ( 'NONE',  ( 80.87154830239147429, 43.64994579682081621, -9.570501097346140185 ) ) ;
#19115=CARTESIAN_POINT ( 'NONE',  ( 88.00064672366042373, 44.55878435733892928, -4.022439529268951652 ) ) ;
#19117=CARTESIAN_POINT ( 'NONE',  ( 81.04961468568201610, 43.68546784643918812, -9.492462169003031747 ) ) ;
#19119=CARTESIAN_POINT ( 'NONE',  ( 82.44310520575160695, 54.28011738120410001, -15.96781897959229113 ) ) ;
#19127=CARTESIAN_POINT ( 'NONE',  ( 74.33436806272575836, 56.35182720436719706, -16.09600543955971830 ) ) ;
#19134=CARTESIAN_POINT ( 'NONE',  ( 72.81050907550364570, 57.13790140118627647, 15.89804358815998953 ) ) ;
#19140=CARTESIAN_POINT ( 'NONE',  ( 36.41017387241338099, 23.94754757982092030, 5.678558825948272215 ) ) ;
#19142=CARTESIAN_POINT ( 'NONE',  ( 75.26996855991060897, 59.55077116385917435, 16.22776523571817364 ) ) ;
#19144=CARTESIAN_POINT ( 'NONE',  ( 20.65814732634927609, 20.43085787977763346, -9.188101187500008038 ) ) ;
#19150=CARTESIAN_POINT ( 'NONE',  ( 86.35455787144825024, 47.24910468700996091, 10.80869237663237570 ) ) ;
#19155=CARTESIAN_POINT ( 'NONE',  ( 75.07675898528307812, 53.26063823009506848, 16.03352913183455186 ) ) ;
#19162=CARTESIAN_POINT ( 'NONE',  ( 73.62962662361488242, 68.62763621100698685, -10.64167080051653613 ) ) ;
#19164=CARTESIAN_POINT ( 'NONE',  ( 77.00910850481051284, 63.69207575539577704, -14.97815254220547487 ) ) ;
#19165=ORIENTED_EDGE ( 'NONE', *, *, #41229, .T. ) ;
#19172=EDGE_CURVE ( 'NONE', #78746, #57975, #44107, .T. ) ;
#19174=VECTOR ( 'NONE', #57040, 1000.000000000000114 ) ;
#19175=CARTESIAN_POINT ( 'NONE',  ( 36.52324494929276710, 26.80170272979929180, 7.433330006724137462 ) ) ;
#19176=CARTESIAN_POINT ( 'NONE',  ( 79.61341344889541460, 58.26341340635389798, -16.23793971862889407 ) ) ;
#19185=CARTESIAN_POINT ( 'NONE',  ( 85.76278670188220588, 48.57154102325930012, -11.82477194771139928 ) ) ;
#19200=CARTESIAN_POINT ( 'NONE',  ( 86.97241420434123427, 45.90339759676925979, -8.144416502837579230 ) ) ;
#19202=CARTESIAN_POINT ( 'NONE',  ( 85.01702307733869191, 42.37204648715616173, -0.3572300862006242972 ) ) ;
#19214=CARTESIAN_POINT ( 'NONE',  ( 72.50310743999735053, 69.30443315113288349, -9.159185671101845116 ) ) ;
#19216=CARTESIAN_POINT ( 'NONE',  ( 69.56331254061269931, 63.09499020812631187, -13.61442372004802159 ) ) ;
#19222=CARTESIAN_POINT ( 'NONE',  ( 81.95468535755843220, 40.99502387196763920, -3.139656615793550820 ) ) ;
#19226=LINE ( 'NONE', #88160, #36845 ) ;
#19229=LINE ( 'NONE', #73412, #26889 ) ;
#19234=CARTESIAN_POINT ( 'NONE',  ( 78.05395834205243943, 61.78695400133908322, 16.08488452160743520 ) ) ;
#19238=CARTESIAN_POINT ( 'NONE',  ( 27.37348498259797935, 38.73705186507756082, -3.090169943749475845 ) ) ;
#19241=CARTESIAN_POINT ( 'NONE',  ( 70.36206151952180221, 64.89165491571560551, -12.13793269121529939 ) ) ;
#19244=CARTESIAN_POINT ( 'NONE',  ( 74.28989463527457815, 55.24825063735668351, 16.60343178153034316 ) ) ;
#19246=CARTESIAN_POINT ( 'NONE',  ( 5.625422033609194017, 26.18080186712590773, 3.090169943749475401 ) ) ;
#19247=CARTESIAN_POINT ( 'NONE',  ( 32.19481522723634725, 40.36126292948897287, 6.180339887498949913 ) ) ;
#19250=CARTESIAN_POINT ( 'NONE',  ( 71.61951074668084516, 58.89861525787757301, -15.38682514613026697 ) ) ;
#19251=CARTESIAN_POINT ( 'NONE',  ( 87.73226871325611853, 43.96903184879543858, -2.008524143530736161 ) ) ;
#19255=CARTESIAN_POINT ( 'NONE',  ( 87.01088915102032217, 46.46540990613273436, 8.894669589848916758 ) ) ;
#19256=CARTESIAN_POINT ( 'NONE',  ( 15.67984500357415278, 27.79103043416548502, 8.090169943749478065 ) ) ;
#19257=CARTESIAN_POINT ( 'NONE',  ( 81.64626603452745712, 41.61031147741153546, 5.575064572453345413 ) ) ;
#19259=VECTOR ( 'NONE', #56208, 1000.000000000000000 ) ;
#19262=CARTESIAN_POINT ( 'NONE',  ( 30.74868702942336895, 36.49103043416551628, -8.090169943749479842 ) ) ;
#19266=CARTESIAN_POINT ( 'NONE',  ( 69.08701910782110645, 67.88901153317110015, -8.224971608199886930 ) ) ;
#19267=B_SPLINE_SURFACE_WITH_KNOTS ( 'NONE', 3, 1, ( 
 ( #7412, #45412 ),
 ( #6436, #45894 ),
 ( #37805, #5929 ),
 ( #60105, #21634 ),
 ( #99639, #14030 ),
 ( #37314, #99139 ),
 ( #61105, #92078 ),
 ( #47409, #320 ),
 ( #24117, #61606 ),
 ( #9935, #46401 ),
 ( #92559, #63117 ),
 ( #70715, #94554 ),
 ( #1832, #84956 ),
 ( #15499, #55008 ),
 ( #1330, #69213 ),
 ( #62600, #77838 ),
 ( #7932, #78839 ),
 ( #25110, #32212 ),
 ( #69712, #94060 ),
 ( #85986, #100141 ),
 ( #30727, #38806 ),
 ( #32714, #23104 ),
 ( #63614, #53995 ),
 ( #16514, #55989 ),
 ( #814, #24613 ),
 ( #77325, #31209 ),
 ( #16017, #55495 ),
 ( #79372, #86481 ),
 ( #78335, #86986 ),
 ( #17008, #62096 ),
 ( #93043, #23599 ) ),
 .UNSPECIFIED., .F., .F., .F.,
 ( 4, 3, 3, 3, 3, 3, 3, 3, 3, 3, 4 ),
 ( 2, 2 ),
 ( 0.000000000000000000, 0.1333490885032353190, 0.3007194338854385363, 0.4699862290245196972, 0.5844252810809350551, 0.6686540514502717913, 0.7354980260655500368, 0.8028463152565585847, 0.8633854507757243724, 0.9437142632667462339, 1.000000000000000000 ),
 ( 0.000000000000000000, 1.000000000000000000 ),
 .UNSPECIFIED. ) ;
#19269=CARTESIAN_POINT ( 'NONE',  ( 83.38047668388445288, 51.78471284047384415, 14.96842148903410319 ) ) ;
#19272=CARTESIAN_POINT ( 'NONE',  ( 75.15470013510049796, 53.07573778316540825, 16.49092276959341064 ) ) ;
#19283=CARTESIAN_POINT ( 'NONE',  ( 24.98947064339976265, 26.37878583063841731, 9.188101187500006262 ) ) ;
#19289=CARTESIAN_POINT ( 'NONE',  ( 19.20273687360401027, 16.80170272979925628, 7.433330006724137462 ) ) ;
#19290=CARTESIAN_POINT ( 'NONE',  ( 68.45344762042827824, 64.57392882346940155, 12.12708197196866600 ) ) ;
#19294=CARTESIAN_POINT ( 'NONE',  ( 72.45938080685448313, 71.20901404950713243, -6.080114014991351290 ) ) ;
#19296=DIRECTION ( 'NONE',  ( -0.8660254037844377084, -0.5000000000000014433, -0.000000000000000000 ) ) ;
#19304=VERTEX_POINT ( 'NONE', #46605 ) ;
#19305=CARTESIAN_POINT ( 'NONE',  ( 65.84722295223909327, 68.92719200281077008, -2.492171992192153240 ) ) ;
#19308=CARTESIAN_POINT ( 'NONE',  ( 69.56017153759040639, 71.20905094733247154, -1.738453268357221582 ) ) ;
#19309=CARTESIAN_POINT ( 'NONE',  ( 78.10947740687990404, 61.47724562959768946, -16.15800848020992930 ) ) ;
#19318=VERTEX_POINT ( 'NONE', #31409 ) ;
#19319=CARTESIAN_POINT ( 'NONE',  ( 32.94608582406294772, 39.99752408145594984, 5.678558825948277544 ) ) ;
#19328=ORIENTED_EDGE ( 'NONE', *, *, #40844, .T. ) ;
#19334=DIRECTION ( 'NONE',  ( -0.8660254037844379305, -0.5000000000000014433, -0.000000000000000000 ) ) ;
#19335=CARTESIAN_POINT ( 'NONE',  ( 68.40658122464360247, 69.43545487971397279, -4.271840473564598284 ) ) ;
#19336=CARTESIAN_POINT ( 'NONE',  ( 79.14312167556931854, 57.64441083166269664, 0.000000000000000000 ) ) ;
#19337=CARTESIAN_POINT ( 'NONE',  ( 80.74781574657599492, 57.21644485803225422, 16.56566952311892749 ) ) ;
#19340=PLANE ( 'NONE',  #48267 ) ;
#19347=CARTESIAN_POINT ( 'NONE',  ( 82.09644834878162101, 44.24571031629783846, -9.484918253198090454 ) ) ;
#19352=CARTESIAN_POINT ( 'NONE',  ( 74.21441779998785648, 58.33243994155952805, 15.86737782346030201 ) ) ;
#19355=CARTESIAN_POINT ( 'NONE',  ( 80.65711718680429954, 57.43377920104063605, -16.23697608741668574 ) ) ;
#19360=ADVANCED_FACE ( 'NONE', ( #16715 ), #9643, .T. ) ;
#19362=CARTESIAN_POINT ( 'NONE',  ( 67.26344415152594536, 67.87376856832382543, 6.424593239651369636 ) ) ;
#19366=CARTESIAN_POINT ( 'NONE',  ( 21.19816502305182837, 13.20801979619928268, -3.090169943749474069 ) ) ;
#19373=CARTESIAN_POINT ( 'NONE',  ( 77.80060431799728349, 52.79663923430527461, -15.76147068082156899 ) ) ;
#19374=ORIENTED_EDGE ( 'NONE', *, *, #67059, .F. ) ;
#19381=CARTESIAN_POINT ( 'NONE',  ( 83.23303302330263875, 41.40721320258948879, 4.067920842383329294 ) ) ;
#19382=CARTESIAN_POINT ( 'NONE',  ( 25.38349897777161246, 16.78380873178787169, -6.180339887498949025 ) ) ;
#19383=CARTESIAN_POINT ( 'NONE',  ( 68.10039974585599509, 65.18542567973287305, -10.72853162865224519 ) ) ;
#19387=CARTESIAN_POINT ( 'NONE',  ( 73.74433816791051299, 55.34249187257252345, -16.59213747446436571 ) ) ;
#19390=CARTESIAN_POINT ( 'NONE',  ( 76.24678322307947553, 56.72522291046242060, 16.60682109591483169 ) ) ;
#19391=CARTESIAN_POINT ( 'NONE',  ( 33.69734285410222441, 21.58380873178789372, 6.180339887498953466 ) ) ;
#19398=CARTESIAN_POINT ( 'NONE',  ( 32.83301474718356161, 37.14336893147758900, 7.433330006724141015 ) ) ;
#19401=CARTESIAN_POINT ( 'NONE',  ( 33.82173346387272517, 28.03085787977764909, 9.188101187500006262 ) ) ;
#19407=CARTESIAN_POINT ( 'NONE',  ( 5.233272902960924178, 23.99752408145590010, 5.678558825948277544 ) ) ;
#19409=CARTESIAN_POINT ( 'NONE',  ( 18.38602693954342371, 22.56628583063840310, 9.188101187500006262 ) ) ;
#19415=CARTESIAN_POINT ( 'NONE',  ( 23.12210336471560623, 25.30066082961422325, -10.00000000000000533 ) ) ;
#19417=EDGE_CURVE ( 'NONE', #68127, #63730, #93253, .T. ) ;
#19423=CARTESIAN_POINT ( 'NONE',  ( 66.54990378112017879, 68.24084232656181825, 4.554841679438449198 ) ) ;
#19424=CARTESIAN_POINT ( 'NONE',  ( 87.52489256634972037, 45.06004022996452107, 6.936227203615883852 ) ) ;
#19430=VERTEX_POINT ( 'NONE', #63315 ) ;
#19431=CARTESIAN_POINT ( 'NONE',  ( 77.69300220237600740, 57.14232284133041873, 16.18446285159314257 ) ) ;
#19436=CARTESIAN_POINT ( 'NONE',  ( 81.34849765221251516, 49.51565197037416510, -13.99490981827331559 ) ) ;
#19437=CARTESIAN_POINT ( 'NONE',  ( 81.01539833309765015, 43.04435665648513520, 9.559117910057512546 ) ) ;
#19438=ORIENTED_EDGE ( 'NONE', *, *, #58095, .F. ) ;
#19441=CARTESIAN_POINT ( 'NONE',  ( 73.35536025913421554, 58.29657773774909657, 15.76285285645408152 ) ) ;
#19451=CARTESIAN_POINT ( 'NONE',  ( 87.80086816424551444, 43.95683443436809767, 1.316077942333925277 ) ) ;
#19453=CARTESIAN_POINT ( 'NONE',  ( 83.00815485991435594, 53.30142267139500234, 15.60062745561815589 ) ) ;
#19459=ORIENTED_EDGE ( 'NONE', *, *, #89556, .F. ) ;
#19460=CARTESIAN_POINT ( 'NONE',  ( 67.66477494612622934, 65.93994996590180335, 10.43000742999573838 ) ) ;
#19461=CARTESIAN_POINT ( 'NONE',  ( 26.56877070717806788, 23.84335787977763843, 9.188101187500006262 ) ) ;
#19466=ORIENTED_EDGE ( 'NONE', *, *, #69535, .F. ) ;
#19483=EDGE_CURVE ( 'NONE', #44296, #82635, #21082, .T. ) ;
#19485=CARTESIAN_POINT ( 'NONE',  ( 84.79698219828915740, 50.36941373931320243, 13.45059404220081234 ) ) ;
#19489=VERTEX_POINT ( 'NONE', #49611 ) ;
#19490=ORIENTED_EDGE ( 'NONE', *, *, #54384, .F. ) ;
#19491=CARTESIAN_POINT ( 'NONE',  ( 73.77070425341645432, 68.39923094797843817, 11.48015304846415141 ) ) ;
#19494=EDGE_CURVE ( 'NONE', #20041, #9204, #92318, .T. ) ;
#19495=CARTESIAN_POINT ( 'NONE',  ( 70.25964755056540412, 71.21311948813186632, -0.4467044605720515982 ) ) ;
#19500=DIRECTION ( 'NONE',  ( 0.8660254037844382635, 0.5000000000000005551, 0.000000000000000000 ) ) ;
#19503=CARTESIAN_POINT ( 'NONE',  ( 79.28866853763615552, 59.92453731934287475, -16.49803216704722786 ) ) ;
#19506=CARTESIAN_POINT ( 'NONE',  ( 68.76972388951917026, 64.18474346107819883, -11.93496927694269871 ) ) ;
#19512=CARTESIAN_POINT ( 'NONE',  ( 68.12666880830131788, 66.36964627602041844, 9.486737533835349012 ) ) ;
#19518=CARTESIAN_POINT ( 'NONE',  ( 20.27082849090286487, 27.10171378149918908, 9.188101187500008038 ) ) ;
#19519=CARTESIAN_POINT ( 'NONE',  ( 74.75515603635287221, 67.17787269918751747, 12.46789500065375123 ) ) ;
#19522=CARTESIAN_POINT ( 'NONE',  ( 81.72320923516716107, 41.47097560424118967, -5.133185482711140502 ) ) ;
#19530=CARTESIAN_POINT ( 'NONE',  ( 81.75576429312462778, 55.32182455908718310, -15.92503432444246769 ) ) ;
#19532=CARTESIAN_POINT ( 'NONE',  ( 69.30351820464169066, 67.54782995425182435, 8.872334801762805867 ) ) ;
#19534=CARTESIAN_POINT ( 'NONE',  ( 84.20645638665105537, 43.21656257813889113, 5.952274718717716517 ) ) ;
#19535=CARTESIAN_POINT ( 'NONE',  ( 79.92914515571509071, 53.26920964233459443, 15.63750486048350474 ) ) ;
#19537=PLANE ( 'NONE',  #29075 ) ;
#19541=CARTESIAN_POINT ( 'NONE',  ( 45.29353982640898835, 28.01110640527296525, 2.839279412974134775 ) ) ;
#19550=CARTESIAN_POINT ( 'NONE',  ( 82.35285118013293015, 53.50770157854819331, -15.77620284334259004 ) ) ;
#19554=CARTESIAN_POINT ( 'NONE',  ( 77.82431933516703282, 52.07990706851629881, -15.61525674500613015 ) ) ;
#19562=VERTEX_POINT ( 'NONE', #13618 ) ;
#19569=CARTESIAN_POINT ( 'NONE',  ( 82.17875632138135700, 40.70310602011421253, 3.701530608362966657 ) ) ;
#19570=CARTESIAN_POINT ( 'NONE',  ( 87.86298961015023679, 44.89260222163543546, 6.207647304897661478 ) ) ;
#19573=CARTESIAN_POINT ( 'NONE',  ( 83.27157833596524483, 41.69773053680957275, -4.903519799690783110 ) ) ;
#19576=CARTESIAN_POINT ( 'NONE',  ( 70.57420050861817629, 60.83333136545436304, -14.51089813485932467 ) ) ;
#19577=CARTESIAN_POINT ( 'NONE',  ( 4.795442299662375341, 20.95586893147752861, 7.433330006724141015 ) ) ;
#19579=CARTESIAN_POINT ( 'NONE',  ( 85.37572018521500183, 48.32884972269767587, -12.27680401939018040 ) ) ;
#19587=CARTESIAN_POINT ( 'NONE',  ( 86.73131677312836985, 44.08822098498369968, 4.652549913689809635 ) ) ;
#19588=CARTESIAN_POINT ( 'NONE',  ( 88.19122672570537702, 43.84786592109882264, -2.112715317146043770 ) ) ;
#19591=EDGE_CURVE ( 'NONE', #4961, #13423, #5262, .T. ) ;
#19592=CARTESIAN_POINT ( 'NONE',  ( 66.46320885748657759, 68.94986384069260055, 0.01364106734874200727 ) ) ;
#19602=FACE_OUTER_BOUND ( 'NONE', #21894, .T. ) ;
#19603=CARTESIAN_POINT ( 'NONE',  ( 88.27664040203158891, 44.35691339321036253, 2.453685708849345115 ) ) ;
#19606=CARTESIAN_POINT ( 'NONE',  ( 78.02536995280269139, 60.40816079000541095, -15.95887260008864139 ) ) ;
#19612=VECTOR ( 'NONE', #25159, 1000.000000000000114 ) ;
#19613=CARTESIAN_POINT ( 'NONE',  ( 80.89756888259256584, 43.32073300323414600, -9.969383766040824213 ) ) ;
#19618=CARTESIAN_POINT ( 'NONE',  ( 73.30483403957811106, 69.17932697374328654, -9.895411455429695025 ) ) ;
#19621=DIRECTION ( 'NONE',  ( -0.8660254037844377084, -0.5000000000000014433, -0.000000000000000000 ) ) ;
#19625=CARTESIAN_POINT ( 'NONE',  ( 84.26883830235146888, 50.64164195736777430, 13.79214756291445454 ) ) ;
#19626=CARTESIAN_POINT ( 'NONE',  ( 75.28183178272522014, 56.04897244165069026, -16.14794119758950686 ) ) ;
#19637=CARTESIAN_POINT ( 'NONE',  ( 39.23796756512304285, 23.44966523072497466, -2.296566073217252530E-15 ) ) ;
#19638=CARTESIAN_POINT ( 'NONE',  ( 77.97190755774620641, 49.62147354114171804, -15.34335462392983729 ) ) ;
#19639=CARTESIAN_POINT ( 'NONE',  ( 85.95130255176152900, 46.56195125003082325, -9.711085333795121954 ) ) ;
#19641=CARTESIAN_POINT ( 'NONE',  ( 29.82838080365165112, 20.14754757982091249, -5.678558825948276656 ) ) ;
#19646=B_SPLINE_CURVE_WITH_KNOTS ( 'NONE', 3,
 ( #87425, #17953, #82282, #28517, #97943, #20443, #52805, #5722, #83253, #76149, #29525, #36114, #12855, #5233, #6723, #98942 ),
 .UNSPECIFIED., .F., .F.,
 ( 4, 1, 2, 2, 2, 1, 2, 2, 4 ),
 ( 0.000000000000000000, 0.1250000000000012212, 0.1875000000000016376, 0.2500000000000020539, 0.5000000000000007772, 0.6250000000000014433, 0.6875000000000007772, 0.7500000000000003331, 1.000000000000000000 ),
 .UNSPECIFIED. ) ;
#19647=CARTESIAN_POINT ( 'NONE',  ( 86.65390046659096868, 47.16758140886460637, 10.54653844973484489 ) ) ;
#19648=CARTESIAN_POINT ( 'NONE',  ( 74.55668988929480179, 63.24185806647356145, 14.99962697611943163 ) ) ;
#19649=CARTESIAN_POINT ( 'NONE',  ( 72.60177889808650775, 71.50969142880882146, 5.552899927521425916 ) ) ;
#19652=CARTESIAN_POINT ( 'NONE',  ( 74.82526768066999523, 53.43972195870694719, 16.54088702656758869 ) ) ;
#19657=CARTESIAN_POINT ( 'NONE',  ( 83.96259819183102024, 41.85579124667931694, 1.613362698078202540 ) ) ;
#19658=CARTESIAN_POINT ( 'NONE',  ( 77.22151312697972969, 62.97658066207817740, -15.28167293043454222 ) ) ;
#19659=ORIENTED_EDGE ( 'NONE', *, *, #64612, .T. ) ;
#19661=CARTESIAN_POINT ( 'NONE',  ( 72.03640812230088386, 71.62847206889918539, 5.517176230632431455 ) ) ;
#19664=CARTESIAN_POINT ( 'NONE',  ( 88.18084728802688232, 44.43898297010869669, -4.607830584147578179 ) ) ;
#19666=CARTESIAN_POINT ( 'NONE',  ( 28.93411276635479368, 38.74646525600392266, 2.839279412974139660 ) ) ;
#19670=CARTESIAN_POINT ( 'NONE',  ( 82.88421405995129021, 40.62802518055320888, -0.2805589297870617060 ) ) ;
#19675=CARTESIAN_POINT ( 'NONE',  ( 41.44395331530407844, 35.87878583063845639, -9.188101187500006262 ) ) ;
#19678=CARTESIAN_POINT ( 'NONE',  ( 85.43645318413936707, 48.61927365843763482, 12.47466632846418122 ) ) ;
#19692=CARTESIAN_POINT ( 'NONE',  ( 87.19297534993042120, 45.95771221245824734, -8.700079422534972906 ) ) ;
#19695=CARTESIAN_POINT ( 'NONE',  ( 7.946103921272086090, 26.36126292948893735, 6.180339887498949913 ) ) ;
#19707=CARTESIAN_POINT ( 'NONE',  ( 69.62288408176668497, 62.35433023048172885, -13.49615336126608867 ) ) ;
#19712=CARTESIAN_POINT ( 'NONE',  ( 82.37580512874393435, 51.26179720552115526, 14.55059045582508404 ) ) ;
#19713=CARTESIAN_POINT ( 'NONE',  ( 82.18985274614976788, 40.66879167456242783, -3.543735024996086835 ) ) ;
#19714=EDGE_CURVE ( 'NONE', #83225, #25393, #34329, .T. ) ;
#19715=CARTESIAN_POINT ( 'NONE',  ( 80.57917228006874666, 43.44270375979753851, 9.528029932415835290 ) ) ;
#19720=CARTESIAN_POINT ( 'NONE',  ( 80.96506752577832344, 55.91141337780396015, 16.08528190432092231 ) ) ;
#19728=CARTESIAN_POINT ( 'NONE',  ( 74.22259355549384452, 55.16627323567375640, 16.60417442601049842 ) ) ;
#19730=CARTESIAN_POINT ( 'NONE',  ( 41.22093855302743748, 25.92755873383629250, 6.180339887498953466 ) ) ;
#19731=CARTESIAN_POINT ( 'NONE',  ( 80.87487590722817288, 55.61906553629490446, -16.40244339227437820 ) ) ;
#19735=CARTESIAN_POINT ( 'NONE',  ( 81.86168173829938155, 43.19759374944588615, -8.265271606104395374 ) ) ;
#19740=CARTESIAN_POINT ( 'NONE',  ( 87.35606880162971777, 45.77061481740688720, 8.290963297571634527 ) ) ;
#19742=CARTESIAN_POINT ( 'NONE',  ( 40.40883878445526278, 23.73415679381825782, -6.890680421881970419E-14 ) ) ;
#19746=CARTESIAN_POINT ( 'NONE',  ( 32.56963740530460427, 41.73705186507756082, -3.090169943749475845 ) ) ;
#19750=CARTESIAN_POINT ( 'NONE',  ( 71.55070063111804757, 67.78110124390339308, -10.19286156064286786 ) ) ;
#19751=CARTESIAN_POINT ( 'NONE',  ( 86.98710364365733483, 45.90732384579192171, -8.137934770119690242 ) ) ;
#19754=CARTESIAN_POINT ( 'NONE',  ( 87.69076027921141758, 45.30224151825790813, -7.205911438339954955 ) ) ;
#19756=CARTESIAN_POINT ( 'NONE',  ( 74.91658594121764736, 53.18802753783876369, 16.51533261098013128 ) ) ;
#19763=CARTESIAN_POINT ( 'NONE',  ( 67.39535085695571581, 67.25041444790150535, -8.623144929768267630 ) ) ;
#19767=DIRECTION ( 'NONE',  ( 0.2649596321166021728, -0.4589235447807153423, -0.8480480961564252906 ) ) ;
#19768=CARTESIAN_POINT ( 'NONE',  ( 29.64555348686941016, 32.51421378149920827, -9.188101187500004485 ) ) ;
#19770=CARTESIAN_POINT ( 'NONE',  ( 86.46983487695372617, 47.48951387118550116, -10.44352480544961637 ) ) ;
#19774=CARTESIAN_POINT ( 'NONE',  ( 9.881553883097156543, 27.74646525600388713, 2.839279412974139660 ) ) ;
#19775=CARTESIAN_POINT ( 'NONE',  ( 22.01921768174555893, 36.21091486745860522, -1.111400068045478839E-16 ) ) ;
#19792=CARTESIAN_POINT ( 'NONE',  ( 78.17513785305828833, 61.62242163703883335, -16.13566992787025356 ) ) ;
#19801=CARTESIAN_POINT ( 'NONE',  ( 40.64525884627276042, 24.26216523072497466, -2.296566073217252530E-15 ) ) ;
#19810=CARTESIAN_POINT ( 'NONE',  ( 73.36337205780706938, 63.47506113005868400, -14.09265201955449598 ) ) ;
#19829=CARTESIAN_POINT ( 'NONE',  ( 74.71934731310142297, 60.78794131512849219, 15.41883525433982527 ) ) ;
#19832=CARTESIAN_POINT ( 'NONE',  ( 76.65664154646117368, 55.40719475734993438, 16.15617875289344596 ) ) ;
#19833=CARTESIAN_POINT ( 'NONE',  ( 72.48661302258760486, 71.52526770760661634, -5.337229783571229014 ) ) ;
#19840=CARTESIAN_POINT ( 'NONE',  ( 69.55672757425234920, 70.47494305999370567, 2.963892479765599663 ) ) ;
#19846=B_SPLINE_SURFACE_WITH_KNOTS ( 'NONE', 3, 1, ( 
 ( #73894, #96729 ),
 ( #13102, #58663 ),
 ( #4483, #20197 ),
 ( #66288, #89635 ),
 ( #11606, #3510 ),
 ( #96226, #65285 ),
 ( #28272, #51067 ),
 ( #59148, #19707 ),
 ( #74413, #4998 ),
 ( #90118, #51581 ),
 ( #67272, #28780 ),
 ( #82538, #43962 ),
 ( #74900, #65771 ),
 ( #90633, #36367 ),
 ( #27294, #98199 ),
 ( #73399, #59661 ),
 ( #34387, #89161 ),
 ( #21196, #3985 ),
 ( #52075, #26790 ),
 ( #81043, #88650 ),
 ( #19216, #50086 ),
 ( #42465, #34871 ),
 ( #15550, #60154 ),
 ( #92130, #54543 ),
 ( #99688, #13589 ),
 ( #14584, #53562 ),
 ( #85006, #83518 ),
 ( #75905, #54048 ),
 ( #30271, #14080 ),
 ( #84514, #91118 ),
 ( #61661, #374 ) ),
 .UNSPECIFIED., .F., .F., .F.,
 ( 4, 3, 3, 3, 3, 3, 3, 3, 3, 3, 4 ),
 ( 2, 2 ),
 ( 0.000000000000000000, 0.1122669598086922238, 0.2243161639709877753, 0.3396355846219357155, 0.4553962076585463259, 0.5677860799922646029, 0.6749047109689955137, 0.7773884377078522645, 0.8775581155834401015, 0.9782364162378043293, 1.000000000000000000 ),
 ( 0.000000000000000000, 1.000000000000000000 ),
 .UNSPECIFIED. ) ;
#19847=CARTESIAN_POINT ( 'NONE',  ( 12.81113585708611957, 26.13478043621386959, 8.090169943749478065 ) ) ;
#19849=CARTESIAN_POINT ( 'NONE',  ( 81.59834852019750429, 41.61476123368048263, 5.652816389801710528 ) ) ;
#19863=CARTESIAN_POINT ( 'NONE',  ( 16.98118013718471886, 32.73705186507753950, -3.090169943749475845 ) ) ;
#19864=CARTESIAN_POINT ( 'NONE',  ( 85.69812724468053489, 48.75358317490552196, 11.98593812281557902 ) ) ;
#19868=CARTESIAN_POINT ( 'NONE',  ( 73.85836482019932703, 55.05148726086135014, -16.60244221165485357 ) ) ;
#19871=CARTESIAN_POINT ( 'NONE',  ( 75.19642846017637794, 67.02491989442394527, 12.74302411039618832 ) ) ;
#19879=CARTESIAN_POINT ( 'NONE',  ( 80.58426559298514746, 57.69291223751457665, -16.24425291953823347 ) ) ;
#19880=CARTESIAN_POINT ( 'NONE',  ( 78.70582684749655300, 59.88532474210303747, 16.12216508957796890 ) ) ;
#19881=CARTESIAN_POINT ( 'NONE',  ( 32.24243340009443415, 30.56628583063843152, 9.188101187500006262 ) ) ;
#19885=CARTESIAN_POINT ( 'NONE',  ( 43.11943305279750405, 25.86426979415093186, -3.090169943749474069 ) ) ;
#19887=CARTESIAN_POINT ( 'NONE',  ( 13.54711677929152636, 28.79752408145592213, -5.678558825948271327 ) ) ;
#19888=CARTESIAN_POINT ( 'NONE',  ( 71.94676095904020485, 72.61122666528670777, 1.254485733363759792 ) ) ;
#19889=CARTESIAN_POINT ( 'NONE',  ( 82.25327158856319443, 54.24549761180711016, 15.63371342117970642 ) ) ;
#19899=CARTESIAN_POINT ( 'NONE',  ( 82.81737761406506593, 40.62361263874299055, 0.9906565629087065172 ) ) ;
#19900=CARTESIAN_POINT ( 'NONE',  ( 66.76973844028468363, 68.39731140017956079, 4.469926681468478158 ) ) ;
#19901=CARTESIAN_POINT ( 'NONE',  ( 87.44971815361896006, 45.51302063199200632, 7.049767141111613178 ) ) ;
#19903=VERTEX_POINT ( 'NONE', #82456 ) ;
#19908=CARTESIAN_POINT ( 'NONE',  ( 80.07812099633126479, 57.44764983040322193, -16.59488970948941500 ) ) ;
#19911=CYLINDRICAL_SURFACE ( 'NONE', #91177, 10.00000000000001066 ) ;
#19913=CARTESIAN_POINT ( 'NONE',  ( 82.09975393820661793, 49.29335735647264016, -13.66301205482166381 ) ) ;
#19915=CARTESIAN_POINT ( 'NONE',  ( 81.24979600617606934, 43.19334784728703625, 9.575909627378866418 ) ) ;
#19924=EDGE_LOOP ( 'NONE', ( #11337, #60085, #87555, #89998 ) ) ;
#19928=EDGE_LOOP ( 'NONE', ( #90848, #23230, #28709, #12809 ) ) ;
#19938=CARTESIAN_POINT ( 'NONE',  ( 77.81781567708489433, 56.70989197899351097, -16.20277462095411281 ) ) ;
#19951=CARTESIAN_POINT ( 'NONE',  ( 83.15864659133335124, 42.41990866257129511, 6.708876870822152227 ) ) ;
#19956=CARTESIAN_POINT ( 'NONE',  ( 82.56404520846588468, 41.04076960736067292, -1.149829612626004360 ) ) ;
#19958=CARTESIAN_POINT ( 'NONE',  ( 84.42755274236627372, 50.68105307249222591, 13.76233527223795683 ) ) ;
#19963=ORIENTED_EDGE ( 'NONE', *, *, #85464, .T. ) ;
#19965=CARTESIAN_POINT ( 'NONE',  ( 15.75562222995320560, 27.83478043621387599, -8.090169943749479842 ) ) ;
#19967=CARTESIAN_POINT ( 'NONE',  ( 74.45487526951390578, 66.04645349175549995, 13.54363770489549879 ) ) ;
#19971=CARTESIAN_POINT ( 'NONE',  ( 68.52675681298484278, 64.32790167916148505, 11.71367573677816942 ) ) ;
#19972=CARTESIAN_POINT ( 'NONE',  ( 74.09415402004458429, 67.86909550972291072, -11.62290297944830542 ) ) ;
#19982=FACE_OUTER_BOUND ( 'NONE', #76178, .T. ) ;
#19985=CARTESIAN_POINT ( 'NONE',  ( 72.52865609845331107, 57.51546068809462753, 16.29679984399868786 ) ) ;
#19992=CARTESIAN_POINT ( 'NONE',  ( 83.61470584636902004, 43.92523517391203569, 8.757796049109066061 ) ) ;
#19995=CARTESIAN_POINT ( 'NONE',  ( 28.62558104116610380, 25.03085787977764198, 9.188101187500006262 ) ) ;
#20001=FACE_OUTER_BOUND ( 'NONE', #58954, .T. ) ;
#20006=CARTESIAN_POINT ( 'NONE',  ( 81.96589639849747755, 58.75522159323007543, -0.2191855733945376195 ) ) ;
#20007=CARTESIAN_POINT ( 'NONE',  ( 81.47495714615762097, 55.16564477528429933, -15.92599370216107602 ) ) ;
#20008=ORIENTED_EDGE ( 'NONE', *, *, #74586, .T. ) ;
#20009=CARTESIAN_POINT ( 'NONE',  ( 71.60067202791792340, 71.17545373159485678, 4.829749188030544538 ) ) ;
#20010=CARTESIAN_POINT ( 'NONE',  ( 82.85376847310632797, 41.32516217177638396, -4.514684729415445297 ) ) ;
#20011=EDGE_CURVE ( 'NONE', #19304, #80050, #42737, .T. ) ;
#20013=CARTESIAN_POINT ( 'NONE',  ( 71.82608767971663610, 72.19311822168063486, 0.5755032799609223204 ) ) ;
#20014=CARTESIAN_POINT ( 'NONE',  ( 83.35959653392400526, 42.22915863639402545, 4.663558883483734263 ) ) ;
#20021=ORIENTED_EDGE ( 'NONE', *, *, #13240, .T. ) ;
#20023=CARTESIAN_POINT ( 'NONE',  ( 38.99862784774133218, 37.91421378149922816, 9.188101187500008038 ) ) ;
#20025=ORIENTED_EDGE ( 'NONE', *, *, #92930, .T. ) ;
#20032=CARTESIAN_POINT ( 'NONE',  ( 72.67905965592419193, 70.26320000030698054, -8.002569769838684621 ) ) ;
#20041=VERTEX_POINT ( 'NONE', #65573 ) ;
#20042=EDGE_CURVE ( 'NONE', #69466, #49291, #87519, .T. ) ;
#20049=DIRECTION ( 'NONE',  ( -0.8660254037844378194, -0.5000000000000013323, -0.000000000000000000 ) ) ;
#20052=CARTESIAN_POINT ( 'NONE',  ( 82.37238700568863692, 40.69398333026209258, 3.209141624528058845 ) ) ;
#20056=CARTESIAN_POINT ( 'NONE',  ( 19.47506710560450216, 33.01751292744056343, 6.180339887498949913 ) ) ;
#20058=DIRECTION ( 'NONE',  ( -0.1378186779084930869, 0.2387089523694814197, -0.9612616959383223358 ) ) ;
#20059=ORIENTED_EDGE ( 'NONE', *, *, #65690, .F. ) ;
#20060=CARTESIAN_POINT ( 'NONE',  ( 76.87919255693888942, 60.90556971193419145, 15.72099009421724602 ) ) ;
#20061=CARTESIAN_POINT ( 'NONE',  ( 14.00658445089738180, 13.80170272979924917, 7.433330006724137462 ) ) ;
#20064=CARTESIAN_POINT ( 'NONE',  ( 85.55975315002648074, 48.35019831671618817, -12.20940535940758132 ) ) ;
#20070=CARTESIAN_POINT ( 'NONE',  ( 84.85238324705348134, 49.19334207431751338, -13.14179292021528056 ) ) ;
#20073=CARTESIAN_POINT ( 'NONE',  ( 87.34045233512981099, 44.85499964951561225, 5.787806721962865275 ) ) ;
#20074=CARTESIAN_POINT ( 'NONE',  ( 88.06934480351134198, 44.11702129290613072, -1.709332125350027765 ) ) ;
#20077=CARTESIAN_POINT ( 'NONE',  ( 66.13500987590335001, 69.30841116337150254, 0.2424399591101732698 ) ) ;
#20083=FACE_OUTER_BOUND ( 'NONE', #1460, .T. ) ;
#20087=CARTESIAN_POINT ( 'NONE',  ( 88.11245462187771693, 44.31171394170508648, 2.759943262836158873 ) ) ;
#20090=ORIENTED_EDGE ( 'NONE', *, *, #30343, .F. ) ;
#20096=CARTESIAN_POINT ( 'NONE',  ( 66.99892443162359257, 66.90181954958814003, -8.791929524054854284 ) ) ;
#20098=CARTESIAN_POINT ( 'NONE',  ( 81.14781783016522354, 43.43044292088951863, -9.929167272279752154 ) ) ;
#20106=CARTESIAN_POINT ( 'NONE',  ( 77.86030215884842676, 50.85760040121600412, 15.26662539205169544 ) ) ;
#20107=CARTESIAN_POINT ( 'NONE',  ( 76.16157665297757262, 51.33368209758570799, 15.63302325843619478 ) ) ;
#20110=EDGE_CURVE ( 'NONE', #75490, #20280, #31546, .T. ) ;
#20111=CARTESIAN_POINT ( 'NONE',  ( 84.43973019491031096, 50.14528805649905507, 13.86389828189430062 ) ) ;
#20114=EDGE_CURVE ( 'NONE', #50302, #7411, #28218, .T. ) ;
#20120=CARTESIAN_POINT ( 'NONE',  ( 84.07324426729904587, 42.29269841712828537, -3.545903798621591996 ) ) ;
#20123=CARTESIAN_POINT ( 'NONE',  ( 36.95804531498377798, 23.19860640527294748, 2.839279412974134775 ) ) ;
#20124=CARTESIAN_POINT ( 'NONE',  ( 83.00815485991435594, 53.30142267139500234, 15.60062745561815589 ) ) ;
#20125=CARTESIAN_POINT ( 'NONE',  ( 74.42516694136719480, 55.76460849002628350, 16.59412675241640756 ) ) ;
#20127=CARTESIAN_POINT ( 'NONE',  ( 26.45569963029868177, 20.98920272979927049, 7.433330006724137462 ) ) ;
#20132=CARTESIAN_POINT ( 'NONE',  ( 70.96326928872720430, 61.01013475532322161, 14.52989670127069921 ) ) ;
#20133=DIRECTION ( 'NONE',  ( 0.03487823687205911238, -0.06041087834082882468, 0.9975640502598247528 ) ) ;
#20137=CARTESIAN_POINT ( 'NONE',  ( 87.34647367080899016, 44.99587983710786432, -6.159439337099199996 ) ) ;
#20141=CARTESIAN_POINT ( 'NONE',  ( 75.47390685083401252, 53.30987980041999919, 16.49587604864008838 ) ) ;
#20142=ORIENTED_EDGE ( 'NONE', *, *, #905, .F. ) ;
#20143=CARTESIAN_POINT ( 'NONE',  ( 70.08393322175207629, 63.28384585981274313, 13.68523560319354360 ) ) ;
#20147=CARTESIAN_POINT ( 'NONE',  ( 81.45101120633425751, 42.17020710753002533, -7.997091885120573451 ) ) ;
#20149=CARTESIAN_POINT ( 'NONE',  ( 86.26394923150375860, 43.12119067694047203, 1.349736823004491049 ) ) ;
#20159=CARTESIAN_POINT ( 'NONE',  ( 35.31080938399455249, 26.10170272979929607, -7.433330006724141015 ) ) ;
#20160=CARTESIAN_POINT ( 'NONE',  ( 73.37987013686270643, 60.48738129690996601, -15.24192514929477404 ) ) ;
#20166=CARTESIAN_POINT ( 'NONE',  ( 84.40498577231251431, 50.09068632715275271, 13.84414505597724521 ) ) ;
#20177=ORIENTED_EDGE ( 'NONE', *, *, #97538, .T. ) ;
#20183=CARTESIAN_POINT ( 'NONE',  ( 87.18478751182242092, 46.16420910987052650, -8.338078487178403719 ) ) ;
#20186=CARTESIAN_POINT ( 'NONE',  ( 16.97222724706317720, 11.92755873383624987, 6.180339887498953466 ) ) ;
#20187=PLANE ( 'NONE',  #51190 ) ;
#20192=ORIENTED_EDGE ( 'NONE', *, *, #71996, .F. ) ;
#20195=CARTESIAN_POINT ( 'NONE',  ( 82.17415024888090613, 44.43251709326036547, 9.654931585787190684 ) ) ;
#20197=CARTESIAN_POINT ( 'NONE',  ( 69.74385355405661358, 62.24098940029958271, -13.60094204340151158 ) ) ;
#20201=CARTESIAN_POINT ( 'NONE',  ( 71.24993629681053164, 61.94327900918170826, 14.19888696492397884 ) ) ;
#20202=CARTESIAN_POINT ( 'NONE',  ( 82.44819350194325125, 40.44303670712709931, -1.385655820001176597 ) ) ;
#20205=CARTESIAN_POINT ( 'NONE',  ( 75.98104421109889017, 51.53574906954565193, 16.18761828508177558 ) ) ;
#20208=CARTESIAN_POINT ( 'NONE',  ( 79.97334651676149520, 50.01100418247790458, 14.56762597300080841 ) ) ;
#20211=CARTESIAN_POINT ( 'NONE',  ( 77.74246467396064020, 62.00370236096145504, 15.64046932493554110 ) ) ;
#20213=VECTOR ( 'NONE', #68197, 1000.000000000000114 ) ;
#20216=B_SPLINE_CURVE_WITH_KNOTS ( 'NONE', 3,
 ( #85191, #20143, #60098, #98142, #21627, #10664, #75341, #25873, #91063, #67217, #74360, #49162, #80098, #29231, #87730, #98648 ),
 .UNSPECIFIED., .F., .F.,
 ( 4, 1, 2, 2, 2, 1, 2, 2, 4 ),
 ( 0.000000000000000000, 0.1250000000000018596, 0.1875000000000026645, 0.2500000000000034972, 0.5000000000000088818, 0.6250000000000092149, 0.6875000000000086597, 0.7500000000000082157, 1.000000000000000000 ),
 .UNSPECIFIED. ) ;
#20217=CARTESIAN_POINT ( 'NONE',  ( 71.31272509113929914, 71.01324172527584722, -4.873768137004467427 ) ) ;
#20221=CARTESIAN_POINT ( 'NONE',  ( 27.55345145191056488, 40.00034080476292786, -1.878358725466461243E-16 ) ) ;
#20224=CARTESIAN_POINT ( 'NONE',  ( 82.57051958873132946, 54.16786056752901857, 15.56146448981428776 ) ) ;
#20229=VERTEX_POINT ( 'NONE', #84072 ) ;
#20230=CARTESIAN_POINT ( 'NONE',  ( 87.37978634506822573, 45.87160741090568905, 8.420816086386249566 ) ) ;
#20232=CARTESIAN_POINT ( 'NONE',  ( 71.97942276284884144, 72.19511207240364570, -1.653363456454256974 ) ) ;
#20234=VECTOR ( 'NONE', #52389, 1000.000000000000000 ) ;
#20235=CARTESIAN_POINT ( 'NONE',  ( 86.79190430688251467, 45.84585087985657736, 8.866399834819148396 ) ) ;
#20238=CARTESIAN_POINT ( 'NONE',  ( 9.573022157908470220, 14.03085787977760646, 9.188101187500006262 ) ) ;
#20247=FACE_OUTER_BOUND ( 'NONE', #87399, .T. ) ;
#20250=VERTEX_POINT ( 'NONE', #45504 ) ;
#20255=CARTESIAN_POINT ( 'NONE',  ( 67.25371248956088266, 66.53894546794931841, -8.600501240181268159 ) ) ;
#20261=CARTESIAN_POINT ( 'NONE',  ( 32.07042461746584650, 33.91421378149919974, 9.188101187500008038 ) ) ;
#20266=CARTESIAN_POINT ( 'NONE',  ( 17.75393198606386136, 12.11110640527291160, -2.839279412974138328 ) ) ;
#20272=CARTESIAN_POINT ( 'NONE',  ( 76.61511796410523800, 54.31696088684743273, 16.52897461885082464 ) ) ;
#20276=ORIENTED_EDGE ( 'NONE', *, *, #20478, .F. ) ;
#20278=CARTESIAN_POINT ( 'NONE',  ( 82.21410988452117863, 40.73976263626466476, 3.762362152834606732 ) ) ;
#20280=VERTEX_POINT ( 'NONE', #37404 ) ;
#20281=CARTESIAN_POINT ( 'NONE',  ( 66.20320037398873581, 68.63009258879732499, -2.167961533895922610 ) ) ;
#20284=CARTESIAN_POINT ( 'NONE',  ( 78.13161584694131534, 61.81224900762369145, -15.72225761198293981 ) ) ;
#20297=CARTESIAN_POINT ( 'NONE',  ( 81.53661897590532703, 55.80016554358400072, 16.37044094275388417 ) ) ;
#20303=CARTESIAN_POINT ( 'NONE',  ( 70.17130392896066837, 64.17533599878278494, -12.55506970741091521 ) ) ;
#20304=CARTESIAN_POINT ( 'NONE',  ( 86.70355446391526755, 43.51144900434398721, -2.455171442191615316 ) ) ;
#20309=EDGE_CURVE ( 'NONE', #96180, #79774, #8462, .T. ) ;
#20317=ORIENTED_EDGE ( 'NONE', *, *, #62888, .F. ) ;
#20321=CARTESIAN_POINT ( 'NONE',  ( 81.35887266585007183, 44.29925860026666129, -10.01769064211159055 ) ) ;
#20322=CARTESIAN_POINT ( 'NONE',  ( 74.34676178584531669, 66.92609087214925978, -12.92232536950610289 ) ) ;
#20324=( BOUNDED_CURVE ( )  B_SPLINE_CURVE ( 2, ( #99412, #58878, #13797, #75608, #29989, #36090, #53289, #44184, #36587, #51288, #51812, #6196, #91832 ),
 .UNSPECIFIED., .F., .T. ) 
 B_SPLINE_CURVE_WITH_KNOTS ( ( 3, 2, 2, 2, 2, 2, 3 ),
 ( 0.8625000000000000444, 0.8649999999999999911, 0.8699999999999999956, 0.8750000000000000000, 0.8800000000000000044, 0.8850000000000000089, 0.8875000000000000666 ),
 .UNSPECIFIED. ) 
 CURVE ( )  GEOMETRIC_REPRESENTATION_ITEM ( )  RATIONAL_B_SPLINE_CURVE ( ( 0.9755282581475767101, 0.9755282581475772652, 1.000000000000000000, 0.9510565162951535312, 1.000000000000000000, 0.9510565162951535312, 1.000000000000000000, 0.9510565162951535312, 1.000000000000000000, 0.9510565162951535312, 1.000000000000000000, 0.9755282581475761550, 0.9755282581475767101 ) ) 
 REPRESENTATION_ITEM ( '' )  );
#20327=CARTESIAN_POINT ( 'NONE',  ( 75.11982177093736368, 62.93972712279792603, 14.81955472308038679 ) ) ;
#20330=CARTESIAN_POINT ( 'NONE',  ( 76.44304877299126133, 54.35907603249690112, 16.08959775360170141 ) ) ;
#20339=CARTESIAN_POINT ( 'NONE',  ( 15.42909579892843652, 33.00034080476290654, -1.878358725466461243E-16 ) ) ;
#20342=DIRECTION ( 'NONE',  ( -0.2347357813929480952, 0.4065742997269687908, 0.8829475928589233247 ) ) ;
#20344=ADVANCED_FACE ( 'NONE', ( #68371 ), #29678, .T. ) ;
#20356=CARTESIAN_POINT ( 'NONE',  ( 85.72142767485377135, 44.68916939864112692, 8.082118614619203001 ) ) ;
#20357=CARTESIAN_POINT ( 'NONE',  ( 27.11554978534049098, 17.78380873178787169, -6.180339887498949025 ) ) ;
#20358=CARTESIAN_POINT ( 'NONE',  ( 85.37538261767947745, 48.57005942898851458, 12.46403972397472337 ) ) ;
#20360=CARTESIAN_POINT ( 'NONE',  ( 72.30772874869472844, 72.01587971836859481, -3.568979074609765600 ) ) ;
#20361=CARTESIAN_POINT ( 'NONE',  ( 74.06184603777616360, 55.64324239481884860, -16.58750451651802393 ) ) ;
#20369=B_SPLINE_CURVE_WITH_KNOTS ( 'NONE', 3,
 ( #75699, #28087, #98511, #36176, #44766, #21014, #90939, #43775, #6784, #68574, #60461, #14871, #21489, #6286, #99001, #45274 ),
 .UNSPECIFIED., .F., .F.,
 ( 4, 1, 2, 2, 2, 1, 2, 2, 4 ),
 ( 0.000000000000000000, 0.1250000000000009159, 0.1874999999999999167, 0.2499999999999989453, 0.5000000000000002220, 0.6250000000000007772, 0.6875000000000014433, 0.7500000000000021094, 1.000000000000000000 ),
 .UNSPECIFIED. ) ;
#20372=CARTESIAN_POINT ( 'NONE',  ( 72.85625868234197355, 71.07309412281131245, -7.586526616956829727 ) ) ;
#20374=CARTESIAN_POINT ( 'NONE',  ( 33.10845880387886808, 31.06628583063843863, -9.188101187500006262 ) ) ;
#20381=CARTESIAN_POINT ( 'NONE',  ( 11.44039960990914651, 28.64646525600389282, -2.839279412974133887 ) ) ;
#20382=CARTESIAN_POINT ( 'NONE',  ( 71.48480579176157335, 72.35852322450823237, 1.080755764661545548 ) ) ;
#20383=CARTESIAN_POINT ( 'NONE',  ( 82.37037437367128234, 54.25728867273632261, 15.61855531662249419 ) ) ;
#20390=CARTESIAN_POINT ( 'NONE',  ( 27.73347817269569404, 16.41603393254326093, -1.583844403245362020 ) ) ;
#20391=CARTESIAN_POINT ( 'NONE',  ( 81.35225493641259220, 42.04531462148436560, 7.888897770668004128 ) ) ;
#20393=ORIENTED_EDGE ( 'NONE', *, *, #19417, .F. ) ;
#20395=CARTESIAN_POINT ( 'NONE',  ( 67.24554735707404518, 69.34905625991120814, 1.330410485716284397 ) ) ;
#20397=CARTESIAN_POINT ( 'NONE',  ( 66.77752810875767864, 68.40544692769398694, 4.459354299965309743 ) ) ;
#20400=ORIENTED_EDGE ( 'NONE', *, *, #22167, .T. ) ;
#20405=CARTESIAN_POINT ( 'NONE',  ( 88.12308754723774484, 43.81089488678613009, -2.128676964009123651 ) ) ;
#20406=CARTESIAN_POINT ( 'NONE',  ( 80.50883317518791671, 57.72730120993125524, 16.59589928958307326 ) ) ;
#20410=CARTESIAN_POINT ( 'NONE',  ( 78.83915903249749135, 50.24778389138201362, -14.90005401999855295 ) ) ;
#20415=VECTOR ( 'NONE', #45830, 1000.000000000000114 ) ;
#20416=CARTESIAN_POINT ( 'NONE',  ( 73.94609423987252228, 60.77720215842664686, 15.26334679630400259 ) ) ;
#20417=EDGE_LOOP ( 'NONE', ( #65504, #18088, #9084, #5464 ) ) ;
#20425=EDGE_LOOP ( 'NONE', ( #99903, #7799, #100018, #2495 ) ) ;
#20426=CARTESIAN_POINT ( 'NONE',  ( 73.07250412799626815, 69.64252590750851368, 9.183134884877944160 ) ) ;
#20428=CARTESIAN_POINT ( 'NONE',  ( 83.01075186827047503, 53.40825386585735401, 15.63370843945822664 ) ) ;
#20434=CARTESIAN_POINT ( 'NONE',  ( 77.02178492951776434, 57.00973823531708717, -16.18317106599237221 ) ) ;
#20435=CARTESIAN_POINT ( 'NONE',  ( 77.47012825831066607, 49.73992442231940458, -15.48190979613537799 ) ) ;
#20440=CARTESIAN_POINT ( 'NONE',  ( 87.63467585155270001, 44.53258862333366608, 5.717273570526079318 ) ) ;
#20442=CARTESIAN_POINT ( 'NONE',  ( 71.49018766940498892, 68.39238998699252647, 9.502106742351175583 ) ) ;
#20443=CARTESIAN_POINT ( 'NONE',  ( 86.09778053344243176, 44.42558544415346944, 7.284472041480639426 ) ) ;
#20450=CARTESIAN_POINT ( 'NONE',  ( 85.21461723709045089, 46.08533025597601807, 10.27714634765069057 ) ) ;
#20465=ADVANCED_FACE ( 'NONE', ( #49081 ), #70884, .T. ) ;
#20466=CARTESIAN_POINT ( 'NONE',  ( 70.71732918945153301, 71.45486987150104596, -1.088542012041604945 ) ) ;
#20476=B_SPLINE_CURVE_WITH_KNOTS ( 'NONE', 3,
 ( #19290, #89707, #50643, #58731, #44531, #12165, #35452, #5552, #82105, #11677 ),
 .UNSPECIFIED., .F., .F.,
 ( 4, 2, 2, 2, 4 ),
 ( 0.000000000000000000, 0.0002622400424273775392, 0.0005244800848547550784, 0.0007867201272821326176, 0.001048960169709510157 ),
 .UNSPECIFIED. ) ;
#20478=EDGE_CURVE ( 'NONE', #63734, #25515, #17266, .T. ) ;
#20482=CARTESIAN_POINT ( 'NONE',  ( 73.80638704669732419, 68.31061168272384521, -11.57820046455322149 ) ) ;
#20484=CARTESIAN_POINT ( 'NONE',  ( 81.13898030988220000, 55.16162329238864004, 16.30930592844974569 ) ) ;
#20485=CARTESIAN_POINT ( 'NONE',  ( 71.62205979867658812, 59.06269311622425988, -15.34006186618645273 ) ) ;
#20486=CARTESIAN_POINT ( 'NONE',  ( 71.92052582790191195, 72.15815999434336447, -1.685033094989828228 ) ) ;
#20491=CARTESIAN_POINT ( 'NONE',  ( 71.76351473723394747, 71.84897031608997509, 2.971691788643012977 ) ) ;
#20492=CARTESIAN_POINT ( 'NONE',  ( 66.06994105266723238, 68.53505336611841869, -4.562350030803943746 ) ) ;
#20498=CARTESIAN_POINT ( 'NONE',  ( 28.09632999608277615, 19.14754757982091604, -5.678558825948276656 ) ) ;
#20499=CARTESIAN_POINT ( 'NONE',  ( 83.62455065227555906, 52.34512318633653649, -15.13772682721065621 ) ) ;
#20500=CARTESIAN_POINT ( 'NONE',  ( 71.88281838930642209, 59.56282477439597756, -15.74156321294392313 ) ) ;
#20502=CARTESIAN_POINT ( 'NONE',  ( 74.78994931159289195, 67.11760897871008069, 12.96302903502453852 ) ) ;
#20511=CARTESIAN_POINT ( 'NONE',  ( 69.78176895985124872, 68.40769324273578889, 8.076221664042178006 ) ) ;
#20514=CARTESIAN_POINT ( 'NONE',  ( 84.25291518742466224, 43.27603625466485227, 6.026143753377182222 ) ) ;
#20520=CARTESIAN_POINT ( 'NONE',  ( 9.089523648746947515, 28.18080186712591484, 3.090169943749475401 ) ) ;
#20521=CARTESIAN_POINT ( 'NONE',  ( 84.21906065053772750, 49.13438831735580692, 13.33485874824731887 ) ) ;
#20522=ORIENTED_EDGE ( 'NONE', *, *, #71582, .T. ) ;
#20523=CARTESIAN_POINT ( 'NONE',  ( 73.67256625907812406, 55.34600686115704349, 16.59066767443098911 ) ) ;
#20524=CARTESIAN_POINT ( 'NONE',  ( 86.17560058389634037, 46.94341623220315540, -10.60084123426473113 ) ) ;
#20538=CARTESIAN_POINT ( 'NONE',  ( 81.38242352901214360, 41.99299366561535862, -7.776076777262098005 ) ) ;
#20543=CARTESIAN_POINT ( 'NONE',  ( 80.60080754873929720, 47.19651915616773152, 12.86587752985571420 ) ) ;
#20544=ORIENTED_EDGE ( 'NONE', *, *, #22284, .T. ) ;
#20554=CARTESIAN_POINT ( 'NONE',  ( 73.20575453205489680, 68.08741268818161529, -10.93745744334090908 ) ) ;
#20556=CARTESIAN_POINT ( 'NONE',  ( 76.33261713024396045, 57.84772012576796385, 16.09447198771029619 ) ) ;
#20557=CARTESIAN_POINT ( 'NONE',  ( 12.79414888559916719, 13.10170272979925166, -7.433330006724141015 ) ) ;
#20566=CARTESIAN_POINT ( 'NONE',  ( 70.50919596007410917, 60.88441437683223256, 14.47383098058850948 ) ) ;
#20567=VECTOR ( 'NONE', #62848, 1000.000000000000114 ) ;
#20570=CARTESIAN_POINT ( 'NONE',  ( 88.24711315651565258, 44.33861006782984759, -2.398047594449144615 ) ) ;
#20571=ORIENTED_EDGE ( 'NONE', *, *, #31289, .F. ) ;
#20573=CARTESIAN_POINT ( 'NONE',  ( 77.01640707515133499, 61.48716887149203814, -15.64119200545269983 ) ) ;
#20581=CARTESIAN_POINT ( 'NONE',  ( 87.88164403350640441, 44.18371841277615175, 2.790213129378243728 ) ) ;
#20584=ORIENTED_EDGE ( 'NONE', *, *, #98161, .F. ) ;
#20590=CARTESIAN_POINT ( 'NONE',  ( 70.81643854103050728, 70.50536786476077111, 6.457179250934519388 ) ) ;
#20596=CARTESIAN_POINT ( 'NONE',  ( 79.10786694755505266, 56.92203217398106574, 16.19829027401005206 ) ) ;
#20604=CARTESIAN_POINT ( 'NONE',  ( 84.40498577231251431, 50.09068632715275271, 13.84414505597724521 ) ) ;
#20610=DIRECTION ( 'NONE',  ( -0.5000000000000013323, 0.8660254037844379305, 0.000000000000000000 ) ) ;
#20612=CARTESIAN_POINT ( 'NONE',  ( 7.127696690345725727, 16.06628583063839244, -9.188101187500006262 ) ) ;
#20617=CARTESIAN_POINT ( 'NONE',  ( 75.67456858315887303, 65.42170317558291970, 14.28506259273864210 ) ) ;
#20619=CARTESIAN_POINT ( 'NONE',  ( 39.87427548755113094, 25.94754757982092741, 5.678558825948272215 ) ) ;
#20623=CARTESIAN_POINT ( 'NONE',  ( 20.18904385193075868, 29.84336893147756342, -7.433330006724137462 ) ) ;
#20629=CARTESIAN_POINT ( 'NONE',  ( 70.65831043835135006, 60.85253071434844685, 14.52235072827622098 ) ) ;
#20630=CARTESIAN_POINT ( 'NONE',  ( 76.03787485198571972, 65.47122818424047352, -14.36642907054480744 ) ) ;
#20634=CARTESIAN_POINT ( 'NONE',  ( 69.42144788871625849, 62.89730317705431872, 13.10748580973936939 ) ) ;
#20640=CARTESIAN_POINT ( 'NONE',  ( 87.10115137904762150, 45.28340438443854055, 6.995308688534716879 ) ) ;
#20649=CARTESIAN_POINT ( 'NONE',  ( 41.71939737199939202, 29.80170272979930246, 7.433330006724137462 ) ) ;
#20650=CARTESIAN_POINT ( 'NONE',  ( 77.74639646092859380, 59.02570175780747519, -16.09564583426548978 ) ) ;
#20653=CARTESIAN_POINT ( 'NONE',  ( 87.25569243610996750, 45.44211441089371561, 7.127650669554064677 ) ) ;
#20655=ORIENTED_EDGE ( 'NONE', *, *, #76077, .T. ) ;
#20659=CARTESIAN_POINT ( 'NONE',  ( 85.31220642273653709, 48.47216915277315508, 12.41700016606928259 ) ) ;
#20661=CARTESIAN_POINT ( 'NONE',  ( 77.85362458321634449, 59.68407148126515693, -16.06148647132319240 ) ) ;
#20662=CARTESIAN_POINT ( 'NONE',  ( 82.12141333937209708, 40.78733220434117612, 1.186632920674746794 ) ) ;
#20665=CARTESIAN_POINT ( 'NONE',  ( 76.86303881961467255, 63.31387137873053916, -15.46595148530503927 ) ) ;
#20666=CARTESIAN_POINT ( 'NONE',  ( 78.91446233654380649, 59.71533271261715470, 16.49719907270641883 ) ) ;
#20675=CARTESIAN_POINT ( 'NONE',  ( 87.06644787366251137, 45.96331769923622801, -8.152425090918923090 ) ) ;
#20677=CARTESIAN_POINT ( 'NONE',  ( 86.12135434523638366, 46.98046262810483142, -10.13131473785488090 ) ) ;
#20678=B_SPLINE_SURFACE_WITH_KNOTS ( 'NONE', 3, 1, ( 
 ( #93840, #9717 ),
 ( #16785, #55759 ),
 ( #41067, #87767 ),
 ( #31977, #64392 ),
 ( #94824, #18305 ),
 ( #47674, #24393 ),
 ( #49204, #10204 ),
 ( #62881, #78607 ),
 ( #55267, #72005 ),
 ( #80137, #63390 ),
 ( #24883, #86247 ),
 ( #71512, #1099 ),
 ( #34014, #9193 ),
 ( #2609, #32499 ),
 ( #48704, #95356 ),
 ( #64899, #40068 ),
 ( #86751, #71011 ),
 ( #25388, #25911 ),
 ( #33497, #17285 ),
 ( #32984, #1613 ),
 ( #10701, #8692 ),
 ( #63888, #56783 ),
 ( #79637, #94330 ),
 ( #48189, #41579 ),
 ( #95845, #2103 ),
 ( #79136, #72520 ),
 ( #26401, #3129 ),
 ( #40572, #56276 ),
 ( #87274, #17804 ),
 ( #57277, #88254 ),
 ( #18801, #49684 ) ),
 .UNSPECIFIED., .F., .F., .F.,
 ( 4, 3, 3, 3, 3, 3, 3, 3, 3, 3, 4 ),
 ( 2, 2 ),
 ( 0.000000000000000000, 0.1333490885032357076, 0.3007194338854359827, 0.4699862290245028773, 0.5844252810809169585, 0.6686540514502661292, 0.7354980260655498148, 0.8028463152565713523, 0.8633854507757302565, 0.9437142632667330222, 1.000000000000000000 ),
 ( 0.000000000000000000, 1.000000000000000000 ),
 .UNSPECIFIED. ) ;
#20680=CARTESIAN_POINT ( 'NONE',  ( 25.48331929688331599, 38.21091486745862653, 7.012934429366973338E-14 ) ) ;
#20690=CARTESIAN_POINT ( 'NONE',  ( 67.18057841095335903, 68.85678461590420341, -3.812741676141380154 ) ) ;
#20692=FACE_OUTER_BOUND ( 'NONE', #34231, .T. ) ;
#20693=CARTESIAN_POINT ( 'NONE',  ( 77.08943580299947484, 49.61595851769167353, 15.51385818994994459 ) ) ;
#20696=CARTESIAN_POINT ( 'NONE',  ( 88.22000632671873177, 44.27423112938744509, 4.003506518527982116 ) ) ;
#20697=CARTESIAN_POINT ( 'NONE',  ( 82.68211672025338999, 52.94826342379619177, 15.15574935255376232 ) ) ;
#20703=CARTESIAN_POINT ( 'NONE',  ( 71.96027346690365789, 72.28811235517684963, 3.313491923126954841 ) ) ;
#20707=CARTESIAN_POINT ( 'NONE',  ( 80.92134340239459789, 55.42731787558462031, 16.01308592331401925 ) ) ;
#20709=CARTESIAN_POINT ( 'NONE',  ( 68.18512844359727865, 69.81902233912992983, -2.062004031463703591 ) ) ;
#20717=B_SPLINE_CURVE_WITH_KNOTS ( 'NONE', 3,
 ( #94119, #40359, #16574, #24672 ),
 .UNSPECIFIED., .F., .F.,
 ( 4, 4 ),
 ( 0.000000000000000000, 0.007499696492506968508 ),
 .UNSPECIFIED. ) ;
#20722=CARTESIAN_POINT ( 'NONE',  ( 12.43831579814173693, 15.38052372038639071, 10.00000000000000533 ) ) ;
#20723=CARTESIAN_POINT ( 'NONE',  ( 36.72872667615778397, 36.90829794293883026, 10.00000000000000355 ) ) ;
#20724=CARTESIAN_POINT ( 'NONE',  ( 81.22979812886450190, 55.45288652294036069, -16.34461090620092349 ) ) ;
#20726=CARTESIAN_POINT ( 'NONE',  ( 72.13517842779845068, 72.31474564102330760, 3.615969315562344910 ) ) ;
#20728=CARTESIAN_POINT ( 'NONE',  ( 69.60933530497638344, 70.67006034057621378, 4.325380387426783102 ) ) ;
#20734=CARTESIAN_POINT ( 'NONE',  ( 33.07613030564196777, 37.83478043621391151, -8.090169943749479842 ) ) ;
#20740=CARTESIAN_POINT ( 'NONE',  ( 10.26584248093601737, 14.43085787977761036, -9.188101187500008038 ) ) ;
#20745=CARTESIAN_POINT ( 'NONE',  ( 73.21559929719344950, 63.73101106623266077, 13.92201872992145084 ) ) ;
#20746=CARTESIAN_POINT ( 'NONE',  ( 68.11513882967693689, 67.84287964856595465, -7.395662205818876345 ) ) ;
#20750=CARTESIAN_POINT ( 'NONE',  ( 87.71554304996901408, 45.29005973903561966, -7.157883044737483047 ) ) ;
#20756=VERTEX_POINT ( 'NONE', #7835 ) ;
#20765=CARTESIAN_POINT ( 'NONE',  ( 36.08541434599421649, 23.76004757982091320, 5.678558825948272215 ) ) ;
#20767=CARTESIAN_POINT ( 'NONE',  ( 86.48142457384331294, 47.12364270815633205, -10.06370626518989830 ) ) ;
#20770=CARTESIAN_POINT ( 'NONE',  ( 20.98529944902502820, 27.51421378149918695, -9.188101187500004485 ) ) ;
#20771=CARTESIAN_POINT ( 'NONE',  ( 28.12420092063944921, 24.43677371833803136, -10.00000000000000355 ) ) ;
#20772=CARTESIAN_POINT ( 'NONE',  ( 71.10390369104861463, 70.26795136552352972, -6.302501079447722532 ) ) ;
#20782=CARTESIAN_POINT ( 'NONE',  ( 71.59328461577142377, 71.47600564087022690, -5.278543987517691605 ) ) ;
#20784=CARTESIAN_POINT ( 'NONE',  ( 65.98617016278960534, 69.07574344600425320, -2.064703022102583940 ) ) ;
#20802=CARTESIAN_POINT ( 'NONE',  ( 81.55638901470594249, 55.99673023569365427, 16.04557931222332101 ) ) ;
#20805=EDGE_CURVE ( 'NONE', #65643, #94602, #14947, .T. ) ;
#20807=EDGE_LOOP ( 'NONE', ( #1795, #60860, #38261, #70605 ) ) ;
#20809=CARTESIAN_POINT ( 'NONE',  ( 87.07071992409855454, 43.63667771387513028, -1.980884226090577238 ) ) ;
#20811=CARTESIAN_POINT ( 'NONE',  ( 66.46251910857498046, 68.82904070585031775, -4.353565755910135948 ) ) ;
#20814=CARTESIAN_POINT ( 'NONE',  ( 77.86555730066852732, 62.20866292688850052, -15.95979438352862445 ) ) ;
#20815=CARTESIAN_POINT ( 'NONE',  ( 76.08286921349539966, 51.17209099756131252, -15.60946675595210387 ) ) ;
#20817=VECTOR ( 'NONE', #75051, 999.9999999999998863 ) ;
#20818=CARTESIAN_POINT ( 'NONE',  ( 78.75297625639956323, 47.66336229257159118, 14.29739783539339371 ) ) ;
#20827=CARTESIAN_POINT ( 'NONE',  ( 66.60661563016273590, 67.77273566365288104, -7.043189648870076702 ) ) ;
#20829=CARTESIAN_POINT ( 'NONE',  ( 79.16557600000783168, 59.08901585114728050, -16.21880825576194951 ) ) ;
#20838=CARTESIAN_POINT ( 'NONE',  ( 80.87089094628977648, 50.87823725607803027, 14.71529395728275347 ) ) ;
#20846=CARTESIAN_POINT ( 'NONE',  ( 18.00728827979274627, 29.13478043621388380, 8.090169943749478065 ) ) ;
#20850=CARTESIAN_POINT ( 'NONE',  ( 68.21406460964578855, 69.18034937236612336, -6.080108713557645039 ) ) ;
#20852=CARTESIAN_POINT ( 'NONE',  ( 72.23520231138428471, 71.91245603983271906, -3.821936190094874508 ) ) ;
#20856=CARTESIAN_POINT ( 'NONE',  ( 66.77848686889967667, 67.34565621990024908, -6.901698923710801736 ) ) ;
#20859=B_SPLINE_CURVE_WITH_KNOTS ( 'NONE', 3,
 ( #47635, #94785, #48147, #41028 ),
 .UNSPECIFIED., .F., .F.,
 ( 4, 4 ),
 ( 0.000000000000000000, 0.02192660554268253612 ),
 .UNSPECIFIED. ) ;
#20861=CARTESIAN_POINT ( 'NONE',  ( 22.27692774695706035, 28.56454794089041727, 10.00000000000000355 ) ) ;
#20862=CARTESIAN_POINT ( 'NONE',  ( 85.73895798293081327, 48.63177274617319057, 12.34992197344710796 ) ) ;
#20864=CARTESIAN_POINT ( 'NONE',  ( 71.97191893240673721, 71.74017062233478725, -3.901372815243289160 ) ) ;
#20879=CARTESIAN_POINT ( 'NONE',  ( 42.56377214068922399, 30.28920272979930672, -7.433330006724141015 ) ) ;
#20887=CARTESIAN_POINT ( 'NONE',  ( 9.333682440526761326, 28.49540643055185640, 3.479690158560446702E-15 ) ) ;
#20888=CARTESIAN_POINT ( 'NONE',  ( 71.97456596565470477, 72.60744930783873485, 1.463844530419971868 ) ) ;
#20889=FACE_OUTER_BOUND ( 'NONE', #39470, .T. ) ;
#20896=CARTESIAN_POINT ( 'NONE',  ( 74.91545508103216378, 53.41488691832748259, -16.53475931695716028 ) ) ;
#20900=CARTESIAN_POINT ( 'NONE',  ( 67.88857314316685176, 69.78661589965172141, 0.4887884946192302404 ) ) ;
#20901=B_SPLINE_CURVE_WITH_KNOTS ( 'NONE', 3,
 ( #31461, #38053, #76582, #52761, #92322, #14281, #29483, #7166, #21875, #68966, #38562, #67981, #83723, #99889, #39050, #53274 ),
 .UNSPECIFIED., .F., .F.,
 ( 4, 1, 2, 2, 2, 1, 2, 2, 4 ),
 ( 0.000000000000000000, 0.1249999999999952538, 0.1874999999999950873, 0.2499999999999949485, 0.4999999999999948930, 0.6249999999999962252, 0.6874999999999970024, 0.7499999999999976685, 1.000000000000000000 ),
 .UNSPECIFIED. ) ;
#20905=AXIS2_PLACEMENT_3D ( 'NONE', #65476, #43148, #95447 ) ;
#20913=CARTESIAN_POINT ( 'NONE',  ( 80.48345259418954356, 57.73457509892514139, -16.59664598758602949 ) ) ;
#20914=CARTESIAN_POINT ( 'NONE',  ( 68.74157960831310277, 69.68624548565989585, -5.631338930608605686 ) ) ;
#20916=CARTESIAN_POINT ( 'NONE',  ( 87.30643095423958755, 44.98864145313458351, -6.191042897133923084 ) ) ;
#20920=CARTESIAN_POINT ( 'NONE',  ( 80.88056646709152631, 43.02648916431432724, 9.632536512155043695 ) ) ;
#20921=EDGE_LOOP ( 'NONE', ( #82746, #71136, #14264, #75238 ) ) ;
#20923=CARTESIAN_POINT ( 'NONE',  ( 74.29078308660947982, 62.27531838756304694, 14.84303450056853180 ) ) ;
#20935=CARTESIAN_POINT ( 'NONE',  ( 73.36558254226180509, 69.84094749084881926, 9.147675672628972521 ) ) ;
#20943=EDGE_LOOP ( 'NONE', ( #96596, #67118, #9129, #28022 ) ) ;
#20947=CARTESIAN_POINT ( 'NONE',  ( 67.24983238577166844, 66.59130585728682661, 8.524349129767776034 ) ) ;
#20953=CARTESIAN_POINT ( 'NONE',  ( 77.95341167405027250, 53.58435032990927738, -15.90803922215739163 ) ) ;
#20955=CARTESIAN_POINT ( 'NONE',  ( 79.64486573815776183, 45.90865440701455213, 12.93595385939046594 ) ) ;
#20960=CARTESIAN_POINT ( 'NONE',  ( 82.35975313173908319, 41.41624149291902057, 5.521678208619409389 ) ) ;
#20977=CARTESIAN_POINT ( 'NONE',  ( 81.87680903571094859, 41.76738865979471171, -5.626291927274185589 ) ) ;
#20981=CARTESIAN_POINT ( 'NONE',  ( 68.61209271804665377, 64.17778009964139585, -12.50907296292702320 ) ) ;
#20983=B_SPLINE_SURFACE_WITH_KNOTS ( 'NONE', 3, 1, ( 
 ( #33074, #48278 ),
 ( #85846, #87361 ),
 ( #47754, #8279 ),
 ( #71095, #55352 ),
 ( #16869, #1183 ),
 ( #78692, #9797 ),
 ( #38667, #77696 ),
 ( #31061, #32059 ),
 ( #31557, #24965 ),
 ( #40658, #71595 ),
 ( #17371, #69570 ),
 ( #17890, #39146 ),
 ( #62970, #70058 ),
 ( #94411, #61951 ),
 ( #78187, #675 ),
 ( #63967, #25472 ),
 ( #16373, #77172 ),
 ( #9280, #62446 ),
 ( #1694, #86330 ),
 ( #40154, #93919 ),
 ( #32578, #56363 ),
 ( #93415, #23964 ),
 ( #7776, #178 ),
 ( #47265, #92903 ),
 ( #24473, #23454 ),
 ( #55842, #54346 ),
 ( #8775, #85318 ),
 ( #86837, #15863 ),
 ( #46772, #54865 ),
 ( #39645, #70566 ),
 ( #89804, #64478 ) ),
 .UNSPECIFIED., .F., .F., .F.,
 ( 4, 3, 3, 3, 3, 3, 3, 3, 3, 3, 4 ),
 ( 2, 2 ),
 ( 0.000000000000000000, 0.1122669598086860482, 0.2243161639709787269, 0.3396355846219236696, 0.4553962076585217345, 0.5677860799922416213, 0.6749047109689670920, 0.7773884377078438268, 0.8775581155834327740, 0.9782364162377975569, 1.000000000000000000 ),
 ( 0.000000000000000000, 1.000000000000000000 ),
 .UNSPECIFIED. ) ;
#20991=CARTESIAN_POINT ( 'NONE',  ( 71.29758602155226299, 68.80057128787699128, -9.575873472329016423 ) ) ;
#20992=CARTESIAN_POINT ( 'NONE',  ( 80.62260327750492195, 51.59452065496885353, 15.50740165936294801 ) ) ;
#20993=CARTESIAN_POINT ( 'NONE',  ( 71.61825016222245210, 59.02498431978696658, -15.35031316840264459 ) ) ;
#20994=CARTESIAN_POINT ( 'NONE',  ( 66.77376812102318127, 68.41195941748605946, -4.433129028897194068 ) ) ;
#20998=CARTESIAN_POINT ( 'NONE',  ( 69.87062716920111427, 69.39590680716997895, 6.536137438613790707 ) ) ;
#21004=CARTESIAN_POINT ( 'NONE',  ( 25.85429974905589745, 23.43085787977764056, -9.188101187500008038 ) ) ;
#21006=CARTESIAN_POINT ( 'NONE',  ( 83.58053473790808141, 52.37444464214736684, -15.15899823554475212 ) ) ;
#21007=CARTESIAN_POINT ( 'NONE',  ( 74.98034739464185350, 53.37963118822899133, -16.04958843571116134 ) ) ;
#21010=CARTESIAN_POINT ( 'NONE',  ( 69.13437078241847189, 64.31265921892629933, 12.00033174088420118 ) ) ;
#21014=CARTESIAN_POINT ( 'NONE',  ( 69.35136632105268006, 67.21048502454044637, -10.10453561268904821 ) ) ;
#21017=CARTESIAN_POINT ( 'NONE',  ( 71.72012509582434348, 71.32916523519146779, 4.604336662656719703 ) ) ;
#21019=CARTESIAN_POINT ( 'NONE',  ( 71.89891490226827386, 72.23425543116729841, 0.5890436832873462425 ) ) ;
#21020=CYLINDRICAL_SURFACE ( 'NONE', #99173, 10.00000000000001066 ) ;
#21023=CARTESIAN_POINT ( 'NONE',  ( 67.45371725586859668, 68.64851772114370476, 4.944568755435953200 ) ) ;
#21028=CARTESIAN_POINT ( 'NONE',  ( 13.32519098795206780, 19.64441083166259361, -10.00000000000000533 ) ) ;
#21029=CARTESIAN_POINT ( 'NONE',  ( 83.13824623788876522, 45.58899862045078066, 11.00933188051684297 ) ) ;
#21030=EDGE_LOOP ( 'NONE', ( #93814, #3014, #36229, #100155 ) ) ;
#21043=CARTESIAN_POINT ( 'NONE',  ( 72.84093999290330146, 56.97456911652175648, -16.40692799624909171 ) ) ;
#21045=ORIENTED_EDGE ( 'NONE', *, *, #58865, .T. ) ;
#21050=CARTESIAN_POINT ( 'NONE',  ( 81.81818204529017180, 52.08743214072829630, 15.02062431075104598 ) ) ;
#21052=EDGE_CURVE ( 'NONE', #59353, #77173, #95703, .T. ) ;
#21057=CARTESIAN_POINT ( 'NONE',  ( 82.66373328861170933, 40.87911596418215510, 3.282672455158152314 ) ) ;
#21060=EDGE_CURVE ( 'NONE', #37680, #24001, #47359, .T. ) ;
#21063=CARTESIAN_POINT ( 'NONE',  ( 70.83016151729651710, 68.41586035902774654, -8.977235470963222497 ) ) ;
#21066=CARTESIAN_POINT ( 'NONE',  ( 76.40286963592521374, 58.21049690025673584, 16.06783727834804409 ) ) ;
#21067=CARTESIAN_POINT ( 'NONE',  ( 4.137530017820134631, 25.49540643055185285, 3.479690158560446702E-15 ) ) ;
#21078=CARTESIAN_POINT ( 'NONE',  ( 85.86558718211738039, 43.20781965171007499, 3.226128779682295722 ) ) ;
#21079=CARTESIAN_POINT ( 'NONE',  ( 88.28703488708569580, 44.33872872310907809, -2.279783701773686388 ) ) ;
#21080=ORIENTED_EDGE ( 'NONE', *, *, #9616, .T. ) ;
#21082=B_SPLINE_CURVE_WITH_KNOTS ( 'NONE', 3,
 ( #71933, #18727, #79565, #81551, #63816, #88180 ),
 .UNSPECIFIED., .F., .F.,
 ( 4, 2, 4 ),
 ( 0.000000000000000000, 0.2986716297182049340, 0.5973432594364098680 ),
 .UNSPECIFIED. ) ;
#21083=CARTESIAN_POINT ( 'NONE',  ( 75.08013308270210473, 67.09339902234965791, -13.09435070823462866 ) ) ;
#21088=CARTESIAN_POINT ( 'NONE',  ( 83.69930633818603383, 44.66246776289806064, -8.864960664055317352 ) ) ;
#21097=CARTESIAN_POINT ( 'NONE',  ( 85.62951787902757417, 48.90316132097375856, -12.13537779016860085 ) ) ;
#21098=CARTESIAN_POINT ( 'NONE',  ( 67.00368147268072505, 66.95831323777278499, -8.716692028962587102 ) ) ;
#21100=CARTESIAN_POINT ( 'NONE',  ( 70.32555767554718784, 69.76210374709671669, 7.334934889506363298 ) ) ;
#21105=CARTESIAN_POINT ( 'NONE',  ( 78.16778150852306339, 52.08950074027319488, 15.56147700446086013 ) ) ;
#21106=B_SPLINE_CURVE_WITH_KNOTS ( 'NONE', 3,
 ( #77759, #47328, #41220, #93979, #79292, #18457, #62514, #40214, #9863, #8342 ),
 .UNSPECIFIED., .F., .F.,
 ( 4, 2, 2, 2, 4 ),
 ( 0.000000000000000000, 0.0002622400424271630840, 0.0005244800848543261680, 0.0007867201272814892520, 0.001048960169708652336 ),
 .UNSPECIFIED. ) ;
#21110=LINE ( 'NONE', #43872, #77672 ) ;
#21113=CARTESIAN_POINT ( 'NONE',  ( 85.05685448785742153, 49.86430017123296210, 13.48384481714161787 ) ) ;
#21122=CARTESIAN_POINT ( 'NONE',  ( 6.742211794378569323, 25.93396525600388003, 2.839279412974139660 ) ) ;
#21123=CARTESIAN_POINT ( 'NONE',  ( 84.55537670905214043, 50.62155581810766591, -14.09136642048689936 ) ) ;
#21129=CARTESIAN_POINT ( 'NONE',  ( 32.54976882715482134, 40.83396525600392835, -2.839279412974133887 ) ) ;
#21131=FACE_BOUND ( 'NONE', #20943, .T. ) ;
#21132=ORIENTED_EDGE ( 'NONE', *, *, #72048, .T. ) ;
#21133=CARTESIAN_POINT ( 'NONE',  ( 28.29779127713939602, 18.19860640527293327, 2.839279412974134775 ) ) ;
#21134=CARTESIAN_POINT ( 'NONE',  ( 17.29678581741014654, 10.39040679176981996, 1.333680081654574804E-15 ) ) ;
#21138=CARTESIAN_POINT ( 'NONE',  ( 70.94564442840402307, 61.10112560036777296, 15.01654231012169483 ) ) ;
#21142=CARTESIAN_POINT ( 'NONE',  ( 75.11446029513938072, 52.98301679529475905, -16.48354851564725365 ) ) ;
#21146=CARTESIAN_POINT ( 'NONE',  ( 86.10138557494317979, 45.87410591191778053, -9.436449708986739182 ) ) ;
#21147=ORIENTED_EDGE ( 'NONE', *, *, #36945, .F. ) ;
#21158=CARTESIAN_POINT ( 'NONE',  ( 42.23901261427005949, 30.10170272979930672, -7.433330006724141015 ) ) ;
#21159=CARTESIAN_POINT ( 'NONE',  ( 77.93566872935365097, 58.95233904213321097, -16.11642214640332327 ) ) ;
#21162=CARTESIAN_POINT ( 'NONE',  ( 87.64900631941344500, 45.32217229061651409, 6.433208773102475853 ) ) ;
#21164=ORIENTED_EDGE ( 'NONE', *, *, #54057, .F. ) ;
#21165=CARTESIAN_POINT ( 'NONE',  ( 81.65310433048475147, 42.64019311979919280, 7.560891536010023728 ) ) ;
#21170=CARTESIAN_POINT ( 'NONE',  ( 73.51647790488874534, 61.26934504900349054, -15.03881460934114678 ) ) ;
#21171=CARTESIAN_POINT ( 'NONE',  ( 82.32345403531087413, 40.35629778586039151, 1.222851117235266960 ) ) ;
#21174=CARTESIAN_POINT ( 'NONE',  ( 76.95483076014906487, 63.96668203270510134, -15.25269828761453894 ) ) ;
#21187=ORIENTED_EDGE ( 'NONE', *, *, #54563, .F. ) ;
#21191=ORIENTED_EDGE ( 'NONE', *, *, #77006, .F. ) ;
#21194=CARTESIAN_POINT ( 'NONE',  ( 83.72465858224470026, 48.53636785707922030, 12.63852326360208522 ) ) ;
#21196=CARTESIAN_POINT ( 'NONE',  ( 69.47943944392696380, 63.02522356655473601, -13.62731951106632344 ) ) ;
#21204=CARTESIAN_POINT ( 'NONE',  ( 72.03850700256526807, 72.31288868693221161, 3.399215934587860755 ) ) ;
#21207=CARTESIAN_POINT ( 'NONE',  ( 69.20277302375480133, 70.19697236206943103, -3.254991052223795034 ) ) ;
#21212=CARTESIAN_POINT ( 'NONE',  ( 66.62667948677777474, 67.60859431869941716, 6.219768998119001857 ) ) ;
#21215=CARTESIAN_POINT ( 'NONE',  ( 66.60565428985405845, 69.00412068662672027, 1.122078433852597756 ) ) ;
#21219=CARTESIAN_POINT ( 'NONE',  ( 74.14312167556930433, 66.30466486950707861, 1.224646799147354045E-15 ) ) ;
#21222=CARTESIAN_POINT ( 'NONE',  ( 72.15865790475056940, 72.27389710013802926, 3.820985825366556288 ) ) ;
#21225=CARTESIAN_POINT ( 'NONE',  ( 44.94038342867872871, 31.11029122506298705, -8.090169943749478065 ) ) ;
#21227=CARTESIAN_POINT ( 'NONE',  ( 71.95941895756688211, 72.18221666786446633, -1.667998158078391580 ) ) ;
#21229=CARTESIAN_POINT ( 'NONE',  ( 18.97660828663255117, 29.14336893147755703, 7.433330006724141015 ) ) ;
#21232=CARTESIAN_POINT ( 'NONE',  ( 10.86724236217879458, 11.98920272979924206, 7.433330006724137462 ) ) ;
#21236=CARTESIAN_POINT ( 'NONE',  ( 82.28994638316029864, 40.89106665807588570, -1.238503865524188230 ) ) ;
#21237=CARTESIAN_POINT ( 'NONE',  ( 72.95907369655466823, 67.57205448826327654, -11.22974281285723386 ) ) ;
#21241=CARTESIAN_POINT ( 'NONE',  ( 73.65303845931325100, 57.26316287700933572, -15.95429008473792010 ) ) ;
#21245=ORIENTED_EDGE ( 'NONE', *, *, #41876, .T. ) ;
#21253=CARTESIAN_POINT ( 'NONE',  ( 79.16585775594589336, 45.99645177219947811, -13.18380221157910981 ) ) ;
#21259=CARTESIAN_POINT ( 'NONE',  ( 25.05680157815287146, 15.26216523072494979, -2.296566073217252530E-15 ) ) ;
#21260=CARTESIAN_POINT ( 'NONE',  ( 25.04820903906726670, 30.16454794089042579, -10.00000000000000355 ) ) ;
#21264=EDGE_CURVE ( 'NONE', #55501, #21644, #36268, .T. ) ;
#21266=CARTESIAN_POINT ( 'NONE',  ( 75.98104421109889017, 51.53574906954564483, 16.18761828508177203 ) ) ;
#21274=CARTESIAN_POINT ( 'NONE',  ( 66.29246560487287354, 68.68673832763016662, -2.132538888833254376 ) ) ;
#21276=CARTESIAN_POINT ( 'NONE',  ( 74.14312167556930433, 66.30466486950707861, 1.224646799147354045E-15 ) ) ;
#21283=DIRECTION ( 'NONE',  ( -0.8660254037844379305, -0.5000000000000014433, -0.000000000000000000 ) ) ;
#21295=CARTESIAN_POINT ( 'NONE',  ( 81.89485588203808675, 55.22971306509116829, 16.24120679747550966 ) ) ;
#21297=CARTESIAN_POINT ( 'NONE',  ( 71.88442714016632351, 67.86911030617876861, 10.31212540994018845 ) ) ;
#21298=EDGE_LOOP ( 'NONE', ( #16374, #25520 ) ) ;
#21301=CARTESIAN_POINT ( 'NONE',  ( 66.07615688706256662, 68.56483294533278183, -4.482668677586966410 ) ) ;
#21303=CARTESIAN_POINT ( 'NONE',  ( 76.11324214256561049, 51.53514024512487168, -16.17221011286880739 ) ) ;
#21311=CARTESIAN_POINT ( 'NONE',  ( 85.64695507815616793, 43.83368588307220648, 5.542843691885481761 ) ) ;
#21312=CARTESIAN_POINT ( 'NONE',  ( 87.86620516538259551, 44.01520320156028987, -1.811253330505868453 ) ) ;
#21313=CARTESIAN_POINT ( 'NONE',  ( 73.03643456002411938, 70.76102034836752352, 7.524419617173737862 ) ) ;
#21317=CARTESIAN_POINT ( 'NONE',  ( 76.05868104838350519, 52.63099806928217106, 15.90100861162440893 ) ) ;
#21327=CARTESIAN_POINT ( 'NONE',  ( 29.42770338693789967, 22.15404122711134960, 8.090169943749479842 ) ) ;
#21330=CARTESIAN_POINT ( 'NONE',  ( 68.99620552988632483, 69.28359185914359841, -6.825668283780611745 ) ) ;
#21335=ORIENTED_EDGE ( 'NONE', *, *, #91502, .T. ) ;
#21337=FACE_OUTER_BOUND ( 'NONE', #97961, .T. ) ;
#21338=CARTESIAN_POINT ( 'NONE',  ( 73.01521690615598459, 70.40106399001336968, -8.092693171194275337 ) ) ;
#21343=CARTESIAN_POINT ( 'NONE',  ( 20.86070775165960001, 33.81751292744056769, -6.180339887498951690 ) ) ;
#21344=CARTESIAN_POINT ( 'NONE',  ( 85.68464957279800842, 48.84619230832644377, 12.06853356899262941 ) ) ;
#21346=CARTESIAN_POINT ( 'NONE',  ( 71.85441816053061359, 72.14404838950795806, -3.648524940272755757 ) ) ;
#21347=B_SPLINE_CURVE_WITH_KNOTS ( 'NONE', 3,
 ( #96105, #57546, #69384, #30887, #54160, #85121, #43341, #36736, #12474, #98575, #81897, #51447, #96607, #82415, #97105, #98068, #5360, #66158, #35252, #42831, #27674, #59022, #73271, #36240, #60029, #21078, #49963, #27169, #58540, #73766, #89515, #28644, #19587, #67146, #34748, #44337, #51954, #81401, #20073, #19084, #65650 ),
 .UNSPECIFIED., .F., .F.,
 ( 4, 2, 1, 1, 1, 2, 2, 1, 1, 2, 2, 1, 1, 2, 2, 1, 1, 2, 2, 1, 1, 1, 2, 2, 1, 1, 1, 4 ),
 ( 0.1734847945017928272, 0.1799419445447479615, 0.1863990945877031236, 0.1993133946736117823, 0.2251419948454298492, 0.2767991951890666491, 0.2897134952749769732, 0.3026277953608873528, 0.3284563955327087226, 0.3801135958763515732, 0.3930278959622621193, 0.4059421960481726099, 0.4317707962199937577, 0.4834279965636352205, 0.4963422966495451005, 0.5092565967354549805, 0.5350851969072738523, 0.5867423972509125951, 0.5996566973368238074, 0.6125709974227346866, 0.6383995975945537804, 0.6900567979381901917, 0.7933711986254616821, 0.8062854987113712291, 0.8191997987972807760, 0.8450283989690978714, 0.8966855993127316182, 1.000000000000000000 ),
 .UNSPECIFIED. ) ;
#21356=LINE ( 'NONE', #52241, #11892 ) ;
#21360=CARTESIAN_POINT ( 'NONE',  ( 78.81389999504742150, 60.06372782575282798, 16.11061031492772955 ) ) ;
#21361=CARTESIAN_POINT ( 'NONE',  ( 41.95273645663377238, 27.14754757982093381, -5.678558825948276656 ) ) ;
#21367=CARTESIAN_POINT ( 'NONE',  ( 12.32504541118064978, 22.51421378149917985, -9.188101187500004485 ) ) ;
#21370=CARTESIAN_POINT ( 'NONE',  ( 71.40044295081541748, 59.41588353585593296, 15.20283060994831104 ) ) ;
#21374=CARTESIAN_POINT ( 'NONE',  ( 3.501222095392049205, 22.99752408145589300, 5.678558825948276656 ) ) ;
#21375=CARTESIAN_POINT ( 'NONE',  ( 81.16104098974128078, 42.41662614947843934, 7.661191396672336396 ) ) ;
#21376=CARTESIAN_POINT ( 'NONE',  ( 35.87562414229657293, 44.21091486745863364, 7.012934429366973338E-14 ) ) ;
#21377=VERTEX_POINT ( 'NONE', #29772 ) ;
#21378=CARTESIAN_POINT ( 'NONE',  ( 81.30818518503046732, 58.89441083166271085, 0.000000000000000000 ) ) ;
#21380=CARTESIAN_POINT ( 'NONE',  ( 76.51987890029035100, 63.61070592637643983, 14.91914813192731337 ) ) ;
#21383=ORIENTED_EDGE ( 'NONE', *, *, #44773, .T. ) ;
#21388=CARTESIAN_POINT ( 'NONE',  ( 88.19122672570537702, 43.84786592109882264, -2.112715317146043770 ) ) ;
#21389=CARTESIAN_POINT ( 'NONE',  ( 31.74858474661088081, 18.73415679381823651, -6.890680421881970419E-14 ) ) ;
#21390=CARTESIAN_POINT ( 'NONE',  ( 80.68870194293324971, 57.51412305112832968, 16.58365939551020318 ) ) ;
#21393=CARTESIAN_POINT ( 'NONE',  ( 87.64894667038031173, 45.18322468047552576, -6.184650709489425857 ) ) ;
#21411=CARTESIAN_POINT ( 'NONE',  ( 73.58067652191090247, 69.78534542737938295, 9.362363942011365125 ) ) ;
#21413=CARTESIAN_POINT ( 'NONE',  ( 82.66218641157266234, 53.85062555766314318, 15.82228755104996765 ) ) ;
#21414=CARTESIAN_POINT ( 'NONE',  ( 10.49025449741314375, 29.55466486950698624, -1.111400068045478839E-16 ) ) ;
#21418=ORIENTED_EDGE ( 'NONE', *, *, #78036, .F. ) ;
#21419=CARTESIAN_POINT ( 'NONE',  ( 73.16723296629628237, 58.29704776030416014, -15.75092464132356262 ) ) ;
#21420=CARTESIAN_POINT ( 'NONE',  ( 39.65533143765975410, 23.86426979415092475, -3.090169943749474069 ) ) ;
#21427=CARTESIAN_POINT ( 'NONE',  ( 75.54132550460440143, 54.37554586383003397, -16.11515908931868779 ) ) ;
#21429=CARTESIAN_POINT ( 'NONE',  ( 79.11618919729676236, 45.91829409069699608, 13.15082663536679242 ) ) ;
#21432=ORIENTED_EDGE ( 'NONE', *, *, #64048, .F. ) ;
#21446=ORIENTED_EDGE ( 'NONE', *, *, #69625, .T. ) ;
#21451=CARTESIAN_POINT ( 'NONE',  ( 81.92950609163860065, 41.13482008182690208, -5.440008311034252309 ) ) ;
#21462=CARTESIAN_POINT ( 'NONE',  ( 3.297978757390601423, 24.83705186507751606, 3.090169943749475401 ) ) ;
#21464=CARTESIAN_POINT ( 'NONE',  ( 71.68777414727941277, 59.55670923871284828, -15.71026032022712293 ) ) ;
#21465=CARTESIAN_POINT ( 'NONE',  ( 73.15617415350918407, 69.83382733437846923, 9.602067989434942774 ) ) ;
#21469=CARTESIAN_POINT ( 'NONE',  ( 72.94218364219292994, 57.09986443339001028, 16.39775231352756180 ) ) ;
#21471=CARTESIAN_POINT ( 'NONE',  ( 68.79257260696145693, 67.61008945445695417, 8.397044590744407344 ) ) ;
#21479=CARTESIAN_POINT ( 'NONE',  ( 23.73493010604062192, 29.10171378149919974, 9.188101187500008038 ) ) ;
#21483=CARTESIAN_POINT ( 'NONE',  ( 88.16334560026523093, 43.89615744693332999, 2.509484348711651602 ) ) ;
#21484=CARTESIAN_POINT ( 'NONE',  ( 74.84209865657220462, 67.13651163270155564, 12.97079428878455332 ) ) ;
#21485=CARTESIAN_POINT ( 'NONE',  ( 69.01345705981862011, 64.44777229250053097, 12.47991269069003906 ) ) ;
#21486=ORIENTED_EDGE ( 'NONE', *, *, #8669, .T. ) ;
#21489=CARTESIAN_POINT ( 'NONE',  ( 73.55377261143068779, 66.54097169440498760, -12.86805831085992047 ) ) ;
#21494=CARTESIAN_POINT ( 'NONE',  ( 69.76251527479838899, 68.37414511987412880, 8.108736765182461781 ) ) ;
#21497=CARTESIAN_POINT ( 'NONE',  ( 6.965316927136144365, 15.97253583063839066, -9.188101187500006262 ) ) ;
#21508=CARTESIAN_POINT ( 'NONE',  ( 16.41743859968233110, 9.288480858562301989, 1.475505719884397138E-15 ) ) ;
#21509=CARTESIAN_POINT ( 'NONE',  ( 84.37825102736907468, 49.99960613749294680, 13.80049582259581520 ) ) ;
#21513=CARTESIAN_POINT ( 'NONE',  ( 79.67773314991492839, 45.75892492389007771, -12.20866718477218704 ) ) ;
#21517=VECTOR ( 'NONE', #98007, 1000.000000000000227 ) ;
#21519=CARTESIAN_POINT ( 'NONE',  ( 88.09383187283991390, 43.67022580382143815, 1.148899272762605506 ) ) ;
#21525=CARTESIAN_POINT ( 'NONE',  ( 81.55438844336480031, 42.25231255016616672, -8.032075583313584843 ) ) ;
#21531=CARTESIAN_POINT ( 'NONE',  ( 81.54502813046227061, 50.64722393506180254, 14.48977360135641135 ) ) ;
#21532=ORIENTED_EDGE ( 'NONE', *, *, #49682, .T. ) ;
#21536=CARTESIAN_POINT ( 'NONE',  ( 82.61071101779671721, 40.83617390237688483, 3.229293852844629331 ) ) ;
#21539=CARTESIAN_POINT ( 'NONE',  ( 68.35468836908422929, 68.36852720251083326, -6.749963640543104049 ) ) ;
#21543=CARTESIAN_POINT ( 'NONE',  ( 14.05709621874952475, 23.51421378149918340, -9.188101187500004485 ) ) ;
#21552=CARTESIAN_POINT ( 'NONE',  ( 40.40883878445526278, 23.73415679381825782, -6.890680421881970419E-14 ) ) ;
#21554=EDGE_CURVE ( 'NONE', #36835, #50903, #86530, .T. ) ;
#21559=CARTESIAN_POINT ( 'NONE',  ( 73.60577444524625434, 62.71670610283283764, -14.51900996758597984 ) ) ;
#21561=ADVANCED_FACE ( 'NONE', ( #8967 ), #866, .T. ) ;
#21566=CARTESIAN_POINT ( 'NONE',  ( 84.67899269911676186, 44.63087609091873986, -8.050483238754811310 ) ) ;
#21569=CARTESIAN_POINT ( 'NONE',  ( 28.91364825607195144, 28.64441083166262203, -10.00000000000000533 ) ) ;
#21576=CARTESIAN_POINT ( 'NONE',  ( 84.75464104472338533, 42.20820103110227706, 0.3493146913119697938 ) ) ;
#21578=CARTESIAN_POINT ( 'NONE',  ( 84.60705283987604730, 47.25696623766521753, 11.22058669928208552 ) ) ;
#21584=CARTESIAN_POINT ( 'NONE',  ( 78.68333733368046978, 54.46560497474366258, 15.97876508924327510 ) ) ;
#21586=B_SPLINE_CURVE_WITH_KNOTS ( 'NONE', 3,
 ( #22944, #70547, #78167, #9776, #40638, #87828, #33050, #32037, #62949, #33562 ),
 .UNSPECIFIED., .F., .F.,
 ( 4, 2, 2, 2, 4 ),
 ( 8.673617379884035472E-19, 0.0002622400424272934051, 0.0005244800848545859429, 0.0007867201272818784806, 0.001048960169709171018 ),
 .UNSPECIFIED. ) ;
#21588=CARTESIAN_POINT ( 'NONE',  ( 82.39043419086114284, 52.72955616827477598, -15.12536216578337012 ) ) ;
#21593=CARTESIAN_POINT ( 'NONE',  ( 84.78687102586546587, 50.23207448519301721, 13.79854428445948678 ) ) ;
#21612=CARTESIAN_POINT ( 'NONE',  ( 42.32740281844729680, 26.29860640527295601, -2.839279412974138328 ) ) ;
#21614=FACE_BOUND ( 'NONE', #40100, .T. ) ;
#21616=CARTESIAN_POINT ( 'NONE',  ( 23.04210978301307122, 28.70171378149919406, -9.188101187500004485 ) ) ;
#21621=CARTESIAN_POINT ( 'NONE',  ( 70.45587595328763086, 60.93839127955427415, 14.43819332404346767 ) ) ;
#21627=CARTESIAN_POINT ( 'NONE',  ( 70.59845676101609513, 64.76082698965105067, 12.92001219729134398 ) ) ;
#21630=CARTESIAN_POINT ( 'NONE',  ( 86.67248974990208410, 44.58726045995240383, 6.056568617757574380 ) ) ;
#21634=CARTESIAN_POINT ( 'NONE',  ( 86.42135960654645999, 47.53165121735794685, -10.51235075660278362 ) ) ;
#21635=CARTESIAN_POINT ( 'NONE',  ( 10.11087252192314345, 14.03677371833799725, 10.00000000000000533 ) ) ;
#21639=CARTESIAN_POINT ( 'NONE',  ( 40.50696180670117741, 29.10170272979929962, -7.433330006724141015 ) ) ;
#21640=DIRECTION ( 'NONE',  ( 0.9646071681523453734, -0.2636911283094539593, 0.000000000000000000 ) ) ;
#21641=DIRECTION ( 'NONE',  ( 0.8660254037844341557, 0.5000000000000082157, -0.000000000000000000 ) ) ;
#21644=VERTEX_POINT ( 'NONE', #50460 ) ;
#21653=CARTESIAN_POINT ( 'NONE',  ( 78.12619150794976974, 59.56496585069915284, -16.10012152594639900 ) ) ;
#21656=CARTESIAN_POINT ( 'NONE',  ( 77.26689473168350730, 63.03694197878571970, -15.27008446967128386 ) ) ;
#21663=CARTESIAN_POINT ( 'NONE',  ( 33.49697393745356777, 27.84335787977765264, 9.188101187500006262 ) ) ;
#21667=CARTESIAN_POINT ( 'NONE',  ( 74.02653709664873816, 68.32631449583556105, -11.67658431812981412 ) ) ;
#21672=VERTEX_POINT ( 'NONE', #34758 ) ;
#21676=ORIENTED_EDGE ( 'NONE', *, *, #30161, .T. ) ;
#21678=FACE_OUTER_BOUND ( 'NONE', #30663, .T. ) ;
#21681=CARTESIAN_POINT ( 'NONE',  ( 83.46892329719068471, 47.64461127584740296, 12.06929726775783962 ) ) ;
#21686=CARTESIAN_POINT ( 'NONE',  ( 66.60661563016273590, 67.77273566365288104, -7.043189648870076702 ) ) ;
#21687=CARTESIAN_POINT ( 'NONE',  ( 82.39461015293801438, 51.35258621359815834, 14.58598051198313783 ) ) ;
#21688=CARTESIAN_POINT ( 'NONE',  ( 82.19476570567245233, 41.21667155281596706, -3.467692515155950339 ) ) ;
#21691=CARTESIAN_POINT ( 'NONE',  ( 72.15692581984221476, 72.29159277512509618, 3.751890296296631178 ) ) ;
#21695=CARTESIAN_POINT ( 'NONE',  ( 82.74681249865726329, 53.90498867430740404, -15.82393922498146566 ) ) ;
#21701=CARTESIAN_POINT ( 'NONE',  ( 67.29078699571681454, 69.45351283087119043, 0.2276663097563886018 ) ) ;
#21704=CARTESIAN_POINT ( 'NONE',  ( 43.80372508975956691, 30.45404122711137163, -8.090169943749478065 ) ) ;
#21706=CARTESIAN_POINT ( 'NONE',  ( 82.62625517957130228, 54.11794360844533003, 15.53797790719450056 ) ) ;
#21707=CARTESIAN_POINT ( 'NONE',  ( 72.17098681862357523, 72.08342691454184603, 2.975191886509651162 ) ) ;
#21714=CARTESIAN_POINT ( 'NONE',  ( 71.86515158781777757, 72.12545754810727772, -1.692783104835278607 ) ) ;
#21716=CARTESIAN_POINT ( 'NONE',  ( 25.24326406500046360, 20.28920272979927475, -7.433330006724141015 ) ) ;
#21719=CARTESIAN_POINT ( 'NONE',  ( 12.88253908977640094, 9.298606405272902720, -2.839279412974138328 ) ) ;
#21724=CARTESIAN_POINT ( 'NONE',  ( 73.57124375542366579, 65.07890931487162334, 13.30975167017917471 ) ) ;
#21728=CARTESIAN_POINT ( 'NONE',  ( 87.79103035407327127, 45.19801466894013942, -6.906962003849810294 ) ) ;
#21747=CARTESIAN_POINT ( 'NONE',  ( 22.06543860749898656, 21.24335787977763346, -9.188101187500008038 ) ) ;
#21748=CARTESIAN_POINT ( 'NONE',  ( 70.27050606688109724, 70.17526897919434248, -5.379368406286444859 ) ) ;
#21759=DIRECTION ( 'NONE',  ( 0.1378186779084994706, -0.2387089523694924387, -0.9612616959383186721 ) ) ;
#21767=EDGE_CURVE ( 'NONE', #57975, #86867, #41252, .T. ) ;
#21773=CARTESIAN_POINT ( 'NONE',  ( 66.97041650028039328, 68.04972680430266507, 6.918031611078456322 ) ) ;
#21776=( BOUNDED_CURVE ( )  B_SPLINE_CURVE ( 2, ( #79722, #72092, #19885, #87363, #57862, #2693, #11792, #17892, #95440, #42648, #64982, #73580, #27485 ),
 .UNSPECIFIED., .F., .T. ) 
 B_SPLINE_CURVE_WITH_KNOTS ( ( 3, 2, 2, 2, 2, 2, 3 ),
 ( 0.8875000000000000666, 0.8900000000000000133, 0.8950000000000000178, 0.9000000000000000222, 0.9050000000000000266, 0.9100000000000000311, 0.9125000000000000888 ),
 .UNSPECIFIED. ) 
 CURVE ( )  GEOMETRIC_REPRESENTATION_ITEM ( )  RATIONAL_B_SPLINE_CURVE ( ( 0.9755282581475767101, 0.9755282581475772652, 1.000000000000000000, 0.9510565162951535312, 1.000000000000000000, 0.9510565162951535312, 1.000000000000000000, 0.9510565162951535312, 1.000000000000000000, 0.9510565162951535312, 1.000000000000000000, 0.9755282581475761550, 0.9755282581475767101 ) ) 
 REPRESENTATION_ITEM ( '' )  );
#21777=CARTESIAN_POINT ( 'NONE',  ( 81.26140763373125253, 56.17807541021651474, 16.09937115873037072 ) ) ;
#21779=CARTESIAN_POINT ( 'NONE',  ( 70.09004903573875822, 62.97794529296450605, 13.29049216610558126 ) ) ;
#21793=DIRECTION ( 'NONE',  ( -0.4972609476841356457, 0.8612812260087758798, 0.1045284632676436315 ) ) ;
#21798=CARTESIAN_POINT ( 'NONE',  ( 81.24342585074298029, 44.30867135165726722, -10.09829603353806071 ) ) ;
#21799=CARTESIAN_POINT ( 'NONE',  ( 79.49951204047911801, 46.37032438487753438, 12.70281872619212926 ) ) ;
#21800=CARTESIAN_POINT ( 'NONE',  ( 88.10271290040205372, 43.80081590334129515, -2.139902876137079080 ) ) ;
#21801=CARTESIAN_POINT ( 'NONE',  ( 79.43566581485079325, 59.14155571097092690, -16.22735706158325542 ) ) ;
#21802=CARTESIAN_POINT ( 'NONE',  ( 70.96263597670173340, 67.29475622062147977, -10.35096767034863774 ) ) ;
#21803=ORIENTED_EDGE ( 'NONE', *, *, #50506, .F. ) ;
#21804=CARTESIAN_POINT ( 'NONE',  ( 76.44905381598371719, 54.38756756234472789, 16.09189434050703582 ) ) ;
#21808=CARTESIAN_POINT ( 'NONE',  ( 80.53565967596219366, 49.57456898333717277, 14.21858742687847688 ) ) ;
#21817=EDGE_CURVE ( 'NONE', #80050, #5537, #33893, .T. ) ;
#21818=CARTESIAN_POINT ( 'NONE',  ( 17.74977768659132593, 33.18080186712593616, 3.090169943749475401 ) ) ;
#21819=CARTESIAN_POINT ( 'NONE',  ( 68.34576586436469370, 65.68917945663493185, -10.35820680181607401 ) ) ;
#21821=CARTESIAN_POINT ( 'NONE',  ( 26.22111236500157361, 16.10801979619929369, 3.090169943749476733 ) ) ;
#21823=CARTESIAN_POINT ( 'NONE',  ( 72.29127226384117932, 72.04750469537891888, -3.387169285285207554 ) ) ;
#21828=CARTESIAN_POINT ( 'NONE',  ( 66.76615945880296010, 67.52988098192712130, -6.530483747860452937 ) ) ;
#21834=CARTESIAN_POINT ( 'NONE',  ( 27.10026011071931151, 20.81029122506295437, 8.090169943749479842 ) ) ;
#21835=CARTESIAN_POINT ( 'NONE',  ( 85.70209702422732789, 48.64685655562228561, 12.37813881961889528 ) ) ;
#21837=CARTESIAN_POINT ( 'NONE',  ( 71.90245059369782155, 72.17364547496468674, -3.641340926847324244 ) ) ;
#21845=PLANE ( 'NONE',  #49056 ) ;
#21850=CARTESIAN_POINT ( 'NONE',  ( 34.65648599653719231, 40.98502408145595410, -5.678558825948271327 ) ) ;
#21857=CARTESIAN_POINT ( 'NONE',  ( 9.881553883097156543, 27.74646525600388713, 2.839279412974139660 ) ) ;
#21859=CARTESIAN_POINT ( 'NONE',  ( 71.49559693922878978, 59.13754170620860862, 15.29921231604372878 ) ) ;
#21862=CARTESIAN_POINT ( 'NONE',  ( 86.63427790160775999, 45.49709482439454433, -7.739417912740459649 ) ) ;
#21864=CARTESIAN_POINT ( 'NONE',  ( 81.85012752262665003, 42.15354315940976448, 7.594371692912019967 ) ) ;
#21865=ORIENTED_EDGE ( 'NONE', *, *, #25882, .F. ) ;
#21867=CARTESIAN_POINT ( 'NONE',  ( 68.11960572793796587, 69.93251101871156550, 0.1879669648890121281 ) ) ;
#21875=CARTESIAN_POINT ( 'NONE',  ( 70.79475271764948729, 66.96855654029467075, 11.21893109225559648 ) ) ;
#21876=CARTESIAN_POINT ( 'NONE',  ( 80.47095457055254997, 57.75622231085855418, 16.59751886879109506 ) ) ;
#21877=CARTESIAN_POINT ( 'NONE',  ( 72.32955901973197399, 69.72760921849626925, -9.141978898838837964 ) ) ;
#21879=DIRECTION ( 'NONE',  ( 0.5000000000000013323, -0.8660254037844378194, 0.000000000000000000 ) ) ;
#21880=AXIS2_PLACEMENT_3D ( 'NONE', #8724, #31506, #85266 ) ;
#21885=ORIENTED_EDGE ( 'NONE', *, *, #57447, .T. ) ;
#21894=EDGE_LOOP ( 'NONE', ( #62764, #37456, #40683, #33864 ) ) ;
#21896=CARTESIAN_POINT ( 'NONE',  ( 79.69350452701492316, 51.55546628257836517, -15.65634712508320803 ) ) ;
#21897=CARTESIAN_POINT ( 'NONE',  ( 73.43762515466688967, 73.52662068827324049, 2.033788753608857291E-15 ) ) ;
#21904=CARTESIAN_POINT ( 'NONE',  ( 75.80790870016019767, 57.44398695910171426, -16.10616469783059301 ) ) ;
#21905=CARTESIAN_POINT ( 'NONE',  ( 71.34475373241517104, 70.22794211031242639, 6.670480703838566505 ) ) ;
#21908=FACE_OUTER_BOUND ( 'NONE', #67035, .T. ) ;
#21910=CARTESIAN_POINT ( 'NONE',  ( 78.74568341211313793, 47.64299656527150262, 14.28912099471933850 ) ) ;
#21914=CARTESIAN_POINT ( 'NONE',  ( 77.34456863197527809, 53.78998963892438212, -15.98317469749341591 ) ) ;
#21917=CARTESIAN_POINT ( 'NONE',  ( 79.35938606471496826, 46.19917012563481507, 12.64008113691103752 ) ) ;
#21925=CARTESIAN_POINT ( 'NONE',  ( 72.09435550024913653, 71.41332343156211948, 5.094207931309262527 ) ) ;
#21933=LINE ( 'NONE', #6743, #30085 ) ;
#21934=EDGE_CURVE ( 'NONE', #35455, #23265, #91847, .T. ) ;
#21938=EDGE_CURVE ( 'NONE', #65006, #86000, #14484, .T. ) ;
#21941=CARTESIAN_POINT ( 'NONE',  ( 81.78504375891562006, 41.48292696562021575, -5.073134180756075473 ) ) ;
#21947=CARTESIAN_POINT ( 'NONE',  ( 78.94155721643031143, 59.44305089757029492, -16.52414004995256036 ) ) ;
#21951=AXIS2_PLACEMENT_3D ( 'NONE', #66789, #96742, #97715 ) ;
#21954=CARTESIAN_POINT ( 'NONE',  ( 68.24462126014344676, 68.81508646265615425, -6.863557568287563804 ) ) ;
#21956=CARTESIAN_POINT ( 'NONE',  ( 71.77078610818966808, 59.27153383271750897, -15.30389425934728642 ) ) ;
#21957=CARTESIAN_POINT ( 'NONE',  ( 73.26476404075305027, 69.81404936883070889, 9.109525140469814986 ) ) ;
#21962=CARTESIAN_POINT ( 'NONE',  ( 73.76061769417498226, 55.25278673652109518, 16.11964219720597669 ) ) ;
#21964=CARTESIAN_POINT ( 'NONE',  ( 66.09818052648262210, 68.58602539020668587, -4.455928803003319061 ) ) ;
#21970=CARTESIAN_POINT ( 'NONE',  ( 19.41443888993109823, 32.18502408145592852, 5.678558825948277544 ) ) ;
#21972=CARTESIAN_POINT ( 'NONE',  ( 83.48909022670937929, 51.62989903239390088, -14.87641496889664694 ) ) ;
#21974=CARTESIAN_POINT ( 'NONE',  ( 69.98840988044214839, 70.01348391617253242, 6.516657591370888625 ) ) ;
#21975=CARTESIAN_POINT ( 'NONE',  ( 74.65263117529048031, 66.98225998262294922, 13.00178404275292543 ) ) ;
#21978=CARTESIAN_POINT ( 'NONE',  ( 73.27328646083023500, 70.16270934360544231, -9.274526489422585840 ) ) ;
#21994=CARTESIAN_POINT ( 'NONE',  ( 18.70427805463205573, 12.92755873383625520, 6.180339887498953466 ) ) ;
#21996=ORIENTED_EDGE ( 'NONE', *, *, #70149, .T. ) ;
#21999=CARTESIAN_POINT ( 'NONE',  ( 82.72443436000141048, 45.32069663430784345, -10.30851497045541088 ) ) ;
#22005=CARTESIAN_POINT ( 'NONE',  ( 21.40066741106990378, 12.75978393459163840, -1.583844403245362020 ) ) ;
#22009=CARTESIAN_POINT ( 'NONE',  ( 82.06353261700769508, 41.00057011406286733, -2.892018250819532454 ) ) ;
#22011=CARTESIAN_POINT ( 'NONE',  ( 81.35301008429968306, 42.53188570201726293, -7.664210345353390075 ) ) ;
#22012=EDGE_LOOP ( 'NONE', ( #56943, #54006, #55145, #65409 ) ) ;
#22017=CARTESIAN_POINT ( 'NONE',  ( 71.63453813518020752, 72.07236434383467838, 0.7172108931481352423 ) ) ;
#22019=FACE_OUTER_BOUND ( 'NONE', #57255, .T. ) ;
#22022=ADVANCED_FACE ( 'NONE', ( #92736 ), #23290, .T. ) ;
#22023=CARTESIAN_POINT ( 'NONE',  ( 82.75425455800102270, 53.83811729049745054, -15.80404254388376906 ) ) ;
#22025=CARTESIAN_POINT ( 'NONE',  ( 76.15254952159935442, 56.95550950617717945, 16.13614341295277654 ) ) ;
#22026=CARTESIAN_POINT ( 'NONE',  ( 11.81506597172265316, 27.79752408145591502, -5.678558825948271327 ) ) ;
#22028=CARTESIAN_POINT ( 'NONE',  ( 85.64302380165412387, 48.93088599686250006, 12.15651094663528653 ) ) ;
#22037=CARTESIAN_POINT ( 'NONE',  ( 77.38507280294756185, 49.73636053508898414, -15.49715387554307355 ) ) ;
#22047=CARTESIAN_POINT ( 'NONE',  ( 82.72380189249818727, 53.29157908679620448, -15.28871581714063588 ) ) ;
#22050=CARTESIAN_POINT ( 'NONE',  ( 72.13188387548123615, 72.33286681718249156, 1.023135554637200961 ) ) ;
#22051=CARTESIAN_POINT ( 'NONE',  ( 72.76085654771455324, 70.95487523876634839, 7.692118034595658571 ) ) ;
#22053=CARTESIAN_POINT ( 'NONE',  ( 87.78081971166569986, 44.10618430004835488, 2.676874261813569245 ) ) ;
#22055=VERTEX_POINT ( 'NONE', #62281 ) ;
#22060=B_SPLINE_CURVE_WITH_KNOTS ( 'NONE', 3,
 ( #37679, #69087, #62992, #31575, #70586, #7798, #16391, #38683, #47282, #1200, #46268, #15883, #78207, #55370, #24491, #93433, #54884, #39165, #196, #77191, #100013, #14407, #30598, #61484 ),
 .UNSPECIFIED., .F., .F.,
 ( 4, 2, 2, 2, 2, 2, 2, 2, 2, 2, 2, 4 ),
 ( 0.000000000000000000, 0.1250000000000018596, 0.2500000000000037192, 0.3750000000000055511, 0.4375000000000049405, 0.5000000000000043299, 0.5625000000000036637, 0.6250000000000031086, 0.6875000000000024425, 0.7500000000000017764, 0.8750000000000008882, 1.000000000000000000 ),
 .UNSPECIFIED. ) ;
#22066=CARTESIAN_POINT ( 'NONE',  ( 70.97982842658589675, 70.74070771080400277, 6.159771955551562428 ) ) ;
#22068=B_SPLINE_CURVE_WITH_KNOTS ( 'NONE', 3,
 ( #87940, #56463, #72703, #9890, #25061, #94505, #33682, #3296, #96017, #56954, #2290, #33167, #2799, #63564, #95015, #40748, #32665, #18484, #64071, #17466, #64578, #57454, #3779, #25577, #88433, #42741, #95532, #49369, #73187, #80313, #81314, #10881, #65067, #87454, #41758, #55937, #71693, #86936, #34175, #48880, #17987, #26579, #48376, #18993, #79322, #49865 ),
 .UNSPECIFIED., .F., .F.,
 ( 4, 1, 1, 1, 2, 2, 1, 1, 1, 2, 2, 1, 1, 2, 2, 1, 1, 2, 2, 1, 1, 2, 2, 1, 2, 2, 1, 2, 2, 4 ),
 ( 0.000000000000000000, 0.06249999999999646116, 0.09374999999999453215, 0.1093749999999932415, 0.1171874999999931027, 0.1249999999999929778, 0.1874999999999940326, 0.2187499999999960587, 0.2343749999999957256, 0.2421874999999963363, 0.2499999999999969469, 0.3124999999999927280, 0.3437499999999900635, 0.3593749999999887312, 0.3749999999999873990, 0.4374999999999868994, 0.4687499999999858447, 0.4843749999999845679, 0.4999999999999832356, 0.5624999999999802380, 0.5937499999999784617, 0.6093749999999783507, 0.6249999999999782396, 0.6874999999999817923, 0.7187499999999836797, 0.7499999999999855671, 0.8124999999999887867, 0.8437499999999908962, 0.8749999999999930056, 1.000000000000000000 ),
 .UNSPECIFIED. ) ;
#22069=EDGE_CURVE ( 'NONE', #57260, #42456, #50712, .T. ) ;
#22073=LINE ( 'NONE', #68166, #96515 ) ;
#22076=DIRECTION ( 'NONE',  ( -0.3940053768033626169, 0.6824373310787468228, 0.6156614753256509642 ) ) ;
#22077=CARTESIAN_POINT ( 'NONE',  ( 80.28770547203146180, 53.50931822275166638, -15.65279642959144901 ) ) ;
#22081=ADVANCED_FACE ( 'NONE', ( #48096 ), #2521, .T. ) ;
#22084=CARTESIAN_POINT ( 'NONE',  ( 68.07050364499654904, 67.45021790136736684, 7.977111741387843402 ) ) ;
#22089=CARTESIAN_POINT ( 'NONE',  ( 11.99789328850488879, 15.43085787977761569, -9.188101187500008038 ) ) ;
#22095=DIRECTION ( 'NONE',  ( -0.8660254037844378194, -0.5000000000000014433, -0.000000000000000000 ) ) ;
#22098=CARTESIAN_POINT ( 'NONE',  ( 35.00289615805098009, 41.18502408145595695, 5.678558825948276656 ) ) ;
#22102=CARTESIAN_POINT ( 'NONE',  ( 32.30976433484754295, 19.44966523072496045, -2.296566073217252530E-15 ) ) ;
#22104=AXIS2_PLACEMENT_3D ( 'NONE', #68748, #29272, #15041 ) ;
#22111=CARTESIAN_POINT ( 'NONE',  ( 70.76739923968082735, 60.93592591164377126, 15.04188609397093757 ) ) ;
#22119=EDGE_LOOP ( 'NONE', ( #80480, #46773, #30457, #21245 ) ) ;
#22120=CARTESIAN_POINT ( 'NONE',  ( 78.31186438638634684, 61.61641173835174357, 16.15355831358047567 ) ) ;
#22121=EDGE_CURVE ( 'NONE', #29087, #7931, #5850, .T. ) ;
#22131=CARTESIAN_POINT ( 'NONE',  ( 32.59967566254915994, 39.79752408145595410, -5.678558825948271327 ) ) ;
#22133=CARTESIAN_POINT ( 'NONE',  ( 81.44589832458051148, 55.42546683620729908, -16.32034488869437538 ) ) ;
#22134=CARTESIAN_POINT ( 'NONE',  ( 75.79717256834328509, 62.26676178855290544, -15.60790356137264823 ) ) ;
#22146=CARTESIAN_POINT ( 'NONE',  ( 72.31909173678994307, 61.61524097631632912, -14.63572028674620817 ) ) ;
#22149=CARTESIAN_POINT ( 'NONE',  ( 76.88818783305237048, 63.31965297372375545, -15.46890590930648912 ) ) ;
#22156=CARTESIAN_POINT ( 'NONE',  ( 39.71190250773520347, 34.87878583063844928, -9.188101187500006262 ) ) ;
#22159=CARTESIAN_POINT ( 'NONE',  ( 86.83317331226271563, 45.77437086576020420, -8.734311406240857778 ) ) ;
#22167=EDGE_CURVE ( 'NONE', #50903, #65006, #31514, .T. ) ;
#22175=CARTESIAN_POINT ( 'NONE',  ( 83.96883838543894285, 49.56557209779730755, 13.24582278230334431 ) ) ;
#22182=CARTESIAN_POINT ( 'NONE',  ( 72.18837429559984287, 65.02575927599113470, 12.81091265492822551 ) ) ;
#22186=CARTESIAN_POINT ( 'NONE',  ( 72.11463582380375215, 72.32045887020245800, 3.546959094384879219 ) ) ;
#22187=CARTESIAN_POINT ( 'NONE',  ( 82.81428708694842555, 42.72530104253821293, 6.546892619254078838 ) ) ;
#22188=CARTESIAN_POINT ( 'NONE',  ( 18.52134341065869805, 22.64441083166260427, -10.00000000000000533 ) ) ;
#22191=CARTESIAN_POINT ( 'NONE',  ( 82.56662147140762897, 53.48431740468424778, -15.73383048919865068 ) ) ;
#22199=CARTESIAN_POINT ( 'NONE',  ( 73.29675513422920119, 69.64584746942686877, -9.922798968680028864 ) ) ;
#22201=CARTESIAN_POINT ( 'NONE',  ( 3.631266576971075910, 20.83478043621385467, -8.090169943749479842 ) ) ;
#22205=CARTESIAN_POINT ( 'NONE',  ( 72.09275328296196506, 72.05865058278648405, 2.889467875048744805 ) ) ;
#22210=CARTESIAN_POINT ( 'NONE',  ( 78.58300731283269158, 51.01195712413127836, -15.19627590126262895 ) ) ;
#22214=CARTESIAN_POINT ( 'NONE',  ( 26.56574046957052460, 17.19860640527293327, 2.839279412974134775 ) ) ;
#22217=CARTESIAN_POINT ( 'NONE',  ( 5.211622267866312441, 23.98502408145590081, -5.678558825948271327 ) ) ;
#22218=CARTESIAN_POINT ( 'NONE',  ( 76.70982964007059479, 63.62857842591434832, 15.32478313419208149 ) ) ;
#22219=CARTESIAN_POINT ( 'NONE',  ( 75.04168434830708634, 54.38814634816782245, 16.60217853031275936 ) ) ;
#22221=CARTESIAN_POINT ( 'NONE',  ( 82.57385212973971989, 41.04541115053230982, -1.138833187496899768 ) ) ;
#22227=ORIENTED_EDGE ( 'NONE', *, *, #95640, .F. ) ;
#22235=FACE_OUTER_BOUND ( 'NONE', #16280, .T. ) ;
#22241=CARTESIAN_POINT ( 'NONE',  ( 24.91850453858129910, 20.10170272979927475, -7.433330006724141015 ) ) ;
#22242=CARTESIAN_POINT ( 'NONE',  ( 75.33346472819354744, 56.39419380256580183, 16.13885548225777811 ) ) ;
#22248=VERTEX_POINT ( 'NONE', #66302 ) ;
#22250=CARTESIAN_POINT ( 'NONE',  ( 83.53571973624073621, 48.86361953640308542, -12.93375367189796243 ) ) ;
#22252=CARTESIAN_POINT ( 'NONE',  ( 72.77465006231518885, 68.95668891863901706, 10.36720942691999525 ) ) ;
#22257=CARTESIAN_POINT ( 'NONE',  ( 78.01627562341427335, 61.04568562798238673, -15.88251659512814662 ) ) ;
#22272=CARTESIAN_POINT ( 'NONE',  ( 66.62431214535784818, 67.55485982655905275, 6.324360224251575069 ) ) ;
#22279=CARTESIAN_POINT ( 'NONE',  ( 87.47635513963552967, 45.03054629282576116, 6.933452704933710464 ) ) ;
#22284=EDGE_CURVE ( 'NONE', #33772, #50515, #26692, .T. ) ;
#22285=ORIENTED_EDGE ( 'NONE', *, *, #174, .F. ) ;
#22286=CARTESIAN_POINT ( 'NONE',  ( 76.15722354489868451, 51.53125197354221854, -15.67564492834882373 ) ) ;
#22295=CARTESIAN_POINT ( 'NONE',  ( 87.78141208182009336, 44.24254441107329683, 4.709165031671994406 ) ) ;
#22296=CARTESIAN_POINT ( 'NONE',  ( 68.96773005203053231, 67.85633357740573501, -9.040919504298567944 ) ) ;
#22297=CARTESIAN_POINT ( 'NONE',  ( 80.01063490705305981, 44.83894994093007824, -11.28620975940164506 ) ) ;
#22299=CARTESIAN_POINT ( 'NONE',  ( 72.70196728203136161, 70.94362825444909504, 7.654249537423025274 ) ) ;
#22310=AXIS2_PLACEMENT_3D ( 'NONE', #45085, #3, #45573 ) ;
#22315=CARTESIAN_POINT ( 'NONE',  ( 24.56267145112387240, 22.38052372038641735, 10.00000000000000533 ) ) ;
#22318=CARTESIAN_POINT ( 'NONE',  ( 73.98570270871887544, 68.92876820612472955, -11.10152750440661862 ) ) ;
#22325=CARTESIAN_POINT ( 'NONE',  ( 66.89157806229785308, 68.17490930942568639, -6.585856375969495247 ) ) ;
#22327=CARTESIAN_POINT ( 'NONE',  ( 73.00222835256424503, 70.74352510380845160, -7.508679084761850753 ) ) ;
#22330=EDGE_CURVE ( 'NONE', #2161, #81326, #99186, .T. ) ;
#22332=CARTESIAN_POINT ( 'NONE',  ( 18.88643602551048417, 33.83705186507754092, 3.090169943749475401 ) ) ;
#22333=CARTESIAN_POINT ( 'NONE',  ( 85.27718046765656368, 42.54128723994562478, -1.177150515647308993 ) ) ;
#22340=EDGE_CURVE ( 'NONE', #40695, #77239, #44790, .T. ) ;
#22346=CARTESIAN_POINT ( 'NONE',  ( 68.59496618099213094, 69.97855879749779717, -4.650311752650147845 ) ) ;
#22348=CARTESIAN_POINT ( 'NONE',  ( 72.59558277096371626, 71.44241063249414481, 5.693108417517408704 ) ) ;
#22349=CARTESIAN_POINT ( 'NONE',  ( 46.16617079539854984, 27.44966523072498177, -2.296566073217252530E-15 ) ) ;
#22352=CYLINDRICAL_SURFACE ( 'NONE', #50762, 16.60714546451156792 ) ;
#22355=CARTESIAN_POINT ( 'NONE',  ( 25.69310950058096310, 17.76004757982090254, 5.678558825948272215 ) ) ;
#22357=CARTESIAN_POINT ( 'NONE',  ( 71.98731340802646628, 59.17192410441948169, 15.86756879471484183 ) ) ;
#22364=( BOUNDED_CURVE ( )  B_SPLINE_CURVE ( 2, ( #19742, #52597, #82070, #50606, #81561, #42993, #35911, #66810, #20734, #90162, #69277, #37864, #44976 ),
 .UNSPECIFIED., .F., .T. ) 
 B_SPLINE_CURVE_WITH_KNOTS ( ( 3, 2, 2, 2, 2, 2, 3 ),
 ( 0.8375000000000000222, 0.8399999999999999689, 0.8449999999999999734, 0.8499999999999999778, 0.8549999999999999822, 0.8599999999999999867, 0.8625000000000000444 ),
 .UNSPECIFIED. ) 
 CURVE ( )  GEOMETRIC_REPRESENTATION_ITEM ( )  RATIONAL_B_SPLINE_CURVE ( ( 0.9755282581475767101, 0.9755282581475772652, 1.000000000000000000, 0.9510565162951535312, 1.000000000000000000, 0.9510565162951535312, 1.000000000000000000, 0.9510565162951535312, 1.000000000000000000, 0.9510565162951535312, 1.000000000000000000, 0.9755282581475761550, 0.9755282581475767101 ) ) 
 REPRESENTATION_ITEM ( '' )  );
#22366=CARTESIAN_POINT ( 'NONE',  ( 69.61553634081849395, 70.72154784002148631, -1.738344088579393043 ) ) ;
#22367=CARTESIAN_POINT ( 'NONE',  ( 20.28716687417668751, 35.21091486745861232, 7.012934429366973338E-14 ) ) ;
#22369=ORIENTED_EDGE ( 'NONE', *, *, #44734, .T. ) ;
#22377=CARTESIAN_POINT ( 'NONE',  ( 79.85415921798438887, 57.97294913568264008, 16.26669915568274050 ) ) ;
#22378=CARTESIAN_POINT ( 'NONE',  ( 70.09637832351664599, 69.82647708718234014, -7.001659778457793415 ) ) ;
#22383=ORIENTED_EDGE ( 'NONE', *, *, #15747, .F. ) ;
#22386=CARTESIAN_POINT ( 'NONE',  ( 74.48947563274340666, 63.15900717418585231, 14.54963554206422849 ) ) ;
#22399=CARTESIAN_POINT ( 'NONE',  ( 73.56791514541508548, 69.79467306600464838, 9.342728403714463781 ) ) ;
#22409=CARTESIAN_POINT ( 'NONE',  ( 70.89288081638191841, 69.42695580627280094, 7.581665190048367364 ) ) ;
#22410=CARTESIAN_POINT ( 'NONE',  ( 68.20887950783240683, 70.50781471800318911, 6.446984873749973067E-06 ) ) ;
#22411=CARTESIAN_POINT ( 'NONE',  ( 66.96856610619528283, 66.96525581452927156, 8.678199790520725543 ) ) ;
#22413=CARTESIAN_POINT ( 'NONE',  ( 78.12712398815010317, 47.68924013269637641, 14.49032448239827886 ) ) ;
#22415=VERTEX_POINT ( 'NONE', #81017 ) ;
#22417=CARTESIAN_POINT ( 'NONE',  ( 71.81875712178876370, 69.15799409778134077, 8.801720388420321228 ) ) ;
#22419=CARTESIAN_POINT ( 'NONE',  ( 79.01901227882056844, 46.16084846667202868, 12.74958081812160948 ) ) ;
#22421=DIRECTION ( 'NONE',  ( 0.5000000000000013323, -0.8660254037844378194, 0.000000000000000000 ) ) ;
#22426=CARTESIAN_POINT ( 'NONE',  ( 72.49874796052694137, 71.64632196231394801, 6.095118657294458231 ) ) ;
#22441=CARTESIAN_POINT ( 'NONE',  ( 81.91113339553959349, 41.29801664419279206, -5.856091804582637117 ) ) ;
#22445=AXIS2_PLACEMENT_3D ( 'NONE', #37611, #84764, #23915 ) ;
#22446=DIRECTION ( 'NONE',  ( 0.6355427771210649945, 0.000000000000000000, -0.7720656568254052887 ) ) ;
#22454=CARTESIAN_POINT ( 'NONE',  ( 69.69180481802852967, 68.87891834069074548, -8.182775995575166661 ) ) ;
#22456=CARTESIAN_POINT ( 'NONE',  ( 71.72224841297412468, 59.56686840634775848, -15.71315591292551872 ) ) ;
#22457=CARTESIAN_POINT ( 'NONE',  ( 73.99515186948657686, 54.97541550358009488, -16.60506967685200763 ) ) ;
#22462=CARTESIAN_POINT ( 'NONE',  ( 73.69000260020860082, 55.31241817090647572, 16.11699230035644703 ) ) ;
#22464=CARTESIAN_POINT ( 'NONE',  ( 66.18199044853756163, 68.66682925730346199, -4.353933929110309187 ) ) ;
#22466=VECTOR ( 'NONE', #62354, 1000.000000000000114 ) ;
#22470=CARTESIAN_POINT ( 'NONE',  ( 28.77833178495667710, 28.56628583063842441, 9.188101187500006262 ) ) ;
#22475=CARTESIAN_POINT ( 'NONE',  ( 70.73695309034920342, 71.03131902187277547, 5.127882233600515427 ) ) ;
#22487=CARTESIAN_POINT ( 'NONE',  ( 71.59874412008122135, 72.43189726433810449, 0.9745913883648592568 ) ) ;
#22492=CARTESIAN_POINT ( 'NONE',  ( 67.90270976675789427, 69.15137710594201792, 4.266361631938849541 ) ) ;
#22495=CARTESIAN_POINT ( 'NONE',  ( 11.78719504716597299, 22.50829794293879260, -10.00000000000000355 ) ) ;
#22496=CARTESIAN_POINT ( 'NONE',  ( 86.72314128514305764, 46.93129043413777168, 10.24845158530357558 ) ) ;
#22499=CARTESIAN_POINT ( 'NONE',  ( 86.51873334781436142, 47.12553361672021879, -10.58414027450332462 ) ) ;
#22500=CARTESIAN_POINT ( 'NONE',  ( 83.71391341011990050, 45.20889584457674459, -9.573811886256185844 ) ) ;
#22503=CARTESIAN_POINT ( 'NONE',  ( 79.09474592215633493, 60.19097512726886379, -16.45688605998255127 ) ) ;
#22505=CARTESIAN_POINT ( 'NONE',  ( 69.91593357268108377, 62.62562713682927296, 13.43404203153625076 ) ) ;
#22506=ORIENTED_EDGE ( 'NONE', *, *, #83301, .T. ) ;
#22510=CARTESIAN_POINT ( 'NONE',  ( 81.81442681794474936, 42.35015792257434697, -7.949573155866509033 ) ) ;
#22512=EDGE_CURVE ( 'NONE', #14298, #55257, #66746, .T. ) ;
#22513=EDGE_LOOP ( 'NONE', ( #15242, #4289, #5943, #1006 ) ) ;
#22515=CARTESIAN_POINT ( 'NONE',  ( 81.03644536932286258, 48.60226841593650704, 13.58935439033044901 ) ) ;
#22527=CARTESIAN_POINT ( 'NONE',  ( 82.78312474470216387, 53.88647634593384339, -15.44496935275225269 ) ) ;
#22530=CARTESIAN_POINT ( 'NONE',  ( 82.44310520575160695, 54.28011738120410001, -15.96781897959229113 ) ) ;
#22531=CARTESIAN_POINT ( 'NONE',  ( 19.31277771287585310, 13.01110640527291551, 2.839279412974134775 ) ) ;
#22542=CARTESIAN_POINT ( 'NONE',  ( 80.47459502809753928, 46.22092247480932770, -12.20579193300740783 ) ) ;
#22547=CARTESIAN_POINT ( 'NONE',  ( 72.44797420414980138, 63.04533137475104354, -14.04204238950079819 ) ) ;
#22553=CARTESIAN_POINT ( 'NONE',  ( 84.91875927444918659, 44.62694446506164070, -7.840877269613704570 ) ) ;
#22556=CARTESIAN_POINT ( 'NONE',  ( 76.26946404230704957, 64.97317754398874001, 14.67006731301515998 ) ) ;
#22560=ORIENTED_EDGE ( 'NONE', *, *, #15071, .T. ) ;
#22564=CARTESIAN_POINT ( 'NONE',  ( 87.34128990652536118, 44.33892918473014078, 4.514138355736077024 ) ) ;
#22574=CARTESIAN_POINT ( 'NONE',  ( 79.36528506407655925, 53.83448769205969597, -15.81908227153714819 ) ) ;
#22579=CARTESIAN_POINT ( 'NONE',  ( 70.66241353812237946, 61.03054431235825916, -14.44723600216412329 ) ) ;
#22580=CARTESIAN_POINT ( 'NONE',  ( 84.37825102736907468, 49.99960613749293969, 13.80049582259582763 ) ) ;
#22582=CARTESIAN_POINT ( 'NONE',  ( 71.20299867106878366, 71.49720395331284806, 2.862355716284322948 ) ) ;
#22589=CARTESIAN_POINT ( 'NONE',  ( 9.658441966945924051, 28.68290643055185996, 3.479690158560446702E-15 ) ) ;
#22594=CARTESIAN_POINT ( 'NONE',  ( 19.62422909362874535, 11.73415679381821342, 1.333680081654574804E-15 ) ) ;
#22599=CARTESIAN_POINT ( 'NONE',  ( 36.01387044229257128, 42.83396525600393545, -2.839279412974133887 ) ) ;
#22600=CARTESIAN_POINT ( 'NONE',  ( 42.95298936059631245, 26.92755873383629606, 6.180339887498953466 ) ) ;
#22603=CARTESIAN_POINT ( 'NONE',  ( 22.33066906249845118, 34.93396525600390845, 2.839279412974139660 ) ) ;
#22608=EDGE_CURVE ( 'NONE', #94224, #71267, #10449, .T. ) ;
#22611=CARTESIAN_POINT ( 'NONE',  ( 84.72527825293784076, 50.50787217764868586, -13.97547420692928277 ) ) ;
#22616=CARTESIAN_POINT ( 'NONE',  ( 74.98768007058501439, 53.07574299652110739, -16.50056621423362202 ) ) ;
#22618=ORIENTED_EDGE ( 'NONE', *, *, #86171, .F. ) ;
#22621=CARTESIAN_POINT ( 'NONE',  ( 34.90123498099573851, 22.01110640527294393, 2.839279412974134775 ) ) ;
#22622=ORIENTED_EDGE ( 'NONE', *, *, #83732, .F. ) ;
#22624=CARTESIAN_POINT ( 'NONE',  ( 86.60460766037567737, 43.36433298709366113, 1.857703978550338642 ) ) ;
#22626=LINE ( 'NONE', #68214, #86287 ) ;
#22628=CARTESIAN_POINT ( 'NONE',  ( 84.98383346588632037, 50.06751842512129258, 13.63401461718180485 ) ) ;
#22632=CARTESIAN_POINT ( 'NONE',  ( 31.85034293892215373, 41.49540643055189548, 3.479690158560446702E-15 ) ) ;
#22633=CARTESIAN_POINT ( 'NONE',  ( 81.56133095906432118, 55.49845989692713744, -16.32137983002411730 ) ) ;
#22647=CARTESIAN_POINT ( 'NONE',  ( 72.24150276065003595, 61.63636719674806130, -14.60790590827561530 ) ) ;
#22655=ORIENTED_EDGE ( 'NONE', *, *, #37082, .T. ) ;
#22657=CARTESIAN_POINT ( 'NONE',  ( 34.33172647011804912, 40.79752408145593989, -5.678558825948271327 ) ) ;
#22662=CARTESIAN_POINT ( 'NONE',  ( 74.19835002362358978, 68.51042020854130499, -11.60174470505228150 ) ) ;
#22664=CARTESIAN_POINT ( 'NONE',  ( 69.93873449799818331, 64.21434714275719102, -12.43005340421474259 ) ) ;
#22673=EDGE_LOOP ( 'NONE', ( #92305, #78451, #99807, #9318 ) ) ;
#22681=CARTESIAN_POINT ( 'NONE',  ( 81.68100823972521596, 43.51052942893925035, 8.843547683132065629 ) ) ;
#22687=CARTESIAN_POINT ( 'NONE',  ( 72.10222062648871599, 64.74920943772764304, 12.95471888058235344 ) ) ;
#22688=CARTESIAN_POINT ( 'NONE',  ( 82.32067382461301008, 40.78355318730610435, -3.695724402018718546 ) ) ;
#22695=CARTESIAN_POINT ( 'NONE',  ( 70.73151905446071908, 61.43491590206733832, -14.82309597659894429 ) ) ;
#22696=B_SPLINE_CURVE_WITH_KNOTS ( 'NONE', 3,
 ( #29096, #27605, #81827, #81335, #43770, #97510, #73697, #28082, #58471, #13879, #44761, #6280, #74714, #4281, #90437, #11909, #90934, #21484, #58952, #20502, #36171, #28577, #68072, #5291, #98996, #91411, #21975, #35180, #66090, #97036, #89444 ),
 .UNSPECIFIED., .F., .F.,
 ( 4, 3, 3, 3, 3, 3, 3, 3, 3, 3, 4 ),
 ( 0.000000000000000000, 0.1333490885032276307, 0.3007194338854349835, 0.4699862290245034879, 0.5844252810809318355, 0.6686540514502756771, 0.7354980260655390456, 0.8028463152565503691, 0.8633854507757023899, 0.9437142632666907227, 1.000000000000000000 ),
 .UNSPECIFIED. ) ;
#22697=CARTESIAN_POINT ( 'NONE',  ( 82.48332016352127027, 53.47388482021811740, -15.74481631320921693 ) ) ;
#22712=CARTESIAN_POINT ( 'NONE',  ( 72.15692581984221476, 72.29159277512509618, 3.751890296296640059 ) ) ;
#22717=CARTESIAN_POINT ( 'NONE',  ( 82.59751384975028543, 49.84330820394566786, -13.79983639419522312 ) ) ;
#22720=CARTESIAN_POINT ( 'NONE',  ( 26.73894555032740783, 17.29860640527292759, -2.839279412974138328 ) ) ;
#22723=CARTESIAN_POINT ( 'NONE',  ( 8.064688198948626763, 22.84336893147754211, -7.433330006724137462 ) ) ;
#22725=CARTESIAN_POINT ( 'NONE',  ( 76.98684284838461167, 63.68060895951392553, 15.36346902396294745 ) ) ;
#22728=CARTESIAN_POINT ( 'NONE',  ( 82.44105267360316702, 40.97854391121963147, -1.240873595747258529 ) ) ;
#22732=CARTESIAN_POINT ( 'NONE',  ( 76.13179367649587448, 56.49312099246306929, -16.15038315265565672 ) ) ;
#22733=CARTESIAN_POINT ( 'NONE',  ( 87.79271458260285499, 45.16522989489592987, -6.842624051142037089 ) ) ;
#22745=CARTESIAN_POINT ( 'NONE',  ( 79.06774487169295185, 46.04232138122480933, -12.65057773476749858 ) ) ;
#22751=CARTESIAN_POINT ( 'NONE',  ( 16.26188567080226477, 32.49540643055187417, 3.479690158560446702E-15 ) ) ;
#22753=CARTESIAN_POINT ( 'NONE',  ( 75.11209585957564627, 67.04221104021077338, -12.68919168548209342 ) ) ;
#22755=DIRECTION ( 'NONE',  ( 0.4556638457577293910, 0.000000000000000000, 0.8901519306664880116 ) ) ;
#22758=ORIENTED_EDGE ( 'NONE', *, *, #37319, .F. ) ;
#22761=EDGE_CURVE ( 'NONE', #16006, #44175, #74762, .T. ) ;
#22762=CARTESIAN_POINT ( 'NONE',  ( 72.19508862719266062, 67.24605117460401971, 11.71507738192612535 ) ) ;
#22763=CARTESIAN_POINT ( 'NONE',  ( 67.73377762630668997, 65.63987058315933609, -10.78464639375587453 ) ) ;
#22779=CARTESIAN_POINT ( 'NONE',  ( 66.97470778035078354, 67.57858517361454176, 6.667077613036518358 ) ) ;
#22783=CARTESIAN_POINT ( 'NONE',  ( 81.17822002178407104, 55.59913327053874355, 16.37131925982175318 ) ) ;
#22785=CARTESIAN_POINT ( 'NONE',  ( 71.83756684404445991, 67.75224793704757076, 10.40286433491243656 ) ) ;
#22790=CARTESIAN_POINT ( 'NONE',  ( 76.27683532132236621, 51.60822212622871774, -15.67723923137847386 ) ) ;
#22791=CARTESIAN_POINT ( 'NONE',  ( 76.28360139951196572, 65.00893075233551599, -14.26754816652215219 ) ) ;
#22798=CARTESIAN_POINT ( 'NONE',  ( 88.26308438319264837, 44.34169033064829080, 4.149168146237482979 ) ) ;
#22802=CARTESIAN_POINT ( 'NONE',  ( 79.48254265572808208, 59.20565343284910398, -16.22433428824159662 ) ) ;
#22815=CARTESIAN_POINT ( 'NONE',  ( 73.72034998377742454, 55.25731110591803485, 16.59469895887937341 ) ) ;
#22816=CARTESIAN_POINT ( 'NONE',  ( 29.44299306155908624, 19.12755873383627403, -6.180339887498949025 ) ) ;
#22823=ORIENTED_EDGE ( 'NONE', *, *, #97348, .T. ) ;
#22825=CARTESIAN_POINT ( 'NONE',  ( 72.71270868682043442, 70.26182901474604137, -8.036085614855659642 ) ) ;
#22826=CARTESIAN_POINT ( 'NONE',  ( 81.58025826021204807, 41.65040128036911682, 5.760828700905646471 ) ) ;
#22828=CARTESIAN_POINT ( 'NONE',  ( 30.05030659499110968, 29.30066082961423746, -10.00000000000000533 ) ) ;
#22829=CARTESIAN_POINT ( 'NONE',  ( 81.78504375891562006, 41.48292696562020865, -5.073134180756075473 ) ) ;
#22844=CARTESIAN_POINT ( 'NONE',  ( 34.45502471548058310, 41.93396525600392977, 2.839279412974139660 ) ) ;
#22850=CARTESIAN_POINT ( 'NONE',  ( 17.35762855594305520, 30.99752408145591431, 5.678558825948277544 ) ) ;
#22851=CARTESIAN_POINT ( 'NONE',  ( 6.386372903753387398, 27.18528772668516069, -1.583844403245363575 ) ) ;
#22852=CARTESIAN_POINT ( 'NONE',  ( 72.04081558064058299, 59.27854915901136934, 15.84716367784278646 ) ) ;
#22855=CARTESIAN_POINT ( 'NONE',  ( 81.47170367160930482, 45.92781089733199451, -12.16060789928866193 ) ) ;
#22856=CARTESIAN_POINT ( 'NONE',  ( 79.14312167556931854, 57.64441083166269664, 0.000000000000000000 ) ) ;
#22857=CARTESIAN_POINT ( 'NONE',  ( 81.40183131072419087, 42.44732485736221150, 7.480571600138957500 ) ) ;
#22861=CARTESIAN_POINT ( 'NONE',  ( 72.59758381146951933, 71.34453924857655238, -5.950632915609824103 ) ) ;
#22862=CARTESIAN_POINT ( 'NONE',  ( 72.67827274082560507, 57.12963284915914386, 16.37181230888942096 ) ) ;
#22863=CARTESIAN_POINT ( 'NONE',  ( 84.01948337656611443, 41.51492700183946738, 2.577254461289238741 ) ) ;
#22870=CARTESIAN_POINT ( 'NONE',  ( 20.92694685269868771, 35.58029201028043076, 1.583844403245363353 ) ) ;
#22871=CARTESIAN_POINT ( 'NONE',  ( 80.03821161748030022, 58.13657998254147685, 16.26793327978904458 ) ) ;
#22881=ORIENTED_EDGE ( 'NONE', *, *, #12141, .T. ) ;
#22898=CARTESIAN_POINT ( 'NONE',  ( 69.56645282547259512, 66.75238641213026369, 10.02794500564488445 ) ) ;
#22901=CARTESIAN_POINT ( 'NONE',  ( 73.74091326739588226, 64.78503309551670952, -13.53863873432484155 ) ) ;
#22902=CARTESIAN_POINT ( 'NONE',  ( 78.75079241178771383, 47.65652836985446328, 14.29454575176127840 ) ) ;
#22903=ORIENTED_EDGE ( 'NONE', *, *, #93627, .T. ) ;
#22906=CARTESIAN_POINT ( 'NONE',  ( 87.62838477539726512, 44.93552847577709031, -6.577990587745525808 ) ) ;
#22907=CARTESIAN_POINT ( 'NONE',  ( 79.49445812923981691, 46.35745038683718633, 12.69593692779722538 ) ) ;
#22909=CARTESIAN_POINT ( 'NONE',  ( 81.46918866590169728, 53.89730630895333974, -16.01726311077535669 ) ) ;
#22913=CARTESIAN_POINT ( 'NONE',  ( 72.24104924332462474, 71.74196171561413848, 5.528620549063446354 ) ) ;
#22922=DIRECTION ( 'NONE',  ( 0.5000000000000013323, -0.8660254037844378194, 0.000000000000000000 ) ) ;
#22923=CARTESIAN_POINT ( 'NONE',  ( 85.71994772693146558, 48.50907089644480408, -12.26219287530962454 ) ) ;
#22925=CARTESIAN_POINT ( 'NONE',  ( 71.14213006355628011, 63.76511893021699962, 13.21577267896801544 ) ) ;
#22928=B_SPLINE_CURVE_WITH_KNOTS ( 'NONE', 3,
 ( #8955, #94097, #32251, #61645, #84989, #9465, #69747, #79404, #77363, #86023, #32749, #39823, #54033, #9970, #48462, #86516, #7968, #23140, #30764, #55530, #62132, #87024, #69250, #63151, #77872, #15534, #54526, #358, #63653, #25146, #46434, #38841, #100178, #93078, #85507, #71275, #92594, #70754, #23634, #1367, #16054, #70246, #24648, #852, #47938, #31731 ),
 .UNSPECIFIED., .F., .F.,
 ( 4, 1, 2, 2, 1, 2, 2, 1, 1, 2, 2, 1, 1, 2, 2, 1, 1, 2, 2, 1, 1, 1, 2, 2, 1, 1, 1, 2, 2, 4 ),
 ( 0.000000000000000000, 0.06250000000000761891, 0.09375000000001204592, 0.1250000000000164591, 0.1875000000000217604, 0.2187500000000238420, 0.2500000000000258682, 0.3125000000000270894, 0.3437500000000293654, 0.3593750000000304756, 0.3750000000000315858, 0.4375000000000447420, 0.4687500000000518474, 0.4843750000000553446, 0.5000000000000587308, 0.5625000000000682787, 0.5937500000000717204, 0.6093750000000711653, 0.6250000000000706102, 0.6875000000000704992, 0.7187500000000703881, 0.7343750000000703881, 0.7421875000000709433, 0.7500000000000713873, 0.8125000000000638378, 0.8437500000000596190, 0.8593750000000576206, 0.8671875000000563993, 0.8750000000000552891, 1.000000000000000000 ),
 .UNSPECIFIED. ) ;
#22935=CARTESIAN_POINT ( 'NONE',  ( 41.03800390905408335, 35.64441083166263979, -10.00000000000000533 ) ) ;
#22938=B_SPLINE_CURVE_WITH_KNOTS ( 'NONE', 3,
 ( #42895, #35321, #88595, #73344, #66233, #97170, #34814, #26240, #88097, #49526, #80479, #94494, #16452, #85929, #24552, #9361, #63058, #24055, #64568, #86926, #41242, #95525, #34167, #18474, #78776, #26070, #47350, #9883, #25054, #48367, #55929, #56946, #72693, #41749, #71181, #40740, #94000, #87932, #49361, #10371, #65059, #95006, #48873, #80305, #47836, #79807 ),
 .UNSPECIFIED., .F., .F.,
 ( 4, 1, 2, 2, 1, 2, 2, 1, 1, 2, 2, 1, 1, 2, 2, 1, 1, 2, 2, 1, 1, 1, 2, 2, 1, 1, 1, 2, 2, 4 ),
 ( 0.000000000000000000, 0.06250000000000634215, 0.09375000000001049161, 0.1250000000000146272, 0.1875000000000240918, 0.2187500000000283662, 0.2500000000000326406, 0.3125000000000425215, 0.3437500000000481282, 0.3593750000000495715, 0.3750000000000510703, 0.4375000000000504596, 0.4687500000000502376, 0.4843750000000494604, 0.5000000000000487388, 0.5625000000000442979, 0.5937500000000436318, 0.6093750000000419664, 0.6250000000000403011, 0.6875000000000366374, 0.7187500000000347500, 0.7343750000000338618, 0.7421875000000334177, 0.7500000000000329736, 0.8125000000000348610, 0.8437500000000348610, 0.8593750000000339728, 0.8671875000000327516, 0.8750000000000314193, 1.000000000000000000 ),
 .UNSPECIFIED. ) ;
#22941=CARTESIAN_POINT ( 'NONE',  ( 12.03141808487008824, 12.11029122506292488, -8.090169943749478065 ) ) ;
#22944=CARTESIAN_POINT ( 'NONE',  ( 66.60661563016273590, 67.77273566365288104, -7.043189648870076702 ) ) ;
#22948=CARTESIAN_POINT ( 'NONE',  ( 73.06869489861219336, 57.16488433617836762, 16.39886474625613388 ) ) ;
#22950=CARTESIAN_POINT ( 'NONE',  ( 8.494131180097229006, 27.83705186507752671, 3.090169943749475401 ) ) ;
#22952=VERTEX_POINT ( 'NONE', #2241 ) ;
#22956=CARTESIAN_POINT ( 'NONE',  ( 32.78250297933140445, 27.43085787977765477, -9.188101187500008038 ) ) ;
#22961=CARTESIAN_POINT ( 'NONE',  ( 67.99021540693823340, 66.60164882251528695, 9.921589984831021169 ) ) ;
#22963=CARTESIAN_POINT ( 'NONE',  ( 68.55207038212054727, 64.21588461577663054, 11.81441866468647994 ) ) ;
#22964=ORIENTED_EDGE ( 'NONE', *, *, #42132, .T. ) ;
#22967=CARTESIAN_POINT ( 'NONE',  ( 5.396842180905148112, 18.51421378149916563, -9.188101187500004485 ) ) ;
#22969=CARTESIAN_POINT ( 'NONE',  ( 16.17343562415726765, 11.19860640527290840, 2.839279412974134775 ) ) ;
#22970=ORIENTED_EDGE ( 'NONE', *, *, #2899, .T. ) ;
#22973=CARTESIAN_POINT ( 'NONE',  ( 69.78620060459685703, 62.54818963133106280, 13.43547245615845576 ) ) ;
#22981=FACE_OUTER_BOUND ( 'NONE', #72870, .T. ) ;
#22985=CARTESIAN_POINT ( 'NONE',  ( 85.44270010841485430, 45.05997736202789383, -8.111341735673667230 ) ) ;
#22986=ORIENTED_EDGE ( 'NONE', *, *, #57301, .F. ) ;
#22988=CARTESIAN_POINT ( 'NONE',  ( 78.99848661620950452, 60.24637179098724005, -16.44349368446546578 ) ) ;
#22990=CARTESIAN_POINT ( 'NONE',  ( 69.35874604783040809, 62.81868137753772174, 13.70911004653519250 ) ) ;
#22997=VERTEX_POINT ( 'NONE', #55393 ) ;
#22999=ORIENTED_EDGE ( 'NONE', *, *, #97908, .F. ) ;
#23000=CARTESIAN_POINT ( 'NONE',  ( 80.31295028949705284, 46.37567276318792153, 12.40275564728421109 ) ) ;
#23002=CARTESIAN_POINT ( 'NONE',  ( 67.73206951906773554, 67.71102699734191788, 7.258094484230766419 ) ) ;
#23005=CARTESIAN_POINT ( 'NONE',  ( 82.07162566433116524, 45.76690361501738380, 11.08599694920283341 ) ) ;
#23008=CARTESIAN_POINT ( 'NONE',  ( 69.37941880040793308, 68.43494161156023381, -7.694138334527842460 ) ) ;
#23009=EDGE_LOOP ( 'NONE', ( #65604, #87668, #40344, #94322 ) ) ;
#23011=CARTESIAN_POINT ( 'NONE',  ( 12.16147613323643029, 27.99752408145590721, 5.678558825948277544 ) ) ;
#23012=EDGE_CURVE ( 'NONE', #50839, #84127, #4807, .T. ) ;
#23014=CARTESIAN_POINT ( 'NONE',  ( 80.61280386015431532, 57.63106766464478881, 16.59051181579431500 ) ) ;
#23015=DIRECTION ( 'NONE',  ( -0.8660254037844377084, -0.5000000000000014433, -0.000000000000000000 ) ) ;
#23019=DIRECTION ( 'NONE',  ( 0.5778974349098185970, 0.4186690413702512936, 0.7005360722495072023 ) ) ;
#23020=CARTESIAN_POINT ( 'NONE',  ( 67.73742752091094133, 65.62596870563270102, -10.80114651390334757 ) ) ;
#23028=CARTESIAN_POINT ( 'NONE',  ( 82.56883094741532148, 53.27102910656019930, -15.30881521583544647 ) ) ;
#23039=CARTESIAN_POINT ( 'NONE',  ( 82.98418032785382081, 46.47283061845390506, -11.29752663545136215 ) ) ;
#23042=CARTESIAN_POINT ( 'NONE',  ( 82.55199557336824512, 43.02032421242048343, 7.382427009242009674 ) ) ;
#23057=EDGE_CURVE ( 'NONE', #60539, #49096, #56967, .T. ) ;
#23071=CARTESIAN_POINT ( 'NONE',  ( 13.78045586392592092, 26.14336893147754282, 7.433330006724141015 ) ) ;
#23074=CARTESIAN_POINT ( 'NONE',  ( 75.16541093910677773, 58.59821464833535742, -16.37950748201892992 ) ) ;
#23076=CARTESIAN_POINT ( 'NONE',  ( 66.42189003655407475, 68.72454749333068946, 2.359676567546969750 ) ) ;
#23083=CARTESIAN_POINT ( 'NONE',  ( 83.00815485991435594, 53.30142267139499523, 15.60062745561815767 ) ) ;
#23085=CARTESIAN_POINT ( 'NONE',  ( 25.24689923506580769, 37.68290643055188838, 3.479690158560446702E-15 ) ) ;
#23086=CARTESIAN_POINT ( 'NONE',  ( 70.43005528255592651, 64.46647551784276686, -13.05606537066291573 ) ) ;
#23091=ORIENTED_EDGE ( 'NONE', *, *, #64612, .F. ) ;
#23093=CARTESIAN_POINT ( 'NONE',  ( 78.89717507877558944, 49.06168382820697360, 14.38932173611067356 ) ) ;
#23099=CARTESIAN_POINT ( 'NONE',  ( 31.98863997849372254, 36.65586893147758474, -7.433330006724137462 ) ) ;
#23100=VERTEX_POINT ( 'NONE', #27533 ) ;
#23102=CARTESIAN_POINT ( 'NONE',  ( 81.78504375891562006, 41.48292696562020865, -5.073134180756075473 ) ) ;
#23104=CARTESIAN_POINT ( 'NONE',  ( 86.33714660501533444, 47.00371335520402738, -10.02508334048726546 ) ) ;
#23111=CARTESIAN_POINT ( 'NONE',  ( 81.53672410393728853, 56.04530558232496418, -16.40539795406884949 ) ) ;
#23112=DIRECTION ( 'NONE',  ( -0.5000000000000082157, 0.8660254037844338226, 0.000000000000000000 ) ) ;
#23114=B_SPLINE_CURVE_WITH_KNOTS ( 'NONE', 3,
 ( #3437, #19638, #57097, #72343, #34798, #34314, #65212, #96154, #64212, #80462, #11033, #3915, #73328, #89089, #88080, #65700 ),
 .UNSPECIFIED., .F., .F.,
 ( 4, 1, 2, 2, 2, 1, 2, 2, 4 ),
 ( 0.000000000000000000, 0.1249999999999995559, 0.1874999999999993339, 0.2499999999999991118, 0.4999999999999977240, 0.6249999999999972244, 0.6874999999999971134, 0.7499999999999970024, 1.000000000000000000 ),
 .UNSPECIFIED. ) ;
#23117=VERTEX_POINT ( 'NONE', #66999 ) ;
#23121=CARTESIAN_POINT ( 'NONE',  ( 76.20055470335279324, 65.09253202017347917, 14.18943646504600054 ) ) ;
#23124=CARTESIAN_POINT ( 'NONE',  ( 82.45865130729738723, 40.97087310285034079, 1.023290110074061898 ) ) ;
#23129=CARTESIAN_POINT ( 'NONE',  ( 70.58939099706752529, 60.68707437868734189, -14.57694795185084580 ) ) ;
#23130=CARTESIAN_POINT ( 'NONE',  ( 37.11382629638189457, 33.37878583063844218, 9.188101187500006262 ) ) ;
#23134=CARTESIAN_POINT ( 'NONE',  ( 86.78119538955827750, 45.86439926875618767, -8.245237605873949605 ) ) ;
#23135=CARTESIAN_POINT ( 'NONE',  ( 71.60199290673480732, 63.90083948714775630, -13.28680243790413051 ) ) ;
#23140=CARTESIAN_POINT ( 'NONE',  ( 72.92328079741919566, 65.18747506910628431, 13.02211304875830677 ) ) ;
#23145=VERTEX_POINT ( 'NONE', #83237 ) ;
#23147=DIRECTION ( 'NONE',  ( 0.5000000000000013323, -0.8660254037844378194, 0.000000000000000000 ) ) ;
#23149=DIRECTION ( 'NONE',  ( 0.5000000000000013323, -0.8660254037844378194, 0.000000000000000000 ) ) ;
#23155=CARTESIAN_POINT ( 'NONE',  ( 69.97821611620445026, 71.48374793263995741, -1.182227389098916781 ) ) ;
#23162=CARTESIAN_POINT ( 'NONE',  ( 71.94540097076600205, 64.24250455633612944, 13.20799783956320539 ) ) ;
#23170=CARTESIAN_POINT ( 'NONE',  ( 83.23481903784592362, 43.31313429786332847, 7.200028244731907279 ) ) ;
#23171=LINE ( 'NONE', #53082, #75414 ) ;
#23173=CARTESIAN_POINT ( 'NONE',  ( 71.09952580927735255, 66.44067406087256700, -11.85013464261816374 ) ) ;
#23182=CARTESIAN_POINT ( 'NONE',  ( 73.58959834336499739, 69.25141985266563438, -10.00371726299768405 ) ) ;
#23183=CARTESIAN_POINT ( 'NONE',  ( 76.45248566530659673, 51.50253309734852536, 15.63309938903474361 ) ) ;
#23184=CARTESIAN_POINT ( 'NONE',  ( 4.858991816890471327, 18.50829794293877839, -10.00000000000000355 ) ) ;
#23193=CARTESIAN_POINT ( 'NONE',  ( 88.10956888842845558, 44.04735113414163550, 0.5588696975863149952 ) ) ;
#23195=CARTESIAN_POINT ( 'NONE',  ( 82.22870199775800870, 49.95230068291388648, -13.96007491776960840 ) ) ;
#23200=CARTESIAN_POINT ( 'NONE',  ( 25.85429974905589390, 23.43085787977764411, -9.188101187500008038 ) ) ;
#23203=CARTESIAN_POINT ( 'NONE',  ( 11.99789328850488879, 15.43085787977761569, -9.188101187500008038 ) ) ;
#23205=CARTESIAN_POINT ( 'NONE',  ( 77.10733807873376122, 63.61886353868632682, 15.40965320646045100 ) ) ;
#23211=CARTESIAN_POINT ( 'NONE',  ( 79.17827112357750252, 55.43091488132045441, -16.07850425917232684 ) ) ;
#23212=CARTESIAN_POINT ( 'NONE',  ( 87.67760366270776728, 45.22517868708455069, -6.234814096420206120 ) ) ;
#23218=CARTESIAN_POINT ( 'NONE',  ( 77.33837241094562387, 49.21827100037820202, 15.32655703911426670 ) ) ;
#23219=CARTESIAN_POINT ( 'NONE',  ( 82.78345634833956979, 53.69061190982764487, 15.38144188222361208 ) ) ;
#23225=AXIS2_PLACEMENT_3D ( 'NONE', #83176, #46111, #84187 ) ;
#23227=CARTESIAN_POINT ( 'NONE',  ( 79.98829826350832661, 44.59498145193617802, 11.76229303994366582 ) ) ;
#23230=ORIENTED_EDGE ( 'NONE', *, *, #81631, .F. ) ;
#23231=CARTESIAN_POINT ( 'NONE',  ( 24.28583178621855865, 34.99752408145592142, 5.678558825948276656 ) ) ;
#23232=FACE_OUTER_BOUND ( 'NONE', #78874, .T. ) ;
#23240=( BOUNDED_CURVE ( )  B_SPLINE_CURVE ( 2, ( #62304, #17214, #48121, #79065, #40509, #10133, #49133, #80067, #71443, #2031, #31910, #33428, #64325 ),
 .UNSPECIFIED., .F., .T. ) 
 B_SPLINE_CURVE_WITH_KNOTS ( ( 3, 2, 2, 2, 2, 2, 3 ),
 ( 0.6875000000000000000, 0.6899999999999999467, 0.6949999999999999512, 0.6999999999999999556, 0.7049999999999999600, 0.7099999999999999645, 0.7125000000000000222 ),
 .UNSPECIFIED. ) 
 CURVE ( )  GEOMETRIC_REPRESENTATION_ITEM ( )  RATIONAL_B_SPLINE_CURVE ( ( 0.9755282581475768211, 0.9755282581475768211, 1.000000000000000000, 0.9510565162951535312, 1.000000000000000000, 0.9510565162951535312, 1.000000000000000000, 0.9510565162951535312, 1.000000000000000000, 0.9510565162951535312, 1.000000000000000000, 0.9755282581475761550, 0.9755282581475767101 ) ) 
 REPRESENTATION_ITEM ( '' )  );
#23241=CARTESIAN_POINT ( 'NONE',  ( 67.78340610521031806, 65.54725019734833324, 10.17040391041397029 ) ) ;
#23242=CARTESIAN_POINT ( 'NONE',  ( 67.76021416997799918, 65.93326558605815535, -10.49598374965347425 ) ) ;
#23253=CARTESIAN_POINT ( 'NONE',  ( 73.91099221338522796, 59.87250767674520091, -15.97378689575042898 ) ) ;
#23255=ORIENTED_EDGE ( 'NONE', *, *, #83732, .T. ) ;
#23258=CARTESIAN_POINT ( 'NONE',  ( 66.59391288086393956, 67.82822080634741724, 6.925870058277245001 ) ) ;
#23263=CARTESIAN_POINT ( 'NONE',  ( 72.19772409968021520, 68.63628420467338742, 9.688590869373431502 ) ) ;
#23265=VERTEX_POINT ( 'NONE', #34495 ) ;
#23270=B_SPLINE_CURVE_WITH_KNOTS ( 'NONE', 3,
 ( #37196, #60479, #90956, #43294, #36690, #36193, #74242, #60983, #53390, #67599, #75222, #82366, #37682, #22499, #12936, #59481, #91948, #13425, #75721, #67099, #43795, #52397, #68594, #74738, #4827, #82855, #44294, #58977, #20524, #59986, #14410 ),
 .UNSPECIFIED., .F., .F.,
 ( 4, 3, 3, 3, 3, 3, 3, 3, 3, 3, 4 ),
 ( 0.000000000000000000, 0.1333490885032353190, 0.3007194338854385363, 0.4699862290245196972, 0.5844252810809350551, 0.6686540514502717913, 0.7354980260655500368, 0.8028463152565585847, 0.8633854507757243724, 0.9437142632667462339, 1.000000000000000000 ),
 .UNSPECIFIED. ) ;
#23271=EDGE_CURVE ( 'NONE', #55813, #58122, #57785, .T. ) ;
#23272=CARTESIAN_POINT ( 'NONE',  ( 76.12288495599533178, 65.36913255257266542, -14.03413756946655511 ) ) ;
#23280=CARTESIAN_POINT ( 'NONE',  ( 29.52096178950397842, 38.81751292744058190, -6.180339887498951690 ) ) ;
#23282=ADVANCED_FACE ( 'NONE', ( #68255 ), #66394, .T. ) ;
#23283=CARTESIAN_POINT ( 'NONE',  ( 72.47401207315012073, 70.81051498135123268, 7.656770371261354846 ) ) ;
#23290=PLANE ( 'NONE',  #85139 ) ;
#23292=CARTESIAN_POINT ( 'NONE',  ( 83.73865579866679809, 51.98612588642360066, 14.96617132975018549 ) ) ;
#23300=CARTESIAN_POINT ( 'NONE',  ( 73.76528436707422998, 55.26057213895941089, 16.11941679284131723 ) ) ;
#23302=CARTESIAN_POINT ( 'NONE',  ( 22.85147042958088193, 25.14441083166261137, 10.00000000000000533 ) ) ;
#23312=EDGE_CURVE ( 'NONE', #20229, #25358, #18836, .T. ) ;
#23313=CARTESIAN_POINT ( 'NONE',  ( 73.10205918017362592, 70.55621008947603912, -7.923255499225144050 ) ) ;
#23317=CARTESIAN_POINT ( 'NONE',  ( 75.48012123272684448, 53.33211347937982794, 16.49774674189050927 ) ) ;
#23318=CARTESIAN_POINT ( 'NONE',  ( 30.91633199877554716, 29.80066082961423746, 10.00000000000000533 ) ) ;
#23319=CARTESIAN_POINT ( 'NONE',  ( 76.72630680417243809, 51.77891733241483507, 16.15279506092123540 ) ) ;
#23330=CARTESIAN_POINT ( 'NONE',  ( 72.79894534421406149, 70.83549005279603250, -7.921956013610881975 ) ) ;
#23339=CARTESIAN_POINT ( 'NONE',  ( 20.65934362447757167, 23.87878583063841376, -9.188101187500006262 ) ) ;
#23345=CARTESIAN_POINT ( 'NONE',  ( 41.60633307851366425, 35.97253583063845639, -9.188101187500006262 ) ) ;
#23346=CARTESIAN_POINT ( 'NONE',  ( 81.65310433048475147, 42.64019311979919991, 7.560891536010019287 ) ) ;
#23347=CARTESIAN_POINT ( 'NONE',  ( 82.80564809338142140, 40.64392876451551473, -1.326136484204850197 ) ) ;
#23350=CARTESIAN_POINT ( 'NONE',  ( 72.40747426417379984, 71.81324781307232286, -5.589457107701495175 ) ) ;
#23359=CARTESIAN_POINT ( 'NONE',  ( 71.64316818921395225, 72.05741665177615118, -3.509880912999884917 ) ) ;
#23360=DIRECTION ( 'NONE',  ( -0.8660254037844379305, -0.5000000000000014433, -0.000000000000000000 ) ) ;
#23371=CARTESIAN_POINT ( 'NONE',  ( 26.87427219475921092, 30.91421378149919974, 9.188101187500008038 ) ) ;
#23381=CARTESIAN_POINT ( 'NONE',  ( 86.85148033070495899, 46.48268733558807497, 9.045030158509874241 ) ) ;
#23392=CARTESIAN_POINT ( 'NONE',  ( 67.59761362805406293, 66.71094541649533483, 8.633997586817105940 ) ) ;
#23394=CARTESIAN_POINT ( 'NONE',  ( 78.12507825963197661, 47.72428238059148953, 14.50788938415275986 ) ) ;
#23398=DIRECTION ( 'NONE',  ( -0.03487823687206607903, 0.06041087834084090530, 0.9975640502598237536 ) ) ;
#23399=CARTESIAN_POINT ( 'NONE',  ( 87.65912573706349065, 45.31011780831707370, -7.252675111195947544 ) ) ;
#23404=CARTESIAN_POINT ( 'NONE',  ( 83.82342001511069896, 52.04024975599947567, -14.96847033955516260 ) ) ;
#23406=ORIENTED_EDGE ( 'NONE', *, *, #2276, .T. ) ;
#23409=CARTESIAN_POINT ( 'NONE',  ( 72.17587820367440088, 71.48161267280252673, 5.042060180291768390 ) ) ;
#23417=CARTESIAN_POINT ( 'NONE',  ( 68.49666587867349676, 66.34648026219538508, -9.764362443893059407 ) ) ;
#23419=CARTESIAN_POINT ( 'NONE',  ( 71.29672626941692215, 64.26515988479742703, 12.96738178296346966 ) ) ;
#23421=CARTESIAN_POINT ( 'NONE',  ( 80.20857538925844210, 44.21345027839176112, -11.30608575764589752 ) ) ;
#23429=B_SPLINE_SURFACE_WITH_KNOTS ( 'NONE', 3, 1, ( 
 ( #82725, #89343 ),
 ( #74093, #28984 ),
 ( #13295, #3699 ),
 ( #4686, #97399 ),
 ( #67466, #89817 ),
 ( #98392, #88852 ),
 ( #20391, #74607 ),
 ( #36062, #5181 ),
 ( #44154, #75090 ),
 ( #5669, #59859 ),
 ( #90822, #21375 ),
 ( #52264, #11313 ),
 ( #45644, #84214 ),
 ( #75580, #29963 ),
 ( #85202, #54234 ),
 ( #14761, #6167 ),
 ( #83203, #7661 ),
 ( #83710, #91302 ),
 ( #53260, #22857 ),
 ( #38549, #53741 ),
 ( #91800, #52748 ),
 ( #84701, #76571 ),
 ( #44646, #61353 ),
 ( #61845, #15746 ),
 ( #92308, #8167 ),
 ( #21864, #14268 ),
 ( #7152, #15240 ),
 ( #30461, #45159 ),
 ( #93294, #46137 ),
 ( #92792, #76097 ),
 ( #39038, #23346 ) ),
 .UNSPECIFIED., .F., .F., .F.,
 ( 4, 3, 3, 3, 3, 3, 3, 3, 3, 3, 4 ),
 ( 2, 2 ),
 ( 0.000000000000000000, 0.1122669598086733639, 0.2243161639709615740, 0.3396355846219071828, 0.4553962076585117424, 0.5677860799922423984, 0.6749047109689585433, 0.7773884377078229546, 0.8775581155834157876, 0.9782364162377870098, 1.000000000000000000 ),
 ( 0.000000000000000000, 1.000000000000000000 ),
 .UNSPECIFIED. ) ;
#23434=CARTESIAN_POINT ( 'NONE',  ( 20.71649992267561302, 12.36477965099639853, 1.583844403245364907 ) ) ;
#23436=CARTESIAN_POINT ( 'NONE',  ( 16.72324493992723049, 11.78380873178785748, -6.180339887498949025 ) ) ;
#23437=LINE ( 'NONE', #31539, #54834 ) ;
#23443=CARTESIAN_POINT ( 'NONE',  ( 73.09454433421316821, 57.18998214774231315, 16.39745951563025628 ) ) ;
#23444=CARTESIAN_POINT ( 'NONE',  ( 69.17743059381074033, 64.85395446877666359, 12.24194748396287480 ) ) ;
#23445=CARTESIAN_POINT ( 'NONE',  ( 9.082762260191243442, 27.01751292744054567, 6.180339887498949913 ) ) ;
#23450=CARTESIAN_POINT ( 'NONE',  ( 29.08566721201706784, 38.83396525600392124, -2.839279412974133887 ) ) ;
#23454=CARTESIAN_POINT ( 'NONE',  ( 66.45738049687504656, 68.75004886898103962, 2.331916367499077047 ) ) ;
#23457=DIRECTION ( 'NONE',  ( 1.000000000000000000, 0.000000000000000000, 0.000000000000000000 ) ) ;
#23461=CARTESIAN_POINT ( 'NONE',  ( 6.194340351808173217, 26.68290643055185285, 3.479690158560446702E-15 ) ) ;
#23463=DIRECTION ( 'NONE',  ( -0.4556638457577367740, 0.000000000000000000, 0.8901519306664842368 ) ) ;
#23467=CARTESIAN_POINT ( 'NONE',  ( 73.51948839908328637, 69.73627507762921596, -9.361350578256052657 ) ) ;
#23471=ORIENTED_EDGE ( 'NONE', *, *, #70133, .F. ) ;
#23476=CARTESIAN_POINT ( 'NONE',  ( 69.85203827438495239, 67.76287465637892637, 9.808276934428768357 ) ) ;
#23477=CARTESIAN_POINT ( 'NONE',  ( 82.46142967334674267, 45.35300679235661647, -10.49381007413441580 ) ) ;
#23480=CARTESIAN_POINT ( 'NONE',  ( 79.50781411973173363, 59.26880192752088305, -16.22028800479747801 ) ) ;
#23482=CARTESIAN_POINT ( 'NONE',  ( 75.31289280905393468, 53.62176160565092431, -16.53289957284814093 ) ) ;
#23483=CARTESIAN_POINT ( 'NONE',  ( 69.93520613851926271, 62.85125605636124391, 13.88333920316857650 ) ) ;
#23492=CARTESIAN_POINT ( 'NONE',  ( 73.12515255232021616, 60.21910268995390680, 15.28705970489183841 ) ) ;
#23494=ORIENTED_EDGE ( 'NONE', *, *, #75401, .F. ) ;
#23498=CARTESIAN_POINT ( 'NONE',  ( 81.14441644904596274, 43.83121929228919811, 9.603772945707428121 ) ) ;
#23501=CARTESIAN_POINT ( 'NONE',  ( 67.07370046796862084, 68.19344093013617680, -5.526046699112809435 ) ) ;
#23503=ORIENTED_EDGE ( 'NONE', *, *, #9183, .F. ) ;
#23505=CARTESIAN_POINT ( 'NONE',  ( 20.49695707787433463, 14.76004757982089188, 5.678558825948272215 ) ) ;
#23511=CARTESIAN_POINT ( 'NONE',  ( 70.37934122712871954, 61.23818324669216651, 14.28954007458889386 ) ) ;
#23515=CARTESIAN_POINT ( 'NONE',  ( 80.82947773944196967, 46.16309167796865864, -12.01060402535779836 ) ) ;
#23519=( BOUNDED_CURVE ( )  B_SPLINE_CURVE ( 2, ( #47290, #78215, #92928, #87748, #30607, #15892, #45782, #85345, #80119, #38178, #15378, #8801, #77200 ),
 .UNSPECIFIED., .F., .T. ) 
 B_SPLINE_CURVE_WITH_KNOTS ( ( 3, 2, 2, 2, 2, 2, 3 ),
 ( 0.1375000000000000111, 0.1400000000000000133, 0.1449999999999999900, 0.1499999999999999944, 0.1549999999999999989, 0.1600000000000000033, 0.1625000000000000056 ),
 .UNSPECIFIED. ) 
 CURVE ( )  GEOMETRIC_REPRESENTATION_ITEM ( )  RATIONAL_B_SPLINE_CURVE ( ( 0.9755282581475768211, 0.9755282581475768211, 1.000000000000000000, 0.9510565162951535312, 1.000000000000000000, 0.9510565162951535312, 1.000000000000000000, 0.9510565162951535312, 1.000000000000000000, 0.9510565162951535312, 1.000000000000000000, 0.9755282581475768211, 0.9755282581475768211 ) ) 
 REPRESENTATION_ITEM ( '' )  );
#23522=CARTESIAN_POINT ( 'NONE',  ( 74.70969265356585254, 66.80295132244253864, -13.14574923971307463 ) ) ;
#23531=DIRECTION ( 'NONE',  ( 0.1710100716628310258, -0.2961981327260192476, 0.9396926207859104263 ) ) ;
#23540=CARTESIAN_POINT ( 'NONE',  ( 82.26786778050022519, 42.61060261517380354, 6.935189047524418449 ) ) ;
#23541=CARTESIAN_POINT ( 'NONE',  ( 74.18809600170575891, 68.48282398988669684, -11.62097119590897520 ) ) ;
#23549=CARTESIAN_POINT ( 'NONE',  ( 80.65606772055953400, 57.41663775889262666, -16.23641822966148851 ) ) ;
#23555=CARTESIAN_POINT ( 'NONE',  ( 73.42390341037517487, 68.98804980449470747, 10.73942965338376254 ) ) ;
#23558=CARTESIAN_POINT ( 'NONE',  ( 69.95749256914241698, 70.12926228225454395, 4.955899210846575365 ) ) ;
#23566=CARTESIAN_POINT ( 'NONE',  ( 11.61057445305848823, 22.10171378149917842, 9.188101187500008038 ) ) ;
#23569=CARTESIAN_POINT ( 'NONE',  ( 74.14070847040734691, 58.91510108708826721, -16.21268320586513667 ) ) ;
#23572=B_SPLINE_CURVE_WITH_KNOTS ( 'NONE', 3,
 ( #50770, #36562, #6674, #97894, #44649, #89820, #28987, #20395, #89346, #90326, #75584, #20900, #51265, #5185, #44158, #21867, #81721, #51789, #6170, #37067, #12297, #67971, #98892, #93297, #16759, #7156, #70459, #22366, #86223, #62343, #69462, #45647, #76575, #24370, #84218, #93810, #38043, #99879, #15245, #69951, #77, #7666, #40043, #60843, #78078, #9169 ),
 .UNSPECIFIED., .F., .F.,
 ( 4, 1, 1, 1, 2, 2, 1, 1, 1, 2, 2, 1, 1, 2, 2, 1, 1, 2, 2, 1, 1, 2, 2, 1, 2, 2, 1, 2, 2, 4 ),
 ( 0.000000000000000000, 0.06250000000000936751, 0.09375000000001323941, 0.1093750000000151545, 0.1171875000000152933, 0.1250000000000154321, 0.1875000000000056899, 0.2187500000000019706, 0.2343749999999997224, 0.2421874999999978628, 0.2499999999999960032, 0.3124999999999953371, 0.3437499999999956701, 0.3593749999999965028, 0.3749999999999973355, 0.4375000000000029976, 0.4687500000000058842, 0.4843750000000073275, 0.5000000000000087708, 0.5625000000000085487, 0.5937500000000077716, 0.6093750000000073275, 0.6250000000000068834, 0.6875000000000107692, 0.7187500000000114353, 0.7500000000000121014, 0.8125000000000128786, 0.8437500000000117684, 0.8750000000000106581, 1.000000000000000000 ),
 .UNSPECIFIED. ) ;
#23578=CARTESIAN_POINT ( 'NONE',  ( 66.89668164680340112, 69.73571018825775525, 0.6674377462804911287 ) ) ;
#23582=CARTESIAN_POINT ( 'NONE',  ( 81.22341047923954704, 48.06708024569342541, 13.74252432062430529 ) ) ;
#23584=ORIENTED_EDGE ( 'NONE', *, *, #47287, .F. ) ;
#23585=CARTESIAN_POINT ( 'NONE',  ( 75.84116199970137018, 65.13315491392486933, -14.47742810051069284 ) ) ;
#23588=CARTESIAN_POINT ( 'NONE',  ( 72.40022343535652283, 71.86297034063233014, -5.456689119915505870 ) ) ;
#23589=CARTESIAN_POINT ( 'NONE',  ( 74.95434044882874502, 53.24670644474785064, -16.03982845221052855 ) ) ;
#23592=CARTESIAN_POINT ( 'NONE',  ( 73.33758058659837786, 69.90254644623917102, 9.645949167502998023 ) ) ;
#23593=CARTESIAN_POINT ( 'NONE',  ( 38.84587710395076954, 34.37878583063844218, 9.188101187500006262 ) ) ;
#23599=CARTESIAN_POINT ( 'NONE',  ( 86.12135434523639788, 46.98046262810482432, -10.13131473785488268 ) ) ;
#23605=CARTESIAN_POINT ( 'NONE',  ( 81.35996782917339942, 56.22057934968196946, -16.44131086233301176 ) ) ;
#23606=ORIENTED_EDGE ( 'NONE', *, *, #2141, .F. ) ;
#23609=CARTESIAN_POINT ( 'NONE',  ( 77.16544646929735052, 49.29022895602057019, -14.87484003624337880 ) ) ;
#23611=CARTESIAN_POINT ( 'NONE',  ( 87.17617632782311432, 45.93339551703158463, -8.679440343565334004 ) ) ;
#23612=CARTESIAN_POINT ( 'NONE',  ( 79.83401254395657531, 57.87045807247318407, 16.26439772172797404 ) ) ;
#23615=CARTESIAN_POINT ( 'NONE',  ( 26.40327033588000560, 37.01751292744058475, 6.180339887498949913 ) ) ;
#23620=CARTESIAN_POINT ( 'NONE',  ( 77.00353437484392316, 62.91037619732002639, -15.26141501223570707 ) ) ;
#23623=CARTESIAN_POINT ( 'NONE',  ( 70.52897103333525308, 60.84962709411536252, -15.02099117819446761 ) ) ;
#23634=CARTESIAN_POINT ( 'NONE',  ( 71.83446468542571495, 61.06084060420133852, 14.73407088629796746 ) ) ;
#23636=CARTESIAN_POINT ( 'NONE',  ( 78.25402821438737533, 51.50098827152044834, 15.87605948207779605 ) ) ;
#23643=CARTESIAN_POINT ( 'NONE',  ( 65.80085019850238837, 69.11466268455660611, -0.2884749532225020507 ) ) ;
#23654=ORIENTED_EDGE ( 'NONE', *, *, #79298, .T. ) ;
#23656=CARTESIAN_POINT ( 'NONE',  ( 71.68455251971286657, 63.38995168949250569, 13.60462078634210670 ) ) ;
#23665=CARTESIAN_POINT ( 'NONE',  ( 69.48347394385132247, 66.66933067140242031, -10.76623218384503744 ) ) ;
#23672=CARTESIAN_POINT ( 'NONE',  ( 78.61102955532449243, 58.84556920875776598, 16.19509477467131831 ) ) ;
#23673=CARTESIAN_POINT ( 'NONE',  ( 84.57213519662508361, 49.80120436375268156, -13.19968558455237861 ) ) ;
#23675=CARTESIAN_POINT ( 'NONE',  ( 78.22442621354822734, 61.78027394037003006, 15.74819469288706664 ) ) ;
#23676=CARTESIAN_POINT ( 'NONE',  ( 73.34339640511194602, 69.67785411864186074, -9.916893174164222557 ) ) ;
#23677=CARTESIAN_POINT ( 'NONE',  ( 70.72288414528865985, 60.52409755963705607, -14.67628891625416898 ) ) ;
#23678=CARTESIAN_POINT ( 'NONE',  ( 72.22334018239831721, 71.90115885523906059, -3.839516039074286180 ) ) ;
#23687=CARTESIAN_POINT ( 'NONE',  ( 88.28323348104321155, 43.74655523625713016, 0.1991997974169889829 ) ) ;
#23688=CARTESIAN_POINT ( 'NONE',  ( 6.499975723459110455, 22.49103043416547010, -8.090169943749479842 ) ) ;
#23693=CARTESIAN_POINT ( 'NONE',  ( 28.62558104116610380, 25.03085787977764198, 9.188101187500006262 ) ) ;
#23697=CARTESIAN_POINT ( 'NONE',  ( 10.75418485208671981, 27.18502408145590010, 5.678558825948277544 ) ) ;
#23699=FACE_OUTER_BOUND ( 'NONE', #71889, .T. ) ;
#23700=CARTESIAN_POINT ( 'NONE',  ( 82.83132155253177586, 53.79349055486937203, -15.41265137785383921 ) ) ;
#23702=CARTESIAN_POINT ( 'NONE',  ( 74.05718643579534444, 66.92064597331267350, 12.30401845754858137 ) ) ;
#23704=EDGE_CURVE ( 'NONE', #52768, #48577, #26514, .T. ) ;
#23711=CARTESIAN_POINT ( 'NONE',  ( 77.08943580307069965, 49.61595851756826647, 15.51385819011977674 ) ) ;
#23721=CARTESIAN_POINT ( 'NONE',  ( 66.00797677831485544, 69.09111565677241629, -2.045358714672447231 ) ) ;
#23726=CARTESIAN_POINT ( 'NONE',  ( 31.32709252658613508, 23.80170272979928114, 7.433330006724137462 ) ) ;
#23727=CARTESIAN_POINT ( 'NONE',  ( 79.96799371511821164, 44.53225917763541020, 11.71816028160813161 ) ) ;
#23729=CARTESIAN_POINT ( 'NONE',  ( 75.02238714290075450, 66.92454316053134278, -13.18498694845918884 ) ) ;
#23730=EDGE_CURVE ( 'NONE', #54490, #83325, #34909, .T. ) ;
#23731=VERTEX_POINT ( 'NONE', #28463 ) ;
#23738=CARTESIAN_POINT ( 'NONE',  ( 68.16602257681624621, 65.65656189039059143, -10.28278815586033623 ) ) ;
#23739=B_SPLINE_CURVE_WITH_KNOTS ( 'NONE', 3,
 ( #37290, #82467, #14002, #14503, #13028, #44881, #75821, #91041, #60574, #76316, #29697, #90555, #52002, #20120, #44386, #75321, #6408, #97151, #91530, #52991, #83940, #6890, #66212, #27717, #58585, #50991, #81941, #12519, #43391, #77813, #92529, #93530, #8396 ),
 .UNSPECIFIED., .F., .F.,
 ( 4, 2, 2, 2, 1, 2, 2, 1, 1, 2, 2, 2, 2, 1, 1, 2, 2, 2, 4 ),
 ( 0.000000000000000000, 0.09685993190008025666, 0.1210749148751011778, 0.1452898978501221128, 0.1937198638001665085, 0.2421498297502108765, 0.2542573212377213232, 0.2663648127252317699, 0.2905797957002522747, 0.3390097616502959488, 0.3874397276003396229, 0.4842996595004269156, 0.5085146424754509731, 0.5327296254504749751, 0.5811595914005229790, 0.6053745743755458708, 0.6295895573505686516, 0.6780195233006141020, 0.7748794552007052250 ),
 .UNSPECIFIED. ) ;
#23750=CARTESIAN_POINT ( 'NONE',  ( 77.94354854059760385, 61.39700473696555605, -16.15480247637162847 ) ) ;
#23758=CARTESIAN_POINT ( 'NONE',  ( 66.64069086730589220, 67.52642362728826697, 6.398950582977087187 ) ) ;
#23762=CARTESIAN_POINT ( 'NONE',  ( 81.27629932712225980, 55.76935796986149541, 16.38776540150240990 ) ) ;
#23763=CARTESIAN_POINT ( 'NONE',  ( 85.51568253422234989, 47.12103425145187430, -10.62146421753836201 ) ) ;
#23769=CARTESIAN_POINT ( 'NONE',  ( 21.79139015901366250, 20.78052372038640527, -10.00000000000000355 ) ) ;
#23773=CARTESIAN_POINT ( 'NONE',  ( 88.06269261788008862, 43.61796610520790551, 0.05835779599787207367 ) ) ;
#23775=B_SPLINE_CURVE_WITH_KNOTS ( 'NONE', 3,
 ( #77035, #7641, #25863, #81958, #56230, #2055, #26353, #32448, #66710, #86203 ),
 .UNSPECIFIED., .F., .F.,
 ( 4, 2, 2, 2, 4 ),
 ( 0.000000000000000000, 0.2500000000000000000, 0.5000000000000000000, 0.7500000000000000000, 1.000000000000000000 ),
 .UNSPECIFIED. ) ;
#23776=CARTESIAN_POINT ( 'NONE',  ( 76.27001746108665259, 64.92218695046919663, -14.30664744964449753 ) ) ;
#23778=EDGE_CURVE ( 'NONE', #14203, #15032, #29183, .T. ) ;
#23786=CARTESIAN_POINT ( 'NONE',  ( 34.73240388683179702, 38.79103043416552765, 8.090169943749478065 ) ) ;
#23790=CARTESIAN_POINT ( 'NONE',  ( 70.49967271327585649, 67.34638213932271356, -9.999908609504970514 ) ) ;
#23791=ORIENTED_EDGE ( 'NONE', *, *, #70279, .F. ) ;
#23796=CARTESIAN_POINT ( 'NONE',  ( 83.58408646423136190, 52.36411970034374974, 14.77742527876824141 ) ) ;
#23802=FACE_BOUND ( 'NONE', #91325, .T. ) ;
#23805=CARTESIAN_POINT ( 'NONE',  ( 26.65225264301594166, 37.16126292948896293, -6.180339887498951690 ) ) ;
#23819=CARTESIAN_POINT ( 'NONE',  ( 26.40327033588000205, 37.01751292744058475, 6.180339887498949913 ) ) ;
#23820=CARTESIAN_POINT ( 'NONE',  ( 78.25846697678839803, 59.65309229871257202, 16.47561015943145435 ) ) ;
#23824=LINE ( 'NONE', #86198, #29058 ) ;
#23831=CARTESIAN_POINT ( 'NONE',  ( 72.69903869004953378, 70.24355232890721368, -8.744048261473219341 ) ) ;
#23832=CARTESIAN_POINT ( 'NONE',  ( 27.81076257310190769, 39.55466486950702176, 7.012934429366973338E-14 ) ) ;
#23840=CARTESIAN_POINT ( 'NONE',  ( 21.52536902826200915, 24.37878583063841376, 9.188101187500006262 ) ) ;
#23844=CARTESIAN_POINT ( 'NONE',  ( 6.244247187202517146, 25.64646525600388216, -2.839279412974133887 ) ) ;
#23847=CARTESIAN_POINT ( 'NONE',  ( 75.31289280903088468, 53.62176160569084260, -16.53289957306499858 ) ) ;
#23848=CARTESIAN_POINT ( 'NONE',  ( 71.22567098774472072, 60.39832601874510942, -14.84358665764284524 ) ) ;
#23850=EDGE_CURVE ( 'NONE', #11388, #62487, #84490, .T. ) ;
#23851=ORIENTED_EDGE ( 'NONE', *, *, #23012, .T. ) ;
#23854=CARTESIAN_POINT ( 'NONE',  ( 85.62087432442550039, 48.96184342359305219, 12.19155329030992618 ) ) ;
#23860=CARTESIAN_POINT ( 'NONE',  ( 68.78996647874213011, 70.77593301599395659, 1.606320726995938530 ) ) ;
#23861=CARTESIAN_POINT ( 'NONE',  ( 84.33518316974296170, 42.63392823952606392, -4.290652948369976905 ) ) ;
#23864=CARTESIAN_POINT ( 'NONE',  ( 71.87942950353104266, 72.15877716270880171, -3.647418342425857052 ) ) ;
#23865=CARTESIAN_POINT ( 'NONE',  ( 72.76771589847461996, 57.00350618467320629, -16.39718444356080695 ) ) ;
#23866=CARTESIAN_POINT ( 'NONE',  ( 76.65872121159138430, 63.56238613867309795, 15.33801735844474834 ) ) ;
#23870=LINE ( 'NONE', #39553, #25598 ) ;
#23873=CARTESIAN_POINT ( 'NONE',  ( 29.59504171901726366, 22.80170272979927759, 7.433330006724137462 ) ) ;
#23878=CARTESIAN_POINT ( 'NONE',  ( 26.66754231763712824, 34.13478043621389446, 8.090169943749478065 ) ) ;
#23880=CARTESIAN_POINT ( 'NONE',  ( 83.82827945288542537, 51.88092520783234818, 14.50189114860043205 ) ) ;
#23882=EDGE_LOOP ( 'NONE', ( #61354, #502, #52545, #5231 ) ) ;
#23887=VECTOR ( 'NONE', #98622, 1000.000000000000114 ) ;
#23888=ORIENTED_EDGE ( 'NONE', *, *, #23271, .F. ) ;
#23899=CARTESIAN_POINT ( 'NONE',  ( 69.39138836530793242, 65.59840692806227480, -11.05004714553397704 ) ) ;
#23900=CARTESIAN_POINT ( 'NONE',  ( 78.75297625648194355, 47.66336229242892131, 14.29739783554173727 ) ) ;
#23904=CARTESIAN_POINT ( 'NONE',  ( 70.04767293653641502, 64.67844632371958369, 12.15646808155997860 ) ) ;
#23906=CARTESIAN_POINT ( 'NONE',  ( 87.43197870664040749, 44.84778077074484770, -6.629285647492168643 ) ) ;
#23910=CARTESIAN_POINT ( 'NONE',  ( 83.51092623577891061, 51.50185674319119045, -14.43088262691037293 ) ) ;
#23911=CARTESIAN_POINT ( 'NONE',  ( 87.53583079710631409, 45.45925790797146249, -6.823327534849023657 ) ) ;
#23915=DIRECTION ( 'NONE',  ( 0.5000000000000013323, -0.8660254037844378194, 0.000000000000000000 ) ) ;
#23916=CARTESIAN_POINT ( 'NONE',  ( 74.65263117529048031, 66.98225998262294922, 13.00178404275292721 ) ) ;
#23923=CARTESIAN_POINT ( 'NONE',  ( 85.48848937474792820, 48.32878387211594884, -12.22513733614604270 ) ) ;
#23925=CARTESIAN_POINT ( 'NONE',  ( 72.31093312958903141, 67.42550271943373730, 11.03266209124485897 ) ) ;
#23927=CARTESIAN_POINT ( 'NONE',  ( 72.73869357531808078, 58.37704337636537133, 16.17108310384250203 ) ) ;
#23929=CARTESIAN_POINT ( 'NONE',  ( 82.29666020798650550, 41.51490518991582945, -5.842944381793243380 ) ) ;
#23932=( GEOMETRIC_REPRESENTATION_CONTEXT ( 3 ) GLOBAL_UNCERTAINTY_ASSIGNED_CONTEXT ( ( #64563 ) ) GLOBAL_UNIT_ASSIGNED_CONTEXT ( ( #13615, #67806, #83544 ) ) REPRESENTATION_CONTEXT ( 'NONE', 'WORKASPACE' ) );
#23935=EDGE_LOOP ( 'NONE', ( #13557, #26546, #36423, #46437 ) ) ;
#23940=CARTESIAN_POINT ( 'NONE',  ( 11.86377311551791358, 18.80066082961420548, 10.00000000000000533 ) ) ;
#23941=DIRECTION ( 'NONE',  ( 0.2033683215378999376, -0.3522442655536480172, -0.9135454576426004225 ) ) ;
#23942=CARTESIAN_POINT ( 'NONE',  ( 71.88281838924127953, 59.56282477450883306, -15.74156321312328011 ) ) ;
#23944=CARTESIAN_POINT ( 'NONE',  ( 10.37514450368026786, 11.15404122711131407, 8.090169943749479842 ) ) ;
#23949=CARTESIAN_POINT ( 'NONE',  ( 70.47412699110996925, 67.85741242599571876, 10.12516759932945476 ) ) ;
#23950=CARTESIAN_POINT ( 'NONE',  ( 14.86318692873816083, 16.78052372038639106, -10.00000000000000355 ) ) ;
#23951=ORIENTED_EDGE ( 'NONE', *, *, #410, .F. ) ;
#23957=CARTESIAN_POINT ( 'NONE',  ( 35.22599450741489591, 22.19860640527294393, 2.839279412974134775 ) ) ;
#23963=CARTESIAN_POINT ( 'NONE',  ( 88.01292981757310940, 43.79437901572623559, 2.423352920943459665 ) ) ;
#23964=CARTESIAN_POINT ( 'NONE',  ( 66.37106933066878867, 68.69559461379999732, 2.357535188532553505 ) ) ;
#23968=AXIS2_PLACEMENT_3D ( 'NONE', #5736, #98461, #29540 ) ;
#23971=CARTESIAN_POINT ( 'NONE',  ( 15.97197434310064423, 12.14754757982088940, -5.678558825948275768 ) ) ;
#23977=CARTESIAN_POINT ( 'NONE',  ( 23.75126848931443746, 37.21091486745861943, 7.012934429366973338E-14 ) ) ;
#23983=ORIENTED_EDGE ( 'NONE', *, *, #3580, .F. ) ;
#23984=ORIENTED_EDGE ( 'NONE', *, *, #24872, .T. ) ;
#23988=CARTESIAN_POINT ( 'NONE',  ( 26.59681983377653580, 15.75978393459164728, -1.583844403245362020 ) ) ;
#23990=ORIENTED_EDGE ( 'NONE', *, *, #66881, .T. ) ;
#23991=CARTESIAN_POINT ( 'NONE',  ( 68.83006821756048055, 63.80255091578027304, -12.25988136761327496 ) ) ;
#23992=CARTESIAN_POINT ( 'NONE',  ( 79.30872066878571047, 59.07782615681725957, -16.22658500882148758 ) ) ;
#23995=CARTESIAN_POINT ( 'NONE',  ( 69.68564319292937626, 62.66806819657130490, 13.90549188088030164 ) ) ;
#23999=CARTESIAN_POINT ( 'NONE',  ( 71.41016749218992743, 59.45273978182970609, 15.69346469599747174 ) ) ;
#24001=VERTEX_POINT ( 'NONE', #91094 ) ;
#24007=CARTESIAN_POINT ( 'NONE',  ( 70.99127280270764118, 71.57001342661881438, 1.849139882998378059 ) ) ;
#24013=CARTESIAN_POINT ( 'NONE',  ( 81.74295896583093679, 45.02925702631734595, 10.54780463062767915 ) ) ;
#24018=CARTESIAN_POINT ( 'NONE',  ( 81.01234624326276901, 54.88323349113267113, -16.28327499330496053 ) ) ;
#24019=CARTESIAN_POINT ( 'NONE',  ( 19.25324864145614612, 26.51421378149919761, -9.188101187500004485 ) ) ;
#24020=AXIS2_PLACEMENT_3D ( 'NONE', #89650, #90652, #44981 ) ;
#24022=CARTESIAN_POINT ( 'NONE',  ( 80.17048798456011127, 57.79824262504150312, 16.60278798193532879 ) ) ;
#24024=ORIENTED_EDGE ( 'NONE', *, *, #21767, .F. ) ;
#24028=CARTESIAN_POINT ( 'NONE',  ( 84.71308721041314982, 45.64921926619080494, -9.416152049834934701 ) ) ;
#24031=ORIENTED_EDGE ( 'NONE', *, *, #42814, .F. ) ;
#24033=CARTESIAN_POINT ( 'NONE',  ( 74.67000616351420206, 66.81477949400924388, -13.12245706047550797 ) ) ;
#24039=CARTESIAN_POINT ( 'NONE',  ( 82.41720788485099547, 40.42146991629093833, -1.345722392452352034 ) ) ;
#24040=VECTOR ( 'NONE', #48662, 1000.000000000000114 ) ;
#24043=VECTOR ( 'NONE', #57147, 999.9999999999998863 ) ;
#24047=CARTESIAN_POINT ( 'NONE',  ( 75.75395351785276432, 65.60989001837319279, 13.81304751500886496 ) ) ;
#24050=VECTOR ( 'NONE', #44044, 1000.000000000000000 ) ;
#24051=ORIENTED_EDGE ( 'NONE', *, *, #98837, .T. ) ;
#24054=CARTESIAN_POINT ( 'NONE',  ( 85.12840156634364064, 46.10501368961206481, -9.731286439397152321 ) ) ;
#24055=CARTESIAN_POINT ( 'NONE',  ( 84.72382484348065645, 44.74833322614003350, 8.228402119231732925 ) ) ;
#24057=AXIS2_PLACEMENT_3D ( 'NONE', #100119, #61584, #39762 ) ;
#24058=CARTESIAN_POINT ( 'NONE',  ( 83.20066689603021359, 44.07261036406099919, 8.458864577965798048 ) ) ;
#24059=CARTESIAN_POINT ( 'NONE',  ( 74.44819773037836796, 68.07767128628745468, -11.61919445340353185 ) ) ;
#24063=CARTESIAN_POINT ( 'NONE',  ( 74.62401959271109320, 66.89443057110611335, 13.05059976691391199 ) ) ;
#24066=CARTESIAN_POINT ( 'NONE',  ( 32.57180473799247977, 34.50829794293882458, -10.00000000000000355 ) ) ;
#24072=CARTESIAN_POINT ( 'NONE',  ( 71.43227217437114973, 62.73058494111581496, 14.40807302911904486 ) ) ;
#24074=CARTESIAN_POINT ( 'NONE',  ( 35.87562414229657293, 44.21091486745863364, 7.012934429366973338E-14 ) ) ;
#24078=ORIENTED_EDGE ( 'NONE', *, *, #77782, .T. ) ;
#24082=CARTESIAN_POINT ( 'NONE',  ( 19.63753723929501760, 13.19860640527291551, 2.839279412974134775 ) ) ;
#24084=CARTESIAN_POINT ( 'NONE',  ( 78.91767422429964540, 57.25042157409582444, -16.60633881229267672 ) ) ;
#24093=ORIENTED_EDGE ( 'NONE', *, *, #65244, .F. ) ;
#24099=CARTESIAN_POINT ( 'NONE',  ( 75.79167905567804553, 65.12415201610325255, -14.46789148266619485 ) ) ;
#24102=DIRECTION ( 'NONE',  ( 0.5000000000000013323, -0.8660254037844378194, 0.000000000000000000 ) ) ;
#24103=CARTESIAN_POINT ( 'NONE',  ( 75.03965799331250253, 52.98571459348521273, -16.01149241364986153 ) ) ;
#24108=VECTOR ( 'NONE', #71284, 1000.000000000000000 ) ;
#24109=CARTESIAN_POINT ( 'NONE',  ( 33.58239374649102871, 42.49540643055189548, 3.479690158560446702E-15 ) ) ;
#24116=AXIS2_PLACEMENT_3D ( 'NONE', #2926, #80445, #87063 ) ;
#24117=CARTESIAN_POINT ( 'NONE',  ( 86.55657754374946933, 47.30628205130771136, -10.74852006680812089 ) ) ;
#24118=DIRECTION ( 'NONE',  ( 0.4635919272833914917, -0.8029647720336136052, 0.3746065934159158450 ) ) ;
#24124=CARTESIAN_POINT ( 'NONE',  ( 82.36604948993920061, 45.22791889282441957, -11.08805331368615832 ) ) ;
#24125=CARTESIAN_POINT ( 'NONE',  ( 80.26965983545827044, 44.82647928622098021, 11.14148114410500412 ) ) ;
#24127=ORIENTED_EDGE ( 'NONE', *, *, #18180, .F. ) ;
#24131=CARTESIAN_POINT ( 'NONE',  ( 77.31232694779509984, 49.13200894661118667, -15.30069998651773311 ) ) ;
#24132=VERTEX_POINT ( 'NONE', #98684 ) ;
#24135=CARTESIAN_POINT ( 'NONE',  ( 79.40743318721024480, 54.34964698095226510, 15.92978307125684445 ) ) ;
#24136=( BOUNDED_CURVE ( )  B_SPLINE_CURVE ( 2, ( #15163, #30884, #68869, #83629, #99797, #23769, #45078, #61770, #99303, #36979, #92717, #15670, #77500 ),
 .UNSPECIFIED., .F., .T. ) 
 B_SPLINE_CURVE_WITH_KNOTS ( ( 3, 2, 2, 2, 2, 2, 3 ),
 ( 0.3875000000000000111, 0.3900000000000000133, 0.3950000000000000178, 0.4000000000000000222, 0.4050000000000000266, 0.4099999999999999756, 0.4124999999999999778 ),
 .UNSPECIFIED. ) 
 CURVE ( )  GEOMETRIC_REPRESENTATION_ITEM ( )  RATIONAL_B_SPLINE_CURVE ( ( 0.9755282581475768211, 0.9755282581475768211, 1.000000000000000000, 0.9510565162951535312, 1.000000000000000000, 0.9510565162951535312, 1.000000000000000000, 0.9510565162951535312, 1.000000000000000000, 0.9510565162951535312, 1.000000000000000000, 0.9755282581475768211, 0.9755282581475768211 ) ) 
 REPRESENTATION_ITEM ( '' )  );
#24142=CARTESIAN_POINT ( 'NONE',  ( 82.61013673858765571, 40.49722781981445507, 0.8877010427639511203 ) ) ;
#24147=CARTESIAN_POINT ( 'NONE',  ( 70.55887007047591908, 60.82933938485357572, -15.03632500835287189 ) ) ;
#24148=CARTESIAN_POINT ( 'NONE',  ( 35.68911091587340678, 42.64646525600393545, -2.839279412974133887 ) ) ;
#24151=CARTESIAN_POINT ( 'NONE',  ( 85.53835401965352503, 48.98340217412621911, -12.70221784291844180 ) ) ;
#24158=CARTESIAN_POINT ( 'NONE',  ( 80.74974841587442143, 43.27611110060701805, 10.01619596027649095 ) ) ;
#24162=VERTEX_POINT ( 'NONE', #76373 ) ;
#24166=DIRECTION ( 'NONE',  ( -0.5000000000000013323, 0.8660254037844379305, 0.000000000000000000 ) ) ;
#24184=CARTESIAN_POINT ( 'NONE',  ( 73.79815732168846409, 68.46225211080071915, 11.43730676814644553 ) ) ;
#24185=CARTESIAN_POINT ( 'NONE',  ( 74.35881753926216220, 68.47570456641908265, 11.21376435697400709 ) ) ;
#24193=CARTESIAN_POINT ( 'NONE',  ( 78.12501046422360673, 47.63414727997927400, 14.46436878840962059 ) ) ;
#24195=CARTESIAN_POINT ( 'NONE',  ( 77.86187795391879263, 53.88640785478639117, 15.96271232416930630 ) ) ;
#24197=CARTESIAN_POINT ( 'NONE',  ( 78.30955769916531040, 61.43963167811126169, 15.82323565659766373 ) ) ;
#24199=CARTESIAN_POINT ( 'NONE',  ( 76.32610495235408621, 51.38149014994888830, 15.62204473798428239 ) ) ;
#24203=B_SPLINE_CURVE_WITH_KNOTS ( 'NONE', 3,
 ( #25627, #2334, #33735, #55006, #72240, #87984, #48926, #86478, #55493, #72752, #40295, #64626, #1328, #62598, #93552, #17006 ),
 .UNSPECIFIED., .F., .F.,
 ( 4, 1, 2, 2, 2, 1, 2, 2, 4 ),
 ( 0.000000000000000000, 0.1250000000000016653, 0.1875000000000024980, 0.2500000000000033307, 0.5000000000000043299, 0.6250000000000048850, 0.6875000000000051070, 0.7500000000000054401, 1.000000000000000000 ),
 .UNSPECIFIED. ) ;
#24206=CARTESIAN_POINT ( 'NONE',  ( 72.69815669700709293, 57.09302316489889506, -15.89630389596367799 ) ) ;
#24211=FACE_OUTER_BOUND ( 'NONE', #31251, .T. ) ;
#24214=CARTESIAN_POINT ( 'NONE',  ( 71.80779569229208903, 72.11915028389421423, -3.640749997624285417 ) ) ;
#24215=CARTESIAN_POINT ( 'NONE',  ( 77.08943580299947484, 49.61595851769168064, 15.51385818994994459 ) ) ;
#24217=VECTOR ( 'NONE', #16502, 1000.000000000000114 ) ;
#24218=CARTESIAN_POINT ( 'NONE',  ( 21.78279761992806129, 35.68290643055188838, 3.479690158560446702E-15 ) ) ;
#24221=CARTESIAN_POINT ( 'NONE',  ( 18.45335787429653607, 11.44966523072493558, -2.296566073217252530E-15 ) ) ;
#24223=CARTESIAN_POINT ( 'NONE',  ( 76.81877415327811320, 63.87294231776800757, 14.88723717811692282 ) ) ;
#24234=CARTESIAN_POINT ( 'NONE',  ( 77.58396476582734635, 49.27429002014808646, 15.29533474293770823 ) ) ;
#24239=CARTESIAN_POINT ( 'NONE',  ( 70.34943318750055141, 68.90035037863729883, -7.849331805225474135 ) ) ;
#24240=ADVANCED_FACE ( 'NONE', ( #69738 ), #32699, .T. ) ;
#24244=CARTESIAN_POINT ( 'NONE',  ( 66.15980552222140432, 69.17909379384724389, -2.043126084711875734 ) ) ;
#24248=CARTESIAN_POINT ( 'NONE',  ( 31.84670776885679899, 24.10170272979928541, -7.433330006724141015 ) ) ;
#24250=FACE_OUTER_BOUND ( 'NONE', #78576, .T. ) ;
#24255=EDGE_LOOP ( 'NONE', ( #22823, #64375, #78127, #25294 ) ) ;
#24257=CARTESIAN_POINT ( 'NONE',  ( 67.94506607690384214, 65.68283619601920975, 10.86420754080536355 ) ) ;
#24258=CARTESIAN_POINT ( 'NONE',  ( 67.99955159661209336, 66.07893017027207350, -10.48801018483890068 ) ) ;
#24264=AXIS2_PLACEMENT_3D ( 'NONE', #10450, #41324, #18559 ) ;
#24275=ORIENTED_EDGE ( 'NONE', *, *, #35995, .F. ) ;
#24276=CARTESIAN_POINT ( 'NONE',  ( 79.92051602943618605, 44.51830849947365465, -11.04832637642992132 ) ) ;
#24279=CARTESIAN_POINT ( 'NONE',  ( 80.97096062864531518, 55.95811706980097000, 16.09172280808637012 ) ) ;
#24280=CARTESIAN_POINT ( 'NONE',  ( 79.30706684625435798, 48.64070561785491265, -14.10287111613649635 ) ) ;
#24284=VECTOR ( 'NONE', #22076, 1000.000000000000114 ) ;
#24286=B_SPLINE_SURFACE_WITH_KNOTS ( 'NONE', 3, 1, ( 
 ( #52836, #21941 ),
 ( #68537, #82799 ),
 ( #21451, #13368 ),
 ( #44232, #44725 ),
 ( #83280, #6243 ),
 ( #98471, #5257 ),
 ( #91889, #75170 ),
 ( #29064, #99460 ),
 ( #89893, #30038 ),
 ( #52339, #74683 ),
 ( #59931, #83786 ),
 ( #36139, #90901 ),
 ( #82309, #45723 ),
 ( #53335, #68043 ),
 ( #22441, #98965 ),
 ( #60925, #45236 ),
 ( #29548, #14348 ),
 ( #35654, #66553 ),
 ( #51343, #67041 ),
 ( #97965, #28541 ),
 ( #90402, #20977 ),
 ( #51859, #39114 ),
 ( #31523, #61921 ),
 ( #69538, #84780 ),
 ( #8740, #39611 ),
 ( #62416, #146 ),
 ( #55319, #86798 ),
 ( #1659, #92870 ),
 ( #99960, #93377 ),
 ( #23929, #8249 ),
 ( #55805, #24931 ) ),
 .UNSPECIFIED., .F., .F., .F.,
 ( 4, 3, 3, 3, 3, 3, 3, 3, 3, 3, 4 ),
 ( 2, 2 ),
 ( 0.000000000000000000, 0.1122669598086838000, 0.2243161639709725652, 0.3396355846219227259, 0.4553962076585201801, 0.5677860799922432866, 0.6749047109689664259, 0.7773884377078287278, 0.8775581155834328850, 0.9782364162377897854, 1.000000000000000000 ),
 ( 0.000000000000000000, 1.000000000000000000 ),
 .UNSPECIFIED. ) ;
#24291=CARTESIAN_POINT ( 'NONE',  ( 19.19489604512981984, 34.58029201028041655, 1.583844403245397769 ) ) ;
#24292=EDGE_CURVE ( 'NONE', #35343, #31579, #39550, .T. ) ;
#24295=CARTESIAN_POINT ( 'NONE',  ( 87.86895504114028199, 44.78688104239807188, 4.940966480777958303 ) ) ;
#24303=CARTESIAN_POINT ( 'NONE',  ( 72.50911665321707744, 70.64777112744620524, 7.215784761677396908 ) ) ;
#24305=ORIENTED_EDGE ( 'NONE', *, *, #15980, .T. ) ;
#24308=DIRECTION ( 'NONE',  ( 0.5000000000000013323, -0.8660254037844378194, 0.000000000000000000 ) ) ;
#24310=CARTESIAN_POINT ( 'NONE',  ( 83.85749844460281111, 51.92724282576335071, 14.91256361652490092 ) ) ;
#24311=EDGE_CURVE ( 'NONE', #11459, #71854, #40821, .T. ) ;
#24317=CARTESIAN_POINT ( 'NONE',  ( 73.67565831133079257, 55.36794421709517167, 16.58968170789317398 ) ) ;
#24319=CARTESIAN_POINT ( 'NONE',  ( 32.00589586780220941, 18.28848085856232331, 1.475505719884397138E-15 ) ) ;
#24334=CARTESIAN_POINT ( 'NONE',  ( 24.67121952831112353, 36.01751292744057764, 6.180339887498949913 ) ) ;
#24335=CARTESIAN_POINT ( 'NONE',  ( 82.28514220754047415, 41.58448466926779474, -4.581006405137011406 ) ) ;
#24337=CARTESIAN_POINT ( 'NONE',  ( 81.66701081066987911, 55.79068320882007725, 16.00012122222618771 ) ) ;
#24338=ADVANCED_FACE ( 'NONE', ( #75255 ), #47986, .T. ) ;
#24343=EDGE_CURVE ( 'NONE', #99018, #33772, #46945, .T. ) ;
#24345=CARTESIAN_POINT ( 'NONE',  ( 71.57492018021982005, 66.57275065399230130, -11.35834070733682744 ) ) ;
#24353=DIRECTION ( 'NONE',  ( 0.1378186779084994706, -0.2387089523694924387, -0.9612616959383186721 ) ) ;
#24358=CARTESIAN_POINT ( 'NONE',  ( 26.03951966209473312, 17.96004757982090538, -5.678558825948276656 ) ) ;
#24363=CARTESIAN_POINT ( 'NONE',  ( 13.40518456965460281, 16.24335787977761925, -9.188101187500008038 ) ) ;
#24367=CARTESIAN_POINT ( 'NONE',  ( 71.81881128194709163, 72.53313204687133009, -1.300380427722385823 ) ) ;
#24368=ORIENTED_EDGE ( 'NONE', *, *, #55451, .F. ) ;
#24370=CARTESIAN_POINT ( 'NONE',  ( 70.36952472774478906, 71.02280663496645730, -2.695929215683882774 ) ) ;
#24376=CARTESIAN_POINT ( 'NONE',  ( 86.68781752468889579, 43.33485113087137819, -1.416241137521898619 ) ) ;
#24378=CARTESIAN_POINT ( 'NONE',  ( 66.10978050773523762, 68.50388961278160593, -2.614487067079704907 ) ) ;
#24380=CARTESIAN_POINT ( 'NONE',  ( 80.12283971196008281, 57.76720862780119603, 16.60271659255639776 ) ) ;
#24381=CARTESIAN_POINT ( 'NONE',  ( 7.533646096595723485, 16.30066082961419482, -10.00000000000000533 ) ) ;
#24385=CYLINDRICAL_SURFACE ( 'NONE', #61155, 16.60714546451156792 ) ;
#24388=CARTESIAN_POINT ( 'NONE',  ( 25.67147243227365294, 35.79752408145593989, -5.678558825948271327 ) ) ;
#24393=CARTESIAN_POINT ( 'NONE',  ( 74.38015889281619764, 68.44084013566667579, 11.25477996513194867 ) ) ;
#24396=CARTESIAN_POINT ( 'NONE',  ( 80.93613592869992601, 42.95327845849681836, -9.503115154567232992 ) ) ;
#24398=CARTESIAN_POINT ( 'NONE',  ( 87.09272086398131307, 46.41253043617862062, 8.753911316151357980 ) ) ;
#24400=CARTESIAN_POINT ( 'NONE',  ( 78.02511763684471191, 53.60668594641142448, 16.35104529020703623 ) ) ;
#24401=ORIENTED_EDGE ( 'NONE', *, *, #33686, .T. ) ;
#24407=CARTESIAN_POINT ( 'NONE',  ( 83.67416965427615594, 41.61942911856458949, 0.1873010706438003881 ) ) ;
#24410=CARTESIAN_POINT ( 'NONE',  ( 67.51011536099680654, 66.65123204117807632, 8.646292631228400083 ) ) ;
#24414=ORIENTED_EDGE ( 'NONE', *, *, #31289, .T. ) ;
#24416=CARTESIAN_POINT ( 'NONE',  ( 69.82278528426677155, 64.04957407583405882, 12.51083613146919227 ) ) ;
#24420=CARTESIAN_POINT ( 'NONE',  ( 83.63562430374231838, 51.63275018564552710, -14.84107497619760174 ) ) ;
#24424=CARTESIAN_POINT ( 'NONE',  ( 80.42443749358989180, 57.88788176714987799, -16.24735605553297191 ) ) ;
#24435=CARTESIAN_POINT ( 'NONE',  ( 85.64890296506385425, 48.36409154393287224, -11.71277604259690541 ) ) ;
#24437=CARTESIAN_POINT ( 'NONE',  ( 72.06403648541707696, 66.67572987517343108, 11.55341923834466833 ) ) ;
#24439=EDGE_CURVE ( 'NONE', #35211, #2161, #62523, .T. ) ;
#24446=CARTESIAN_POINT ( 'NONE',  ( 45.44687632901609931, 27.20801979619932709, -3.090169943749474069 ) ) ;
#24450=CARTESIAN_POINT ( 'NONE',  ( 16.96546585850747491, 10.76426979415088603, 3.090169943749476733 ) ) ;
#24451=CARTESIAN_POINT ( 'NONE',  ( 77.13473189285724629, 50.76288165847083178, -15.86405702230585213 ) ) ;
#24453=CARTESIAN_POINT ( 'NONE',  ( 71.81468377527440339, 71.89775840070207380, 2.890995686414929544 ) ) ;
#24456=CARTESIAN_POINT ( 'NONE',  ( 5.363317384539951327, 21.83478043621385822, -8.090169943749479842 ) ) ;
#24467=CARTESIAN_POINT ( 'NONE',  ( 29.36891313204580456, 35.14336893147757479, 7.433330006724141015 ) ) ;
#24473=CARTESIAN_POINT ( 'NONE',  ( 66.23268198520062811, 69.13923810758623745, 2.551101940990796901 ) ) ;
#24476=CARTESIAN_POINT ( 'NONE',  ( 3.154811933878272523, 22.79752408145590081, -5.678558825948271327 ) ) ;
#24478=CARTESIAN_POINT ( 'NONE',  ( 13.18987451683679524, 19.56628583063839244, 9.188101187500006262 ) ) ;
#24489=VERTEX_POINT ( 'NONE', #7321 ) ;
#24491=CARTESIAN_POINT ( 'NONE',  ( 72.83836408177631938, 70.83590621374696639, 7.219044590757257573 ) ) ;
#24494=DIRECTION ( 'NONE',  ( -1.000000000000000000, 0.000000000000000000, 0.000000000000000000 ) ) ;
#24497=CARTESIAN_POINT ( 'NONE',  ( 79.28302063466352934, 59.54490948036853126, -16.53220260971269795 ) ) ;
#24499=CARTESIAN_POINT ( 'NONE',  ( 10.53464200728543254, 29.58029201028040944, 1.583844403245363353 ) ) ;
#24505=ORIENTED_EDGE ( 'NONE', *, *, #37368, .F. ) ;
#24508=CARTESIAN_POINT ( 'NONE',  ( 80.05911005159690319, 45.70205177477036074, 12.00129917442164285 ) ) ;
#24510=DIRECTION ( 'NONE',  ( 0.000000000000000000, -0.6050222638427519284, -0.7962085532412920275 ) ) ;
#24513=CARTESIAN_POINT ( 'NONE',  ( 81.98024531596684028, 45.55728866792462384, 10.93523696988690830 ) ) ;
#24516=EDGE_CURVE ( 'NONE', #7077, #82637, #57919, .T. ) ;
#24518=CARTESIAN_POINT ( 'NONE',  ( 82.66149664020484522, 53.53843108144140928, -15.73363621927587097 ) ) ;
#24521=CARTESIAN_POINT ( 'NONE',  ( 21.52536902826200915, 24.37878583063841376, 9.188101187500006262 ) ) ;
#24531=CYLINDRICAL_SURFACE ( 'NONE', #45029, 10.00000000000001066 ) ;
#24534=CARTESIAN_POINT ( 'NONE',  ( 74.98927683103343611, 66.88159155676943612, -13.20077067326868381 ) ) ;
#24539=CARTESIAN_POINT ( 'NONE',  ( 82.14417565007086353, 40.79354657814926099, -1.097195410270651816 ) ) ;
#24543=CARTESIAN_POINT ( 'NONE',  ( 75.52144112198921277, 65.39696173216708530, 13.85314077474386707 ) ) ;
#24551=EDGE_CURVE ( 'NONE', #47570, #53490, #11842, .T. ) ;
#24552=CARTESIAN_POINT ( 'NONE',  ( 84.86883313302882925, 45.02243900927756215, 8.511842229617958111 ) ) ;
#24555=CARTESIAN_POINT ( 'NONE',  ( 74.34754423757576092, 68.44411287762122242, -11.23027362005041319 ) ) ;
#24558=CARTESIAN_POINT ( 'NONE',  ( 74.81832046901195099, 67.48663194201290594, -12.71244991431774984 ) ) ;
#24560=CARTESIAN_POINT ( 'NONE',  ( 81.52469153597657225, 59.51941083166271795, 0.2499999999999960032 ) ) ;
#24579=CARTESIAN_POINT ( 'NONE',  ( 10.40777469057294091, 26.98502408145591502, -5.678558825948271327 ) ) ;
#24584=CARTESIAN_POINT ( 'NONE',  ( 23.91155070014810136, 29.50829794293881392, -10.00000000000000355 ) ) ;
#24588=CARTESIAN_POINT ( 'NONE',  ( 86.13417129343109480, 47.68469467925804395, 10.84946945994417611 ) ) ;
#24598=CARTESIAN_POINT ( 'NONE',  ( 78.63094854509681397, 48.18467340716805580, 14.04610061905436424 ) ) ;
#24600=DIRECTION ( 'NONE',  ( -0.3213938048432640748, 0.5566703992264119272, -0.7660444431189857850 ) ) ;
#24601=CARTESIAN_POINT ( 'NONE',  ( 74.97683113034595692, 53.08780515268223610, -16.02469623271439048 ) ) ;
#24603=ORIENTED_EDGE ( 'NONE', *, *, #41738, .F. ) ;
#24604=DIRECTION ( 'NONE',  ( 0.7162481363636747922, 0.000000000000000000, 0.6978456900745053648 ) ) ;
#24606=CARTESIAN_POINT ( 'NONE',  ( 40.42517716772906056, 31.84335787977767041, 9.188101187500006262 ) ) ;
#24607=CARTESIAN_POINT ( 'NONE',  ( 83.33965292895494770, 40.89095863664473995, 0.2909840089494764581 ) ) ;
#24613=CARTESIAN_POINT ( 'NONE',  ( 86.26706070573375484, 46.98025876953199287, -10.04304018679821731 ) ) ;
#24623=CARTESIAN_POINT ( 'NONE',  ( 77.25192996872536355, 49.17366000481920452, -15.32849534080991916 ) ) ;
#24626=CARTESIAN_POINT ( 'NONE',  ( 74.95592743341377684, 58.52978105962555588, 15.90320610924748301 ) ) ;
#24627=CARTESIAN_POINT ( 'NONE',  ( 78.35439122558771885, 49.50317310883020383, 14.71240697276643239 ) ) ;
#24634=CARTESIAN_POINT ( 'NONE',  ( 78.87932154437264387, 46.39673357570728029, 12.96173668562228620 ) ) ;
#24642=CARTESIAN_POINT ( 'NONE',  ( 20.33155438404897808, 35.23654200823202132, 1.583844403245397769 ) ) ;
#24648=CARTESIAN_POINT ( 'NONE',  ( 71.74471703213781382, 60.72069063942237221, 14.83967380431143823 ) ) ;
#24663=CARTESIAN_POINT ( 'NONE',  ( 81.13608137687064925, 42.60696278352305200, 7.988320930663086905 ) ) ;
#24668=VERTEX_POINT ( 'NONE', #25015 ) ;
#24672=CARTESIAN_POINT ( 'NONE',  ( 87.85430303351097336, 43.89859490532884223, 0.3596698246726173775 ) ) ;
#24677=CARTESIAN_POINT ( 'NONE',  ( 74.01669459151050035, 68.61891074470059948, 11.40943161386742233 ) ) ;
#24678=CARTESIAN_POINT ( 'NONE',  ( 69.47607923203149483, 70.76119968013694006, -0.4672567883698480751 ) ) ;
#24683=CARTESIAN_POINT ( 'NONE',  ( 88.14071703455390150, 44.55363679567808788, -5.002659464432036351 ) ) ;
#24686=CARTESIAN_POINT ( 'NONE',  ( 78.42360325331485171, 47.41383149739777281, 14.26703730024508054 ) ) ;
#24690=CARTESIAN_POINT ( 'NONE',  ( 76.35458056077806077, 51.11712984296273277, 16.05186526122436064 ) ) ;
#24696=CARTESIAN_POINT ( 'NONE',  ( 72.73719086776743836, 57.26489226207078787, -15.87218763176317537 ) ) ;
#24701=CARTESIAN_POINT ( 'NONE',  ( 88.26944586016423955, 44.13856730148188490, 0.4509010169863623685 ) ) ;
#24704=CARTESIAN_POINT ( 'NONE',  ( 67.65279290918169863, 70.10559244845448745, -1.558233695405924601 ) ) ;
#24706=CARTESIAN_POINT ( 'NONE',  ( 32.17146729527596705, 24.28920272979928541, -7.433330006724141015 ) ) ;
#24708=CARTESIAN_POINT ( 'NONE',  ( 82.49298411987194868, 47.17765150883158753, -12.09122284588559992 ) ) ;
#24709=CARTESIAN_POINT ( 'NONE',  ( 7.290083236948966317, 25.18502408145589655, 5.678558825948277544 ) ) ;
#24711=DIRECTION ( 'NONE',  ( 0.8660254037844377084, 0.5000000000000015543, -0.000000000000000000 ) ) ;
#24716=CARTESIAN_POINT ( 'NONE',  ( 81.85713351507602908, 54.37717625304360070, -15.69185593827182856 ) ) ;
#24722=CARTESIAN_POINT ( 'NONE',  ( 77.45085267822321384, 49.21833083662652086, 15.30297809502122952 ) ) ;
#24727=CARTESIAN_POINT ( 'NONE',  ( 70.42716005707438853, 68.90180154463854478, -7.919248421219340806 ) ) ;
#24731=CARTESIAN_POINT ( 'NONE',  ( 65.86957007823072274, 68.92796865271058948, -2.560965087547883989 ) ) ;
#24736=ORIENTED_EDGE ( 'NONE', *, *, #44896, .T. ) ;
#24737=CARTESIAN_POINT ( 'NONE',  ( 21.59633513308047270, 30.65586893147756697, -7.433330006724137462 ) ) ;
#24738=CARTESIAN_POINT ( 'NONE',  ( 79.85812127980112507, 44.70746904388536791, 11.25005473392974054 ) ) ;
#24740=CARTESIAN_POINT ( 'NONE',  ( 74.98927683103342190, 66.88159155676945034, -13.20077067326868558 ) ) ;
#24741=CARTESIAN_POINT ( 'NONE',  ( 80.92877085092437994, 48.89368045554081021, -13.76466174163450340 ) ) ;
#24743=VERTEX_POINT ( 'NONE', #19460 ) ;
#24748=CARTESIAN_POINT ( 'NONE',  ( 67.77383089997810828, 65.57049627815092663, 10.14032301746840403 ) ) ;
#24749=CARTESIAN_POINT ( 'NONE',  ( 68.33938886113043054, 65.68960829769598320, -10.35387598406562226 ) ) ;
#24750=CARTESIAN_POINT ( 'NONE',  ( 81.71195745382044606, 55.24878511337072950, -15.91731695540261171 ) ) ;
#24757=CARTESIAN_POINT ( 'NONE',  ( 79.01330593081745235, 59.80254073573071594, 16.49416071572547793 ) ) ;
#24761=CARTESIAN_POINT ( 'NONE',  ( 78.15719359349522222, 61.55473184547404486, -16.14768920957587284 ) ) ;
#24769=CARTESIAN_POINT ( 'NONE',  ( 29.53625146412516500, 35.79103043416551344, 8.090169943749478065 ) ) ;
#24777=CARTESIAN_POINT ( 'NONE',  ( 75.65276086696347591, 65.13941327059393416, -14.42100060933655570 ) ) ;
#24780=CARTESIAN_POINT ( 'NONE',  ( 88.05889915941182267, 44.40447472371889148, 4.714184461739163723 ) ) ;
#24790=EDGE_CURVE ( 'NONE', #64236, #8542, #67006, .T. ) ;
#24795=CARTESIAN_POINT ( 'NONE',  ( 83.63860429472313740, 52.00081728452852303, 14.99618877770985037 ) ) ;
#24798=EDGE_CURVE ( 'NONE', #7307, #75846, #51826, .T. ) ;
#24800=CARTESIAN_POINT ( 'NONE',  ( 67.16256804578091533, 66.80979783321161847, 8.146902435796070208 ) ) ;
#24801=DIRECTION ( 'NONE',  ( -0.8660254037844378194, -0.5000000000000014433, -0.000000000000000000 ) ) ;
#24802=CLOSED_SHELL ( 'NONE', ( #44072, #70329, #13512, #58361, #36264, #30283, #2153, #33384, #62783, #10148, #50741, #27320, #88941, #90056, #92383, #45445, #31717, #19360, #47972, #1467, #94142, #53696, #50072, #81296, #21561, #40783, #22081, #4261, #75599, #95085, #39849, #81578, #17033, #35198, #73899, #11966, #96794, #10744, #85595, #80758, #98733, #40668, #64116, #70402, #7763, #29939, #25576, #90216, #11417, #10013, #17707, #14397, #90584, #97304, #76019, #43495, #39867, #95667, #37345, #58441, #39820, #5632, #73292, #58752, #95308, #2514, #74916, #89504, #51217, #66679, #95778, #55335, #85990, #17302, #65176, #88950, #92674, #64250, #33169, #18398, #36209, #17966, #34250, #88780, #94515, #52684, #1240, #77757, #87326, #77417, #52249, #3541, #32675, #69027, #62346, #76785, #82619, #30088, #39816, #13099, #86640, #52125, #9704, #99595, #18358, #77290, #28559, #13958, #18747, #44563, #72074, #77609, #26962, #100091, #62717, #14709, #36823, #8420, #2856, #59940, #54853, #17737, #6894, #54322, #4012, #92204, #44066, #58265, #44229, #32802, #56152, #70417, #62780, #86412, #71365, #25746, #6495, #57096, #44879, #38631, #32801, #69278, #1739, #71043, #96904, #64248, #59801, #40986, #60226, #25765, #50126, #24240, #60177, #2859, #73654, #79652, #43221, #23282, #59043, #80769, #11623, #12546, #17956, #48248, #49696, #83796, #85712, #60493, #5271, #51077, #85794, #45707, #2910, #844, #35940, #78057, #28440, #42292, #32904, #40673, #83381, #8429, #35675, #1823, #88448, #70028, #8482, #78246, #62911, #12584, #81009, #27589, #88742, #39896, #82642, #2348, #32360, #49191, #42055, #72339, #12266, #42241, #39879, #69408, #44237, #72403, #46732, #88947, #97958, #59876, #14472, #6950, #67070, #94374, #18717, #5234, #32371, #67870, #18851, #91171, #42519, #8747, #71490, #22022, #44114, #27779, #78623, #66723, #97336, #76915, #89715, #58077, #75348, #30183, #52458, #55852, #68203, #2983, #4707, #11775, #5846, #48241, #75725, #96477, #90282, #95503, #95657, #43683, #9892, #4075, #45470, #52420, #608, #32975, #14614, #13218, #8006, #80922, #10057, #34879, #20465, #66768, #36901, #96859, #32466, #36642, #34254, #26309, #58186, #52386, #72598, #94089, #95492, #43135, #36768, #45252, #35264, #49943, #47898, #94506, #70537, #67084, #70085, #20344, #38636, #18891, #15225, #89987, #7658, #768, #27093, #24338 ) ) ;
#24803=CARTESIAN_POINT ( 'NONE',  ( 74.01887009131820605, 64.01258356010848161, -14.05577849739043650 ) ) ;
#24807=CARTESIAN_POINT ( 'NONE',  ( 29.77967365985639248, 29.14441083166262203, 10.00000000000000533 ) ) ;
#24814=CIRCLE ( 'NONE', #89607, 16.60714546451156792 ) ;
#24815=CARTESIAN_POINT ( 'NONE',  ( 81.46622351318225697, 45.77194399688346493, 11.40994803060552520 ) ) ;
#24817=AXIS2_PLACEMENT_3D ( 'NONE', #48692, #18295, #64381 ) ;
#24820=DIRECTION ( 'NONE',  ( 0.6758705274779430727, 0.2489746672676115269, -0.6936934806855756808 ) ) ;
#24823=CARTESIAN_POINT ( 'NONE',  ( 22.35053764064823767, 35.83705186507754803, 3.090169943749475401 ) ) ;
#24824=CARTESIAN_POINT ( 'NONE',  ( 30.93718178480143877, 33.56454794089042792, 10.00000000000000355 ) ) ;
#24827=CARTESIAN_POINT ( 'NONE',  ( 73.55923329020097867, 67.59775090522703067, 12.07291635799731999 ) ) ;
#24828=CARTESIAN_POINT ( 'NONE',  ( 81.89930626873778863, 42.21375885382297355, 7.647715624843501203 ) ) ;
#24833=CARTESIAN_POINT ( 'NONE',  ( 68.12436787710551300, 66.83910121369015656, -8.880904761776434952 ) ) ;
#24847=CARTESIAN_POINT ( 'NONE',  ( 23.32838594064934767, 31.65586893147757408, -7.433330006724137462 ) ) ;
#24852=ORIENTED_EDGE ( 'NONE', *, *, #10502, .F. ) ;
#24853=CARTESIAN_POINT ( 'NONE',  ( 4.685401460390529849, 24.74646525600388003, 2.839279412974139660 ) ) ;
#24854=CARTESIAN_POINT ( 'NONE',  ( 72.21948760849898008, 60.12913787482489880, -15.14087808330432594 ) ) ;
#24855=CARTESIAN_POINT ( 'NONE',  ( 71.77363275119753894, 72.50400781664164640, -1.333432854898964681 ) ) ;
#24859=CARTESIAN_POINT ( 'NONE',  ( 85.45686282584428284, 49.07624996843039611, 12.35599031532369452 ) ) ;
#24862=EDGE_CURVE ( 'NONE', #11364, #20041, #95265, .T. ) ;
#24866=CARTESIAN_POINT ( 'NONE',  ( 83.42425903942064735, 42.46362989694333834, -5.239620355152831976 ) ) ;
#24869=CARTESIAN_POINT ( 'NONE',  ( 71.90245059369782155, 72.17364547496468674, -3.641340926847324244 ) ) ;
#24870=CARTESIAN_POINT ( 'NONE',  ( 72.71113525135035616, 57.05229220753940211, -15.90378019451816094 ) ) ;
#24872=EDGE_CURVE ( 'NONE', #20250, #93322, #81760, .T. ) ;
#24880=CARTESIAN_POINT ( 'NONE',  ( 30.88926192328758447, 20.76004757982090609, 5.678558825948272215 ) ) ;
#24883=CARTESIAN_POINT ( 'NONE',  ( 74.20995892610953604, 68.60058487300136676, 11.52733404855582755 ) ) ;
#24895=CARTESIAN_POINT ( 'NONE',  ( 69.87205324732853740, 69.72719669029187628, -5.804370611097000143 ) ) ;
#24901=CARTESIAN_POINT ( 'NONE',  ( 86.23513880351241312, 43.01419119376065936, -3.607706737359228644 ) ) ;
#24902=CARTESIAN_POINT ( 'NONE',  ( 67.34941845850391928, 66.92956724091470733, 9.029314852957725179 ) ) ;
#24903=CARTESIAN_POINT ( 'NONE',  ( 75.79750337254498049, 64.14884731463476442, -14.49056795948485110 ) ) ;
#24909=CARTESIAN_POINT ( 'NONE',  ( 84.12544262676013318, 41.86299551560625076, -0.4765227021652564954 ) ) ;
#24913=DIRECTION ( 'NONE',  ( -0.1710100716628374096, 0.2961981327260301833, 0.9396926207859057634 ) ) ;
#24916=CARTESIAN_POINT ( 'NONE',  ( 80.55623134086874870, 57.74356886441330516, -16.24537044847425804 ) ) ;
#24927=CARTESIAN_POINT ( 'NONE',  ( 85.35443477132466228, 48.30880629543902671, -11.80360700664791018 ) ) ;
#24928=CARTESIAN_POINT ( 'NONE',  ( 87.78619429942361307, 44.41240826577528367, -3.951812172081524022 ) ) ;
#24931=CARTESIAN_POINT ( 'NONE',  ( 82.10523990517462778, 41.85707133252697076, -5.529865280922466653 ) ) ;
#24936=CARTESIAN_POINT ( 'NONE',  ( 76.58844930818931118, 53.16667539083663030, -15.92936049379509456 ) ) ;
#24939=CARTESIAN_POINT ( 'NONE',  ( 88.00125901251291793, 44.79538816511593069, 4.736495928124922372 ) ) ;
#24941=CARTESIAN_POINT ( 'NONE',  ( 9.082762260191241666, 27.01751292744054567, 6.180339887498949913 ) ) ;
#24950=CARTESIAN_POINT ( 'NONE',  ( 17.93656579593215028, 10.75978393459163307, -1.583844403245362020 ) ) ;
#24953=AXIS2_PLACEMENT_3D ( 'NONE', #53707, #61314, #37025 ) ;
#24958=CARTESIAN_POINT ( 'NONE',  ( 31.10096393961467598, 36.14336893147757479, 7.433330006724141015 ) ) ;
#24961=CARTESIAN_POINT ( 'NONE',  ( 25.46698091360950045, 30.10171378149919974, 9.188101187500008038 ) ) ;
#24965=CARTESIAN_POINT ( 'NONE',  ( 66.04563933824955768, 68.55708310873542644, 2.069072683234986609 ) ) ;
#24967=CARTESIAN_POINT ( 'NONE',  ( 80.33508072308801218, 44.92307697338561212, 11.19555900290710326 ) ) ;
#24970=CARTESIAN_POINT ( 'NONE',  ( 16.34664070491415444, 11.29860640527290983, -2.839279412974138328 ) ) ;
#24984=CARTESIAN_POINT ( 'NONE',  ( 86.26094451566392252, 47.67890430677171310, 10.76907119421248460 ) ) ;
#24986=CARTESIAN_POINT ( 'NONE',  ( 24.75116620650193866, 19.45404122711133965, -8.090169943749478065 ) ) ;
#24991=CARTESIAN_POINT ( 'NONE',  ( 84.71672111353214518, 48.50487602508921725, -12.22989703533773032 ) ) ;
#24992=CARTESIAN_POINT ( 'NONE',  ( 80.73512995292455230, 43.24773137545005142, 9.993358235750852359 ) ) ;
#25001=EDGE_CURVE ( 'NONE', #14695, #24162, #15049, .T. ) ;
#25005=CARTESIAN_POINT ( 'NONE',  ( 72.97982471419457795, 59.59981046274725003, 15.43291100737614663 ) ) ;
#25006=VERTEX_POINT ( 'NONE', #73515 ) ;
#25009=CARTESIAN_POINT ( 'NONE',  ( 83.23886772428572556, 49.12744029586829697, 13.18137976536933031 ) ) ;
#25010=CARTESIAN_POINT ( 'NONE',  ( 69.98658646620340562, 66.36472102019232011, 10.66432767654794311 ) ) ;
#25015=CARTESIAN_POINT ( 'NONE',  ( 78.44203751522358914, 61.21016990572090322, 16.24725970467587643 ) ) ;
#25016=CARTESIAN_POINT ( 'NONE',  ( 18.54180792094154029, 32.74646525600390135, 2.839279412974139660 ) ) ;
#25030=ORIENTED_EDGE ( 'NONE', *, *, #44451, .T. ) ;
#25034=DIRECTION ( 'NONE',  ( 0.3715724127386967335, -0.6435822975543782354, -0.6691306063588567943 ) ) ;
#25038=CARTESIAN_POINT ( 'NONE',  ( 82.26726714915119487, 40.87605626266926606, -1.219143652196071459 ) ) ;
#25045=CARTESIAN_POINT ( 'NONE',  ( 75.53874658597716518, 65.44746306994376539, 13.83256553230837760 ) ) ;
#25053=CARTESIAN_POINT ( 'NONE',  ( 67.33690759333875064, 68.97606460400891137, 3.668405113326242084 ) ) ;
#25054=CARTESIAN_POINT ( 'NONE',  ( 83.83342451037863441, 43.32515297521197084, 6.643328278011193078 ) ) ;
#25056=CARTESIAN_POINT ( 'NONE',  ( 74.17344901341724039, 68.45477986254626046, -11.63824756869785659 ) ) ;
#25061=CARTESIAN_POINT ( 'NONE',  ( 82.12214578622800332, 43.36728084772444447, 8.278842856071861434 ) ) ;
#25065=CARTESIAN_POINT ( 'NONE',  ( 69.04169954231571182, 64.33839118639518517, -11.93766638194810703 ) ) ;
#25069=CARTESIAN_POINT ( 'NONE',  ( 72.79105583609376140, 67.08523038410258721, 12.12250871139724318 ) ) ;
#25076=CARTESIAN_POINT ( 'NONE',  ( 15.51250667149479590, 27.14336893147754992, 7.433330006724141015 ) ) ;
#25077=CARTESIAN_POINT ( 'NONE',  ( 75.03548522729336412, 67.17073137636660363, 12.58381819018166325 ) ) ;
#25078=CYLINDRICAL_SURFACE ( 'NONE', #64581, 10.00000000000001066 ) ;
#25082=CARTESIAN_POINT ( 'NONE',  ( 28.21526782163968861, 21.45404122711134320, -8.090169943749478065 ) ) ;
#25093=CARTESIAN_POINT ( 'NONE',  ( 75.69558293296576323, 65.12864963431647425, -14.43849588152979813 ) ) ;
#25095=CARTESIAN_POINT ( 'NONE',  ( 75.37843707191279918, 53.50823561223473490, 16.04097401286667335 ) ) ;
#25096=CARTESIAN_POINT ( 'NONE',  ( 74.90335404720867984, 53.25525787180524873, -16.52187237106487672 ) ) ;
#25098=EDGE_LOOP ( 'NONE', ( #94829, #22881, #63781, #6594, #96321, #29263, #94655, #16292, #15495, #50331, #29491, #59142, #40676, #77957, #68519, #4410, #85342, #32624, #89637, #4424, #91206, #28102, #89823, #6929, #14941, #72500, #6679, #88496, #26409, #4537, #23888, #85149, #57303, #94489, #42620, #93421, #75702, #16025 ) ) ;
#25100=B_SPLINE_SURFACE_WITH_KNOTS ( 'NONE', 3, 1, ( 
 ( #77709, #70580 ),
 ( #55857, #86852 ),
 ( #55365, #47767 ),
 ( #78706, #9292 ),
 ( #40167, #71108 ),
 ( #17384, #48295 ),
 ( #9813, #65483 ),
 ( #2711, #3221 ),
 ( #34583, #34106 ),
 ( #94928, #11319 ),
 ( #11807, #4178 ),
 ( #95454, #49785 ),
 ( #18912, #72108 ),
 ( #73597, #19901 ),
 ( #10297, #73112 ),
 ( #33598, #79737 ),
 ( #80747, #80235 ),
 ( #96935, #50772 ),
 ( #42177, #64493 ),
 ( #19424, #87377 ),
 ( #64997, #26006 ),
 ( #56379, #41170 ),
 ( #48803, #81723 ),
 ( #57379, #56876 ),
 ( #25488, #17906 ),
 ( #27502, #65982 ),
 ( #58372, #88858 ),
 ( #50280, #89348 ),
 ( #87860, #88352 ),
 ( #18404, #81232 ),
 ( #35078, #12300 ) ),
 .UNSPECIFIED., .F., .F., .F.,
 ( 4, 3, 3, 3, 3, 3, 3, 3, 3, 3, 4 ),
 ( 2, 2 ),
 ( 0.000000000000000000, 0.1333490885032321271, 0.3007194338854310423, 0.4699862290245110930, 0.5844252810809297261, 0.6686540514502729016, 0.7354980260655470392, 0.8028463152565559202, 0.8633854507757028340, 0.9437142632666930542, 1.000000000000000000 ),
 ( 0.000000000000000000, 1.000000000000000000 ),
 .UNSPECIFIED. ) ;
#25101=CARTESIAN_POINT ( 'NONE',  ( 43.01361757626971638, 27.76004757982093452, 5.678558825948272215 ) ) ;
#25109=EDGE_CURVE ( 'NONE', #40944, #329, #816, .T. ) ;
#25110=CARTESIAN_POINT ( 'NONE',  ( 86.44808582675112518, 47.03435218195901513, -10.53111747673478860 ) ) ;
#25112=CARTESIAN_POINT ( 'NONE',  ( 82.43803718576400286, 44.54370618503160983, -10.34432007801551912 ) ) ;
#25114=CARTESIAN_POINT ( 'NONE',  ( 80.31207982290658265, 44.87798361127789093, 11.16639872694695867 ) ) ;
#25116=B_SPLINE_CURVE_WITH_KNOTS ( 'NONE', 3,
 ( #58887, #11353, #42208, #73143, #50312, #73628, #3739, #72656, #51297, #65516, #27031, #34134 ),
 .UNSPECIFIED., .F., .F.,
 ( 4, 2, 2, 2, 2, 4 ),
 ( 0.000000000000000000, 0.1516647414800683380, 0.2274971122201024931, 0.2654132975901196123, 0.2843713902751267564, 0.3033294829601337894 ),
 .UNSPECIFIED. ) ;
#25123=CARTESIAN_POINT ( 'NONE',  ( 77.32958686580666097, 49.14630502970322112, -14.78873007407067419 ) ) ;
#25133=DIRECTION ( 'NONE',  ( -0.2649596321165964552, 0.4589235447807054058, -0.8480480961564325071 ) ) ;
#25136=CARTESIAN_POINT ( 'NONE',  ( 70.60504524851407382, 60.65317718845415129, -14.59496475064744914 ) ) ;
#25137=CARTESIAN_POINT ( 'NONE',  ( 44.29582294825809896, 31.28920272979930672, -7.433330006724141015 ) ) ;
#25140=CARTESIAN_POINT ( 'NONE',  ( 86.73551935668791657, 43.70951659908644160, -4.914342582248948155 ) ) ;
#25146=CARTESIAN_POINT ( 'NONE',  ( 72.32316037510372553, 62.91300431845684926, 14.06911090390365082 ) ) ;
#25150=CARTESIAN_POINT ( 'NONE',  ( 33.22292548896825082, 27.38052372038642801, 10.00000000000000533 ) ) ;
#25154=EDGE_CURVE ( 'NONE', #37549, #36202, #9978, .T. ) ;
#25159=DIRECTION ( 'NONE',  ( 0.2938926261462335709, -0.5090369604551240323, 0.8090169943749504489 ) ) ;
#25166=ORIENTED_EDGE ( 'NONE', *, *, #70341, .T. ) ;
#25176=CARTESIAN_POINT ( 'NONE',  ( 73.96424987833113107, 68.60250435897062005, 11.39670188853132160 ) ) ;
#25178=CARTESIAN_POINT ( 'NONE',  ( 67.72630526519628802, 69.57018049443510677, 1.992863756904409867 ) ) ;
#25182=CARTESIAN_POINT ( 'NONE',  ( 87.95730997019668962, 44.52059963167226186, -3.981301762289743085 ) ) ;
#25184=CARTESIAN_POINT ( 'NONE',  ( 78.66865037864833710, 47.51313895851910729, 14.24506864829981190 ) ) ;
#25185=CARTESIAN_POINT ( 'NONE',  ( 78.37684991480820429, 56.91902664479916041, 16.21588224672203538 ) ) ;
#25187=CARTESIAN_POINT ( 'NONE',  ( 77.70381431022140362, 61.98645263265593286, 15.63931947556489099 ) ) ;
#25189=CARTESIAN_POINT ( 'NONE',  ( 77.54361356138011274, 49.75803992512373952, -14.96129575302290249 ) ) ;
#25192=CARTESIAN_POINT ( 'NONE',  ( 76.22048776404022874, 55.73695481322819489, -16.16703596060795078 ) ) ;
#25195=CARTESIAN_POINT ( 'NONE',  ( 73.66914651274929327, 69.65765408683024873, 9.569081530089540877 ) ) ;
#25201=CARTESIAN_POINT ( 'NONE',  ( 88.45958475239287111, 43.85926912372239883, -0.5941283661710237141 ) ) ;
#25207=CARTESIAN_POINT ( 'NONE',  ( 23.65314546706850862, 31.84336893147757408, -7.433330006724137462 ) ) ;
#25208=CARTESIAN_POINT ( 'NONE',  ( 81.13754030168745146, 45.92056744364227683, 12.30823813837155001 ) ) ;
#25209=CARTESIAN_POINT ( 'NONE',  ( 79.57385746726255604, 47.78104568962750420, -13.55650246241271439 ) ) ;
#25211=CARTESIAN_POINT ( 'NONE',  ( 21.16812676580727270, 15.14754757982089650, -5.678558825948276656 ) ) ;
#25216=CARTESIAN_POINT ( 'NONE',  ( 73.85305739393403712, 66.14698956378720140, 12.75270311107614774 ) ) ;
#25229=CARTESIAN_POINT ( 'NONE',  ( 71.17702396458545877, 68.89634176143304956, -8.584545784728861761 ) ) ;
#25234=CARTESIAN_POINT ( 'NONE',  ( 72.32137329212656596, 71.76143927211870732, 5.594163357809725845 ) ) ;
#25238=CARTESIAN_POINT ( 'NONE',  ( 24.12344523961532161, 25.87878583063842086, -9.188101187500006262 ) ) ;
#25240=CARTESIAN_POINT ( 'NONE',  ( 84.69667606500864565, 50.48814749939704427, -13.55077694746726280 ) ) ;
#25252=CARTESIAN_POINT ( 'NONE',  ( 81.77850890590235622, 55.52106599324014269, -15.95406647289506985 ) ) ;
#25254=CARTESIAN_POINT ( 'NONE',  ( 36.97850982526662023, 33.30066082961424456, -10.00000000000000533 ) ) ;
#25257=CARTESIAN_POINT ( 'NONE',  ( 76.05587244885492737, 61.43040213351050483, -15.89239421180067069 ) ) ;
#25258=LINE ( 'NONE', #41959, #24043 ) ;
#25262=CARTESIAN_POINT ( 'NONE',  ( 78.06822720212770150, 61.43946511097403373, -16.16087495820213960 ) ) ;
#25263=VERTEX_POINT ( 'NONE', #95113 ) ;
#25267=CARTESIAN_POINT ( 'NONE',  ( 80.03413267745405335, 44.49255549320951530, -11.65001753154222186 ) ) ;
#25268=CARTESIAN_POINT ( 'NONE',  ( 66.90444770391341933, 67.53953207032016337, 6.664260923135624459 ) ) ;
#25269=FACE_OUTER_BOUND ( 'NONE', #77497, .T. ) ;
#25270=CARTESIAN_POINT ( 'NONE',  ( 38.08139550823666042, 22.39040679176985904, -6.890680421881970419E-14 ) ) ;
#25274=ORIENTED_EDGE ( 'NONE', *, *, #56796, .T. ) ;
#25281=CARTESIAN_POINT ( 'NONE',  ( 69.89261943739826677, 69.35781508005003104, -6.634928327201882858 ) ) ;
#25286=CARTESIAN_POINT ( 'NONE',  ( 80.76394201868582456, 45.93450986988883500, 11.85631275749819835 ) ) ;
#25292=CARTESIAN_POINT ( 'NONE',  ( 81.19656099875513178, 43.43094936621162105, -9.896970666190501476 ) ) ;
#25294=ORIENTED_EDGE ( 'NONE', *, *, #67322, .T. ) ;
#25299=CARTESIAN_POINT ( 'NONE',  ( 83.22496320156969318, 52.34403607930074287, 14.85522145549952100 ) ) ;
#25306=CARTESIAN_POINT ( 'NONE',  ( 74.15368421650904907, 55.28562771191141678, 16.12354357782822589 ) ) ;
#25308=CARTESIAN_POINT ( 'NONE',  ( 33.14931559527707350, 20.10801979619930435, 3.090169943749476733 ) ) ;
#25313=AXIS2_PLACEMENT_3D ( 'NONE', #56840, #38770, #774 ) ;
#25316=( BOUNDED_CURVE ( )  B_SPLINE_CURVE ( 2, ( #79253, #24499, #40686, #55377, #86866, #86363, #71625, #65010, #40180, #1724, #10314, #10814, #2221 ),
 .UNSPECIFIED., .F., .T. ) 
 B_SPLINE_CURVE_WITH_KNOTS ( ( 3, 2, 2, 2, 2, 2, 3 ),
 ( 0.2625000000000000111, 0.2650000000000000133, 0.2700000000000000178, 0.2750000000000000222, 0.2800000000000000266, 0.2849999999999999756, 0.2874999999999999778 ),
 .UNSPECIFIED. ) 
 CURVE ( )  GEOMETRIC_REPRESENTATION_ITEM ( )  RATIONAL_B_SPLINE_CURVE ( ( 0.9755282581475768211, 0.9755282581475768211, 1.000000000000000000, 0.9510565162951535312, 1.000000000000000000, 0.9510565162951535312, 1.000000000000000000, 0.9510565162951535312, 1.000000000000000000, 0.9510565162951535312, 1.000000000000000000, 0.9755282581475768211, 0.9755282581475768211 ) ) 
 REPRESENTATION_ITEM ( '' )  );
#25323=CARTESIAN_POINT ( 'NONE',  ( 82.35608806024791306, 41.41197313041440253, 5.516391017443479150 ) ) ;
#25326=CARTESIAN_POINT ( 'NONE',  ( 40.95666657127031840, 28.81029122506297924, 8.090169943749479842 ) ) ;
#25331=CARTESIAN_POINT ( 'NONE',  ( 4.743097115929088226, 26.23654200823200000, 1.583844403245363353 ) ) ;
#25333=CARTESIAN_POINT ( 'NONE',  ( 84.04820955589276821, 51.68058956114519731, 14.75728579592695588 ) ) ;
#25335=CARTESIAN_POINT ( 'NONE',  ( 74.82470458544302971, 65.83378423986729899, -13.33277362726854776 ) ) ;
#25339=LINE ( 'NONE', #95800, #66577 ) ;
#25342=FACE_OUTER_BOUND ( 'NONE', #14291, .T. ) ;
#25348=CARTESIAN_POINT ( 'NONE',  ( 29.50362127723248662, 19.96004757982091604, -5.678558825948276656 ) ) ;
#25355=CARTESIAN_POINT ( 'NONE',  ( 5.869580825389008716, 26.49540643055185640, 3.479690158560446702E-15 ) ) ;
#25356=CARTESIAN_POINT ( 'NONE',  ( 79.80752115302324512, 57.35651460586262829, -16.24722079539231956 ) ) ;
#25357=CARTESIAN_POINT ( 'NONE',  ( 71.91886814437489761, 72.60555707853946217, -1.127020781340661193 ) ) ;
#25358=VERTEX_POINT ( 'NONE', #57049 ) ;
#25361=CARTESIAN_POINT ( 'NONE',  ( 81.93820057532437318, 58.80319216612334543, 0.3078307376628310332 ) ) ;
#25365=ORIENTED_EDGE ( 'NONE', *, *, #98313, .F. ) ;
#25366=ORIENTED_EDGE ( 'NONE', *, *, #79415, .T. ) ;
#25373=CARTESIAN_POINT ( 'NONE',  ( 72.73224412574886344, 56.97554388665330549, -15.91743659082035123 ) ) ;
#25374=CARTESIAN_POINT ( 'NONE',  ( 77.20655462988578677, 63.53086439471233859, 15.45977356242439349 ) ) ;
#25384=CARTESIAN_POINT ( 'NONE',  ( 25.58005199048888656, 32.95586893147756768, 7.433330006724141015 ) ) ;
#25386=CARTESIAN_POINT ( 'NONE',  ( 67.59162108422654569, 69.94611594471417959, -2.429117792699152734 ) ) ;
#25388=CARTESIAN_POINT ( 'NONE',  ( 73.98997032606590096, 68.61244119570729083, 11.40121143613689192 ) ) ;
#25393=VERTEX_POINT ( 'NONE', #28155 ) ;
#25394=CARTESIAN_POINT ( 'NONE',  ( 75.36396396989580637, 58.32137975822279685, -15.97037604966454438 ) ) ;
#25404=CARTESIAN_POINT ( 'NONE',  ( 75.98882072545443123, 65.54910008167897217, 13.91231000067740275 ) ) ;
#25410=CARTESIAN_POINT ( 'NONE',  ( 84.11621381539826814, 42.22557305609230838, 3.174655551866189196 ) ) ;
#25413=CARTESIAN_POINT ( 'NONE',  ( 83.60569444237076198, 51.47509952066116767, -14.39597358549856843 ) ) ;
#25416=CARTESIAN_POINT ( 'NONE',  ( 80.58776074949071244, 57.68173972368585112, -16.24394003362809968 ) ) ;
#25428=CARTESIAN_POINT ( 'NONE',  ( 70.42029346824453739, 62.39263015420969083, -14.29769421334009749 ) ) ;
#25432=CARTESIAN_POINT ( 'NONE',  ( 68.39600206231747848, 70.06355299527018587, -1.199260098510152028 ) ) ;
#25440=CARTESIAN_POINT ( 'NONE',  ( 18.81282613181931040, 26.56454794089041371, 10.00000000000000355 ) ) ;
#25444=CARTESIAN_POINT ( 'NONE',  ( 87.04122873496829982, 46.31593380912286761, -9.298662157179395038 ) ) ;
#25446=CARTESIAN_POINT ( 'NONE',  ( 16.01096549046674511, 31.01751292744055988, 6.180339887498949913 ) ) ;
#25447=CARTESIAN_POINT ( 'NONE',  ( 85.93470712620026575, 48.23248545518190866, 11.93606436224419198 ) ) ;
#25451=FACE_OUTER_BOUND ( 'NONE', #38668, .T. ) ;
#25465=CARTESIAN_POINT ( 'NONE',  ( 36.29711636232130445, 39.14336893147758900, 7.433330006724141015 ) ) ;
#25469=CARTESIAN_POINT ( 'NONE',  ( 22.53213034355506750, 33.98502408145593279, -5.678558825948271327 ) ) ;
#25472=CARTESIAN_POINT ( 'NONE',  ( 66.18591460530085158, 68.59894752875132440, 2.300355685169377828 ) ) ;
#25477=CARTESIAN_POINT ( 'NONE',  ( 16.02188117849498639, 11.11110640527290983, -2.839279412974138328 ) ) ;
#25479=CARTESIAN_POINT ( 'NONE',  ( 12.48623565965559479, 28.18502408145590721, 5.678558825948276656 ) ) ;
#25482=CARTESIAN_POINT ( 'NONE',  ( 87.98439851106198262, 44.06910850096573995, -1.717092390252117573 ) ) ;
#25487=CARTESIAN_POINT ( 'NONE',  ( 66.25644290789426805, 68.19202803638752641, 4.197190157902950247 ) ) ;
#25488=CARTESIAN_POINT ( 'NONE',  ( 87.41847558182290356, 44.98594970355499356, 6.912341091792672643 ) ) ;
#25493=CARTESIAN_POINT ( 'NONE',  ( 85.86500116153743534, 47.48139021253037839, 10.80080889994705906 ) ) ;
#25497=LINE ( 'NONE', #8303, #95361 ) ;
#25499=CARTESIAN_POINT ( 'NONE',  ( 78.35410446158606135, 61.54825803293332598, -15.81517172436243790 ) ) ;
#25501=CARTESIAN_POINT ( 'NONE',  ( 79.13712759260106111, 59.42437504702360940, -16.53516983581165434 ) ) ;
#25502=CARTESIAN_POINT ( 'NONE',  ( 80.59841950988781889, 48.28954382714877624, -14.06662836619941892 ) ) ;
#25504=CARTESIAN_POINT ( 'NONE',  ( 80.72615790689530968, 43.21908027699803512, 9.966345867180507412 ) ) ;
#25510=CARTESIAN_POINT ( 'NONE',  ( 29.58720089054306968, 40.58029201028043786, 1.583844403245363353 ) ) ;
#25514=CARTESIAN_POINT ( 'NONE',  ( 37.57390229391633341, 33.64441083166263979, -10.00000000000000533 ) ) ;
#25515=VERTEX_POINT ( 'NONE', #40724 ) ;
#25520=ORIENTED_EDGE ( 'NONE', *, *, #71507, .T. ) ;
#25528=CARTESIAN_POINT ( 'NONE',  ( 82.63376612087627393, 53.27330958937008631, -15.29856784112376822 ) ) ;
#25531=ORIENTED_EDGE ( 'NONE', *, *, #51563, .F. ) ;
#25533=CARTESIAN_POINT ( 'NONE',  ( 16.91979795264450459, 27.95586893147755347, 7.433330006724141015 ) ) ;
#25538=AXIS2_PLACEMENT_3D ( 'NONE', #43822, #36221, #69114 ) ;
#25540=DIRECTION ( 'NONE',  ( 0.5000000000000014433, -0.8660254037844378194, 0.000000000000000000 ) ) ;
#25542=CARTESIAN_POINT ( 'NONE',  ( 38.90461549961826648, 38.16454794089045066, -10.00000000000000355 ) ) ;
#25546=EDGE_LOOP ( 'NONE', ( #27525, #50120, #99775, #18172 ) ) ;
#25548=CARTESIAN_POINT ( 'NONE',  ( 13.85453579343919905, 10.12755873383624383, -6.180339887498949025 ) ) ;
#25554=CARTESIAN_POINT ( 'NONE',  ( 82.09616139842204063, 40.74998018113815590, -0.9067466716294869666 ) ) ;
#25555=B_SPLINE_CURVE_WITH_KNOTS ( 'NONE', 3,
 ( #24158, #39824, #55043, #71778, #56031, #16551, #47446, #78375, #17048, #63152 ),
 .UNSPECIFIED., .F., .F.,
 ( 4, 2, 2, 2, 4 ),
 ( 0.000000000000000000, 0.0002622400424273465310, 0.0005244800848546930620, 0.0007867201272820395930, 0.001048960169709386124 ),
 .UNSPECIFIED. ) ;
#25556=CARTESIAN_POINT ( 'NONE',  ( 14.54318666465499632, 27.13478043621387314, 8.090169943749478065 ) ) ;
#25562=VERTEX_POINT ( 'NONE', #34152 ) ;
#25565=CARTESIAN_POINT ( 'NONE',  ( 67.37707244819222296, 69.01508689139724595, 3.611659466110988870 ) ) ;
#25566=CARTESIAN_POINT ( 'NONE',  ( 29.75882387383049377, 25.38052372038642446, 10.00000000000000533 ) ) ;
#25569=CARTESIAN_POINT ( 'NONE',  ( 69.10817959322751847, 64.24658173014449858, 12.03926405174448000 ) ) ;
#25570=CARTESIAN_POINT ( 'NONE',  ( 74.06641568892433725, 68.90029856846140888, -11.17356148674937444 ) ) ;
#25576=ADVANCED_FACE ( 'NONE', ( #41222 ), #18459, .T. ) ;
#25577=CARTESIAN_POINT ( 'NONE',  ( 83.47332239865056636, 45.96411348524937068, 10.52733798611148508 ) ) ;
#25582=CARTESIAN_POINT ( 'NONE',  ( 68.94203703131894656, 64.31246542778407616, -11.91225929259457672 ) ) ;
#25586=CARTESIAN_POINT ( 'NONE',  ( 87.98594423550160570, 43.75089820288621212, -2.253463800273092676 ) ) ;
#25595=CARTESIAN_POINT ( 'NONE',  ( 21.54279312762077936, 14.29860640527291871, -2.839279412974138328 ) ) ;
#25596=CARTESIAN_POINT ( 'NONE',  ( 75.18968313674336912, 67.03148441216438869, 12.73605655727703123 ) ) ;
#25598=VECTOR ( 'NONE', #69969, 1000.000000000000114 ) ;
#25602=ORIENTED_EDGE ( 'NONE', *, *, #65306, .F. ) ;
#25607=CARTESIAN_POINT ( 'NONE',  ( 81.56781671333388317, 55.98423300004855463, -16.39433532902865309 ) ) ;
#25609=CARTESIAN_POINT ( 'NONE',  ( 75.31289280905393468, 53.62176160565092431, -16.53289957284814449 ) ) ;
#25613=CARTESIAN_POINT ( 'NONE',  ( 71.97456596565469056, 72.60744930783874906, 1.463844530419991852 ) ) ;
#25616=CARTESIAN_POINT ( 'NONE',  ( 72.29675234079142854, 71.91852905550483399, -5.160928375136445645 ) ) ;
#25621=CARTESIAN_POINT ( 'NONE',  ( 36.41018743920069056, 41.99752408145594273, 5.678558825948277544 ) ) ;
#25624=CARTESIAN_POINT ( 'NONE',  ( 77.72420466810140738, 61.55156736199941037, 16.09483585134336181 ) ) ;
#25627=CARTESIAN_POINT ( 'NONE',  ( 87.74907107289486419, 44.16117455547063742, -4.521424286948807492 ) ) ;
#25629=CARTESIAN_POINT ( 'NONE',  ( 78.70723262944966336, 59.87900897892416197, 16.12280052229424498 ) ) ;
#25632=B_SPLINE_CURVE_WITH_KNOTS ( 'NONE', 3,
 ( #68033, #7220, #98954, #76635, #38104, #69017, #61418, #38616, #69524, #136 ),
 .UNSPECIFIED., .F., .F.,
 ( 4, 2, 2, 2, 4 ),
 ( 0.000000000000000000, 0.2500000000000000000, 0.5000000000000000000, 0.7500000000000000000, 1.000000000000000000 ),
 .UNSPECIFIED. ) ;
#25633=CARTESIAN_POINT ( 'NONE',  ( 17.41845772768865075, 33.55466486950699334, -1.111400068045478839E-16 ) ) ;
#25635=CARTESIAN_POINT ( 'NONE',  ( 79.65090360336043318, 51.49598528711052836, -15.19126888219039451 ) ) ;
#25636=CARTESIAN_POINT ( 'NONE',  ( 80.55107469691334643, 44.51596713245550063, 11.40293197512799672 ) ) ;
#25643=ORIENTED_EDGE ( 'NONE', *, *, #92264, .F. ) ;
#25644=CYLINDRICAL_SURFACE ( 'NONE', #46748, 16.60714546451156792 ) ;
#25652=DIRECTION ( 'NONE',  ( 0.8660254037844339337, 0.5000000000000081046, -0.000000000000000000 ) ) ;
#25657=TOROIDAL_SURFACE ( 'NONE', #45084, 16.10714546451156437, 0.5000000000000000000 ) ;
#25660=CARTESIAN_POINT ( 'NONE',  ( 70.64756877957057668, 61.00196420740825687, -14.45602737464827392 ) ) ;
#25661=CARTESIAN_POINT ( 'NONE',  ( 44.05945362601616466, 27.29860640527295956, -2.839279412974138328 ) ) ;
#25664=CARTESIAN_POINT ( 'NONE',  ( 88.33748333995926316, 44.07075497373335793, -2.898134731201833070 ) ) ;
#25672=CARTESIAN_POINT ( 'NONE',  ( 79.07351061557720584, 55.41849508022395554, 16.50442470572476594 ) ) ;
#25675=VECTOR ( 'NONE', #99299, 999.9999999999998863 ) ;
#25688=AXIS2_PLACEMENT_3D ( 'NONE', #29423, #14227, #60297 ) ;
#25692=CARTESIAN_POINT ( 'NONE',  ( 74.39841895140679640, 68.21392270468032848, 11.95628786500076579 ) ) ;
#25694=CARTESIAN_POINT ( 'NONE',  ( 71.74349412889739597, 65.94227022788277282, -11.98261597976729753 ) ) ;
#25696=CARTESIAN_POINT ( 'NONE',  ( 74.38015889281619764, 68.44084013566667579, 11.75477996513195045 ) ) ;
#25697=CARTESIAN_POINT ( 'NONE',  ( 81.19029346057565988, 43.43118860823614114, -9.901472530966298535 ) ) ;
#25698=CARTESIAN_POINT ( 'NONE',  ( 67.18445374837708073, 69.11489579876541711, 2.756726376966783132 ) ) ;
#25709=CARTESIAN_POINT ( 'NONE',  ( 5.530962353892125094, 15.14441083166257584, 0.000000000000000000 ) ) ;
#25710=CARTESIAN_POINT ( 'NONE',  ( 76.61888230030999125, 51.35972145264445032, 16.07233720539656119 ) ) ;
#25716=CARTESIAN_POINT ( 'NONE',  ( 77.47733472172021152, 54.59384519352943954, -16.52087748544757417 ) ) ;
#25718=CARTESIAN_POINT ( 'NONE',  ( 66.43953443436691941, 68.06212878376058484, -4.898982275787033380 ) ) ;
#25720=CARTESIAN_POINT ( 'NONE',  ( 76.77731254116882553, 64.09355814141257213, -15.16545583891343263 ) ) ;
#25727=DIRECTION ( 'NONE',  ( 0.8660254037844379305, 0.5000000000000014433, 0.000000000000000000 ) ) ;
#25730=CARTESIAN_POINT ( 'NONE',  ( 33.38390286057418166, 24.98920272979928470, 7.433330006724137462 ) ) ;
#25731=CARTESIAN_POINT ( 'NONE',  ( 81.33727068537973537, 46.45028969087891824, 12.62407423705470144 ) ) ;
#25734=CARTESIAN_POINT ( 'NONE',  ( 14.85459438965255607, 31.68290643055187061, 3.479690158560446702E-15 ) ) ;
#25742=CARTESIAN_POINT ( 'NONE',  ( 86.47115166784590201, 47.25330420953332577, 10.74459335058070941 ) ) ;
#25746=ADVANCED_FACE ( 'NONE', ( #78137 ), #1130, .T. ) ;
#25747=CARTESIAN_POINT ( 'NONE',  ( 75.24899567225237718, 53.31857512432304702, 16.02918851208695017 ) ) ;
#25753=DIRECTION ( 'NONE',  ( -0.3978777116982054607, -0.7304723483372553838, -0.5550706935593476832 ) ) ;
#25761=CARTESIAN_POINT ( 'NONE',  ( 81.70949458604077620, 44.04605918311328594, 10.26744876709650534 ) ) ;
#25763=VERTEX_POINT ( 'NONE', #15811 ) ;
#25764=CARTESIAN_POINT ( 'NONE',  ( 36.79557518129325899, 43.01751292744059896, 6.180339887498949913 ) ) ;
#25765=ADVANCED_FACE ( 'NONE', ( #46716 ), #30207, .T. ) ;
#25766=CARTESIAN_POINT ( 'NONE',  ( 34.51575008502857855, 31.87878583063843863, -9.188101187500006262 ) ) ;
#25767=CARTESIAN_POINT ( 'NONE',  ( 84.83932634351975821, 50.31781210311571328, -13.41000248947998941 ) ) ;
#25768=CARTESIAN_POINT ( 'NONE',  ( 85.69676750305241342, 47.72673510730739821, -11.08893409868475821 ) ) ;
#25771=ORIENTED_EDGE ( 'NONE', *, *, #21052, .F. ) ;
#25774=CARTESIAN_POINT ( 'NONE',  ( 68.22205435732229262, 65.90345407231323804, 10.80313017776371254 ) ) ;
#25779=CARTESIAN_POINT ( 'NONE',  ( 70.88228214377448921, 60.99952434776093924, 15.04298896821893727 ) ) ;
#25782=CARTESIAN_POINT ( 'NONE',  ( 69.95523204135936624, 62.90150226501648234, 13.86126985460704653 ) ) ;
#25785=CARTESIAN_POINT ( 'NONE',  ( 73.76988841918569051, 55.47430203404649518, -16.58764015103525580 ) ) ;
#25786=CARTESIAN_POINT ( 'NONE',  ( 77.87641386972968860, 61.39850456329286743, -16.14647179981831115 ) ) ;
#25790=CARTESIAN_POINT ( 'NONE',  ( 80.02161912385248854, 44.37003809598091664, -11.54766014928761386 ) ) ;
#25792=DIRECTION ( 'NONE',  ( -0.9634819383873028942, 0.2491829092639709919, -0.09803281150813239475 ) ) ;
#25793=CARTESIAN_POINT ( 'NONE',  ( 35.76051414856368638, 25.81029122506296858, 8.090169943749479842 ) ) ;
#25804=FACE_OUTER_BOUND ( 'NONE', #18681, .T. ) ;
#25805=CARTESIAN_POINT ( 'NONE',  ( 21.47138989493050332, 31.13478043621388736, 8.090169943749478065 ) ) ;
#25806=CARTESIAN_POINT ( 'NONE',  ( 67.97625722659998360, 69.06288173737418390, -4.661947418481645400 ) ) ;
#25807=CARTESIAN_POINT ( 'NONE',  ( 87.79103035407327127, 45.19801466894013942, -6.906962003849810294 ) ) ;
#25808=LINE ( 'NONE', #56683, #26704 ) ;
#25809=CARTESIAN_POINT ( 'NONE',  ( 87.79117399615233808, 44.76081256804975794, 4.995967170566625093 ) ) ;
#25810=AXIS2_PLACEMENT_3D ( 'NONE', #63820, #9128, #1542 ) ;
#25813=CARTESIAN_POINT ( 'NONE',  ( 81.33832127110852639, 47.47515066021468044, 12.76697642013896505 ) ) ;
#25816=CARTESIAN_POINT ( 'NONE',  ( 71.45874632471999632, 59.24191456302641257, -15.76368813740517538 ) ) ;
#25817=CARTESIAN_POINT ( 'NONE',  ( 76.28872632190459058, 51.00282802105012081, -16.03419075268624994 ) ) ;
#25823=CARTESIAN_POINT ( 'NONE',  ( 86.54292033101232562, 46.25028892199808439, 8.970843135639702481 ) ) ;
#25824=CARTESIAN_POINT ( 'NONE',  ( 24.48906155743269508, 15.10801979619929014, 3.090169943749476733 ) ) ;
#25825=CARTESIAN_POINT ( 'NONE',  ( 78.38601017018802963, 61.50250219569392129, 16.18534724403903269 ) ) ;
#25835=CARTESIAN_POINT ( 'NONE',  ( 29.70092825881656751, 40.08080186712595605, -3.090169943749475845 ) ) ;
#25843=CARTESIAN_POINT ( 'NONE',  ( 81.44852512392907329, 45.72822924548952273, 11.37997471554883155 ) ) ;
#25845=CARTESIAN_POINT ( 'NONE',  ( 86.59946856559290040, 46.34450665633656996, 9.054963042594563305 ) ) ;
#25846=CARTESIAN_POINT ( 'NONE',  ( 81.78702560211090145, 41.63811551741589767, 5.443813600127541008 ) ) ;
#25850=CARTESIAN_POINT ( 'NONE',  ( 36.09163463545626627, 29.03677371833804344, 10.00000000000000533 ) ) ;
#25861=CARTESIAN_POINT ( 'NONE',  ( 39.76905880593325548, 23.36477965099643228, 1.583844403245330712 ) ) ;
#25863=CARTESIAN_POINT ( 'NONE',  ( 67.28998128626176367, 66.40108913371626898, -8.819887048254448914 ) ) ;
#25868=DIRECTION ( 'NONE',  ( 0.8660254037844378194, 0.5000000000000016653, 0.000000000000000000 ) ) ;
#25869=ORIENTED_EDGE ( 'NONE', *, *, #53586, .T. ) ;
#25870=CARTESIAN_POINT ( 'NONE',  ( 73.98570270871888965, 68.92876820612470112, -11.10152750440662750 ) ) ;
#25873=CARTESIAN_POINT ( 'NONE',  ( 71.24283209038772213, 66.52597613840981694, 11.86082254693358173 ) ) ;
#25874=CARTESIAN_POINT ( 'NONE',  ( 22.00590953607929023, 34.74646525600390845, 2.839279412974139660 ) ) ;
#25879=CARTESIAN_POINT ( 'NONE',  ( 6.618913549016022912, 24.79752408145590081, -5.678558825948271327 ) ) ;
#25882=EDGE_CURVE ( 'NONE', #83882, #53490, #41904, .T. ) ;
#25885=B_SPLINE_CURVE_WITH_KNOTS ( 'NONE', 3,
 ( #93527, #39263, #79338, #31668, #32182, #23569, #23074, #62066, #47380, #46365, #17487, #100112, #24084, #93014, #77294, #92527 ),
 .UNSPECIFIED., .F., .F.,
 ( 4, 1, 2, 2, 2, 1, 2, 2, 4 ),
 ( 0.000000000000000000, 0.1249999999999998057, 0.1874999999999997224, 0.2499999999999996114, 0.5000000000000031086, 0.6250000000000028866, 0.6875000000000027756, 0.7500000000000026645, 1.000000000000000000 ),
 .UNSPECIFIED. ) ;
#25886=CARTESIAN_POINT ( 'NONE',  ( 85.17400780349038314, 49.04769795992583425, 12.45946173256488265 ) ) ;
#25888=CARTESIAN_POINT ( 'NONE',  ( 71.98077362405804536, 64.91430807166688055, -13.35472713366527486 ) ) ;
#25889=ORIENTED_EDGE ( 'NONE', *, *, #64816, .F. ) ;
#25892=CARTESIAN_POINT ( 'NONE',  ( 69.93330931759959412, 71.50341667604121199, 8.155205941333377477E-06 ) ) ;
#25898=CARTESIAN_POINT ( 'NONE',  ( 70.40987744940257187, 71.50345078331645254, -2.811369489084570183 ) ) ;
#25899=CARTESIAN_POINT ( 'NONE',  ( 78.04364300777291419, 61.42399649461658129, -16.16113552180852508 ) ) ;
#25907=CARTESIAN_POINT ( 'NONE',  ( 32.78369927745970358, 30.87878583063843863, -9.188101187500006262 ) ) ;
#25911=CARTESIAN_POINT ( 'NONE',  ( 73.98997032606590096, 68.61244119570729083, 10.90121143613688304 ) ) ;
#25921=CARTESIAN_POINT ( 'NONE',  ( 67.53901457411087961, 69.18284913860507856, -3.335900949275148353 ) ) ;
#25926=CARTESIAN_POINT ( 'NONE',  ( 84.98744680587442701, 42.71960512013303912, -5.006987873416975710 ) ) ;
#25931=ORIENTED_EDGE ( 'NONE', *, *, #81673, .F. ) ;
#25933=CARTESIAN_POINT ( 'NONE',  ( 83.20693519809137229, 41.48837047502863840, 1.928222989275212740 ) ) ;
#25934=CARTESIAN_POINT ( 'NONE',  ( 74.32283972735670829, 55.33658384534069796, 16.60204640374922036 ) ) ;
#25938=ORIENTED_EDGE ( 'NONE', *, *, #63705, .F. ) ;
#25939=CARTESIAN_POINT ( 'NONE',  ( 80.09948508391848065, 57.43746099958096352, -16.59413991463535964 ) ) ;
#25940=( BOUNDED_CURVE ( )  B_SPLINE_CURVE ( 2, ( #66140, #88507, #89497, #20056, #35739, #12455, #73256, #98050, #43326, #28627, #72780, #50929, #51940 ),
 .UNSPECIFIED., .F., .F. ) 
 B_SPLINE_CURVE_WITH_KNOTS ( ( 3, 2, 2, 2, 2, 2, 3 ),
 ( 0.4625000000000000222, 0.4650000000000000244, 0.4699999999999999734, 0.4749999999999999778, 0.4799999999999999822, 0.4849999999999999867, 0.4874999999999999889 ),
 .UNSPECIFIED. ) 
 CURVE ( )  GEOMETRIC_REPRESENTATION_ITEM ( )  RATIONAL_B_SPLINE_CURVE ( ( 0.9755282581475768211, 0.9755282581475768211, 1.000000000000000000, 0.9510565162951535312, 1.000000000000000000, 0.9510565162951535312, 1.000000000000000000, 0.9510565162951535312, 1.000000000000000000, 0.9510565162951535312, 1.000000000000000000, 0.9755282581475768211, 0.9755282581475768211 ) ) 
 REPRESENTATION_ITEM ( '' )  );
#25948=CARTESIAN_POINT ( 'NONE',  ( 67.16327201103491973, 67.73731889023999031, 6.573435314091262249 ) ) ;
#25956=DIRECTION ( 'NONE',  ( -0.5000000000000043299, 0.8660254037844362651, -8.973825869789965068E-15 ) ) ;
#25962=CARTESIAN_POINT ( 'NONE',  ( 77.14157061559578210, 52.99909543789008382, -15.86103023851207361 ) ) ;
#25968=CARTESIAN_POINT ( 'NONE',  ( 15.42233441037273423, 31.83705186507753382, 3.090169943749475401 ) ) ;
#25970=FACE_OUTER_BOUND ( 'NONE', #94022, .T. ) ;
#25971=CARTESIAN_POINT ( 'NONE',  ( 72.28517652677638239, 71.97109234898169916, -3.701588698221916829 ) ) ;
#25973=CARTESIAN_POINT ( 'NONE',  ( 71.93359151460639112, 71.98077168563673922, 2.829254084576380723 ) ) ;
#25974=PLANE ( 'NONE',  #2428 ) ;
#25984=CARTESIAN_POINT ( 'NONE',  ( 38.48863484149602954, 25.14754757982092670, -5.678558825948276656 ) ) ;
#25988=CARTESIAN_POINT ( 'NONE',  ( 29.08566721201706784, 38.83396525600392124, -2.839279412974133887 ) ) ;
#25992=FACE_OUTER_BOUND ( 'NONE', #93448, .T. ) ;
#25994=CARTESIAN_POINT ( 'NONE',  ( 13.40518456965460281, 16.24335787977761925, -9.188101187500008038 ) ) ;
#25996=CARTESIAN_POINT ( 'NONE',  ( 18.31506083472495661, 16.28920272979926054, -7.433330006724141015 ) ) ;
#25999=CARTESIAN_POINT ( 'NONE',  ( 84.60239308390620749, 50.60453406874029270, -14.06751209996561158 ) ) ;
#26002=ORIENTED_EDGE ( 'NONE', *, *, #37953, .T. ) ;
#26005=CARTESIAN_POINT ( 'NONE',  ( 66.28155827565299774, 68.16852158415039753, 4.313148695808196820 ) ) ;
#26006=CARTESIAN_POINT ( 'NONE',  ( 87.26772313172064344, 45.44742106685279737, 7.124560975800460660 ) ) ;
#26011=CARTESIAN_POINT ( 'NONE',  ( 86.29568871537288999, 47.66748683144847831, 10.73674591253165822 ) ) ;
#26013=CARTESIAN_POINT ( 'NONE',  ( 78.03746721159666322, 59.28273036852866085, 16.09598523568621076 ) ) ;
#26016=CARTESIAN_POINT ( 'NONE',  ( 38.34546801798370552, 23.10801979619931501, 3.090169943749476733 ) ) ;
#26017=CARTESIAN_POINT ( 'NONE',  ( 83.96860308896397385, 48.73281357008495718, -12.68925788642582297 ) ) ;
#26021=EDGE_LOOP ( 'NONE', ( #66849, #40280, #68154, #53909 ) ) ;
#26028=ORIENTED_EDGE ( 'NONE', *, *, #40977, .F. ) ;
#26037=EDGE_CURVE ( 'NONE', #2384, #77129, #40970, .T. ) ;
#26043=CARTESIAN_POINT ( 'NONE',  ( 20.65934362447757167, 23.87878583063841376, -9.188101187500006262 ) ) ;
#26045=CARTESIAN_POINT ( 'NONE',  ( 77.53919650534660946, 49.73269318645782988, -15.46600695893548227 ) ) ;
#26051=CARTESIAN_POINT ( 'NONE',  ( 85.49318370521093868, 48.99722645306705715, -12.73116331006621493 ) ) ;
#26060=CARTESIAN_POINT ( 'NONE',  ( 82.52994871329097748, 40.49336819921385455, -1.416186232783453125 ) ) ;
#26061=CARTESIAN_POINT ( 'NONE',  ( 12.55362526388469746, 30.18080186712592194, 3.090169943749475401 ) ) ;
#26069=CARTESIAN_POINT ( 'NONE',  ( 69.40068436163360843, 70.67970960180943507, 0.7597560883736370618 ) ) ;
#26070=CARTESIAN_POINT ( 'NONE',  ( 83.97020538542169277, 43.52084701081836471, 6.873119719476476597 ) ) ;
#26083=CARTESIAN_POINT ( 'NONE',  ( 69.07519263286346245, 64.34084314335252941, -11.95120022168340412 ) ) ;
#26097=CARTESIAN_POINT ( 'NONE',  ( 26.56574046957052460, 17.19860640527293327, 2.839279412974134775 ) ) ;
#26098=CARTESIAN_POINT ( 'NONE',  ( 75.26069627141727381, 66.83174392109067696, 12.89175359686561961 ) ) ;
#26106=LINE ( 'NONE', #3807, #8626 ) ;
#26108=CARTESIAN_POINT ( 'NONE',  ( 81.70827727213743685, 55.24394141669957747, -15.91687133283663869 ) ) ;
#26116=CARTESIAN_POINT ( 'NONE',  ( 72.38671951208186783, 71.75852817245944948, -5.691748070601700960 ) ) ;
#26118=ORIENTED_EDGE ( 'NONE', *, *, #32475, .T. ) ;
#26120=CARTESIAN_POINT ( 'NONE',  ( 7.095368192108828076, 22.83478043621386178, -8.090169943749479842 ) ) ;
#26130=CARTESIAN_POINT ( 'NONE',  ( 88.05069107734583156, 43.77613950941169918, -2.175448891271404506 ) ) ;
#26139=CARTESIAN_POINT ( 'NONE',  ( 76.99824972205654205, 49.58236607186867673, 15.01116573833570378 ) ) ;
#26142=CARTESIAN_POINT ( 'NONE',  ( 88.28592015977814356, 44.16006502160688996, -0.2344584660017056954 ) ) ;
#26145=CARTESIAN_POINT ( 'NONE',  ( 82.58415536943712709, 40.81765542747830722, 3.215309922963823563 ) ) ;
#26146=CARTESIAN_POINT ( 'NONE',  ( 80.67724759154341996, 43.51231060136900197, -9.541306243518663521 ) ) ;
#26155=CARTESIAN_POINT ( 'NONE',  ( 70.62074857767794356, 61.40485173823782361, -14.80809279627126607 ) ) ;
#26156=ORIENTED_EDGE ( 'NONE', *, *, #8925, .F. ) ;
#26159=VERTEX_POINT ( 'NONE', #3032 ) ;
#26166=CARTESIAN_POINT ( 'NONE',  ( 83.90596095485256001, 41.21795184261720379, -1.108148245180562033E-06 ) ) ;
#26171=ORIENTED_EDGE ( 'NONE', *, *, #28447, .F. ) ;
#26173=CARTESIAN_POINT ( 'NONE',  ( 76.19955060832064930, 61.81918726698732769, -15.41303817956920064 ) ) ;
#26185=CARTESIAN_POINT ( 'NONE',  ( 76.35339246177476014, 61.05343328037434247, -15.60956989098418290 ) ) ;
#26190=CARTESIAN_POINT ( 'NONE',  ( 80.67704869399170775, 43.49956702784530904, -9.526446727701394224 ) ) ;
#26191=CARTESIAN_POINT ( 'NONE',  ( 67.08348705826007574, 69.02495177153369355, 2.899183874508027170 ) ) ;
#26195=CARTESIAN_POINT ( 'NONE',  ( 88.17106782721933200, 44.41923492627702075, -4.565543248975953539 ) ) ;
#26199=CARTESIAN_POINT ( 'NONE',  ( 81.54419519852100962, 59.48562949720209048, 0.3078307376628255376 ) ) ;
#26208=CARTESIAN_POINT ( 'NONE',  ( 79.82019804487738668, 54.41907435463492959, -15.91247824403962596 ) ) ;
#26209=CARTESIAN_POINT ( 'NONE',  ( 76.24020477147122676, 54.98903279212289164, -16.58624229681600326 ) ) ;
#26210=CARTESIAN_POINT ( 'NONE',  ( 73.37237386183839760, 69.84228272576173424, 9.150815133132212509 ) ) ;
#26212=CARTESIAN_POINT ( 'NONE',  ( 86.78549426258130950, 45.83013854792883990, 8.849882187839872572 ) ) ;
#26215=CARTESIAN_POINT ( 'NONE',  ( 72.48667266402317466, 57.40015563624327655, 15.83031223551729560 ) ) ;
#26220=CARTESIAN_POINT ( 'NONE',  ( 29.25887229277395463, 38.93396525600392266, 2.839279412974139660 ) ) ;
#26222=CARTESIAN_POINT ( 'NONE',  ( 85.56354969485944650, 46.62399995276157227, -10.02333073147364040 ) ) ;
#26224=CARTESIAN_POINT ( 'NONE',  ( 16.65397613197454518, 21.56628583063840310, 9.188101187500006262 ) ) ;
#26232=FACE_OUTER_BOUND ( 'NONE', #81118, .T. ) ;
#26234=CARTESIAN_POINT ( 'NONE',  ( 72.06694649076332837, 71.38420282548176488, 5.126693848571997059 ) ) ;
#26235=CARTESIAN_POINT ( 'NONE',  ( 87.30348251005597149, 44.98986743115608533, -6.196706157115566604 ) ) ;
#26238=CARTESIAN_POINT ( 'NONE',  ( 75.00053908662732738, 53.26751709772522503, 16.03872633732851227 ) ) ;
#26240=CARTESIAN_POINT ( 'NONE',  ( 85.42093500504424242, 46.21730090332891905, 9.681390438263864695 ) ) ;
#26246=CARTESIAN_POINT ( 'NONE',  ( 77.31150235362825640, 63.25814829948299689, -15.20253986937943935 ) ) ;
#26250=CARTESIAN_POINT ( 'NONE',  ( 84.14312167556933275, 48.98415679381830756, 0.000000000000000000 ) ) ;
#26254=CARTESIAN_POINT ( 'NONE',  ( 36.08541434599421649, 23.76004757982091675, 5.678558825948272215 ) ) ;
#26255=CARTESIAN_POINT ( 'NONE',  ( 84.21135162255031048, 48.08253741963655159, -12.07440697007694119 ) ) ;
#26259=ORIENTED_EDGE ( 'NONE', *, *, #74231, .T. ) ;
#26260=ORIENTED_EDGE ( 'NONE', *, *, #94144, .F. ) ;
#26275=ORIENTED_EDGE ( 'NONE', *, *, #24311, .F. ) ;
#26278=ORIENTED_EDGE ( 'NONE', *, *, #54891, .F. ) ;
#26279=CARTESIAN_POINT ( 'NONE',  ( 80.14239153911771041, 44.91288235749343727, -11.28435394345837928 ) ) ;
#26288=ORIENTED_EDGE ( 'NONE', *, *, #60564, .T. ) ;
#26289=ORIENTED_EDGE ( 'NONE', *, *, #45134, .T. ) ;
#26293=CARTESIAN_POINT ( 'NONE',  ( 75.69558293296576323, 65.12864963431647425, -14.43849588152979813 ) ) ;
#26298=CARTESIAN_POINT ( 'NONE',  ( 87.95111445425231977, 44.80020534355205797, 4.839585637743885727 ) ) ;
#26300=CARTESIAN_POINT ( 'NONE',  ( 88.19053702688614749, 44.32527345396092500, -2.493626234014364673 ) ) ;
#26303=CARTESIAN_POINT ( 'NONE',  ( 82.35140075591571929, 40.37528365890498350, -1.256860545790653205 ) ) ;
#26305=CARTESIAN_POINT ( 'NONE',  ( 71.79944583284617465, 59.58521246314043651, -15.72103291199168318 ) ) ;
#26309=ADVANCED_FACE ( 'NONE', ( #83030 ), #44474, .T. ) ;
#26311=CARTESIAN_POINT ( 'NONE',  ( 82.98592046873434924, 41.48112914865087220, 2.708872267169455839 ) ) ;
#26312=CARTESIAN_POINT ( 'NONE',  ( 13.99874362242318604, 31.58029201028041300, 1.583844403245363353 ) ) ;
#26313=CARTESIAN_POINT ( 'NONE',  ( 78.31032011038168150, 61.54964048803103793, 15.80295067388503050 ) ) ;
#26317=EDGE_CURVE ( 'NONE', #27838, #76006, #12615, .T. ) ;
#26321=CARTESIAN_POINT ( 'NONE',  ( 74.20017517015935482, 55.33913510227883847, 16.12309036971300458 ) ) ;
#26322=EDGE_CURVE ( 'NONE', #10212, #45167, #19229, .T. ) ;
#26323=CARTESIAN_POINT ( 'NONE',  ( 79.00824644612984571, 51.04380436647237929, 15.61778681553768244 ) ) ;
#26324=CARTESIAN_POINT ( 'NONE',  ( 32.37774987120970849, 30.64441083166263269, -10.00000000000000533 ) ) ;
#26328=CARTESIAN_POINT ( 'NONE',  ( 85.47202168011459378, 43.45241828910128135, -4.867446897391397798 ) ) ;
#26330=CARTESIAN_POINT ( 'NONE',  ( 82.54152556014342679, 49.05345396727486218, 13.38640032703253624 ) ) ;
#26332=CARTESIAN_POINT ( 'NONE',  ( 87.34667321826604791, 45.97495992385612595, 8.598559468654661586 ) ) ;
#26333=CARTESIAN_POINT ( 'NONE',  ( 65.74726825304114186, 69.08659106095529978, 2.128305819671951817E-12 ) ) ;
#26334=CARTESIAN_POINT ( 'NONE',  ( 82.35975313184987101, 41.41624149272713851, 5.521678208627143647 ) ) ;
#26338=CARTESIAN_POINT ( 'NONE',  ( 87.06988255670405863, 46.05766899987094831, 8.936389965629217613 ) ) ;
#26340=CARTESIAN_POINT ( 'NONE',  ( 32.66923259237032084, 34.56454794089044213, 10.00000000000000355 ) ) ;
#26353=CARTESIAN_POINT ( 'NONE',  ( 67.37944191706843355, 66.71681795993420394, -8.450929298107464405 ) ) ;
#26363=CARTESIAN_POINT ( 'NONE',  ( 80.96546451793241772, 46.78193962505741865, -13.01366642040773947 ) ) ;
#26364=CARTESIAN_POINT ( 'NONE',  ( 33.16918417342686354, 21.01110640527294038, 2.839279412974134775 ) ) ;
#26368=ORIENTED_EDGE ( 'NONE', *, *, #65306, .T. ) ;
#26369=CARTESIAN_POINT ( 'NONE',  ( 12.32504541118064978, 22.51421378149917985, -9.188101187500004485 ) ) ;
#26373=CARTESIAN_POINT ( 'NONE',  ( 72.23468229527969697, 71.59820328793978206, -5.860928441596811922 ) ) ;
#26385=CARTESIAN_POINT ( 'NONE',  ( 72.98169074979469428, 57.62652471086132522, -16.32181584066402991 ) ) ;
#26386=CARTESIAN_POINT ( 'NONE',  ( 78.39164420400439326, 61.24742163703882625, -15.88566992787024823 ) ) ;
#26396=CARTESIAN_POINT ( 'NONE',  ( 32.59967566254915994, 39.79752408145595410, -5.678558825948271327 ) ) ;
#26398=CARTESIAN_POINT ( 'NONE',  ( 78.15916255518206412, 47.79662076820892480, -13.98612838149463755 ) ) ;
#26401=CARTESIAN_POINT ( 'NONE',  ( 73.79815732168846409, 68.46225211080071915, 11.43730676814645442 ) ) ;
#26406=ORIENTED_EDGE ( 'NONE', *, *, #18434, .F. ) ;
#26407=CARTESIAN_POINT ( 'NONE',  ( 75.51395409436767636, 58.27241819066912853, -15.98951179309681159 ) ) ;
#26409=ORIENTED_EDGE ( 'NONE', *, *, #11528, .F. ) ;
#26417=CARTESIAN_POINT ( 'NONE',  ( 83.00815485991435594, 53.30142267139499523, 15.60062745561815767 ) ) ;
#26420=EDGE_LOOP ( 'NONE', ( #64676, #8686, #18138, #18562 ) ) ;
#26425=CARTESIAN_POINT ( 'NONE',  ( 83.94709567845697507, 42.07943496863257593, 2.936195033694379841 ) ) ;
#26427=DIRECTION ( 'NONE',  ( -0.1378186779084930869, 0.2387089523694814197, -0.9612616959383223358 ) ) ;
#26432=CARTESIAN_POINT ( 'NONE',  ( 80.63145207929048297, 57.26919043701818879, -16.23179315233208087 ) ) ;
#26433=EDGE_CURVE ( 'NONE', #30181, #90587, #23171, .T. ) ;
#26448=CARTESIAN_POINT ( 'NONE',  ( 11.96499418379068480, 31.00034080476288878, -1.878358725466461243E-16 ) ) ;
#26455=CARTESIAN_POINT ( 'NONE',  ( 78.36746962641299774, 52.62081666013096992, -15.66493875128054469 ) ) ;
#26462=CARTESIAN_POINT ( 'NONE',  ( 14.83370333027871801, 32.65659080271450421, -1.878358725466461243E-16 ) ) ;
#26467=CARTESIAN_POINT ( 'NONE',  ( 73.94850163436859702, 55.42609493996558001, -16.11567799753128227 ) ) ;
#26470=CARTESIAN_POINT ( 'NONE',  ( 74.93659349595930053, 67.20166626244473207, 12.52374196637391357 ) ) ;
#26478=CARTESIAN_POINT ( 'NONE',  ( 35.85928575902275384, 36.10171378149922106, 9.188101187500008038 ) ) ;
#26481=DIRECTION ( 'NONE',  ( 0.5000000000000013323, -0.8660254037844378194, 0.000000000000000000 ) ) ;
#26482=CARTESIAN_POINT ( 'NONE',  ( 35.55378427144160014, 29.03085787977765264, 9.188101187500006262 ) ) ;
#26483=CARTESIAN_POINT ( 'NONE',  ( 16.86745276891122103, 33.23654200823202842, 1.583844403245363353 ) ) ;
#26485=CARTESIAN_POINT ( 'NONE',  ( 81.12452645434240139, 43.43369904203282772, -9.948711836735455449 ) ) ;
#26488=CARTESIAN_POINT ( 'NONE',  ( 14.00658445089738180, 13.80170272979924917, 7.433330006724137462 ) ) ;
#26490=CARTESIAN_POINT ( 'NONE',  ( 16.11390655273756778, 24.70171378149918340, -9.188101187500004485 ) ) ;
#26494=CARTESIAN_POINT ( 'NONE',  ( 88.24741913774678892, 44.24286465476006924, -1.859444097506131488 ) ) ;
#26495=EDGE_LOOP ( 'NONE', ( #98774, #99302, #12043, #23255 ) ) ;
#26500=AXIS2_PLACEMENT_3D ( 'NONE', #69061, #7770, #47749 ) ;
#26506=CARTESIAN_POINT ( 'NONE',  ( 86.47552948348150892, 47.43782623826668043, 10.38323646570730752 ) ) ;
#26508=CARTESIAN_POINT ( 'NONE',  ( 77.33305236775244396, 55.26159023894539501, 16.12204705925791970 ) ) ;
#26512=CARTESIAN_POINT ( 'NONE',  ( 82.32629372474684715, 49.22594776363517610, -13.55554168643329049 ) ) ;
#26514=B_SPLINE_CURVE_WITH_KNOTS ( 'NONE', 3,
 ( #43340, #76737, #23020, #38724, #69629, #84873, #15415, #61530, #15928, #7331 ),
 .UNSPECIFIED., .F., .F.,
 ( 4, 2, 2, 2, 4 ),
 ( 0.000000000000000000, 0.0002622400424273768345, 0.0005244800848547536689, 0.0007867201272821304492, 0.001048960169709507338 ),
 .UNSPECIFIED. ) ;
#26515=CARTESIAN_POINT ( 'NONE',  ( 80.79660903030796248, 43.04784081911883220, 9.716927669273982104 ) ) ;
#26529=CARTESIAN_POINT ( 'NONE',  ( 80.09120749856197108, 44.41673742825524585, -10.86461196121644157 ) ) ;
#26530=VERTEX_POINT ( 'NONE', #6497 ) ;
#26534=CARTESIAN_POINT ( 'NONE',  ( 72.56680254073344827, 71.38637538794351656, 5.777867564336608197 ) ) ;
#26535=CARTESIAN_POINT ( 'NONE',  ( 81.89485588203808675, 55.22971306509118250, 16.24120679747552032 ) ) ;
#26540=CARTESIAN_POINT ( 'NONE',  ( 28.52090319329063206, 17.26216523072495690, -2.296566073217252530E-15 ) ) ;
#26542=CARTESIAN_POINT ( 'NONE',  ( 77.55384616172401024, 49.72970008889385696, -15.46212513759681428 ) ) ;
#26543=CARTESIAN_POINT ( 'NONE',  ( 69.35253854976201637, 63.01665765323906498, 13.58811665770852350 ) ) ;
#26546=ORIENTED_EDGE ( 'NONE', *, *, #70885, .T. ) ;
#26568=CARTESIAN_POINT ( 'NONE',  ( 88.14145358481059134, 44.06566488169897866, 0.5518357132556823696 ) ) ;
#26573=CARTESIAN_POINT ( 'NONE',  ( 68.59280378597286187, 64.14102549347582283, 11.89188498909244629 ) ) ;
#26577=EDGE_CURVE ( 'NONE', #73884, #39921, #32423, .T. ) ;
#26579=CARTESIAN_POINT ( 'NONE',  ( 84.52987419023656912, 49.02393738901606923, 12.65494964629210983 ) ) ;
#26584=CARTESIAN_POINT ( 'NONE',  ( 68.71429273641867042, 63.93483983531514525, -12.10708682878116527 ) ) ;
#26596=CARTESIAN_POINT ( 'NONE',  ( 20.04711164229383513, 17.28920272979926764, -7.433330006724141015 ) ) ;
#26597=CARTESIAN_POINT ( 'NONE',  ( 74.89402362195637863, 67.20670802991241999, 12.50338612930198146 ) ) ;
#26606=CARTESIAN_POINT ( 'NONE',  ( 81.66708723681374238, 55.20605668156866841, -15.91457100465458474 ) ) ;
#26610=CARTESIAN_POINT ( 'NONE',  ( 72.10745786146183889, 72.33289146567349803, 0.8714635118042719508 ) ) ;
#26611=CARTESIAN_POINT ( 'NONE',  ( 77.71017327488615933, 49.43655273470124456, 15.32784876113035288 ) ) ;
#26614=CARTESIAN_POINT ( 'NONE',  ( 72.33760062768145360, 71.68797599686796218, -5.790821312261726916 ) ) ;
#26618=CARTESIAN_POINT ( 'NONE',  ( 7.614983434379491101, 23.13478043621386249, 8.090169943749478065 ) ) ;
#26621=CARTESIAN_POINT ( 'NONE',  ( 77.92825354283080230, 61.79113456967466789, 16.06764011202815468 ) ) ;
#26625=CARTESIAN_POINT ( 'NONE',  ( 79.31323107047896315, 59.76145823410249136, 16.51491591541846660 ) ) ;
#26628=CARTESIAN_POINT ( 'NONE',  ( 77.74446929066526479, 52.10494957478874767, -15.63064665268012376 ) ) ;
#26635=DIRECTION ( 'NONE',  ( 0.3978777116982039619, 0.7304723483372554949, 0.5550706935593484603 ) ) ;
#26639=CARTESIAN_POINT ( 'NONE',  ( 88.34040369365730783, 44.17924546850527179, 0.3139463615716704958 ) ) ;
#26642=CARTESIAN_POINT ( 'NONE',  ( 82.15513920341352616, 40.66133961728853308, 3.593347833157086502 ) ) ;
#26647=EDGE_CURVE ( 'NONE', #76194, #15371, #13911, .T. ) ;
#26652=CARTESIAN_POINT ( 'NONE',  ( 88.06269261788008862, 43.61796610520790551, 0.05835779599787207367 ) ) ;
#26655=ORIENTED_EDGE ( 'NONE', *, *, #22761, .T. ) ;
#26662=CARTESIAN_POINT ( 'NONE',  ( 72.48661302258760486, 71.52526770760661634, -5.337229783571229014 ) ) ;
#26663=CARTESIAN_POINT ( 'NONE',  ( 88.30455217607853058, 43.91915848855261828, -2.151936166193182398 ) ) ;
#26664=ORIENTED_EDGE ( 'NONE', *, *, #60072, .F. ) ;
#26666=CARTESIAN_POINT ( 'NONE',  ( 65.95405552260710635, 69.20365738631340946, 0.2585006146049920739 ) ) ;
#26668=CARTESIAN_POINT ( 'NONE',  ( 88.33748333995926316, 44.07075497373335793, -2.898134731201826852 ) ) ;
#26674=CARTESIAN_POINT ( 'NONE',  ( 88.08517209305595941, 44.29913593851635767, 2.778213776158472648 ) ) ;
#26678=CARTESIAN_POINT ( 'NONE',  ( 74.04344310693554121, 61.81268583747974077, -14.95296161341949848 ) ) ;
#26679=CARTESIAN_POINT ( 'NONE',  ( 79.83401254395657531, 57.87045807247318407, 16.26439772172797404 ) ) ;
#26682=CARTESIAN_POINT ( 'NONE',  ( 80.82399500712998019, 43.24504854750488647, -9.930955225068224479 ) ) ;
#26690=B_SPLINE_CURVE_WITH_KNOTS ( 'NONE', 3,
 ( #20960, #58905, #91360, #19951, #59916, #44707, #90384, #82784, #36120, #28523, #29046, #20450, #5240, #97950, #12861, #75640 ),
 .UNSPECIFIED., .F., .F.,
 ( 4, 1, 2, 2, 2, 1, 2, 2, 4 ),
 ( 0.000000000000000000, 0.1249999999999992506, 0.1874999999999994449, 0.2499999999999996669, 0.4999999999999998890, 0.6250000000000001110, 0.6875000000000003331, 0.7500000000000004441, 1.000000000000000000 ),
 .UNSPECIFIED. ) ;
#26692=B_SPLINE_CURVE_WITH_KNOTS ( 'NONE', 3,
 ( #42480, #65301, #75408, #35392, #65786, #73910, #81056, #74915, #43481, #35889, #5010, #96243, #97717, #28285, #90649, #20709, #82550, #50101, #13115, #43974, #5498, #67285, #21207, #4001, #52087, #98212, #83033, #13603, #44477, #26804, #57687, #11619, #34887, #27307, #85020, #46987, #7999, #36886, #83532, #76410, #99204, #67794, #60166, #14096, #29790, #69282 ),
 .UNSPECIFIED., .F., .F.,
 ( 4, 1, 1, 1, 2, 2, 1, 1, 1, 2, 2, 1, 1, 2, 2, 1, 1, 2, 2, 1, 1, 2, 2, 1, 2, 2, 1, 2, 2, 4 ),
 ( 0.000000000000000000, 0.06250000000000983935, 0.09375000000001355860, 0.1093750000000154321, 0.1171875000000157513, 0.1250000000000160705, 0.1875000000000305589, 0.2187500000000371925, 0.2343750000000392741, 0.2421875000000397460, 0.2500000000000401901, 0.3125000000000500711, 0.3437500000000562883, 0.3593750000000585643, 0.3750000000000608957, 0.4375000000000651701, 0.4687500000000668909, 0.4843750000000661138, 0.5000000000000652811, 0.5625000000000554001, 0.5937500000000518474, 0.6093750000000499600, 0.6250000000000480727, 0.6875000000000401901, 0.7187500000000348610, 0.7500000000000295319, 0.8125000000000217604, 0.8437500000000176525, 0.8750000000000136557, 1.000000000000000000 ),
 .UNSPECIFIED. ) ;
#26694=CARTESIAN_POINT ( 'NONE',  ( 77.15155500632977237, 50.73808484653564221, 15.35664286137126489 ) ) ;
#26702=CARTESIAN_POINT ( 'NONE',  ( 78.04917184312711242, 55.09204980408419772, -16.10415483157210659 ) ) ;
#26704=VECTOR ( 'NONE', #18700, 1000.000000000000114 ) ;
#26711=CARTESIAN_POINT ( 'NONE',  ( 82.09936887833779906, 51.48109869154082219, -15.14494387904524864 ) ) ;
#26713=CARTESIAN_POINT ( 'NONE',  ( 86.81854227949330038, 43.42264536667640584, -3.855948753652409522 ) ) ;
#26715=CARTESIAN_POINT ( 'NONE',  ( 66.54264984482914258, 68.81226801441182772, 2.258477026830895795 ) ) ;
#26716=CARTESIAN_POINT ( 'NONE',  ( 35.63556891041371699, 26.28920272979929607, -7.433330006724141015 ) ) ;
#26718=CARTESIAN_POINT ( 'NONE',  ( 74.57503898873223136, 56.40329876199222525, 16.56847014829402553 ) ) ;
#26719=VERTEX_POINT ( 'NONE', #1893 ) ;
#26720=CARTESIAN_POINT ( 'NONE',  ( 17.19404571121151548, 18.43085787977762280, -9.188101187500008038 ) ) ;
#26725=CARTESIAN_POINT ( 'NONE',  ( 86.25117823697901542, 47.20812847272011226, 10.82755581481952056 ) ) ;
#26730=CARTESIAN_POINT ( 'NONE',  ( 74.96166150690207530, 53.27833328053394979, 16.04207443345645245 ) ) ;
#26733=VERTEX_POINT ( 'NONE', #58438 ) ;
#26735=CARTESIAN_POINT ( 'NONE',  ( 1.030962353892107330, 22.93863946572252743, 0.000000000000000000 ) ) ;
#26738=CARTESIAN_POINT ( 'NONE',  ( 77.30414578634690770, 63.13278840050173812, -15.24465609931389487 ) ) ;
#26743=CARTESIAN_POINT ( 'NONE',  ( 83.13827405794465619, 47.56982798971775139, 12.68584740263780297 ) ) ;
#26747=CARTESIAN_POINT ( 'NONE',  ( 28.38624132378438958, 39.49540643055189548, 3.479690158560446702E-15 ) ) ;
#26748=CARTESIAN_POINT ( 'NONE',  ( 84.80399932964064647, 47.93957977109545254, -11.70082172808313103 ) ) ;
#26750=FACE_OUTER_BOUND ( 'NONE', #50913, .T. ) ;
#26751=B_SPLINE_CURVE_WITH_KNOTS ( 'NONE', 3,
 ( #82963, #85327, #97650, #5429, #15872, #8288, #13048, #8782, #28217, #16381, #54873, #82485, #26494, #33083, #87855, #41669, #80229, #17901, #63978, #48290, #25482, #48798, #79729, #10797 ),
 .UNSPECIFIED., .F., .F.,
 ( 4, 2, 2, 2, 2, 2, 2, 2, 2, 2, 2, 4 ),
 ( 0.000000000000000000, 0.1249999999999956701, 0.2499999999999913403, 0.3749999999999870104, 0.4374999999999887312, 0.4999999999999900080, 0.5624999999999912292, 0.6249999999999925615, 0.6874999999999937828, 0.7499999999999951150, 0.8749999999999975575, 1.000000000000000000 ),
 .UNSPECIFIED. ) ;
#26758=CARTESIAN_POINT ( 'NONE',  ( 85.51397903554266122, 48.65227260402726017, 12.46570927396283146 ) ) ;
#26766=CARTESIAN_POINT ( 'NONE',  ( 79.40659458863603959, 59.69041580281565018, 16.52608132308843736 ) ) ;
#26768=ORIENTED_EDGE ( 'NONE', *, *, #69625, .F. ) ;
#26774=CARTESIAN_POINT ( 'NONE',  ( 86.97822204926990253, 45.79386009709899952, -8.643660422075560845 ) ) ;
#26785=( GEOMETRIC_REPRESENTATION_CONTEXT ( 3 ) GLOBAL_UNCERTAINTY_ASSIGNED_CONTEXT ( ( #79803 ) ) GLOBAL_UNIT_ASSIGNED_CONTEXT ( ( #80219, #17894, #57364 ) ) REPRESENTATION_CONTEXT ( 'NONE', 'WORKASPACE' ) );
#26790=CARTESIAN_POINT ( 'NONE',  ( 69.70373566977634994, 62.70902085928403835, -13.31389724659099016 ) ) ;
#26793=CARTESIAN_POINT ( 'NONE',  ( 86.85456002791893582, 44.01107763648593618, -4.201576838953794635 ) ) ;
#26794=CARTESIAN_POINT ( 'NONE',  ( 81.44373164288916200, 47.79091324518223871, 12.93866338402850147 ) ) ;
#26798=B_SPLINE_CURVE_WITH_KNOTS ( 'NONE', 3,
 ( #55139, #10067, #86124, #17667, #16654, #95209, #38944, #69850 ),
 .UNSPECIFIED., .F., .F.,
 ( 4, 2, 2, 4 ),
 ( 0.6245648125881849699, 0.7184236094411386997, 0.8122824062940925405, 1.000000000000000000 ),
 .UNSPECIFIED. ) ;
#26803=CARTESIAN_POINT ( 'NONE',  ( 80.01120875526221710, 50.16365770749508357, 14.62385428340041926 ) ) ;
#26804=CARTESIAN_POINT ( 'NONE',  ( 70.25980337983864388, 70.48501441192767913, -4.468181338594434671 ) ) ;
#26806=CARTESIAN_POINT ( 'NONE',  ( 78.17252251050902601, 61.73722341659915713, 16.11086890919064274 ) ) ;
#26809=CARTESIAN_POINT ( 'NONE',  ( 30.24436146177389162, 33.16454794089043645, -10.00000000000000355 ) ) ;
#26812=CARTESIAN_POINT ( 'NONE',  ( 70.67237675181191037, 64.83686998721212547, -12.31838050195076839 ) ) ;
#26816=CARTESIAN_POINT ( 'NONE',  ( 29.28550225947944341, 41.00034080476293497, -1.878358725466461243E-16 ) ) ;
#26818=( BOUNDED_CURVE ( )  B_SPLINE_CURVE ( 2, ( #62469, #23988, #84835, #40175, #24986, #15373, #31081, #1715, #15885, #47284, #38686, #46271, #16393 ),
 .UNSPECIFIED., .F., .T. ) 
 B_SPLINE_CURVE_WITH_KNOTS ( ( 3, 2, 2, 2, 2, 2, 3 ),
 ( 0.4375000000000000000, 0.4400000000000000022, 0.4450000000000000067, 0.4500000000000000111, 0.4550000000000000155, 0.4600000000000000200, 0.4625000000000000222 ),
 .UNSPECIFIED. ) 
 CURVE ( )  GEOMETRIC_REPRESENTATION_ITEM ( )  RATIONAL_B_SPLINE_CURVE ( ( 0.9755282581475768211, 0.9755282581475768211, 1.000000000000000000, 0.9510565162951535312, 1.000000000000000000, 0.9510565162951535312, 1.000000000000000000, 0.9510565162951535312, 1.000000000000000000, 0.9510565162951535312, 1.000000000000000000, 0.9755282581475768211, 0.9755282581475768211 ) ) 
 REPRESENTATION_ITEM ( '' )  );
#26821=CARTESIAN_POINT ( 'NONE',  ( 83.86240323164606991, 43.27496035831070742, -6.513153732076713887 ) ) ;
#26824=PLANE ( 'NONE',  #25810 ) ;
#26827=CARTESIAN_POINT ( 'NONE',  ( 86.91463931152809153, 46.48516107814676701, 8.998642835661645023 ) ) ;
#26829=CARTESIAN_POINT ( 'NONE',  ( 81.72551602421658856, 41.61951536209159741, 5.485699263129209413 ) ) ;
#26834=CARTESIAN_POINT ( 'NONE',  ( 37.49256495613256845, 26.81029122506297568, 8.090169943749479842 ) ) ;
#26848=CARTESIAN_POINT ( 'NONE',  ( 39.81344631580554250, 23.39040679176985904, -6.890680421881970419E-14 ) ) ;
#26853=CARTESIAN_POINT ( 'NONE',  ( 67.04979016446885964, 67.03861818912726278, -8.640631002729076471 ) ) ;
#26854=VERTEX_POINT ( 'NONE', #45232 ) ;
#26858=CARTESIAN_POINT ( 'NONE',  ( 28.45357225853751260, 28.37878583063842441, 9.188101187500006262 ) ) ;
#26860=CARTESIAN_POINT ( 'NONE',  ( 86.50518482659130370, 47.16427830571769420, -10.09192607653805318 ) ) ;
#26863=CARTESIAN_POINT ( 'NONE',  ( 13.34565549823491004, 29.74646525600389424, 2.839279412974139660 ) ) ;
#26864=CARTESIAN_POINT ( 'NONE',  ( 76.05556955939475472, 60.28745929515056901, 15.74899105576687397 ) ) ;
#26866=CARTESIAN_POINT ( 'NONE',  ( 12.20045371381521626, 28.81751292744055348, -6.180339887498951690 ) ) ;
#26867=EDGE_CURVE ( 'NONE', #26719, #56559, #69525, .T. ) ;
#26875=EDGE_CURVE ( 'NONE', #67548, #11833, #7736, .T. ) ;
#26880=CARTESIAN_POINT ( 'NONE',  ( 66.19894089851189278, 69.19767938403377627, -2.070941327739651339 ) ) ;
#26882=CARTESIAN_POINT ( 'NONE',  ( 68.20887950783240683, 70.50781471800318911, 6.446984873749973067E-06 ) ) ;
#26883=CARTESIAN_POINT ( 'NONE',  ( 77.82180247422382990, 61.41261899432889493, -16.13690189282890941 ) ) ;
#26889=VECTOR ( 'NONE', #28793, 1000.000000000000000 ) ;
#26892=ORIENTED_EDGE ( 'NONE', *, *, #21264, .F. ) ;
#26894=CARTESIAN_POINT ( 'NONE',  ( 37.65389587561885776, 30.24335787977765833, -9.188101187500008038 ) ) ;
#26896=CARTESIAN_POINT ( 'NONE',  ( 75.28544958660151565, 66.51564022635962203, -13.12383671828155407 ) ) ;
#26903=CARTESIAN_POINT ( 'NONE',  ( 79.06560434158508599, 56.99523315522970535, -16.20124195947191126 ) ) ;
#26905=EDGE_LOOP ( 'NONE', ( #79321, #23851, #56130, #57829 ) ) ;
#26907=CARTESIAN_POINT ( 'NONE',  ( 66.90064016111628575, 68.95865979773512322, -2.633467781610826286 ) ) ;
#26913=CARTESIAN_POINT ( 'NONE',  ( 75.59250669426468505, 65.53249472979591417, 13.80495133635462679 ) ) ;
#26919=CARTESIAN_POINT ( 'NONE',  ( 86.14665820123012452, 44.21313626661029872, -5.852833583934166306 ) ) ;
#26920=CYLINDRICAL_SURFACE ( 'NONE', #69125, 16.60714546451156792 ) ;
#26921=DIRECTION ( 'NONE',  ( -0.1039558454088829048, 0.1800568059919617214, 0.9781476007338041345 ) ) ;
#26924=CARTESIAN_POINT ( 'NONE',  ( 73.91315373279360301, 56.96484810097162210, 16.01878388499446615 ) ) ;
#26930=CARTESIAN_POINT ( 'NONE',  ( 79.14312167556931854, 57.64441083166269664, 0.000000000000000000 ) ) ;
#26936=CARTESIAN_POINT ( 'NONE',  ( 23.01911539893306013, 18.45404122711133255, -8.090169943749478065 ) ) ;
#26943=CARTESIAN_POINT ( 'NONE',  ( 82.42646601710040954, 51.29741023544101353, -14.55490622455238992 ) ) ;
#26952=CARTESIAN_POINT ( 'NONE',  ( 20.50317736733639862, 20.03677371833801502, 10.00000000000000533 ) ) ;
#26958=CARTESIAN_POINT ( 'NONE',  ( 73.81127463411883127, 55.52226492712755856, -16.58648971016070561 ) ) ;
#26961=CARTESIAN_POINT ( 'NONE',  ( 74.61640982031720171, 67.04502654152244645, 12.50436240261666576 ) ) ;
#26962=ADVANCED_FACE ( 'NONE', ( #59757 ), #68361, .T. ) ;
#26972=CARTESIAN_POINT ( 'NONE',  ( 33.27084535048209091, 40.18502408145594273, 5.678558825948277544 ) ) ;
#26975=CARTESIAN_POINT ( 'NONE',  ( 39.09967052555147404, 28.28920272979929962, -7.433330006724141015 ) ) ;
#26981=CARTESIAN_POINT ( 'NONE',  ( 14.52619969316804394, 14.10170272979925699, -7.433330006724141015 ) ) ;
#26983=CARTESIAN_POINT ( 'NONE',  ( 14.21828646722447154, 29.18502408145591431, 5.678558825948276656 ) ) ;
#26988=CARTESIAN_POINT ( 'NONE',  ( 25.88782454542109335, 20.11029122506295153, -8.090169943749478065 ) ) ;
#26993=VECTOR ( 'NONE', #8202, 1000.000000000000114 ) ;
#26994=CARTESIAN_POINT ( 'NONE',  ( 66.21641665491797824, 68.54611642907939029, 4.779534852452537841 ) ) ;
#27001=CARTESIAN_POINT ( 'NONE',  ( 85.94067892034982492, 47.59093751143262807, 10.86761488427001687 ) ) ;
#27003=CARTESIAN_POINT ( 'NONE',  ( 77.27978102768229007, 55.00308727795876962, 16.10417966147982582 ) ) ;
#27006=CARTESIAN_POINT ( 'NONE',  ( 77.08943580299947484, 49.61595851769168064, 15.51385818994994459 ) ) ;
#27007=CARTESIAN_POINT ( 'NONE',  ( 79.50011211534433642, 50.05647880806598948, -14.69180297385495670 ) ) ;
#27011=CARTESIAN_POINT ( 'NONE',  ( 80.98820082504030893, 43.58192978494404457, 9.409748623455859828 ) ) ;
#27016=ORIENTED_EDGE ( 'NONE', *, *, #351, .T. ) ;
#27019=CARTESIAN_POINT ( 'NONE',  ( 41.98277471387834225, 25.20801979619931998, -3.090169943749474069 ) ) ;
#27031=CARTESIAN_POINT ( 'NONE',  ( 86.38422984226583878, 43.10374499244417024, 0.3565776162481382738 ) ) ;
#27035=CARTESIAN_POINT ( 'NONE',  ( 23.41017057962146097, 28.91421378149919619, 9.188101187500008038 ) ) ;
#27045=CARTESIAN_POINT ( 'NONE',  ( 38.67678797688638070, 22.73415679381825072, -6.890680421881970419E-14 ) ) ;
#27047=CARTESIAN_POINT ( 'NONE',  ( 10.05297690690921897, 28.73705186507752529, -3.090169943749475845 ) ) ;
#27058=CARTESIAN_POINT ( 'NONE',  ( 82.55891087508022963, 41.03829285859550424, -1.155036376835396839 ) ) ;
#27068=CARTESIAN_POINT ( 'NONE',  ( 71.96766164200448657, 71.97375519272833344, -2.838622940868376077 ) ) ;
#27073=CARTESIAN_POINT ( 'NONE',  ( 74.22912425478418186, 67.87594522781263606, -11.68556788600236374 ) ) ;
#27078=CARTESIAN_POINT ( 'NONE',  ( 79.22574914704958360, 60.04803162267379690, -16.48148452078546100 ) ) ;
#27085=CARTESIAN_POINT ( 'NONE',  ( 79.11036565982459479, 46.22622971652937451, -12.75658226733973066 ) ) ;
#27087=CARTESIAN_POINT ( 'NONE',  ( 74.81832046901196520, 67.48663194201290594, -12.71244991431774984 ) ) ;
#27093=ADVANCED_FACE ( 'NONE', ( #94716 ), #30047, .T. ) ;
#27096=DIRECTION ( 'NONE',  ( -0.2551196190400349950, -0.9669094993746143452, 0.000000000000000000 ) ) ;
#27098=CARTESIAN_POINT ( 'NONE',  ( 16.11390655273756778, 24.70171378149918340, -9.188101187500004485 ) ) ;
#27099=CARTESIAN_POINT ( 'NONE',  ( 78.70378768487077537, 58.88177420653629213, -16.56922034439224234 ) ) ;
#27110=CARTESIAN_POINT ( 'NONE',  ( 81.44281134420617718, 55.17415802334473085, -15.93029283586374412 ) ) ;
#27112=CARTESIAN_POINT ( 'NONE',  ( 69.24454181484452420, 67.43800925919231304, 8.968860985737871161 ) ) ;
#27113=AXIS2_PLACEMENT_3D ( 'NONE', #89922, #40400, #9018 ) ;
#27116=CARTESIAN_POINT ( 'NONE',  ( 83.96855558776917405, 42.91945120030306526, 5.578457850387072980 ) ) ;
#27117=CARTESIAN_POINT ( 'NONE',  ( 79.54380123660683921, 51.49935735363682454, 15.19165240974427000 ) ) ;
#27125=CARTESIAN_POINT ( 'NONE',  ( 5.867642952189433103, 25.16126292948893450, -6.180339887498951690 ) ) ;
#27137=CARTESIAN_POINT ( 'NONE',  ( 82.49529963037764446, 50.53747482938361202, -14.21121686865391354 ) ) ;
#27150=CARTESIAN_POINT ( 'NONE',  ( 82.15942678738257143, 40.67362617692227644, 3.631441412251192880 ) ) ;
#27157=CARTESIAN_POINT ( 'NONE',  ( 70.57887313579936972, 60.86954541810593611, -14.49646675233496218 ) ) ;
#27158=CARTESIAN_POINT ( 'NONE',  ( 9.248262631489305718, 13.84335787977760823, 9.188101187500006262 ) ) ;
#27162=ORIENTED_EDGE ( 'NONE', *, *, #22340, .F. ) ;
#27164=CARTESIAN_POINT ( 'NONE',  ( 78.21652899302088713, 47.47575335428597043, -13.80965570268340414 ) ) ;
#27165=CARTESIAN_POINT ( 'NONE',  ( 76.08212860749918605, 65.40353610076411428, -14.00331547028825518 ) ) ;
#27169=CARTESIAN_POINT ( 'NONE',  ( 85.98998294167898848, 43.32359931212324966, 3.421509554684789567 ) ) ;
#27170=CARTESIAN_POINT ( 'NONE',  ( 88.30125181426937786, 44.32158129576059480, -2.141221342158480923 ) ) ;
#27173=CARTESIAN_POINT ( 'NONE',  ( 66.16284130609386693, 69.32471991931953426, 0.2281878490819576055 ) ) ;
#27183=CARTESIAN_POINT ( 'NONE',  ( 88.18822050095108978, 44.34076438004694154, 2.673349022503985761 ) ) ;
#27186=VECTOR ( 'NONE', #11053, 1000.000000000000114 ) ;
#27187=CARTESIAN_POINT ( 'NONE',  ( 77.19709256177225143, 60.73830195696542233, -15.79962378659312883 ) ) ;
#27188=CARTESIAN_POINT ( 'NONE',  ( 79.85233299459939360, 57.97614157916506628, 16.26679898004111990 ) ) ;
#27189=CARTESIAN_POINT ( 'NONE',  ( 71.25744581038296133, 66.03388063194447000, -11.67341175673348630 ) ) ;
#27192=CARTESIAN_POINT ( 'NONE',  ( 80.63212551389750615, 43.28576471723870611, -9.304653108355022795 ) ) ;
#27197=CARTESIAN_POINT ( 'NONE',  ( 87.76333951327919181, 44.16327574611633366, -4.502641440754712399 ) ) ;
#27199=CARTESIAN_POINT ( 'NONE',  ( 77.61491115650760264, 49.94450177510211830, 15.01392251353181528 ) ) ;
#27201=CARTESIAN_POINT ( 'NONE',  ( 77.26541432047375224, 51.19878943637716873, 15.46470134853914047 ) ) ;
#27205=CARTESIAN_POINT ( 'NONE',  ( 84.81139823732658556, 50.24252652397250785, 13.36660589061055404 ) ) ;
#27207=CARTESIAN_POINT ( 'NONE',  ( 79.33432753241152113, 54.60848390438605549, -15.97798455793337347 ) ) ;
#27208=CARTESIAN_POINT ( 'NONE',  ( 82.12925965045128862, 52.94868272234815265, -15.66193675175870226 ) ) ;
#27223=CARTESIAN_POINT ( 'NONE',  ( 31.37640799630998956, 30.06628583063843507, -9.188101187500006262 ) ) ;
#27224=CARTESIAN_POINT ( 'NONE',  ( 78.92023586790456591, 59.45316570216661489, -16.52216786098995982 ) ) ;
#27225=CARTESIAN_POINT ( 'NONE',  ( 75.74710703992727190, 61.96519950925610942, 15.69174628608256405 ) ) ;
#27227=CARTESIAN_POINT ( 'NONE',  ( 21.92109465949963720, 30.84336893147756697, -7.433330006724137462 ) ) ;
#27231=CARTESIAN_POINT ( 'NONE',  ( 86.41183189003805865, 47.25727891775800771, 10.78350007392548271 ) ) ;
#27232=CARTESIAN_POINT ( 'NONE',  ( 74.15819116760899021, 61.47642609411447268, 15.57054964276887077 ) ) ;
#27236=CARTESIAN_POINT ( 'NONE',  ( 74.95803460708295063, 53.16054836391673177, 16.51037805420591198 ) ) ;
#27237=ORIENTED_EDGE ( 'NONE', *, *, #41670, .T. ) ;
#27238=AXIS2_PLACEMENT_3D ( 'NONE', #6752, #5260, #59934 ) ;
#27244=CARTESIAN_POINT ( 'NONE',  ( 88.00349997577261263, 44.64923112938743088, 4.253506518527973235 ) ) ;
#27250=CARTESIAN_POINT ( 'NONE',  ( 87.84569706029115821, 44.18597558567909545, -4.425511980624547093 ) ) ;
#27254=CARTESIAN_POINT ( 'NONE',  ( 32.78369927745970358, 30.87878583063843863, -9.188101187500006262 ) ) ;
#27255=CARTESIAN_POINT ( 'NONE',  ( 72.17023661803692391, 60.81924424899344928, -14.88691701024394298 ) ) ;
#27261=CARTESIAN_POINT ( 'NONE',  ( 68.21305639376519991, 65.88604169822291112, 10.81547118242297678 ) ) ;
#27263=CARTESIAN_POINT ( 'NONE',  ( 85.73895798293081327, 48.63177274617319057, 12.34992197344710796 ) ) ;
#27266=FACE_OUTER_BOUND ( 'NONE', #91157, .T. ) ;
#27276=ORIENTED_EDGE ( 'NONE', *, *, #89556, .T. ) ;
#27278=CARTESIAN_POINT ( 'NONE',  ( 87.11842579636694950, 45.87328929624024454, -8.641498891285833039 ) ) ;
#27281=CARTESIAN_POINT ( 'NONE',  ( 15.57129692638689633, 14.15404122711132295, 8.090169943749479842 ) ) ;
#27292=CARTESIAN_POINT ( 'NONE',  ( 72.06406741461755416, 69.35207420037858128, -8.748526250032554685 ) ) ;
#27294=CARTESIAN_POINT ( 'NONE',  ( 69.42008239677498693, 62.93315161398718516, -13.66206540601166175 ) ) ;
#27299=CARTESIAN_POINT ( 'NONE',  ( 81.69026040342092188, 48.56800976308773699, 13.34553584479553123 ) ) ;
#27306=CARTESIAN_POINT ( 'NONE',  ( 80.19859069096013116, 50.95987101629014404, 14.90308782861245263 ) ) ;
#27307=CARTESIAN_POINT ( 'NONE',  ( 70.63484837994894860, 70.56325258955124013, -4.892680775417415084 ) ) ;
#27312=LINE ( 'NONE', #42484, #33278 ) ;
#27318=CARTESIAN_POINT ( 'NONE',  ( 74.24838807813938502, 55.19146615926651123, 16.60400907293851347 ) ) ;
#27320=ADVANCED_FACE ( 'NONE', ( #15542 ), #53062, .T. ) ;
#27321=CARTESIAN_POINT ( 'NONE',  ( 38.10324709940346821, 24.12755873383628114, -6.180339887498949025 ) ) ;
#27331=CARTESIAN_POINT ( 'NONE',  ( 86.75161163761312366, 46.45414409713080062, 9.084461998406249350 ) ) ;
#27333=CARTESIAN_POINT ( 'NONE',  ( 71.56491451745446852, 72.38511813685279606, -1.315970478074329764 ) ) ;
#27338=CARTESIAN_POINT ( 'NONE',  ( 38.01218019840322881, 27.11029122506296929, -8.090169943749478065 ) ) ;
#27342=CARTESIAN_POINT ( 'NONE',  ( 74.75130681297544299, 67.15234032204921277, -12.45738157583526373 ) ) ;
#27343=B_SPLINE_SURFACE_WITH_KNOTS ( 'NONE', 3, 1, ( 
 ( #56340, #55822 ),
 ( #62429, #54843 ),
 ( #86816, #10263 ),
 ( #41132, #85824 ),
 ( #19868, #50246 ),
 ( #35546, #3672 ),
 ( #4145, #3190 ),
 ( #73074, #80198 ),
 ( #80706, #90296 ),
 ( #74065, #11282 ),
 ( #64964, #42142 ),
 ( #34073, #28434 ),
 ( #19387, #59316 ),
 ( #66447, #34550 ),
 ( #49262, #95909 ),
 ( #65448, #27468 ),
 ( #43122, #96394 ),
 ( #26958, #96898 ),
 ( #97375, #57841 ),
 ( #35040, #26467 ),
 ( #88821, #10767 ),
 ( #41641, #27941 ),
 ( #72584, #58823 ),
 ( #81200, #57343 ),
 ( #88317, #89785 ),
 ( #20361, #11769 ),
 ( #12263, #5152 ),
 ( #18871, #51232 ),
 ( #89314, #49754 ),
 ( #42632, #50735 ),
 ( #58338, #82200 ) ),
 .UNSPECIFIED., .F., .F., .F.,
 ( 4, 3, 3, 3, 3, 3, 3, 3, 3, 3, 4 ),
 ( 2, 2 ),
 ( 0.000000000000000000, 0.1122669598086892678, 0.2243161639709728983, 0.3396355846219379915, 0.4553962076585332253, 0.5677860799922617163, 0.6749047109689904067, 0.7773884377078581487, 0.8775581155834453195, 0.9782364162378207606, 1.000000000000000000 ),
 ( 0.000000000000000000, 1.000000000000000000 ),
 .UNSPECIFIED. ) ;
#27353=CARTESIAN_POINT ( 'NONE',  ( 67.01113855788433682, 66.95909584220486011, -8.721462188034738716 ) ) ;
#27358=CARTESIAN_POINT ( 'NONE',  ( 27.31210279805776509, 33.95586893147756768, 7.433330006724141015 ) ) ;
#27360=CARTESIAN_POINT ( 'NONE',  ( 86.30977306730703447, 47.58285218899635538, -10.62438056216880611 ) ) ;
#27362=ORIENTED_EDGE ( 'NONE', *, *, #87886, .F. ) ;
#27363=CARTESIAN_POINT ( 'NONE',  ( 17.37926562425035826, 12.96004757982089117, -5.678558825948275768 ) ) ;
#27364=CARTESIAN_POINT ( 'NONE',  ( 30.99507739981537213, 18.86426979415090699, -3.090169943749474069 ) ) ;
#27368=CARTESIAN_POINT ( 'NONE',  ( 77.62509034109919526, 60.55547991676347408, 16.28574085379002412 ) ) ;
#27371=ORIENTED_EDGE ( 'NONE', *, *, #17547, .T. ) ;
#27375=CARTESIAN_POINT ( 'NONE',  ( 66.54075137518582039, 68.81555626029070538, -2.231460399992864829 ) ) ;
#27378=DIRECTION ( 'NONE',  ( -0.4851478631379979034, 0.8403007481384877631, 0.2419218955996582654 ) ) ;
#27379=CARTESIAN_POINT ( 'NONE',  ( 78.17692338680700459, 61.78069039082561886, -15.73643159653562229 ) ) ;
#27392=CARTESIAN_POINT ( 'NONE',  ( 40.09738740370236343, 25.01110640527295104, 2.839279412974134775 ) ) ;
#27394=CARTESIAN_POINT ( 'NONE',  ( 75.32215929224730644, 66.75623307483839142, -12.97587438736732857 ) ) ;
#27404=( BOUNDED_CURVE ( )  B_SPLINE_CURVE ( 2, ( #43027, #5063, #27364, #12676, #27855, #20771, #59737, #21260, #83089, #90197, #13660, #73968, #19775 ),
 .UNSPECIFIED., .F., .T. ) 
 B_SPLINE_CURVE_WITH_KNOTS ( ( 3, 2, 2, 2, 2, 2, 3 ),
 ( 0.5375000000000000888, 0.5400000000000000355, 0.5450000000000000400, 0.5500000000000000444, 0.5550000000000000488, 0.5600000000000000533, 0.5625000000000000000 ),
 .UNSPECIFIED. ) 
 CURVE ( )  GEOMETRIC_REPRESENTATION_ITEM ( )  RATIONAL_B_SPLINE_CURVE ( ( 0.9755282581475767101, 0.9755282581475772652, 1.000000000000000000, 0.9510565162951535312, 1.000000000000000000, 0.9510565162951535312, 1.000000000000000000, 0.9510565162951535312, 1.000000000000000000, 0.9510565162951535312, 1.000000000000000000, 0.9755282581475768211, 0.9755282581475768211 ) ) 
 REPRESENTATION_ITEM ( '' )  );
#27405=CARTESIAN_POINT ( 'NONE',  ( 79.72917429462620476, 56.72943457089122887, -16.18511265363209262 ) ) ;
#27406=CARTESIAN_POINT ( 'NONE',  ( 86.88643351309953289, 43.57251993220791064, -2.221051584189594141 ) ) ;
#27410=CARTESIAN_POINT ( 'NONE',  ( 72.15083153978913799, 69.85550926597292687, -8.070654529112998077 ) ) ;
#27423=ORIENTED_EDGE ( 'NONE', *, *, #56831, .F. ) ;
#27424=CARTESIAN_POINT ( 'NONE',  ( 83.33713981978522156, 44.18474327606488572, -8.510079784887897958 ) ) ;
#27430=CARTESIAN_POINT ( 'NONE',  ( 75.35881874794577584, 64.35819607451507807, 14.30177369286720612 ) ) ;
#27433=CARTESIAN_POINT ( 'NONE',  ( 77.40971008714576840, 60.09314948727423200, 15.95988927257681311 ) ) ;
#27440=CARTESIAN_POINT ( 'NONE',  ( 69.68758890477889167, 70.59674914774343790, 2.763705297544655437 ) ) ;
#27444=CARTESIAN_POINT ( 'NONE',  ( 12.55362526388469746, 30.18080186712592194, 3.090169943749475401 ) ) ;
#27463=CARTESIAN_POINT ( 'NONE',  ( 22.42372293028334340, 18.11029122506294442, -8.090169943749478065 ) ) ;
#27464=CARTESIAN_POINT ( 'NONE',  ( 68.03436534181504669, 65.58245731312226212, -10.28075334492668880 ) ) ;
#27468=CARTESIAN_POINT ( 'NONE',  ( 73.85921800226309131, 55.30839618332183250, -16.11850250866768874 ) ) ;
#27469=B_SPLINE_CURVE_WITH_KNOTS ( 'NONE', 3,
 ( #39542, #31457, #85737, #23860, #48685, #25892 ),
 .UNSPECIFIED., .F., .F.,
 ( 4, 2, 4 ),
 ( 0.000000000000000000, 0.3122824062940924850, 0.6245648125881849699 ),
 .UNSPECIFIED. ) ;
#27473=CARTESIAN_POINT ( 'NONE',  ( 75.23386090781256996, 66.95079165826535927, 12.80542170859955498 ) ) ;
#27482=CARTESIAN_POINT ( 'NONE',  ( 29.36891313204580456, 35.14336893147757479, 7.433330006724141015 ) ) ;
#27485=CARTESIAN_POINT ( 'NONE',  ( 34.14357333472769085, 43.21091486745863364, 7.012934429366973338E-14 ) ) ;
#27488=CARTESIAN_POINT ( 'NONE',  ( 11.06209807803029221, 12.10170272979924988, -7.433330006724141015 ) ) ;
#27490=CARTESIAN_POINT ( 'NONE',  ( 21.25954720759204974, 17.98920272979926338, 7.433330006724137462 ) ) ;
#27497=AXIS2_PLACEMENT_3D ( 'NONE', #69907, #70415, #47608 ) ;
#27501=CARTESIAN_POINT ( 'NONE',  ( 66.56247904705401197, 68.75629519960098435, 4.749523133327839375 ) ) ;
#27502=CARTESIAN_POINT ( 'NONE',  ( 87.39560864876780499, 44.96555158233554295, 6.898727475461874370 ) ) ;
#27504=EDGE_LOOP ( 'NONE', ( #41806, #13303, #61865, #21676 ) ) ;
#27506=DIRECTION ( 'NONE',  ( 0.000000000000000000, 0.4385670422228088450, 0.8986984752829710876 ) ) ;
#27509=CARTESIAN_POINT ( 'NONE',  ( 77.13411046628633017, 54.31893080425083298, 16.04542608317086660 ) ) ;
#27511=ORIENTED_EDGE ( 'NONE', *, *, #87161, .T. ) ;
#27512=CARTESIAN_POINT ( 'NONE',  ( 77.99518601148065500, 61.05539905302716619, -15.87786080876372274 ) ) ;
#27513=CARTESIAN_POINT ( 'NONE',  ( 88.50685567279400345, 43.87431988399859506, -0.03150979628302760099 ) ) ;
#27514=B_SPLINE_CURVE_WITH_KNOTS ( 'NONE', 3,
 ( #58864, #98409, #14286, #81733, #6689, #29487, #28482, #68473, #44172, #51278, #90340, #6184, #50783, #12310, #21393, #82245, #12820, #76115, #36080, #75109, #90842, #29003, #20916, #36575 ),
 .UNSPECIFIED., .F., .F.,
 ( 4, 2, 2, 2, 2, 2, 2, 2, 2, 2, 2, 4 ),
 ( 0.000000000000000000, 0.1249999999999918954, 0.2499999999999837907, 0.3749999999999756861, 0.4374999999999744094, 0.4999999999999731326, 0.5624999999999718003, 0.6249999999999705791, 0.6874999999999692468, 0.7499999999999680256, 0.8749999999999840128, 1.000000000000000000 ),
 .UNSPECIFIED. ) ;
#27515=CARTESIAN_POINT ( 'NONE',  ( 80.90734640522499888, 43.51802416776986604, 9.388539139721732596 ) ) ;
#27516=EDGE_CURVE ( 'NONE', #74992, #59506, #84506, .T. ) ;
#27525=ORIENTED_EDGE ( 'NONE', *, *, #51666, .F. ) ;
#27527=EDGE_LOOP ( 'NONE', ( #98190, #6754, #16953, #86042 ) ) ;
#27533=CARTESIAN_POINT ( 'NONE',  ( 88.45958475239287111, 43.85926912372239883, -0.5941283661710258235 ) ) ;
#27540=CARTESIAN_POINT ( 'NONE',  ( 73.85277556690290623, 58.08781524499210747, -15.86821318995104768 ) ) ;
#27542=CARTESIAN_POINT ( 'NONE',  ( 77.45268913986690507, 49.77012986150322149, -14.98312777078430535 ) ) ;
#27566=CARTESIAN_POINT ( 'NONE',  ( 13.14225634397871367, 29.36126292948895156, 6.180339887498949913 ) ) ;
#27589=ADVANCED_FACE ( 'NONE', ( #46962 ), #99789, .T. ) ;
#27601=CARTESIAN_POINT ( 'NONE',  ( 25.46698091360950045, 30.10171378149919974, 9.188101187500008038 ) ) ;
#27605=CARTESIAN_POINT ( 'NONE',  ( 75.29614551415185986, 66.72342768736930907, 13.41754944753248324 ) ) ;
#27612=CARTESIAN_POINT ( 'NONE',  ( 81.37674444193763179, 55.19836804271280073, -15.94010240901345909 ) ) ;
#27614=CARTESIAN_POINT ( 'NONE',  ( 69.29409999990139113, 67.53033690639284714, 8.887769012565335913 ) ) ;
#27617=CARTESIAN_POINT ( 'NONE',  ( 83.19806100981892882, 42.06058512007242456, 4.429552854493146619 ) ) ;
#27620=CARTESIAN_POINT ( 'NONE',  ( 70.31263914188156150, 71.26601167383878987, 0.5666459716601885965 ) ) ;
#27626=CARTESIAN_POINT ( 'NONE',  ( 5.625422033609194017, 26.18080186712590773, 3.090169943749475401 ) ) ;
#27630=EDGE_CURVE ( 'NONE', #63867, #9557, #60884, .T. ) ;
#27634=CARTESIAN_POINT ( 'NONE',  ( 78.76778807799331616, 60.01474888753965331, 16.11287639625045287 ) ) ;
#27635=CYLINDRICAL_SURFACE ( 'NONE', #7104, 10.00000000000001066 ) ;
#27640=CARTESIAN_POINT ( 'NONE',  ( 83.81360984122501634, 50.06911063634414916, -13.60028881744086604 ) ) ;
#27643=EDGE_LOOP ( 'NONE', ( #87273, #95, #70590, #72914 ) ) ;
#27648=VERTEX_POINT ( 'NONE', #91480 ) ;
#27651=VERTEX_POINT ( 'NONE', #52942 ) ;
#27652=CARTESIAN_POINT ( 'NONE',  ( 80.66432953410600248, 43.23603845041665750, -9.222336552745701965 ) ) ;
#27654=CARTESIAN_POINT ( 'NONE',  ( 85.88522298860537774, 42.48983236706607158, -1.987639973148706440 ) ) ;
#27655=EDGE_CURVE ( 'NONE', #50908, #16006, #94863, .T. ) ;
#27661=CARTESIAN_POINT ( 'NONE',  ( 11.67313376208573139, 15.24335787977761747, -9.188101187500008038 ) ) ;
#27665=ORIENTED_EDGE ( 'NONE', *, *, #55435, .T. ) ;
#27668=CARTESIAN_POINT ( 'NONE',  ( 76.27995519852129291, 65.06343769965553747, -14.23913457056448451 ) ) ;
#27671=CARTESIAN_POINT ( 'NONE',  ( 70.76455878343632833, 60.85362355774473997, 14.54687513196817861 ) ) ;
#27674=CARTESIAN_POINT ( 'NONE',  ( 85.45242742188823115, 42.84966524789818010, 2.600776799952281504 ) ) ;
#27675=CARTESIAN_POINT ( 'NONE',  ( 88.30346302270005765, 44.31045525142044994, -2.071979982890664651 ) ) ;
#27678=CARTESIAN_POINT ( 'NONE',  ( 66.37277438342361791, 68.89659095610979023, 0.08793121599326786386 ) ) ;
#27683=CARTESIAN_POINT ( 'NONE',  ( 80.79863759358339337, 44.88662211388689371, -10.92354475286181525 ) ) ;
#27686=CARTESIAN_POINT ( 'NONE',  ( 88.46324942983896733, 43.96425106107525949, 1.817931795122156080 ) ) ;
#27689=ORIENTED_EDGE ( 'NONE', *, *, #87804, .T. ) ;
#27690=CARTESIAN_POINT ( 'NONE',  ( 76.06646813575576971, 61.15541120234568240, -15.53810128048082539 ) ) ;
#27692=CARTESIAN_POINT ( 'NONE',  ( 70.44830684995079650, 66.16034588321909382, -11.13951868050791383 ) ) ;
#27696=CARTESIAN_POINT ( 'NONE',  ( 80.86920046867821554, 43.29757878561761686, -9.961566104854268744 ) ) ;
#27705=CARTESIAN_POINT ( 'NONE',  ( 77.43171394984256040, 51.88891212959239851, 15.61825462552096333 ) ) ;
#27709=CARTESIAN_POINT ( 'NONE',  ( 84.82554225155547556, 50.21385520134798242, 13.77498508261128407 ) ) ;
#27712=LINE ( 'NONE', #36785, #23887 ) ;
#27717=CARTESIAN_POINT ( 'NONE',  ( 85.83204607333262004, 42.89671213125961913, -1.490302785022404430 ) ) ;
#27718=CARTESIAN_POINT ( 'NONE',  ( 75.60765592493140730, 65.32810859375902623, 14.31319638027754237 ) ) ;
#27720=CARTESIAN_POINT ( 'NONE',  ( 30.81771801958594281, 39.83396525600392835, -2.839279412974133887 ) ) ;
#27724=CARTESIAN_POINT ( 'NONE',  ( 19.06802872841732466, 31.98502408145592568, -5.678558825948271327 ) ) ;
#27725=DIRECTION ( 'NONE',  ( -0.5000000000000016653, 0.8660254037844375974, 0.000000000000000000 ) ) ;
#27727=CARTESIAN_POINT ( 'NONE',  ( 70.92041665751398227, 60.95568174592694533, 14.54198497113668864 ) ) ;
#27731=CARTESIAN_POINT ( 'NONE',  ( 87.43197870664040749, 44.84778077074484770, -6.629285647492168643 ) ) ;
#27734=CARTESIAN_POINT ( 'NONE',  ( 28.12636825332733537, 17.20801979619929512, -3.090169943749474069 ) ) ;
#27739=CARTESIAN_POINT ( 'NONE',  ( 86.02466929436550913, 43.73270210902676780, 4.814314935600976675 ) ) ;
#27742=CARTESIAN_POINT ( 'NONE',  ( 85.73021612718905260, 42.77422022262896206, 0.5906291777517241881 ) ) ;
#27744=CARTESIAN_POINT ( 'NONE',  ( 72.07419404290544662, 71.65773480557935216, 5.498832909113059664 ) ) ;
#27747=CARTESIAN_POINT ( 'NONE',  ( 88.18429177444041045, 44.53138063026126048, -4.871266200417315950 ) ) ;
#27748=CARTESIAN_POINT ( 'NONE',  ( 80.96506752577832344, 55.91141337780396015, 16.08528190432092231 ) ) ;
#27749=CARTESIAN_POINT ( 'NONE',  ( 33.49697393745356777, 27.84335787977765264, 9.188101187500006262 ) ) ;
#27755=ORIENTED_EDGE ( 'NONE', *, *, #4916, .F. ) ;
#27759=CARTESIAN_POINT ( 'NONE',  ( 85.81856918057869166, 48.58455003273027017, 12.27698013059672455 ) ) ;
#27760=CARTESIAN_POINT ( 'NONE',  ( 66.08737768631668530, 68.54322828898675368, -2.301609525100600795 ) ) ;
#27764=CARTESIAN_POINT ( 'NONE',  ( 78.99848661620951873, 60.24637179098722584, -16.44349368446545867 ) ) ;
#27772=CARTESIAN_POINT ( 'NONE',  ( 87.12765551004491726, 46.34683270939126487, -8.629118549295082374 ) ) ;
#27773=CARTESIAN_POINT ( 'NONE',  ( 72.02063440569831698, 59.20206202002285067, 15.36478115506978881 ) ) ;
#27775=CARTESIAN_POINT ( 'NONE',  ( 17.56085832715719164, 11.10801979619927948, 3.090169943749476733 ) ) ;
#27778=ORIENTED_EDGE ( 'NONE', *, *, #59259, .F. ) ;
#27779=ADVANCED_FACE ( 'NONE', ( #41224 ), #34153, .T. ) ;
#27780=ORIENTED_EDGE ( 'NONE', *, *, #34423, .F. ) ;
#27788=CARTESIAN_POINT ( 'NONE',  ( 83.95007842832860945, 49.47769780624822999, 13.19600533624758043 ) ) ;
#27794=CARTESIAN_POINT ( 'NONE',  ( 71.64910063594055600, 63.27319121282799586, 13.65625867040954233 ) ) ;
#27795=CARTESIAN_POINT ( 'NONE',  ( 82.20602006260367034, 40.68642891347821688, -3.576342120315587181 ) ) ;
#27798=CARTESIAN_POINT ( 'NONE',  ( 76.04745143182429956, 51.22931105158178866, -16.11652841588801621 ) ) ;
#27799=CARTESIAN_POINT ( 'NONE',  ( 82.18336151548079727, 40.66633616100362758, -3.549285645192841621 ) ) ;
#27801=CARTESIAN_POINT ( 'NONE',  ( 79.67207043538442690, 48.87950828229436695, 14.12217693801051333 ) ) ;
#27802=EDGE_CURVE ( 'NONE', #17891, #67005, #65046, .T. ) ;
#27804=CARTESIAN_POINT ( 'NONE',  ( 19.38736881444313198, 23.14441083166260782, 10.00000000000000533 ) ) ;
#27805=CARTESIAN_POINT ( 'NONE',  ( 77.67488635742661529, 61.95705115926814699, 15.64220015554268173 ) ) ;
#27807=CARTESIAN_POINT ( 'NONE',  ( 69.16577226868226091, 70.40701545813222140, -2.181849231202375172 ) ) ;
#27808=CARTESIAN_POINT ( 'NONE',  ( 80.87517248313827167, 58.64441083166272506, 0.000000000000000000 ) ) ;
#27809=CARTESIAN_POINT ( 'NONE',  ( 67.66477494612622934, 65.93994996590180335, 10.43000742999573482 ) ) ;
#27810=CARTESIAN_POINT ( 'NONE',  ( 27.96887745124769253, 39.08080186712594895, -3.090169943749475845 ) ) ;
#27814=CARTESIAN_POINT ( 'NONE',  ( 82.44511272049554407, 43.20545074304087052, -7.784461827744890705 ) ) ;
#27818=B_SPLINE_CURVE_WITH_KNOTS ( 'NONE', 3,
 ( #81752, #75127, #67497, #74134, #66509, #29020, #19451, #97435, #81260, #28005, #91838 ),
 .UNSPECIFIED., .F., .F.,
 ( 4, 2, 2, 2, 1, 4 ),
 ( 0.7748794552007052250, 0.8311595914005293073, 0.8874397276003532786, 0.9155797957002653753, 0.9437198638001773610, 1.000000000000000000 ),
 .UNSPECIFIED. ) ;
#27819=CARTESIAN_POINT ( 'NONE',  ( 86.96880057233924788, 46.02321981727299516, 8.968744825131210519 ) ) ;
#27821=CARTESIAN_POINT ( 'NONE',  ( 72.13778271599493053, 72.31753100054153549, -1.256476775470434237 ) ) ;
#27824=CARTESIAN_POINT ( 'NONE',  ( 86.82393771405537564, 45.90093866298671799, 8.916403221032373594 ) ) ;
#27827=CARTESIAN_POINT ( 'NONE',  ( 38.19650550196953986, 40.79103043416552765, 8.090169943749478065 ) ) ;
#27828=CARTESIAN_POINT ( 'NONE',  ( 81.38228331512368641, 42.18052851754683275, 8.075145019496556387 ) ) ;
#27832=CARTESIAN_POINT ( 'NONE',  ( 68.09634862398104360, 67.84148155887413623, -7.379325992333486184 ) ) ;
#27838=VERTEX_POINT ( 'NONE', #72676 ) ;
#27843=CARTESIAN_POINT ( 'NONE',  ( 67.60658015080353778, 66.82409088742160463, -8.485143750796469320 ) ) ;
#27848=CARTESIAN_POINT ( 'NONE',  ( 28.60632300232807879, 31.91421378149921040, 9.188101187500008038 ) ) ;
#27854=CARTESIAN_POINT ( 'NONE',  ( 14.59716579798650571, 20.37878583063839955, 9.188101187500006262 ) ) ;
#27855=CARTESIAN_POINT ( 'NONE',  ( 29.35192616055884685, 22.11029122506295863, -8.090169943749478065 ) ) ;
#27857=CARTESIAN_POINT ( 'NONE',  ( 11.62691283633230377, 30.21091486745859811, -1.111400068045478839E-16 ) ) ;
#27868=CARTESIAN_POINT ( 'NONE',  ( 65.83016338625502328, 68.95036046686468012, -2.295610735544858283 ) ) ;
#27871=CARTESIAN_POINT ( 'NONE',  ( 78.15719359349522222, 61.55473184547404486, -16.14768920957587284 ) ) ;
#27875=VERTEX_POINT ( 'NONE', #57430 ) ;
#27883=FACE_OUTER_BOUND ( 'NONE', #37070, .T. ) ;
#27889=CARTESIAN_POINT ( 'NONE',  ( 72.50276366761895019, 63.69479216147543355, -13.71156667146904340 ) ) ;
#27891=CARTESIAN_POINT ( 'NONE',  ( 66.18968672761215544, 68.49487770601442094, -4.881532527435783919 ) ) ;
#27900=CARTESIAN_POINT ( 'NONE',  ( 82.41914487369291464, 41.31337197830497132, 3.340431838514237750 ) ) ;
#27904=CARTESIAN_POINT ( 'NONE',  ( 85.88757390701229610, 44.14475701618168557, 5.957954596235570222 ) ) ;
#27906=CARTESIAN_POINT ( 'NONE',  ( 79.28658851328975743, 59.85324873312088556, -16.14828164407633082 ) ) ;
#27907=CARTESIAN_POINT ( 'NONE',  ( 74.20275025028655591, 58.27827946831821748, 15.87466641876757478 ) ) ;
#27909=ORIENTED_EDGE ( 'NONE', *, *, #67258, .T. ) ;
#27919=CIRCLE ( 'NONE', #81420, 15.60714546451156970 ) ;
#27921=CARTESIAN_POINT ( 'NONE',  ( 11.41020553640983515, 28.36126292948894800, 6.180339887498949913 ) ) ;
#27930=CARTESIAN_POINT ( 'NONE',  ( 66.60661563005250230, 67.77273566384381809, -7.043189648893246613 ) ) ;
#27936=CARTESIAN_POINT ( 'NONE',  ( 85.25467255710213976, 43.90411826015589725, 7.227896802836702328 ) ) ;
#27937=CARTESIAN_POINT ( 'NONE',  ( 33.14255420672135699, 18.94473085651394229, 1.475505719884397138E-15 ) ) ;
#27938=CARTESIAN_POINT ( 'NONE',  ( 85.18660547738458888, 49.05202258069147803, 12.45721658011292732 ) ) ;
#27941=CARTESIAN_POINT ( 'NONE',  ( 74.01103629804136119, 55.46278365816274913, -16.11564949998087215 ) ) ;
#27943=CARTESIAN_POINT ( 'NONE',  ( 77.12260313221874242, 61.62046618767455186, 16.01160934822282655 ) ) ;
#27950=CARTESIAN_POINT ( 'NONE',  ( 72.82118101371949592, 71.12637341421533677, -7.461520388884603783 ) ) ;
#27952=CARTESIAN_POINT ( 'NONE',  ( 79.06624833104577021, 60.08073726494826161, 16.12333911585958290 ) ) ;
#27953=CARTESIAN_POINT ( 'NONE',  ( 27.35361640444819287, 37.83396525600391413, -2.839279412974133887 ) ) ;
#27959=CARTESIAN_POINT ( 'NONE',  ( 17.47068606603513530, 15.80170272979925628, 7.433330006724137462 ) ) ;
#27961=CARTESIAN_POINT ( 'NONE',  ( 82.38367100173057622, 53.80119691343342225, 15.85271891126490829 ) ) ;
#27966=CARTESIAN_POINT ( 'NONE',  ( 75.02124847967681376, 53.56804290023246296, -16.54202287972591279 ) ) ;
#27971=CARTESIAN_POINT ( 'NONE',  ( 82.76646413971928951, 40.58977954809799371, 0.9263384072861480245 ) ) ;
#27973=CARTESIAN_POINT ( 'NONE',  ( 66.57026871552700698, 68.76443072711541049, 4.738950751824671848 ) ) ;
#27977=ORIENTED_EDGE ( 'NONE', *, *, #71624, .F. ) ;
#27981=CARTESIAN_POINT ( 'NONE',  ( 87.98594423550160570, 43.75089820288621212, -2.253463800273092676 ) ) ;
#27982=CARTESIAN_POINT ( 'NONE',  ( 80.34499676519902778, 57.43793486056498665, -16.58883017036144381 ) ) ;
#27986=CARTESIAN_POINT ( 'NONE',  ( 83.44610441601685125, 48.89063263195148323, -12.98306697336452409 ) ) ;
#27989=CARTESIAN_POINT ( 'NONE',  ( 81.22596495421952056, 43.17011023298827865, 9.564257120711848970 ) ) ;
#27993=CARTESIAN_POINT ( 'NONE',  ( 73.73381220379675938, 59.87433565520142764, 15.47193064673703411 ) ) ;
#27998=VECTOR ( 'NONE', #54214, 1000.000000000000000 ) ;
#28005=CARTESIAN_POINT ( 'NONE',  ( 88.14265167143706492, 44.20527097481110701, 1.888012356971680683 ) ) ;
#28006=LINE ( 'NONE', #21897, #16936 ) ;
#28008=CARTESIAN_POINT ( 'NONE',  ( 15.05724179552094277, 20.64441083166259716, -10.00000000000000533 ) ) ;
#28015=DIRECTION ( 'NONE',  ( -0.1710100716628374096, 0.2961981327260301833, 0.9396926207859057634 ) ) ;
#28022=ORIENTED_EDGE ( 'NONE', *, *, #18143, .F. ) ;
#28023=CARTESIAN_POINT ( 'NONE',  ( 81.74830055843420951, 52.20847043234677187, -15.07709221969326308 ) ) ;
#28024=CARTESIAN_POINT ( 'NONE',  ( 87.62133583293774564, 45.31115884160845297, -7.293173845241971875 ) ) ;
#28037=CARTESIAN_POINT ( 'NONE',  ( 6.599962460801562791, 15.76159833115048770, -9.594050593750004907 ) ) ;
#28042=ORIENTED_EDGE ( 'NONE', *, *, #83409, .T. ) ;
#28044=CARTESIAN_POINT ( 'NONE',  ( 74.46528254340208264, 68.13939222454926892, -11.57304410484971235 ) ) ;
#28045=CARTESIAN_POINT ( 'NONE',  ( 70.03054751895673746, 71.08012399627183697, -0.1251406234029079911 ) ) ;
#28050=CARTESIAN_POINT ( 'NONE',  ( 73.86461842229320496, 68.29997319365683950, -11.61748300246921417 ) ) ;
#28054=B_SPLINE_CURVE_WITH_KNOTS ( 'NONE', 3,
 ( #50944, #89990, #90503, #42339, #20566, #73269, #27671, #65154, #89513, #72796 ),
 .UNSPECIFIED., .F., .F.,
 ( 4, 2, 2, 2, 4 ),
 ( 0.000000000000000000, 0.2500000000000000000, 0.5000000000000000000, 0.7500000000000000000, 1.000000000000000000 ),
 .UNSPECIFIED. ) ;
#28064=EDGE_CURVE ( 'NONE', #315, #52745, #85167, .T. ) ;
#28066=CARTESIAN_POINT ( 'NONE',  ( 72.55192422928334395, 57.28793452964083599, 16.33633438825195938 ) ) ;
#28067=CARTESIAN_POINT ( 'NONE',  ( 71.56411227120165108, 71.63451761208904145, 3.366307055662708603 ) ) ;
#28068=CARTESIAN_POINT ( 'NONE',  ( 66.06661787456808099, 68.52074721796333279, -4.599897531117440153 ) ) ;
#28072=DIRECTION ( 'NONE',  ( -0.9669094993746144562, 0.2551196190400350505, 0.000000000000000000 ) ) ;
#28075=CARTESIAN_POINT ( 'NONE',  ( 31.93509797303403630, 20.29860640527293825, -2.839279412974138328 ) ) ;
#28081=CARTESIAN_POINT ( 'NONE',  ( 81.64762987783682036, 41.52940341837351923, -5.382017555150636845 ) ) ;
#28082=CARTESIAN_POINT ( 'NONE',  ( 75.19340432564982279, 67.01774300492178327, 13.18884388031393051 ) ) ;
#28083=CARTESIAN_POINT ( 'NONE',  ( 68.43388330429554856, 64.50992442928946957, 12.16968166442065957 ) ) ;
#28087=CARTESIAN_POINT ( 'NONE',  ( 67.78796486963464929, 67.26057969838673500, -8.930145946851032690 ) ) ;
#28091=CARTESIAN_POINT ( 'NONE',  ( 68.76233101952506388, 66.50715880584016304, 9.743774830957411481 ) ) ;
#28095=CARTESIAN_POINT ( 'NONE',  ( 85.51217825735186295, 45.18995095854337762, 8.208790583656876194 ) ) ;
#28100=CARTESIAN_POINT ( 'NONE',  ( 5.882932626810616128, 22.13478043621385893, 8.090169943749478065 ) ) ;
#28102=ORIENTED_EDGE ( 'NONE', *, *, #99272, .F. ) ;
#28104=CARTESIAN_POINT ( 'NONE',  ( 71.80750138150710882, 71.32421890607284354, 5.932341145765938073 ) ) ;
#28106=ORIENTED_EDGE ( 'NONE', *, *, #29269, .T. ) ;
#28114=CARTESIAN_POINT ( 'NONE',  ( 73.41259731428677071, 70.10201033320841191, -9.453773877498623079 ) ) ;
#28116=CARTESIAN_POINT ( 'NONE',  ( 81.22775765764330913, 42.26095023371678394, -7.344287333291148911 ) ) ;
#28120=CARTESIAN_POINT ( 'NONE',  ( 88.49445028879968334, 43.86712364161932243, -9.307608808691473302E-08 ) ) ;
#28129=CARTESIAN_POINT ( 'NONE',  ( 68.20887950783240683, 70.50781471800318911, 6.446984873749973067E-06 ) ) ;
#28130=CARTESIAN_POINT ( 'NONE',  ( 74.67000616351418785, 66.81477949400925809, -13.12245706047551330 ) ) ;
#28138=CARTESIAN_POINT ( 'NONE',  ( 7.601631632957884577, 27.49540643055185285, 3.479690158560446702E-15 ) ) ;
#28139=ORIENTED_EDGE ( 'NONE', *, *, #93977, .F. ) ;
#28147=CARTESIAN_POINT ( 'NONE',  ( 75.97055471119503522, 64.69957879015430535, -14.33112692621818596 ) ) ;
#28154=ORIENTED_EDGE ( 'NONE', *, *, #342, .T. ) ;
#28155=CARTESIAN_POINT ( 'NONE',  ( 72.95830788359974406, 56.77128196665827176, -15.96545419981962333 ) ) ;
#28156=CARTESIAN_POINT ( 'NONE',  ( 65.99695077750568828, 68.68160084762847362, -0.09952674157115595777 ) ) ;
#28162=CARTESIAN_POINT ( 'NONE',  ( 82.41072854848420093, 44.74050089573861300, -9.837669175488398920 ) ) ;
#28165=CARTESIAN_POINT ( 'NONE',  ( 88.21274111123641148, 43.92339361237885242, 2.502205135834632443 ) ) ;
#28172=CARTESIAN_POINT ( 'NONE',  ( 68.63426881352062026, 66.33891898837059387, -9.865409556835679439 ) ) ;
#28179=CARTESIAN_POINT ( 'NONE',  ( 87.74907107289484998, 44.16117455547062320, -4.521424286948812821 ) ) ;
#28181=CARTESIAN_POINT ( 'NONE',  ( 78.39381814541518168, 53.07351838901534080, 15.75876637147476877 ) ) ;
#28184=CARTESIAN_POINT ( 'NONE',  ( 76.51987890029035100, 63.61070592637643983, 14.91914813192731337 ) ) ;
#28190=CARTESIAN_POINT ( 'NONE',  ( 72.21491844529387549, 53.64441083166271085, 0.000000000000000000 ) ) ;
#28192=CARTESIAN_POINT ( 'NONE',  ( 6.943673075435188302, 24.98502408145590437, -5.678558825948271327 ) ) ;
#28198=CARTESIAN_POINT ( 'NONE',  ( 75.74251350868291865, 65.46771939187904366, 14.28157630633085162 ) ) ;
#28200=CARTESIAN_POINT ( 'NONE',  ( 29.08566721201706784, 38.83396525600392124, -2.839279412974133887 ) ) ;
#28202=CARTESIAN_POINT ( 'NONE',  ( 84.07848607763526161, 46.87983176300981114, -11.10104033282832958 ) ) ;
#28204=CARTESIAN_POINT ( 'NONE',  ( 24.63222838094502265, 17.14754757982090894, -5.678558825948276656 ) ) ;
#28211=CARTESIAN_POINT ( 'NONE',  ( 70.36958601292586479, 61.09422941142852892, 14.35025779664269763 ) ) ;
#28214=CARTESIAN_POINT ( 'NONE',  ( 73.42798026292116731, 58.39006275434417859, 16.23893788096608404 ) ) ;
#28217=CARTESIAN_POINT ( 'NONE',  ( 88.29204076689052272, 44.29173939258662074, -2.000454734116386302 ) ) ;
#28218=B_SPLINE_CURVE_WITH_KNOTS ( 'NONE', 3,
 ( #14855, #23444, #76664, #77685, #91398, #29568, #6767, #23949, #53838, #85830, #37645, #54333, #7252, #8268, #99982, #62434 ),
 .UNSPECIFIED., .F., .F.,
 ( 4, 1, 2, 2, 2, 1, 2, 2, 4 ),
 ( 0.000000000000000000, 0.1250000000000024425, 0.1875000000000014433, 0.2500000000000004441, 0.5000000000000011102, 0.6250000000000014433, 0.6875000000000021094, 0.7500000000000027756, 1.000000000000000000 ),
 .UNSPECIFIED. ) ;
#28219=EDGE_LOOP ( 'NONE', ( #27755, #16560, #79516, #67504 ) ) ;
#28223=CARTESIAN_POINT ( 'NONE',  ( 81.37287889836444776, 42.00540010751133480, -7.805683437329571817 ) ) ;
#28231=CARTESIAN_POINT ( 'NONE',  ( 87.74907107289486419, 44.16117455547063742, -4.521424286948807492 ) ) ;
#28233=CARTESIAN_POINT ( 'NONE',  ( 43.56148901884012048, 27.01110640527296169, 2.839279412974134775 ) ) ;
#28234=CARTESIAN_POINT ( 'NONE',  ( 76.78229342072877728, 59.38575705617227385, -15.96769424347941779 ) ) ;
#28236=CARTESIAN_POINT ( 'NONE',  ( 87.51245999513413665, 45.51585123121132881, 6.985658356529230950 ) ) ;
#28243=CARTESIAN_POINT ( 'NONE',  ( 85.55195523353168596, 48.95437131750654203, -12.20589517503823807 ) ) ;
#28254=CARTESIAN_POINT ( 'NONE',  ( 79.14312167556931854, 57.64441083166269664, 0.000000000000000000 ) ) ;
#28256=ORIENTED_EDGE ( 'NONE', *, *, #95857, .T. ) ;
#28258=CARTESIAN_POINT ( 'NONE',  ( 87.22108034532067222, 46.19249316086605006, -9.000540691006557736 ) ) ;
#28259=EDGE_CURVE ( 'NONE', #47283, #11459, #33101, .T. ) ;
#28265=VERTEX_POINT ( 'NONE', #6313 ) ;
#28270=CARTESIAN_POINT ( 'NONE',  ( 81.74687756906948266, 43.62721439716015936, 8.949604777968817260 ) ) ;
#28272=CARTESIAN_POINT ( 'NONE',  ( 69.44557037078072881, 62.66829723885497572, -13.82623753713334303 ) ) ;
#28277=CARTESIAN_POINT ( 'NONE',  ( 82.22171533294620360, 40.70355118814068618, -3.607997168176046543 ) ) ;
#28282=CARTESIAN_POINT ( 'NONE',  ( 82.28003896795380001, 40.62557011406286733, -3.142018250819525793 ) ) ;
#28284=CARTESIAN_POINT ( 'NONE',  ( 79.39955210850102674, 47.95772480916883040, 13.72164937866508616 ) ) ;
#28285=CARTESIAN_POINT ( 'NONE',  ( 68.01518537448079371, 69.74548201687068172, -1.860190901650351503 ) ) ;
#28288=CARTESIAN_POINT ( 'NONE',  ( 77.72825959162678089, 61.57464001967338163, 16.09025617263268870 ) ) ;
#28298=CARTESIAN_POINT ( 'NONE',  ( 82.78635604014235128, 53.79147356194603447, 15.41260086504908600 ) ) ;
#28307=CARTESIAN_POINT ( 'NONE',  ( 71.85962433970722429, 72.56121191805073067, -1.249447308665279088 ) ) ;
#28310=CARTESIAN_POINT ( 'NONE',  ( 87.35606880162971777, 45.77061481740688009, 8.290963297571636303 ) ) ;
#28313=CARTESIAN_POINT ( 'NONE',  ( 13.25720545158990937, 8.449665230724928477, -2.296566073217252530E-15 ) ) ;
#28317=CARTESIAN_POINT ( 'NONE',  ( 72.98545333942395530, 62.85874912432204553, 14.26892869598277436 ) ) ;
#28318=CARTESIAN_POINT ( 'NONE',  ( 69.04645348238025804, 67.88810431568464310, -8.190965530494443314 ) ) ;
#28322=CARTESIAN_POINT ( 'NONE',  ( 81.91818524605139373, 41.06078777436991345, 3.494940157278100923 ) ) ;
#28337=CARTESIAN_POINT ( 'NONE',  ( 26.01788259378743717, 35.99752408145593563, 5.678558825948277544 ) ) ;
#28342=CARTESIAN_POINT ( 'NONE',  ( 24.68213521633936836, 16.11110640527292759, -2.839279412974138328 ) ) ;
#28350=VECTOR ( 'NONE', #20049, 1000.000000000000114 ) ;
#28356=CARTESIAN_POINT ( 'NONE',  ( 71.96639307748559133, 71.49757472301890004, -5.734781593071435424 ) ) ;
#28358=CARTESIAN_POINT ( 'NONE',  ( 66.22776509639551534, 69.21226861589723001, -2.085083696610475545 ) ) ;
#28369=CARTESIAN_POINT ( 'NONE',  ( 87.63119364650854948, 45.29408460765224476, 6.394950601605615681 ) ) ;
#28371=ORIENTED_EDGE ( 'NONE', *, *, #98837, .F. ) ;
#28381=CARTESIAN_POINT ( 'NONE',  ( 71.07962098583328725, 64.00820346700967889, -13.02735857669132535 ) ) ;
#28385=LINE ( 'NONE', #20814, #92276 ) ;
#28386=CARTESIAN_POINT ( 'NONE',  ( 76.30616544034062088, 50.97262258187969763, -15.53540872755634084 ) ) ;
#28398=CARTESIAN_POINT ( 'NONE',  ( 79.95001512610187433, 44.77191418025095260, -11.25851131356374069 ) ) ;
#28400=CARTESIAN_POINT ( 'NONE',  ( 79.39506416949035383, 59.74337618841887121, -16.16789220604118427 ) ) ;
#28406=CARTESIAN_POINT ( 'NONE',  ( 72.52340034770776356, 71.25924148755669307, -6.049577167954354628 ) ) ;
#28411=CARTESIAN_POINT ( 'NONE',  ( 70.72027907625651721, 71.44976051602542100, 1.172912725620659735 ) ) ;
#28414=CARTESIAN_POINT ( 'NONE',  ( 16.01772687902244741, 32.18080186712592905, 3.090169943749475401 ) ) ;
#28425=CARTESIAN_POINT ( 'NONE',  ( 66.55102321144717337, 67.77113377364665325, -6.986612483274318386 ) ) ;
#28430=CARTESIAN_POINT ( 'NONE',  ( 28.84760059290936951, 18.78380873178787880, -6.180339887498949025 ) ) ;
#28431=CARTESIAN_POINT ( 'NONE',  ( 85.14384985004556938, 49.02042691017501141, 12.45195446300535913 ) ) ;
#28433=CARTESIAN_POINT ( 'NONE',  ( 71.96596176604222705, 72.21842720279319394, -3.609932465874673646 ) ) ;
#28434=CARTESIAN_POINT ( 'NONE',  ( 73.82676074875507766, 55.15409192242278635, -16.12371039794902572 ) ) ;
#28437=CARTESIAN_POINT ( 'NONE',  ( 74.88684299965727575, 67.20604708707715247, 12.50098552432902999 ) ) ;
#28440=ADVANCED_FACE ( 'NONE', ( #29126 ), #92544, .T. ) ;
#28444=EDGE_CURVE ( 'NONE', #7164, #22055, #4622, .T. ) ;
#28446=CARTESIAN_POINT ( 'NONE',  ( 72.85870443091528159, 70.94102631263369574, -7.807649534274237801 ) ) ;
#28447=EDGE_CURVE ( 'NONE', #49096, #7164, #25316, .T. ) ;
#28448=CARTESIAN_POINT ( 'NONE',  ( 79.42893949975002954, 59.60668959204592454, 16.17820502721878739 ) ) ;
#28449=CARTESIAN_POINT ( 'NONE',  ( 42.48198750171711424, 33.03085787977767041, 9.188101187500006262 ) ) ;
#28456=CARTESIAN_POINT ( 'NONE',  ( 17.99030130830579566, 16.10170272979926054, -7.433330006724141015 ) ) ;
#28458=CARTESIAN_POINT ( 'NONE',  ( 83.00815485991435594, 53.30142267139499523, 15.60062745561815944 ) ) ;
#28463=CARTESIAN_POINT ( 'NONE',  ( 41.03800390905408335, 35.64441083166263979, -10.00000000000000533 ) ) ;
#28478=CARTESIAN_POINT ( 'NONE',  ( 88.16692178265705593, 43.83444978110026824, -2.116868534317887462 ) ) ;
#28479=CARTESIAN_POINT ( 'NONE',  ( 80.61280386015431532, 57.63106766464478170, 16.59051181579432210 ) ) ;
#28482=CARTESIAN_POINT ( 'NONE',  ( 87.70143564587257856, 45.35820550660533712, -6.464259315817296958 ) ) ;
#28487=CARTESIAN_POINT ( 'NONE',  ( 74.07498815047767948, 61.33227585059758979, 15.11922174825890863 ) ) ;
#28491=ORIENTED_EDGE ( 'NONE', *, *, #46624, .T. ) ;
#28500=CARTESIAN_POINT ( 'NONE',  ( 82.83837546952335629, 53.74639695667534767, 15.76443799962147096 ) ) ;
#28506=CARTESIAN_POINT ( 'NONE',  ( 80.38715323973768534, 55.64886525756523383, -16.07503577061131139 ) ) ;
#28508=CARTESIAN_POINT ( 'NONE',  ( 33.70846307691164156, 35.16454794089043645, -10.00000000000000355 ) ) ;
#28516=CARTESIAN_POINT ( 'NONE',  ( 70.71838976632287199, 66.47366496125707158, 11.00380527725184088 ) ) ;
#28517=CARTESIAN_POINT ( 'NONE',  ( 86.30490461368275135, 44.79992195346583372, 7.720146956292412987 ) ) ;
#28523=CARTESIAN_POINT ( 'NONE',  ( 84.89294916980452399, 45.33893183262856041, 9.636921286913860740 ) ) ;
#28530=DIRECTION ( 'NONE',  ( -0.4330127018922169113, -0.2500000000000014433, -0.8660254037844393737 ) ) ;
#28541=CARTESIAN_POINT ( 'NONE',  ( 81.84558054786948844, 41.74795303040114192, -5.623115284622243415 ) ) ;
#28548=CARTESIAN_POINT ( 'NONE',  ( 79.21141449090156073, 59.45940664425067723, -16.53580481313993289 ) ) ;
#28554=CARTESIAN_POINT ( 'NONE',  ( 10.80369284495069238, 14.43677371833799405, -10.00000000000000355 ) ) ;
#28556=CARTESIAN_POINT ( 'NONE',  ( 80.36164233910257337, 50.39821764556134553, 15.11645672796150208 ) ) ;
#28558=CARTESIAN_POINT ( 'NONE',  ( 73.39522077465731797, 69.90148087279546019, 9.687480369506271671 ) ) ;
#28559=ADVANCED_FACE ( 'NONE', ( #63001 ), #15663, .T. ) ;
#28563=CARTESIAN_POINT ( 'NONE',  ( 70.95257891153383412, 70.90720881971088829, 4.546241700195112756 ) ) ;
#28564=CARTESIAN_POINT ( 'NONE',  ( 66.10053949976611420, 68.48843487209605030, -4.753018814780690882 ) ) ;
#28569=CARTESIAN_POINT ( 'NONE',  ( 77.32817876982271343, 63.13942984521013813, 15.61058464551962288 ) ) ;
#28571=CARTESIAN_POINT ( 'NONE',  ( 30.43941648770709207, 23.28920272979928541, -7.433330006724141015 ) ) ;
#28577=CARTESIAN_POINT ( 'NONE',  ( 74.74196695595742312, 67.08715363026114176, 12.96493619559571719 ) ) ;
#28578=CARTESIAN_POINT ( 'NONE',  ( 69.02995391522775037, 64.48250336152477757, 12.46069185683908387 ) ) ;
#28586=CARTESIAN_POINT ( 'NONE',  ( 71.35764812850149497, 70.85251640463194178, 5.283905016801779375 ) ) ;
#28588=CARTESIAN_POINT ( 'NONE',  ( 85.82462382841984549, 45.79497946314377543, 8.828125997675229542 ) ) ;
#28591=CARTESIAN_POINT ( 'NONE',  ( 69.04595564537558516, 70.27680155102625292, 2.523699088812808355 ) ) ;
#28595=CARTESIAN_POINT ( 'NONE',  ( 6.768841761084057218, 28.00034080476288878, -1.878358725466461243E-16 ) ) ;
#28601=ORIENTED_EDGE ( 'NONE', *, *, #59058, .T. ) ;
#28608=ORIENTED_EDGE ( 'NONE', *, *, #98906, .F. ) ;
#28613=CARTESIAN_POINT ( 'NONE',  ( 81.41336698633861602, 41.94612678490528168, -7.669352666741279911 ) ) ;
#28621=CARTESIAN_POINT ( 'NONE',  ( 76.08510198875326580, 64.37462812208569574, 14.47852601845500509 ) ) ;
#28627=CARTESIAN_POINT ( 'NONE',  ( 28.50119043139559238, 18.58380873178787951, 6.180339887498953466 ) ) ;
#28628=LINE ( 'NONE', #71890, #64014 ) ;
#28630=CARTESIAN_POINT ( 'NONE',  ( 76.20553726834548058, 57.21450367305868667, 16.12638719470323778 ) ) ;
#28631=CARTESIAN_POINT ( 'NONE',  ( 11.06209807803029221, 12.10170272979924988, -7.433330006724141015 ) ) ;
#28632=ORIENTED_EDGE ( 'NONE', *, *, #50952, .T. ) ;
#28644=CARTESIAN_POINT ( 'NONE',  ( 86.51306616006753814, 43.84325935889563652, 4.272406052666638310 ) ) ;
#28645=CARTESIAN_POINT ( 'NONE',  ( 88.24590225192910964, 44.24085665668349776, -1.852495053617905230 ) ) ;
#28648=CARTESIAN_POINT ( 'NONE',  ( 74.86346538573359055, 67.47285165321515876, -12.74145591711592118 ) ) ;
#28654=CARTESIAN_POINT ( 'NONE',  ( 84.23654874160455108, 44.64216667711589537, -8.426356101742397797 ) ) ;
#28657=CARTESIAN_POINT ( 'NONE',  ( 76.19402696226363503, 65.29190987809512592, 14.49924708549197483 ) ) ;
#28660=B_SPLINE_CURVE_WITH_KNOTS ( 'NONE', 3,
 ( #37889, #68797, #76898, #44995, #99725, #14117, #52595, #52104, #44496, #61196 ),
 .UNSPECIFIED., .F., .F.,
 ( 4, 2, 2, 2, 4 ),
 ( 0.000000000000000000, 0.2500000000000000000, 0.5000000000000000000, 0.7500000000000000000, 1.000000000000000000 ),
 .UNSPECIFIED. ) ;
#28665=CARTESIAN_POINT ( 'NONE',  ( 85.57852021786813168, 48.96074862228688573, -12.66870494374460776 ) ) ;
#28667=CARTESIAN_POINT ( 'NONE',  ( 87.14756827322403865, 44.11579270599533942, 4.133463102786264720 ) ) ;
#28668=CARTESIAN_POINT ( 'NONE',  ( 85.00801151538682632, 48.68758372926721023, 12.25568936537549902 ) ) ;
#28670=B_SPLINE_CURVE_WITH_KNOTS ( 'NONE', 3,
 ( #22017, #100036, #77735, #84853, #99042, #54905, #24007, #31101, #61988, #83866, #38704, #13929, #46288, #54385, #30118, #53894, #15395, #53410, #45311, #29625, #44805, #69612, #75742, #14907, #38193, #45797, #37216, #76247, #85359, #37704, #68116, #92941, #68612, #61000, #46812, #60498, #91971, #76718, #69109, #30623, #92457, #23002, #48832, #80262, #86377, #1221 ),
 .UNSPECIFIED., .F., .F.,
 ( 4, 1, 2, 2, 1, 2, 2, 1, 1, 2, 2, 1, 1, 2, 2, 1, 1, 2, 2, 1, 1, 1, 2, 2, 1, 1, 1, 2, 2, 4 ),
 ( 0.000000000000000000, 0.06249999999998609446, 0.09374999999998014089, 0.1249999999999741873, 0.1874999999999622802, 0.2187499999999571176, 0.2499999999999519829, 0.3124999999999434896, 0.3437499999999402700, 0.3593749999999396039, 0.3749999999999388822, 0.4374999999999416023, 0.4687499999999439892, 0.4843749999999444333, 0.4999999999999448219, 0.5624999999999447109, 0.5937499999999434896, 0.6093749999999437117, 0.6249999999999438227, 0.6874999999999463762, 0.7187499999999478195, 0.7343749999999483746, 0.7421874999999488187, 0.7499999999999491518, 0.8124999999999610312, 0.8437499999999665823, 0.8593749999999694689, 0.8671874999999716893, 0.8749999999999739098, 1.000000000000000000 ),
 .UNSPECIFIED. ) ;
#28673=CARTESIAN_POINT ( 'NONE',  ( 75.28650001057751240, 66.67572118895704136, 13.44401380721711270 ) ) ;
#28675=CARTESIAN_POINT ( 'NONE',  ( 79.34762228877008283, 58.72377720057313866, 16.21937645494816849 ) ) ;
#28678=CARTESIAN_POINT ( 'NONE',  ( 82.92870420767373218, 52.52116137057526402, -14.95649373007994498 ) ) ;
#28686=B_SPLINE_CURVE_WITH_KNOTS ( 'NONE', 3,
 ( #16020, #31213, #38810, #69716, #62099, #25112, #70207, #17519, #55011, #77841, #93046, #47901, #17011, #94556, #78338, #94063 ),
 .UNSPECIFIED., .F., .F.,
 ( 4, 1, 2, 2, 2, 1, 2, 2, 4 ),
 ( 0.000000000000000000, 0.1250000000000011657, 0.1875000000000017486, 0.2500000000000023315, 0.5000000000000039968, 0.6250000000000033307, 0.6875000000000033307, 0.7500000000000032196, 1.000000000000000000 ),
 .UNSPECIFIED. ) ;
#28687=CARTESIAN_POINT ( 'NONE',  ( 84.13554962843576845, 50.44679214584963489, 13.72453037626170058 ) ) ;
#28697=EDGE_CURVE ( 'NONE', #50302, #50839, #74504, .T. ) ;
#28698=CARTESIAN_POINT ( 'NONE',  ( 6.194340351808173217, 26.68290643055185285, 3.479690158560446702E-15 ) ) ;
#28704=CARTESIAN_POINT ( 'NONE',  ( 75.99079911453461023, 65.46731794264749738, 14.35477091480207612 ) ) ;
#28706=CARTESIAN_POINT ( 'NONE',  ( 41.44275701717578642, 32.43085787977767609, -9.188101187500008038 ) ) ;
#28708=FACE_BOUND ( 'NONE', #80870, .T. ) ;
#28709=ORIENTED_EDGE ( 'NONE', *, *, #28064, .T. ) ;
#28710=CARTESIAN_POINT ( 'NONE',  ( 18.97660828663255117, 29.14336893147755703, 7.433330006724141015 ) ) ;
#28719=CARTESIAN_POINT ( 'NONE',  ( 70.98043770365947580, 61.04086187986361978, 14.52140827553137470 ) ) ;
#28729=CARTESIAN_POINT ( 'NONE',  ( 69.61542750552385428, 62.56132062511078828, -13.94275833699888700 ) ) ;
#28732=CARTESIAN_POINT ( 'NONE',  ( 87.83526388831070619, 44.46237794634081553, 3.930408651391872343 ) ) ;
#28733=ORIENTED_EDGE ( 'NONE', *, *, #60320, .T. ) ;
#28736=CARTESIAN_POINT ( 'NONE',  ( 84.74507488503365948, 50.24295689512916141, 13.81875560728438224 ) ) ;
#28740=CARTESIAN_POINT ( 'NONE',  ( 44.10936046141050326, 26.26216523072498532, -2.296566073217252530E-15 ) ) ;
#28741=CARTESIAN_POINT ( 'NONE',  ( 72.02429414335679780, 60.85727294438741808, -14.84082463543404806 ) ) ;
#28744=ORIENTED_EDGE ( 'NONE', *, *, #11365, .T. ) ;
#28746=FACE_OUTER_BOUND ( 'NONE', #20921, .T. ) ;
#28750=CARTESIAN_POINT ( 'NONE',  ( 66.48373673643996540, 68.79225009967480275, -2.167545776629342225 ) ) ;
#28752=FACE_OUTER_BOUND ( 'NONE', #70059, .T. ) ;
#28755=FACE_OUTER_BOUND ( 'NONE', #67536, .T. ) ;
#28764=CARTESIAN_POINT ( 'NONE',  ( 87.13833003848017711, 45.89157147215227894, -8.651152695689850347 ) ) ;
#28776=CARTESIAN_POINT ( 'NONE',  ( 72.46511837996449401, 71.56249752072032777, 6.234640293157917235 ) ) ;
#28780=CARTESIAN_POINT ( 'NONE',  ( 69.59366227530321680, 62.45191379327602732, -13.42933426267537378 ) ) ;
#28786=CARTESIAN_POINT ( 'NONE',  ( 82.27576515736316765, 50.79558287279384388, 14.36463698561768965 ) ) ;
#28790=CARTESIAN_POINT ( 'NONE',  ( 72.14611019483686505, 72.30310738408833515, 3.684292749196569350 ) ) ;
#28793=DIRECTION ( 'NONE',  ( 0.1710100716628310258, -0.2961981327260192476, 0.9396926207859104263 ) ) ;
#28794=CARTESIAN_POINT ( 'NONE',  ( 80.82203068068015739, 54.54264130141514499, 15.85416842091752088 ) ) ;
#28799=CARTESIAN_POINT ( 'NONE',  ( 77.72205534048291042, 61.52847525230062331, 16.09962475150208761 ) ) ;
#28801=CARTESIAN_POINT ( 'NONE',  ( 66.66342508697569258, 67.67433879810246822, 6.129251300726017426 ) ) ;
#28803=CARTESIAN_POINT ( 'NONE',  ( 74.39841895140679640, 68.21392270468032848, 11.95628786500076579 ) ) ;
#28804=CARTESIAN_POINT ( 'NONE',  ( 73.65879925253982208, 69.67557606723219976, -9.540597966332084567 ) ) ;
#28807=CARTESIAN_POINT ( 'NONE',  ( 44.13025152078434132, 25.28848085856235173, 1.475505719884397138E-15 ) ) ;
#28810=CARTESIAN_POINT ( 'NONE',  ( 71.76780065431621836, 72.18842372171909005, 3.264426277842173096 ) ) ;
#28820=CARTESIAN_POINT ( 'NONE',  ( 71.75070072382382591, 72.06332698807560178, -1.650535781253756662 ) ) ;
#28824=CARTESIAN_POINT ( 'NONE',  ( 20.59861825492957621, 33.93396525600390845, 2.839279412974139660 ) ) ;
#28827=CARTESIAN_POINT ( 'NONE',  ( 46.41032958717836010, 27.76426979415094110, 3.090169943749476733 ) ) ;
#28834=CARTESIAN_POINT ( 'NONE',  ( 70.08428920641576099, 67.88371280376459538, -9.044488858928271924 ) ) ;
#28849=VECTOR ( 'NONE', #57931, 1000.000000000000000 ) ;
#28851=CARTESIAN_POINT ( 'NONE',  ( 79.27712787825650764, 45.82676469203064329, -12.41914995154098200 ) ) ;
#28856=ORIENTED_EDGE ( 'NONE', *, *, #56228, .F. ) ;
#28857=B_SPLINE_CURVE_WITH_KNOTS ( 'NONE', 3,
 ( #534, #55212, #16233, #30930, #22333, #92282, #31917, #16730, #62309, #54712, #8139, #31420, #32434, #38520, #14733, #8635, #92764, #38008, #85175, #7629, #84184, #45616, #46620, #69920, #24335, #9136, #22829 ),
 .UNSPECIFIED., .F., .F.,
 ( 4, 2, 2, 2, 1, 1, 2, 2, 1, 2, 2, 1, 2, 2, 1, 4 ),
 ( 0.3033294829601337894, 0.4774971122201073781, 0.4992680658776057490, 0.5101535427063552675, 0.5210390195351046749, 0.5645809268500957545, 0.6081228341650868341, 0.6298937878225825404, 0.6516647414800782467, 0.7387485561100566311, 0.7822904634250469336, 0.8258323707400372360, 0.8693742780550275384, 0.8911452317125228006, 0.9129161853700180629, 1.000000000000000000 ),
 .UNSPECIFIED. ) ;
#28858=CARTESIAN_POINT ( 'NONE',  ( 23.32475077058400004, 14.26216523072494446, -2.296566073217252530E-15 ) ) ;
#28859=CARTESIAN_POINT ( 'NONE',  ( 76.18316680938646357, 61.09795948472795857, 15.59353031967901693 ) ) ;
#28861=CARTESIAN_POINT ( 'NONE',  ( 74.97996761797445231, 67.38724533294663388, -12.85106452774880381 ) ) ;
#28869=CARTESIAN_POINT ( 'NONE',  ( 71.97460576983348801, 66.57329172194043565, 12.17197637779258734 ) ) ;
#28872=CARTESIAN_POINT ( 'NONE',  ( 66.17027418025043062, 69.18316985973861222, -2.056876225022604920 ) ) ;
#28878=FACE_OUTER_BOUND ( 'NONE', #61862, .T. ) ;
#28886=ORIENTED_EDGE ( 'NONE', *, *, #66514, .T. ) ;
#28888=CARTESIAN_POINT ( 'NONE',  ( 75.31813185017509227, 66.77598452293851494, -12.96073926456471881 ) ) ;
#28892=CARTESIAN_POINT ( 'NONE',  ( 81.65957865058895493, 55.81781964966066312, 16.00564737419913186 ) ) ;
#28894=CARTESIAN_POINT ( 'NONE',  ( 72.92667516200663158, 70.31269505470191916, 8.108358915573942838 ) ) ;
#28895=CARTESIAN_POINT ( 'NONE',  ( 87.70668618551661666, 45.11329565042249357, 6.837976445409226223 ) ) ;
#28897=CARTESIAN_POINT ( 'NONE',  ( 73.59724665734155735, 63.41105048715310488, -14.19156318116282378 ) ) ;
#28902=CARTESIAN_POINT ( 'NONE',  ( 72.51315417358483728, 69.83750700119627197, -8.417205730241819950 ) ) ;
#28903=CARTESIAN_POINT ( 'NONE',  ( 76.06215586834144915, 51.32791385274359186, -15.64516872477013365 ) ) ;
#28905=EDGE_CURVE ( 'NONE', #94224, #56024, #93414, .T. ) ;
#28907=CARTESIAN_POINT ( 'NONE',  ( 80.41801566324240014, 54.65175397312741978, 16.29095433313647234 ) ) ;
#28915=CARTESIAN_POINT ( 'NONE',  ( 87.98321614449201888, 44.37542847539244661, 4.756797044073172387 ) ) ;
#28916=CARTESIAN_POINT ( 'NONE',  ( 86.01542015185120249, 44.31831041030510221, 6.184598332866396930 ) ) ;
#28919=CARTESIAN_POINT ( 'NONE',  ( 72.80104277311302496, 70.83185719937777947, 7.190015310759124034 ) ) ;
#28923=CARTESIAN_POINT ( 'NONE',  ( 77.19380876746809861, 58.51342845908217072, 16.11897871819916972 ) ) ;
#28926=CARTESIAN_POINT ( 'NONE',  ( 72.60433947765299934, 71.50525637487901065, -5.566970196651008784 ) ) ;
#28927=CARTESIAN_POINT ( 'NONE',  ( 81.51711570496432557, 54.24218815797082982, 15.69287892032614273 ) ) ;
#28933=CARTESIAN_POINT ( 'NONE',  ( 21.80251038182309387, 34.36126292948896577, 6.180339887498949913 ) ) ;
#28935=CARTESIAN_POINT ( 'NONE',  ( 21.35627990119762032, 12.73415679381821519, 1.333680081654574804E-15 ) ) ;
#28943=CARTESIAN_POINT ( 'NONE',  ( 66.61927972294286349, 68.05145527290748930, -6.517764413741313767 ) ) ;
#28944=CARTESIAN_POINT ( 'NONE',  ( 72.84756190538607257, 70.91156448913385191, -7.844936087786372525 ) ) ;
#28948=CARTESIAN_POINT ( 'NONE',  ( 23.31615823149838462, 29.16454794089042579, -10.00000000000000355 ) ) ;
#28955=CARTESIAN_POINT ( 'NONE',  ( 82.36042285506233895, 42.91861834903688333, 8.349967097983880038 ) ) ;
#28959=CARTESIAN_POINT ( 'NONE',  ( 70.99909089399695006, 61.09348569631758608, 14.50421621802051853 ) ) ;
#28964=CARTESIAN_POINT ( 'NONE',  ( 79.40635770460171727, 59.70624924693522928, 16.17064410388787365 ) ) ;
#28965=CARTESIAN_POINT ( 'NONE',  ( 45.07042791025775585, 28.94754757982093452, 5.678558825948272215 ) ) ;
#28975=CARTESIAN_POINT ( 'NONE',  ( 17.75393198606386136, 12.11110640527291160, -2.839279412974138328 ) ) ;
#28976=CARTESIAN_POINT ( 'NONE',  ( 71.49724145223211735, 72.36708001998829332, 1.062265253749092420 ) ) ;
#28977=CARTESIAN_POINT ( 'NONE',  ( 82.95708619573620979, 53.58516627418447342, 15.69712586674409849 ) ) ;
#28978=CARTESIAN_POINT ( 'NONE',  ( 71.41016749218992743, 59.45273978182969188, 15.69346469621916995 ) ) ;
#28983=CARTESIAN_POINT ( 'NONE',  ( 2.953350652821653988, 23.74646525600387648, 2.839279412974139660 ) ) ;
#28984=CARTESIAN_POINT ( 'NONE',  ( 81.11978968823368064, 42.58148117026868107, 7.963302174025969293 ) ) ;
#28987=CARTESIAN_POINT ( 'NONE',  ( 67.23170740046823823, 69.33908408813277902, 1.348601409716759347 ) ) ;
#28988=CARTESIAN_POINT ( 'NONE',  ( 76.81132113734133782, 63.87275317464699498, 14.88576141942193942 ) ) ;
#28993=LINE ( 'NONE', #84710, #34128 ) ;
#28995=B_SPLINE_CURVE_WITH_KNOTS ( 'NONE', 3,
 ( #12765, #50729, #19381, #12257, #35541, #97370, #73555, #5147, #27936, #89780, #20356, #50240, #51226, #81194, #82194, #36028 ),
 .UNSPECIFIED., .F., .F.,
 ( 4, 1, 2, 2, 2, 1, 2, 2, 4 ),
 ( 0.000000000000000000, 0.1250000000000036360, 0.1875000000000049405, 0.2500000000000062728, 0.5000000000000048850, 0.6250000000000044409, 0.6875000000000039968, 0.7500000000000035527, 1.000000000000000000 ),
 .UNSPECIFIED. ) ;
#28998=CARTESIAN_POINT ( 'NONE',  ( 88.36865033182888851, 43.96674011622069855, -2.220889795100837283 ) ) ;
#28999=CARTESIAN_POINT ( 'NONE',  ( 80.50291573656390653, 57.83591419990552396, 16.24909409233076119 ) ) ;
#29003=CARTESIAN_POINT ( 'NONE',  ( 87.34722152284756191, 44.99461385121256285, -6.156066689881265930 ) ) ;
#29019=CARTESIAN_POINT ( 'NONE',  ( 81.62548306449865265, 50.91212887389385600, -15.04074333791695572 ) ) ;
#29020=CARTESIAN_POINT ( 'NONE',  ( 87.75573343511427993, 43.92582870660319827, 1.242921438624202901 ) ) ;
#29027=ORIENTED_EDGE ( 'NONE', *, *, #2276, .F. ) ;
#29028=CARTESIAN_POINT ( 'NONE',  ( 74.41611649102104309, 57.90871829712388319, -15.94991086904226663 ) ) ;
#29037=CARTESIAN_POINT ( 'NONE',  ( 78.05657720352552076, 53.54917886275364225, -15.89405086258497235 ) ) ;
#29039=CARTESIAN_POINT ( 'NONE',  ( 79.43493723186259103, 45.78179558321050990, 12.93201222421020447 ) ) ;
#29043=CYLINDRICAL_SURFACE ( 'NONE', #95213, 10.00000000000001066 ) ;
#29046=CARTESIAN_POINT ( 'NONE',  ( 85.08842198125357470, 45.78556742147969771, 10.02268771122703050 ) ) ;
#29052=CARTESIAN_POINT ( 'NONE',  ( 66.22544472841278207, 69.36168339246577830, 0.1681495645362227065 ) ) ;
#29058=VECTOR ( 'NONE', #76550, 1000.000000000000000 ) ;
#29062=CARTESIAN_POINT ( 'NONE',  ( 70.43250933021919025, 71.30870369305561951, -0.6892231058542993560 ) ) ;
#29064=CARTESIAN_POINT ( 'NONE',  ( 81.85620833974131472, 41.16559107020475494, -5.619287453036919011 ) ) ;
#29067=CARTESIAN_POINT ( 'NONE',  ( 74.14312167556930433, 66.30466486950707861, 1.224646799147354045E-15 ) ) ;
#29070=B_SPLINE_SURFACE_WITH_KNOTS ( 'NONE', 3, 1, ( 
 ( #23711, #39903 ),
 ( #53617, #15111 ),
 ( #8534, #69329 ),
 ( #14637, #46004 ),
 ( #76922, #61221 ),
 ( #92665, #31322 ),
 ( #93670, #7521 ),
 ( #93161, #38414 ),
 ( #935, #99746 ),
 ( #55112, #30331 ),
 ( #37909, #86099 ),
 ( #92185, #32327 ),
 ( #16130, #100250 ),
 ( #7025, #30832 ),
 ( #23218, #47028 ),
 ( #77945, #39406 ),
 ( #70321, #9031 ),
 ( #24722, #31811 ),
 ( #85064, #15612 ),
 ( #62711, #77448 ),
 ( #46510, #8044 ),
 ( #24234, #16625 ),
 ( #63228, #94170 ),
 ( #47521, #78449 ),
 ( #45517, #70835 ),
 ( #1447, #76448 ),
 ( #55605, #19031 ),
 ( #26611, #66598 ),
 ( #5305, #58483 ),
 ( #17124, #4816 ),
 ( #57487, #78963 ) ),
 .UNSPECIFIED., .F., .F., .F.,
 ( 4, 3, 3, 3, 3, 3, 3, 3, 3, 3, 4 ),
 ( 2, 2 ),
 ( 0.000000000000000000, 0.1122669598086679377, 0.2243161639709564115, 0.3396355846218893637, 0.4553962076585015284, 0.5677860799922294088, 0.6749047109689492174, 0.7773884377078165153, 0.8775581155833958036, 0.9782364162377762407, 1.000000000000000000 ),
 ( 0.000000000000000000, 1.000000000000000000 ),
 .UNSPECIFIED. ) ;
#29072=CARTESIAN_POINT ( 'NONE',  ( 79.31081143133006606, 59.61002059306026268, -16.52811874246031465 ) ) ;
#29075=AXIS2_PLACEMENT_3D ( 'NONE', #18522, #88472, #19034 ) ;
#29077=CARTESIAN_POINT ( 'NONE',  ( 11.84292332949202020, 15.03677371833799903, 10.00000000000000533 ) ) ;
#29079=CARTESIAN_POINT ( 'NONE',  ( 71.65615954623328321, 59.54154983785703337, -15.70934178226849731 ) ) ;
#29084=CARTESIAN_POINT ( 'NONE',  ( 72.49015541307309718, 57.42129546939775508, 15.82701281140211691 ) ) ;
#29085=CARTESIAN_POINT ( 'NONE',  ( 67.96351782124591523, 66.04854104595484898, 9.746239896112580681 ) ) ;
#29087=VERTEX_POINT ( 'NONE', #76485 ) ;
#29091=CARTESIAN_POINT ( 'NONE',  ( 19.06802872841732466, 31.98502408145592568, -5.678558825948271327 ) ) ;
#29095=CARTESIAN_POINT ( 'NONE',  ( 88.23680129110753967, 43.93620611740951176, 2.496076054743395556 ) ) ;
#29096=CARTESIAN_POINT ( 'NONE',  ( 75.28650001057752661, 66.67572118895705557, 13.44401380721711270 ) ) ;
#29097=CARTESIAN_POINT ( 'NONE',  ( 68.97219946460526785, 64.39425464503430874, 12.50242288874033392 ) ) ;
#29102=CARTESIAN_POINT ( 'NONE',  ( 81.82036482989325066, 42.35048943672428834, -7.944650131338364396 ) ) ;
#29103=FACE_OUTER_BOUND ( 'NONE', #91220, .T. ) ;
#29106=CARTESIAN_POINT ( 'NONE',  ( 69.66188720561194714, 68.19766641142308572, 8.278177376932148945 ) ) ;
#29108=CARTESIAN_POINT ( 'NONE',  ( 82.21410988452117863, 40.73976263626466476, 3.762362152834610729 ) ) ;
#29114=CARTESIAN_POINT ( 'NONE',  ( 8.500892568652933079, 29.00034080476289233, -1.878358725466461243E-16 ) ) ;
#29120=CARTESIAN_POINT ( 'NONE',  ( 80.06222361221591655, 45.69665893710951821, -11.99569225509787351 ) ) ;
#29124=DIRECTION ( 'NONE',  ( 0.9619696745371171254, -0.2731562652969042326, 0.000000000000000000 ) ) ;
#29126=FACE_OUTER_BOUND ( 'NONE', #6547, .T. ) ;
#29131=CARTESIAN_POINT ( 'NONE',  ( 81.27662216513620308, 42.46107531295264437, -7.622153486729677851 ) ) ;
#29132=VERTEX_POINT ( 'NONE', #49076 ) ;
#29136=CARTESIAN_POINT ( 'NONE',  ( 81.59591673450252358, 50.88875380172861185, 14.58497109559629479 ) ) ;
#29144=CARTESIAN_POINT ( 'NONE',  ( 82.69964235597838353, 53.57960405717556540, -15.73923566368025995 ) ) ;
#29147=CARTESIAN_POINT ( 'NONE',  ( 66.00490917976195249, 68.68606793243894515, -0.05709965366314424112 ) ) ;
#29148=CARTESIAN_POINT ( 'NONE',  ( 15.30080465516770616, 11.76004757982088300, 5.678558825948272215 ) ) ;
#29156=DIRECTION ( 'NONE',  ( 0.7713975076906492978, 0.000000000000000000, -0.6363535849892373308 ) ) ;
#29162=CARTESIAN_POINT ( 'NONE',  ( 69.69046828898208901, 63.66106611675193250, -12.72546107364192913 ) ) ;
#29170=CARTESIAN_POINT ( 'NONE',  ( 82.47404279536071670, 44.73581219917306839, -9.792184509178092355 ) ) ;
#29176=ORIENTED_EDGE ( 'NONE', *, *, #56808, .F. ) ;
#29183=( BOUNDED_CURVE ( )  B_SPLINE_CURVE ( 2, ( #71478, #69945, #61348, #78071, #9161, #84698, #31444, #93290, #40037, #31943, #32462, #94298, #70876 ),
 .UNSPECIFIED., .F., .T. ) 
 B_SPLINE_CURVE_WITH_KNOTS ( ( 3, 2, 2, 2, 2, 2, 3 ),
 ( 0.9375000000000000000, 0.9399999999999999467, 0.9449999999999999512, 0.9499999999999999556, 0.9549999999999999600, 0.9599999999999999645, 0.9625000000000000222 ),
 .UNSPECIFIED. ) 
 CURVE ( )  GEOMETRIC_REPRESENTATION_ITEM ( )  RATIONAL_B_SPLINE_CURVE ( ( 0.9755282581475768211, 0.9755282581475768211, 1.000000000000000000, 0.9510565162951535312, 1.000000000000000000, 0.9510565162951535312, 1.000000000000000000, 0.9510565162951535312, 1.000000000000000000, 0.9510565162951535312, 1.000000000000000000, 0.9755282581475761550, 0.9755282581475767101 ) ) 
 REPRESENTATION_ITEM ( '' )  );
#29191=CARTESIAN_POINT ( 'NONE',  ( 79.20958550591666381, 57.62938875652737636, 16.22140153437238297 ) ) ;
#29193=CARTESIAN_POINT ( 'NONE',  ( 76.71058889096842393, 54.71840718949849958, -16.09767432139937782 ) ) ;
#29196=CARTESIAN_POINT ( 'NONE',  ( 83.03373565306426940, 49.73266685372522744, 14.08671670346445204 ) ) ;
#29198=CARTESIAN_POINT ( 'NONE',  ( 84.79185039598577589, 50.39256584352096269, 13.46671255472566564 ) ) ;
#29201=CYLINDRICAL_SURFACE ( 'NONE', #75518, 10.00000000000001066 ) ;
#29206=CARTESIAN_POINT ( 'NONE',  ( 67.74244556568478970, 65.67873629388216727, 10.75033511117075413 ) ) ;
#29215=CARTESIAN_POINT ( 'NONE',  ( 40.22068564906490451, 26.14754757982093381, -5.678558825948275768 ) ) ;
#29217=FACE_BOUND ( 'NONE', #12702, .T. ) ;
#29219=CARTESIAN_POINT ( 'NONE',  ( 27.11361191214091804, 16.44966523072495335, -2.296566073217252530E-15 ) ) ;
#29223=ORIENTED_EDGE ( 'NONE', *, *, #51709, .F. ) ;
#29224=CARTESIAN_POINT ( 'NONE',  ( 70.65976107414203966, 60.91110302911690866, 15.02673238886433893 ) ) ;
#29231=CARTESIAN_POINT ( 'NONE',  ( 72.49754614901047489, 69.63129987044148095, 9.402869901847884293 ) ) ;
#29234=CARTESIAN_POINT ( 'NONE',  ( 85.78016935146355593, 43.45830298991825202, 4.388455215017684097 ) ) ;
#29242=CARTESIAN_POINT ( 'NONE',  ( 88.03469742524457331, 44.28626028149027860, -4.397723919905308421 ) ) ;
#29244=CARTESIAN_POINT ( 'NONE',  ( 35.68911091587340678, 42.64646525600393545, -2.839279412974133887 ) ) ;
#29245=CARTESIAN_POINT ( 'NONE',  ( 80.09407555685091040, 44.71242426696124994, 11.12975979062820642 ) ) ;
#29246=CARTESIAN_POINT ( 'NONE',  ( 79.15025889697260197, 58.45979598525892840, -16.21445014555780872 ) ) ;
#29249=ORIENTED_EDGE ( 'NONE', *, *, #87198, .T. ) ;
#29250=ORIENTED_EDGE ( 'NONE', *, *, #8847, .T. ) ;
#29252=DIRECTION ( 'NONE',  ( 0.8660254037844378194, 0.5000000000000014433, 0.000000000000000000 ) ) ;
#29256=CARTESIAN_POINT ( 'NONE',  ( 68.42202639013687815, 68.53051497116777568, 7.558587510793364217 ) ) ;
#29258=CARTESIAN_POINT ( 'NONE',  ( 82.09069798584521038, 40.79266795312825877, 1.461721908553118343 ) ) ;
#29260=CARTESIAN_POINT ( 'NONE',  ( 77.22560725433092443, 63.51237900320956697, -15.09333827328594779 ) ) ;
#29263=ORIENTED_EDGE ( 'NONE', *, *, #63853, .F. ) ;
#29265=CARTESIAN_POINT ( 'NONE',  ( 36.43182450750798296, 23.96004757982092315, -5.678558825948276656 ) ) ;
#29269=EDGE_CURVE ( 'NONE', #78719, #54783, #48720, .T. ) ;
#29270=CARTESIAN_POINT ( 'NONE',  ( 86.76444126019434577, 45.86660341771494842, -8.261827951889216592 ) ) ;
#29272=DIRECTION ( 'NONE',  ( -0.4386133837897759347, -0.6599160945941885403, -0.6100238090894788412 ) ) ;
#29280=CARTESIAN_POINT ( 'NONE',  ( 74.14312167556930433, 66.30466486950707861, 1.224646799147354045E-15 ) ) ;
#29287=CARTESIAN_POINT ( 'NONE',  ( 82.73930168436014299, 45.65283476154188236, 10.64355013692776808 ) ) ;
#29288=FACE_OUTER_BOUND ( 'NONE', #37214, .T. ) ;
#29294=CARTESIAN_POINT ( 'NONE',  ( 71.34228633229245986, 62.25329621047778517, 14.07928033790851252 ) ) ;
#29304=CARTESIAN_POINT ( 'NONE',  ( 82.74206721279597332, 53.66691124579689642, -15.75745978315255513 ) ) ;
#29313=CARTESIAN_POINT ( 'NONE',  ( 35.32779635548150310, 39.13478043621390867, 8.090169943749478065 ) ) ;
#29316=CARTESIAN_POINT ( 'NONE',  ( 71.87971293488917013, 71.94524500174831871, 2.848367791380675307 ) ) ;
#29320=CARTESIAN_POINT ( 'NONE',  ( 78.90362582645330747, 50.91995579366576408, -15.11086290727698334 ) ) ;
#29324=CARTESIAN_POINT ( 'NONE',  ( 24.44820476603448611, 26.06628583063842086, -9.188101187500006262 ) ) ;
#29327=CARTESIAN_POINT ( 'NONE',  ( 5.120201826081539842, 21.14336893147752861, 7.433330006724141015 ) ) ;
#29330=CARTESIAN_POINT ( 'NONE',  ( 75.23362143766534871, 55.25164565488622515, 16.61958235066795453 ) ) ;
#29332=CARTESIAN_POINT ( 'NONE',  ( 73.51157771055966350, 64.85277606651841609, 13.41954812668761043 ) ) ;
#29333=CARTESIAN_POINT ( 'NONE',  ( 69.54925760825628345, 67.89440790003212101, -8.609516418554425954 ) ) ;
#29338=CARTESIAN_POINT ( 'NONE',  ( 87.69706225426612889, 45.27692322852378481, -6.313661759682479335 ) ) ;
#29342=ORIENTED_EDGE ( 'NONE', *, *, #27802, .T. ) ;
#29352=CARTESIAN_POINT ( 'NONE',  ( 71.63207289816666901, 60.29376661390504211, 15.47974284963322766 ) ) ;
#29353=CARTESIAN_POINT ( 'NONE',  ( 73.10219508433868896, 70.64483191105212256, -7.776791464595123493 ) ) ;
#29354=CARTESIAN_POINT ( 'NONE',  ( 82.41933087055697627, 40.38430946167127189, -0.8419157719606927825 ) ) ;
#29357=CARTESIAN_POINT ( 'NONE',  ( 14.52983486323338802, 31.49540643055186706, 3.479690158560446702E-15 ) ) ;
#29358=CARTESIAN_POINT ( 'NONE',  ( 67.93740734008792970, 69.57397595783162103, -2.710152877030299390 ) ) ;
#29367=CARTESIAN_POINT ( 'NONE',  ( 72.92559869912804515, 69.38761754411618199, 9.979010455306335459 ) ) ;
#29372=CARTESIAN_POINT ( 'NONE',  ( 81.58121470000600084, 55.78443411318616540, 16.36431025809738671 ) ) ;
#29376=ORIENTED_EDGE ( 'NONE', *, *, #58612, .T. ) ;
#29378=CARTESIAN_POINT ( 'NONE',  ( 74.52062983175133581, 59.67663687933149674, -16.10628646854518919 ) ) ;
#29386=CARTESIAN_POINT ( 'NONE',  ( 66.74918157967780985, 67.50276577062598449, 6.564943354671691544 ) ) ;
#29389=CARTESIAN_POINT ( 'NONE',  ( 81.69344565705650041, 55.64297880859076173, 15.97102128751869543 ) ) ;
#29391=CARTESIAN_POINT ( 'NONE',  ( 71.15088032201443013, 65.96942632406533846, 11.64872445604752471 ) ) ;
#29405=CARTESIAN_POINT ( 'NONE',  ( 88.00768034709845722, 44.38581256804975794, 4.745967170566631310 ) ) ;
#29409=CARTESIAN_POINT ( 'NONE',  ( 72.99786219007800980, 70.75108751906873295, 8.232086053012805493 ) ) ;
#29410=CARTESIAN_POINT ( 'NONE',  ( 72.11059876947601310, 67.12034913926613910, -11.19373116030997295 ) ) ;
#29411=ORIENTED_EDGE ( 'NONE', *, *, #73942, .T. ) ;
#29415=CARTESIAN_POINT ( 'NONE',  ( 72.51849084938635315, 71.52899382949979668, -5.376470287118201519 ) ) ;
#29416=CARTESIAN_POINT ( 'NONE',  ( 80.31617148571714893, 48.80743944517941202, 13.89541408168290992 ) ) ;
#29422=CARTESIAN_POINT ( 'NONE',  ( 27.69565257936902469, 21.15404122711134605, 8.090169943749479842 ) ) ;
#29423=CARTESIAN_POINT ( 'NONE',  ( 73.08094384907833785, 54.14441083166271795, 0.000000000000000000 ) ) ;
#29427=CARTESIAN_POINT ( 'NONE',  ( 72.17591038400095727, 71.86111175976400034, -3.889098828490574533 ) ) ;
#29431=CARTESIAN_POINT ( 'NONE',  ( 66.46511978770725193, 67.85058371895827634, -6.740288372309689358 ) ) ;
#29432=CARTESIAN_POINT ( 'NONE',  ( 73.06733342522696262, 70.46939842116798047, -8.031525681787078597 ) ) ;
#29437=CARTESIAN_POINT ( 'NONE',  ( 20.02985575298534471, 35.65659080271450421, -1.878358725466461243E-16 ) ) ;
#29438=CARTESIAN_POINT ( 'NONE',  ( 85.07387056782178547, 48.93214387692037093, 12.41537898381571026 ) ) ;
#29440=CARTESIAN_POINT ( 'NONE',  ( 72.15423005933928380, 71.84479394171614786, -3.903858941020849738 ) ) ;
#29448=VECTOR ( 'NONE', #92890, 1000.000000000000000 ) ;
#29452=CARTESIAN_POINT ( 'NONE',  ( 42.04415689841856363, 29.98920272979930246, 7.433330006724137462 ) ) ;
#29454=B_SPLINE_CURVE_WITH_KNOTS ( 'NONE', 3,
 ( #88879, #3723, #65500, #19441, #66003, #43178, #96954, #49313, #89363, #50791, #12315, #4715, #35600, #66498, #27993, #97912, #58872, #20416, #51283, #82252, #12825, #28487, #59368, #18423, #80252, #41695, #20923, #36581, #37569, #22386, #76119, #5690, #83730, #15264, #52283, #6692, #83224, #51806, #67989, #92330, #90847, #53283, #67486, #99898, #45180, #60863 ),
 .UNSPECIFIED., .F., .F.,
 ( 4, 1, 1, 1, 2, 2, 1, 1, 1, 2, 2, 1, 1, 2, 2, 1, 1, 2, 2, 1, 1, 2, 2, 1, 2, 2, 1, 2, 2, 4 ),
 ( 0.000000000000000000, 0.06250000000002371714, 0.09375000000003461120, 0.1093750000000400652, 0.1171875000000423134, 0.1250000000000445755, 0.1875000000000582590, 0.2187500000000651423, 0.2343750000000676403, 0.2421875000000674738, 0.2500000000000672795, 0.3125000000000652811, 0.3437500000000648370, 0.3593750000000646150, 0.3750000000000643374, 0.4375000000000635048, 0.4687500000000631162, 0.4843750000000619504, 0.5000000000000607292, 0.5625000000000570655, 0.5937500000000536238, 0.6093750000000520695, 0.6250000000000504041, 0.6875000000000429656, 0.7187500000000411893, 0.7500000000000393019, 0.8125000000000316414, 0.8437500000000254241, 0.8750000000000192069, 1.000000000000000000 ),
 .UNSPECIFIED. ) ;
#29460=CARTESIAN_POINT ( 'NONE',  ( 19.31277771287585310, 13.01110640527291551, 2.839279412974134775 ) ) ;
#29462=CARTESIAN_POINT ( 'NONE',  ( 71.70303330742534342, 59.04301762528319131, 15.85811543470831353 ) ) ;
#29467=CARTESIAN_POINT ( 'NONE',  ( 75.04791297046116938, 53.45263424984147349, -16.05211567179630805 ) ) ;
#29468=CARTESIAN_POINT ( 'NONE',  ( 88.26230900456008044, 44.35601202938862997, 2.501165180090373141 ) ) ;
#29470=ORIENTED_EDGE ( 'NONE', *, *, #75706, .F. ) ;
#29474=CARTESIAN_POINT ( 'NONE',  ( 77.14822757211506143, 63.64430466641118755, 15.03252049986617500 ) ) ;
#29483=CARTESIAN_POINT ( 'NONE',  ( 71.43724303959665178, 68.55867823653906612, 9.960316262241418528 ) ) ;
#29484=CARTESIAN_POINT ( 'NONE',  ( 80.31886729598942054, 57.42767889257750369, -16.58902572440456780 ) ) ;
#29487=CARTESIAN_POINT ( 'NONE',  ( 87.69383267149372330, 45.37878083771482807, -6.511118445142236588 ) ) ;
#29491=ORIENTED_EDGE ( 'NONE', *, *, #93713, .F. ) ;
#29498=CARTESIAN_POINT ( 'NONE',  ( 41.54549712337441747, 24.39040679176986615, -6.890680421881970419E-14 ) ) ;
#29499=B_SPLINE_CURVE_WITH_KNOTS ( 'NONE', 3,
 ( #51566, #72905, #57656, #4469, #43948, #58161, #41968, #74398, #27773, #4983 ),
 .UNSPECIFIED., .F., .F.,
 ( 4, 2, 2, 2, 4 ),
 ( 0.000000000000000000, 0.2500000000000000000, 0.5000000000000000000, 0.7500000000000000000, 1.000000000000000000 ),
 .UNSPECIFIED. ) ;
#29502=EDGE_CURVE ( 'NONE', #34466, #57243, #60684, .T. ) ;
#29503=CARTESIAN_POINT ( 'NONE',  ( 73.47134878188418838, 69.83576924732003022, 9.227620320897900186 ) ) ;
#29523=CARTESIAN_POINT ( 'NONE',  ( 76.63684583903793168, 54.02340966775668107, -16.04885996875553644 ) ) ;
#29525=CARTESIAN_POINT ( 'NONE',  ( 84.23708473736340352, 41.98719078163990304, 4.050242299038782079 ) ) ;
#29526=CARTESIAN_POINT ( 'NONE',  ( 79.22627167205122589, 45.80186466725063354, 13.02917726998096271 ) ) ;
#29529=CARTESIAN_POINT ( 'NONE',  ( 69.23870777756563655, 65.06122599265698625, -11.45902463328623178 ) ) ;
#29533=CARTESIAN_POINT ( 'NONE',  ( 72.32137329212656596, 71.76143927211870732, 5.594163357809740944 ) ) ;
#29540=DIRECTION ( 'NONE',  ( 0.5000000000000014433, -0.8660254037844378194, 0.000000000000000000 ) ) ;
#29548=CARTESIAN_POINT ( 'NONE',  ( 81.95746785621842889, 41.34290087354509780, -5.897592725355119470 ) ) ;
#29560=CARTESIAN_POINT ( 'NONE',  ( 7.533646096595723485, 16.30066082961419482, -10.00000000000000533 ) ) ;
#29562=CARTESIAN_POINT ( 'NONE',  ( 71.65411058451715576, 58.83614272603743700, -15.40970175268381404 ) ) ;
#29563=CARTESIAN_POINT ( 'NONE',  ( 73.09565900097605606, 69.67901489450639474, 9.155081292670679716 ) ) ;
#29567=CARTESIAN_POINT ( 'NONE',  ( 73.13622937094719134, 57.24645749009919626, 16.39293205268555909 ) ) ;
#29568=CARTESIAN_POINT ( 'NONE',  ( 69.82165319358976774, 66.39592426718104434, 11.22546775247526973 ) ) ;
#29569=CARTESIAN_POINT ( 'NONE',  ( 66.15839288007977359, 68.64661655514622396, -4.374828951538166422 ) ) ;
#29574=CARTESIAN_POINT ( 'NONE',  ( 24.77416059058194620, 29.70171378149920471, -9.188101187500004485 ) ) ;
#29576=LINE ( 'NONE', #36663, #67821 ) ;
#29579=CARTESIAN_POINT ( 'NONE',  ( 84.89744547285587828, 41.79037650531964943, -3.168800655305855967E-06 ) ) ;
#29581=CARTESIAN_POINT ( 'NONE',  ( 68.79284463328235688, 64.08361226851032200, 12.02460708678565560 ) ) ;
#29583=CARTESIAN_POINT ( 'NONE',  ( 81.18224314092121574, 50.95777291934366104, 15.14991892385681282 ) ) ;
#29589=PLANE ( 'NONE',  #48983 ) ;
#29590=CARTESIAN_POINT ( 'NONE',  ( 81.98204644731730184, 41.14170830008083612, -5.380964918418897902 ) ) ;
#29591=CARTESIAN_POINT ( 'NONE',  ( 75.30369160444902832, 53.36362683429165088, 16.03060775139856631 ) ) ;
#29593=B_SPLINE_SURFACE_WITH_KNOTS ( 'NONE', 3, 1, ( 
 ( #25201, #31299 ),
 ( #78938, #69800 ),
 ( #63206, #62690 ),
 ( #62186, #94148 ),
 ( #54582, #100227 ),
 ( #9007, #1421 ),
 ( #70815, #87079 ),
 ( #94646, #56084 ),
 ( #15589, #38896 ),
 ( #93646, #17611 ),
 ( #70299, #46490 ),
 ( #48519, #9526 ),
 ( #40387, #24701 ),
 ( #55092, #93138 ),
 ( #8024, #85563 ),
 ( #39381, #39878 ),
 ( #86078, #55583 ),
 ( #86568, #79455 ),
 ( #71327, #909 ),
 ( #23687, #23193 ),
 ( #16108, #47007 ),
 ( #16602, #1918 ),
 ( #47501, #61692 ),
 ( #32804, #77921 ),
 ( #31788, #8513 ),
 ( #78426, #38394 ),
 ( #69305, #30813 ),
 ( #92645, #54086 ),
 ( #77423, #85040 ),
 ( #89555, #79950 ),
 ( #10517, #41899 ) ),
 .UNSPECIFIED., .F., .F., .F.,
 ( 4, 3, 3, 3, 3, 3, 3, 3, 3, 3, 4 ),
 ( 2, 2 ),
 ( 0.000000000000000000, 0.1333490885032313222, 0.3007194338854298210, 0.4699862290245092056, 0.5844252810809273946, 0.6686540514502635757, 0.7354980260655534785, 0.8028463152565743499, 0.8633854507757382502, 0.9437142632667581132, 1.000000000000000000 ),
 ( 0.000000000000000000, 1.000000000000000000 ),
 .UNSPECIFIED. ) ;
#29599=CARTESIAN_POINT ( 'NONE',  ( 68.41443082112564866, 69.68312250061349289, 3.489189732842724379 ) ) ;
#29602=CARTESIAN_POINT ( 'NONE',  ( 16.09091216865756024, 14.45404122711132366, -8.090169943749478065 ) ) ;
#29607=CARTESIAN_POINT ( 'NONE',  ( 81.64570241471020040, 45.46107742057574086, -11.03823634419222088 ) ) ;
#29613=CARTESIAN_POINT ( 'NONE',  ( 69.54173309467141451, 62.57597753113334704, 13.33913063052011516 ) ) ;
#29618=CARTESIAN_POINT ( 'NONE',  ( 81.56933533924238588, 42.63988948739947205, -7.637657182551536472 ) ) ;
#29619=B_SPLINE_SURFACE_WITH_KNOTS ( 'NONE', 3, 1, ( 
 ( #88738, #65373 ),
 ( #35468, #20284 ),
 ( #96821, #27379 ),
 ( #3594, #49670 ),
 ( #73987, #51158 ),
 ( #82122, #43043 ),
 ( #80124, #64887 ),
 ( #58751, #3116 ),
 ( #81612, #95833 ),
 ( #81128, #58264 ),
 ( #97303, #34002 ),
 ( #12695, #89242 ),
 ( #19792, #26386 ),
 ( #64380, #50660 ),
 ( #27871, #57762 ),
 ( #4571, #42554 ),
 ( #89723, #12182 ),
 ( #19309, #74501 ),
 ( #34474, #5079 ),
 ( #95342, #56771 ),
 ( #25899, #87753 ),
 ( #42072, #18294 ),
 ( #49188, #10686 ),
 ( #41564, #57264 ),
 ( #50175, #72508 ),
 ( #88239, #18790 ),
 ( #80626, #11202 ),
 ( #73004, #96315 ),
 ( #26883, #11695 ),
 ( #73487, #22257 ),
 ( #97791, #45055 ) ),
 .UNSPECIFIED., .F., .F., .F.,
 ( 4, 3, 3, 3, 3, 3, 3, 3, 3, 3, 4 ),
 ( 2, 2 ),
 ( 0.000000000000000000, 0.1333490885032390105, 0.3007194338854328186, 0.4699862290245252483, 0.5844252810809424936, 0.6686540514502805621, 0.7354980260655528124, 0.8028463152565618044, 0.8633854507757205976, 0.9437142632667329112, 1.000000000000000000 ),
 ( 0.000000000000000000, 1.000000000000000000 ),
 .UNSPECIFIED. ) ;
#29625=CARTESIAN_POINT ( 'NONE',  ( 69.55938073166919366, 70.14142446728632763, 4.291733062184300174 ) ) ;
#29628=EDGE_CURVE ( 'NONE', #2384, #94954, #13547, .T. ) ;
#29629=CARTESIAN_POINT ( 'NONE',  ( 82.38632442250769827, 41.28528657744342922, 3.301102426468717432 ) ) ;
#29632=CARTESIAN_POINT ( 'NONE',  ( 82.69574664279603837, 54.03060105484253484, -15.86596363536033394 ) ) ;
#29634=ORIENTED_EDGE ( 'NONE', *, *, #68811, .T. ) ;
#29635=CARTESIAN_POINT ( 'NONE',  ( 76.92699712112981558, 61.20612098636846099, 15.66493907231634708 ) ) ;
#29636=CARTESIAN_POINT ( 'NONE',  ( 17.37926562425035826, 12.96004757982088762, -5.678558825948276656 ) ) ;
#29639=CARTESIAN_POINT ( 'NONE',  ( 80.07172880487748046, 57.71088839156739425, 16.60216399474093052 ) ) ;
#29653=CARTESIAN_POINT ( 'NONE',  ( 82.86199955364607206, 53.47446029988319793, -15.31866780845555098 ) ) ;
#29656=CARTESIAN_POINT ( 'NONE',  ( 85.60939809066302075, 44.62657166848472912, -7.207540832648801299 ) ) ;
#29660=CARTESIAN_POINT ( 'NONE',  ( 76.09137042060903866, 65.46242010497813624, 13.98445105613830286 ) ) ;
#29667=CARTESIAN_POINT ( 'NONE',  ( 87.51647913336857698, 44.56403561216112053, 4.883618514853080406 ) ) ;
#29669=CARTESIAN_POINT ( 'NONE',  ( 83.75618562079634444, 45.13567822924630235, 9.457446474821283644 ) ) ;
#29678=CONICAL_SURFACE ( 'NONE', #54798, 10.00000000000000711, 0.7853981633974608245 ) ;
#29681=CARTESIAN_POINT ( 'NONE',  ( 77.91090169867500492, 54.32762231749097026, -16.00590757115833540 ) ) ;
#29693=CARTESIAN_POINT ( 'NONE',  ( 14.44138481658839090, 10.19860640527290663, 2.839279412974134775 ) ) ;
#29697=CARTESIAN_POINT ( 'NONE',  ( 83.90285338613423960, 42.24628314658283301, -3.729123792273444149 ) ) ;
#29701=CARTESIAN_POINT ( 'NONE',  ( 32.17510246534131113, 41.68290643055190259, 3.479690158560446702E-15 ) ) ;
#29705=CARTESIAN_POINT ( 'NONE',  ( 31.76189289227714951, 20.19860640527293683, 2.839279412974134775 ) ) ;
#29711=CARTESIAN_POINT ( 'NONE',  ( 70.54793603911069511, 60.92313004140932264, 14.99536235483401292 ) ) ;
#29719=CARTESIAN_POINT ( 'NONE',  ( 73.04738217724886340, 69.71546789186045601, 9.669594540409617522 ) ) ;
#29722=CARTESIAN_POINT ( 'NONE',  ( 78.38601017018802963, 61.50250219569392129, 16.18534724403902914 ) ) ;
#29731=VECTOR ( 'NONE', #5544, 1000.000000000000114 ) ;
#29732=CARTESIAN_POINT ( 'NONE',  ( 32.50825522076439000, 36.95586893147758190, 7.433330006724141015 ) ) ;
#29733=CARTESIAN_POINT ( 'NONE',  ( 81.62968001876643598, 55.78593752935011452, -16.36028778889454927 ) ) ;
#29735=CARTESIAN_POINT ( 'NONE',  ( 87.45809072578427390, 45.51379687347738923, 7.041989649719552880 ) ) ;
#29736=ORIENTED_EDGE ( 'NONE', *, *, #53101, .F. ) ;
#29741=CARTESIAN_POINT ( 'NONE',  ( 79.60263393892513761, 55.67592396758841744, 16.11189329299018880 ) ) ;
#29742=B_SPLINE_CURVE_WITH_KNOTS ( 'NONE', 3,
 ( #13147, #50615, #82584, #97265, #66822, #12651, #27832, #20746, #75440, #51117, #73447, #89202, #28318, #19266, #81085, #98246, #29333, #67318, #6023, #60199, #28834, #34919, #81569, #59715, #74459, #36414, #90681, #36919, #19750, #44004, #65815, #5039, #11651, #35921, #50133, #96777, #21237, #42511, #74946, #98753, #51632, #44510, #97750, #52116, #27342, #59197 ),
 .UNSPECIFIED., .F., .F.,
 ( 4, 1, 1, 1, 2, 2, 1, 1, 1, 2, 2, 1, 1, 2, 2, 1, 1, 2, 2, 1, 1, 2, 2, 1, 2, 2, 1, 2, 2, 4 ),
 ( 0.000000000000000000, 0.06250000000001772194, 0.09375000000002634004, 0.1093750000000307532, 0.1171875000000328210, 0.1250000000000348888, 0.1875000000000514588, 0.2187500000000598410, 0.2343750000000623945, 0.2421875000000621170, 0.2500000000000618394, 0.3125000000000588973, 0.3437500000000590084, 0.3593750000000572875, 0.3750000000000555112, 0.4375000000000416334, 0.4687500000000364708, 0.4843750000000339173, 0.5000000000000313083, 0.5625000000000253131, 0.5937500000000219824, 0.6093750000000203171, 0.6250000000000186517, 0.6875000000000177636, 0.7187500000000156541, 0.7500000000000134337, 0.8125000000000118794, 0.8437500000000092149, 0.8750000000000065503, 1.000000000000000000 ),
 .UNSPECIFIED. ) ;
#29745=CARTESIAN_POINT ( 'NONE',  ( 78.60735446187601383, 47.91558663937575346, -14.46554739992949834 ) ) ;
#29747=CARTESIAN_POINT ( 'NONE',  ( 76.11246596381349150, 60.38636913568999631, -15.73763889482215284 ) ) ;
#29748=CARTESIAN_POINT ( 'NONE',  ( 82.11498198633205448, 40.81356640863849350, 1.533337055892688428 ) ) ;
#29750=CARTESIAN_POINT ( 'NONE',  ( 77.10166062722221625, 63.64310012191319288, -15.01751612965061788 ) ) ;
#29754=EDGE_LOOP ( 'NONE', ( #19165, #73836, #66615, #93167 ) ) ;
#29756=CARTESIAN_POINT ( 'NONE',  ( 38.99862784774133218, 37.91421378149922816, 9.188101187500008038 ) ) ;
#29760=CARTESIAN_POINT ( 'NONE',  ( 86.79909420986851387, 45.86349359382401047, -8.229471332425589480 ) ) ;
#29761=FACE_OUTER_BOUND ( 'NONE', #73105, .T. ) ;
#29763=CARTESIAN_POINT ( 'NONE',  ( 25.64143417502910083, 37.73705186507756082, -3.090169943749475845 ) ) ;
#29769=ORIENTED_EDGE ( 'NONE', *, *, #5220, .F. ) ;
#29772=CARTESIAN_POINT ( 'NONE',  ( 8.758203689844268780, 28.55466486950697913, -1.111400068045478839E-16 ) ) ;
#29774=CARTESIAN_POINT ( 'NONE',  ( 83.23441648756779898, 46.93106052681729778, 11.58471493876596270 ) ) ;
#29778=ORIENTED_EDGE ( 'NONE', *, *, #72017, .F. ) ;
#29781=CARTESIAN_POINT ( 'NONE',  ( 70.99909089399695006, 61.09348569631758608, 14.50421621802051853 ) ) ;
#29787=CARTESIAN_POINT ( 'NONE',  ( 82.37260210843921016, 42.16043560824383718, 5.885805237006764834 ) ) ;
#29788=CARTESIAN_POINT ( 'NONE',  ( 21.28706459136418871, 17.45404122711133255, -8.090169943749478065 ) ) ;
#29790=CARTESIAN_POINT ( 'NONE',  ( 72.66873115938952310, 70.75946716845891160, -7.138114697723673352 ) ) ;
#29795=EDGE_CURVE ( 'NONE', #58166, #20250, #17099, .T. ) ;
#29798=CARTESIAN_POINT ( 'NONE',  ( 66.87949033550695788, 69.18773745924302432, 0.7640449060900401657 ) ) ;
#29799=CARTESIAN_POINT ( 'NONE',  ( 73.47103776244834705, 69.18898954907001553, -9.996715955230138562 ) ) ;
#29802=CARTESIAN_POINT ( 'NONE',  ( 36.54023192077972482, 39.83478043621391151, -8.090169943749479842 ) ) ;
#29805=CARTESIAN_POINT ( 'NONE',  ( 72.14269493036653103, 72.23228066185846785, 3.937576401637844281 ) ) ;
#29815=CARTESIAN_POINT ( 'NONE',  ( 20.18904385193075868, 29.84336893147756342, -7.433330006724137462 ) ) ;
#29818=CARTESIAN_POINT ( 'NONE',  ( 36.20694410119924811, 43.83705186507757645, 3.090169943749475401 ) ) ;
#29820=CARTESIAN_POINT ( 'NONE',  ( 77.17614375499567814, 63.59805229717832731, 15.05336917137992359 ) ) ;
#29821=CARTESIAN_POINT ( 'NONE',  ( 76.62156306105930526, 63.43458379359962152, 15.37592086074861619 ) ) ;
#29823=CARTESIAN_POINT ( 'NONE',  ( 82.10205964440194748, 40.74581685175329682, -0.8055849532097474341 ) ) ;
#29825=EDGE_CURVE ( 'NONE', #52395, #31328, #36484, .T. ) ;
#29827=CARTESIAN_POINT ( 'NONE',  ( 87.76806118867082773, 45.25231315247835084, -7.033483185435909668 ) ) ;
#29839=VERTEX_POINT ( 'NONE', #55567 ) ;
#29841=CARTESIAN_POINT ( 'NONE',  ( 79.26833296275110285, 45.71260820663386681, -12.95081413666752113 ) ) ;
#29844=CARTESIAN_POINT ( 'NONE',  ( 70.34454795188869980, 61.29844696716961749, 14.78467410895967760 ) ) ;
#29847=CARTESIAN_POINT ( 'NONE',  ( 15.07770630580378501, 30.74646525600389424, 2.839279412974139660 ) ) ;
#29848=CARTESIAN_POINT ( 'NONE',  ( 75.87287823110008844, 59.20612602118985279, 15.91568303443457388 ) ) ;
#29849=CARTESIAN_POINT ( 'NONE',  ( 69.39565660130948288, 70.00884411262029516, -4.393149027308437482 ) ) ;
#29851=VERTEX_POINT ( 'NONE', #87058 ) ;
#29854=ORIENTED_EDGE ( 'NONE', *, *, #65299, .F. ) ;
#29855=VERTEX_POINT ( 'NONE', #45967 ) ;
#29856=CARTESIAN_POINT ( 'NONE',  ( 80.96765023889031454, 49.62782080103354332, -14.15289701881580520 ) ) ;
#29867=ORIENTED_EDGE ( 'NONE', *, *, #83155, .F. ) ;
#29872=ORIENTED_EDGE ( 'NONE', *, *, #1488, .F. ) ;
#29875=CARTESIAN_POINT ( 'NONE',  ( 66.81218498664068761, 67.51421540899519869, 6.611934933653538238 ) ) ;
#29878=CARTESIAN_POINT ( 'NONE',  ( 15.09101445147005727, 32.21091486745859811, -1.111400068045478839E-16 ) ) ;
#29880=CARTESIAN_POINT ( 'NONE',  ( 73.04277380876573034, 70.56196896876862468, 7.835544939490341143 ) ) ;
#29882=AXIS2_PLACEMENT_3D ( 'NONE', #87018, #31724, #17549 ) ;
#29885=B_SPLINE_CURVE_WITH_KNOTS ( 'NONE', 3,
 ( #49530, #67092, #50037, #5797, #74732, #80989, #57119, #64747, #83334, #49043 ),
 .UNSPECIFIED., .F., .F.,
 ( 4, 2, 2, 2, 4 ),
 ( 0.000000000000000000, 0.0002622400424272852194, 0.0005244800848545704388, 0.0007867201272818557124, 0.001048960169709140878 ),
 .UNSPECIFIED. ) ;
#29886=CARTESIAN_POINT ( 'NONE',  ( 76.05862284836669573, 51.28839337040800217, -15.63733761827814561 ) ) ;
#29888=CARTESIAN_POINT ( 'NONE',  ( 76.03787485198571972, 65.47122818424047352, -14.36642907054480744 ) ) ;
#29899=CARTESIAN_POINT ( 'NONE',  ( 72.78673888116644264, 70.95540242780744222, 7.715912594624938059 ) ) ;
#29900=CARTESIAN_POINT ( 'NONE',  ( 69.93916249099559934, 67.39072072629922161, -9.564019846174506512 ) ) ;
#29901=ORIENTED_EDGE ( 'NONE', *, *, #72773, .T. ) ;
#29904=CARTESIAN_POINT ( 'NONE',  ( 72.40111988405350019, 71.17098879578473714, -6.090184461575853803 ) ) ;
#29906=CARTESIAN_POINT ( 'NONE',  ( 73.71283706923053103, 69.58716896801121266, -9.688382991847833026 ) ) ;
#29911=CARTESIAN_POINT ( 'NONE',  ( 71.23505992429709011, 71.80871246845643441, 0.3731813833289527316 ) ) ;
#29917=CARTESIAN_POINT ( 'NONE',  ( 29.68521398013932711, 18.10801979619930080, 3.090169943749476733 ) ) ;
#29918=EDGE_CURVE ( 'NONE', #82741, #40944, #9960, .T. ) ;
#29927=CARTESIAN_POINT ( 'NONE',  ( 72.57773168451070944, 70.69087215581754435, -7.948841485240754068 ) ) ;
#29930=CARTESIAN_POINT ( 'NONE',  ( 21.58410742392950610, 28.16454794089041869, -10.00000000000000355 ) ) ;
#29931=CARTESIAN_POINT ( 'NONE',  ( 85.41200716118709124, 49.08779630762384727, 12.38492377717305182 ) ) ;
#29933=CARTESIAN_POINT ( 'NONE',  ( 71.86410153269953582, 71.70156373010919992, -3.808556656956898490 ) ) ;
#29939=ADVANCED_FACE ( 'NONE', ( #49485 ), #80949, .T. ) ;
#29944=CARTESIAN_POINT ( 'NONE',  ( 67.00398746445188181, 69.51674466867500257, -2.934459324224529819 ) ) ;
#29945=CARTESIAN_POINT ( 'NONE',  ( 36.37119629183458613, 23.12755873383628114, -6.180339887498949025 ) ) ;
#29946=CARTESIAN_POINT ( 'NONE',  ( 74.18762515466688967, 72.22758258259658248, 0.000000000000000000 ) ) ;
#29954=CARTESIAN_POINT ( 'NONE',  ( 14.05709621874952475, 23.51421378149918340, -9.188101187500004485 ) ) ;
#29956=CARTESIAN_POINT ( 'NONE',  ( 72.00843944767480309, 59.19984693747115045, 15.36336254789745581 ) ) ;
#29958=ORIENTED_EDGE ( 'NONE', *, *, #94882, .F. ) ;
#29962=CARTESIAN_POINT ( 'NONE',  ( 75.30550521261754682, 53.62394084548385109, -16.53342909214022782 ) ) ;
#29963=CARTESIAN_POINT ( 'NONE',  ( 81.23883169307138985, 42.40595559033209838, 7.569205759766643560 ) ) ;
#29965=FACE_OUTER_BOUND ( 'NONE', #92220, .T. ) ;
#29966=CARTESIAN_POINT ( 'NONE',  ( 72.59885289546373599, 71.51145701098552365, -5.543222466649145197 ) ) ;
#29975=CARTESIAN_POINT ( 'NONE',  ( 24.60437102317565206, 29.90829794293881605, 10.00000000000000355 ) ) ;
#29977=CARTESIAN_POINT ( 'NONE',  ( 77.32817876982272765, 63.13942984521013813, 15.61058464551962111 ) ) ;
#29978=ORIENTED_EDGE ( 'NONE', *, *, #51565, .T. ) ;
#29989=CARTESIAN_POINT ( 'NONE',  ( 33.59574554791263523, 38.13478043621391578, 8.090169943749478065 ) ) ;
#29990=CARTESIAN_POINT ( 'NONE',  ( 78.18060451095965391, 47.59931466318645477, -14.43139321312144219 ) ) ;
#29994=CARTESIAN_POINT ( 'NONE',  ( 73.09460200958936582, 69.68087498946766800, 9.152088038772804524 ) ) ;
#30002=CARTESIAN_POINT ( 'NONE',  ( 70.34102847698805761, 68.37141199246802614, 8.639829021907296180 ) ) ;
#30005=CARTESIAN_POINT ( 'NONE',  ( 66.96692701909594803, 66.98780766957318633, 8.644895272513664963 ) ) ;
#30007=CARTESIAN_POINT ( 'NONE',  ( 78.69402153464497474, 47.55556487758106954, 14.25945737374057742 ) ) ;
#30009=CIRCLE ( 'NONE', #2790, 15.60714546451148799 ) ;
#30011=CARTESIAN_POINT ( 'NONE',  ( 75.37844399319210709, 54.42689092199589851, -16.12112201184755733 ) ) ;
#30013=CARTESIAN_POINT ( 'NONE',  ( 78.88938659514667506, 46.33750193266715911, 12.91880430790163281 ) ) ;
#30016=CARTESIAN_POINT ( 'NONE',  ( 75.78590872935743050, 56.04690169322937265, -16.60533866342026244 ) ) ;
#30021=CARTESIAN_POINT ( 'NONE',  ( 72.49672817265226854, 71.70303783552662935, 5.966909785267820787 ) ) ;
#30024=EDGE_CURVE ( 'NONE', #58166, #10592, #58088, .T. ) ;
#30026=CARTESIAN_POINT ( 'NONE',  ( 79.14312167556931854, 57.64441083166269664, 0.000000000000000000 ) ) ;
#30035=CARTESIAN_POINT ( 'NONE',  ( 73.60582443374298123, 62.09963750435122165, 15.23117417853161548 ) ) ;
#30038=CARTESIAN_POINT ( 'NONE',  ( 81.65512716465181597, 41.52065711327874453, -5.350319245000699553 ) ) ;
#30042=CARTESIAN_POINT ( 'NONE',  ( 65.88310562893971678, 69.02589174555536999, 1.996831191813055240 ) ) ;
#30044=DIRECTION ( 'NONE',  ( 0.4755282581475757664, -0.8236391035463335175, -0.3090169943749448977 ) ) ;
#30047=TOROIDAL_SURFACE ( 'NONE', #86743, 16.10714546451156437, 0.5000000000000000000 ) ;
#30049=CARTESIAN_POINT ( 'NONE',  ( 72.09295132551602592, 68.68266118357180972, -10.22840576930964396 ) ) ;
#30056=CARTESIAN_POINT ( 'NONE',  ( 72.87126216515173383, 57.15041428312686378, 15.90107093336461475 ) ) ;
#30058=CARTESIAN_POINT ( 'NONE',  ( 66.26881226693740246, 68.72770711070297978, -4.319471721241867179 ) ) ;
#30067=CARTESIAN_POINT ( 'NONE',  ( 33.38390286057418166, 24.98920272979928470, 7.433330006724137462 ) ) ;
#30071=LINE ( 'NONE', #6278, #10917 ) ;
#30073=CARTESIAN_POINT ( 'NONE',  ( 73.12133584826474930, 57.41764960941905116, -15.88333458976553381 ) ) ;
#30081=CARTESIAN_POINT ( 'NONE',  ( 3.104905098483929482, 23.83396525600387506, -2.839279412974133887 ) ) ;
#30085=VECTOR ( 'NONE', #97959, 1000.000000000000000 ) ;
#30087=CARTESIAN_POINT ( 'NONE',  ( 71.49724145223210314, 72.36708001998830753, 1.062265253749112626 ) ) ;
#30088=ADVANCED_FACE ( 'NONE', ( #96136 ), #11013, .T. ) ;
#30093=CARTESIAN_POINT ( 'NONE',  ( 68.70380343559517655, 69.96303083712633963, 3.047589648568798104 ) ) ;
#30097=CARTESIAN_POINT ( 'NONE',  ( 15.58658660100807580, 11.12755873383624561, -6.180339887498949025 ) ) ;
#30099=EDGE_LOOP ( 'NONE', ( #35257, #85635, #21132, #78208 ) ) ;
#30102=CARTESIAN_POINT ( 'NONE',  ( 80.60014811170655946, 45.61340808052423768, -11.68284267982980751 ) ) ;
#30105=CARTESIAN_POINT ( 'NONE',  ( 79.28866853763614131, 59.92453731934288896, -16.49803216704724207 ) ) ;
#30107=CARTESIAN_POINT ( 'NONE',  ( 69.44126986223525932, 62.66889528608714244, 13.25115268555880377 ) ) ;
#30112=CARTESIAN_POINT ( 'NONE',  ( 81.77397856916392982, 42.34590070723890420, -7.979864230673365810 ) ) ;
#30114=ORIENTED_EDGE ( 'NONE', *, *, #49674, .F. ) ;
#30116=CARTESIAN_POINT ( 'NONE',  ( 81.96106570470071517, 53.04313638909700046, 15.32626709879401616 ) ) ;
#30118=CARTESIAN_POINT ( 'NONE',  ( 70.05430382187989835, 70.68195646498267593, 3.459074501075599883 ) ) ;
#30119=VERTEX_POINT ( 'NONE', #19117 ) ;
#30124=CARTESIAN_POINT ( 'NONE',  ( 82.74279437798169567, 53.94163497425878262, -15.46549534628083400 ) ) ;
#30125=CARTESIAN_POINT ( 'NONE',  ( 73.42314397212541621, 57.50016318312121655, -16.38349303661395950 ) ) ;
#30126=CARTESIAN_POINT ( 'NONE',  ( 21.04482852044473162, 14.01110640527291906, 2.839279412974134775 ) ) ;
#30129=CARTESIAN_POINT ( 'NONE',  ( 80.25249281668115486, 57.81819139295712517, 16.60223264289302847 ) ) ;
#30136=CARTESIAN_POINT ( 'NONE',  ( 79.98071600351464383, 46.30330387653911828, -12.47010283063279878 ) ) ;
#30141=CARTESIAN_POINT ( 'NONE',  ( 75.01383350950912643, 67.34328350408775066, -12.89590634041037909 ) ) ;
#30144=EDGE_CURVE ( 'NONE', #67223, #50031, #248, .T. ) ;
#30149=CARTESIAN_POINT ( 'NONE',  ( 72.45510692969175182, 70.78848362686431983, 7.675293421552848550 ) ) ;
#30154=ORIENTED_EDGE ( 'NONE', *, *, #63678, .T. ) ;
#30160=CARTESIAN_POINT ( 'NONE',  ( 85.52188629250015595, 42.69847903795108124, 1.431352116385852469 ) ) ;
#30161=EDGE_CURVE ( 'NONE', #93933, #78755, #91509, .T. ) ;
#30163=CARTESIAN_POINT ( 'NONE',  ( 68.22205435738101187, 65.90345407221148832, 10.80313017757570826 ) ) ;
#30169=PLANE ( 'NONE',  #39941 ) ;
#30170=CARTESIAN_POINT ( 'NONE',  ( 81.96547941067910870, 41.17040324926905015, 3.814626384468428721 ) ) ;
#30178=CARTESIAN_POINT ( 'NONE',  ( 70.92518752925752779, 71.21820892678006487, 3.335809568748416165 ) ) ;
#30181=VERTEX_POINT ( 'NONE', #45363 ) ;
#30183=ADVANCED_FACE ( 'NONE', ( #76296 ), #30169, .T. ) ;
#30187=CARTESIAN_POINT ( 'NONE',  ( 9.185703322462060783, 20.70171378149917629, -9.188101187500004485 ) ) ;
#30196=CARTESIAN_POINT ( 'NONE',  ( 39.01788588657935719, 31.03085787977765975, 9.188101187500006262 ) ) ;
#30200=CARTESIAN_POINT ( 'NONE',  ( 24.61059131263772670, 35.18502408145592852, 5.678558825948277544 ) ) ;
#30206=ORIENTED_EDGE ( 'NONE', *, *, #62312, .F. ) ;
#30207=B_SPLINE_SURFACE_WITH_KNOTS ( 'NONE', 3, 1, ( 
 ( #32006, #77644 ),
 ( #7214, #8228 ),
 ( #39097, #24424 ),
 ( #41101, #87304 ),
 ( #2135, #17837 ),
 ( #79169, #24916 ),
 ( #3638, #25416 ),
 ( #41608, #79670 ),
 ( #57312, #72551 ),
 ( #88785, #56815 ),
 ( #34041, #19355 ),
 ( #18835, #56308 ),
 ( #2640, #55790 ),
 ( #72037, #73532 ),
 ( #49233, #26432 ),
 ( #11248, #32529 ),
 ( #63423, #9748 ),
 ( #48737, #18339 ),
 ( #94362, #10232 ),
 ( #95875, #86783 ),
 ( #33528, #64930 ),
 ( #87797, #50216 ),
 ( #49716, #94856 ),
 ( #34519, #64424 ),
 ( #3156, #63917 ),
 ( #88282, #80167 ),
 ( #81170, #11734 ),
 ( #80671, #17317 ),
 ( #95387, #42598 ),
 ( #25939, #10734 ),
 ( #42111, #73045 ) ),
 .UNSPECIFIED., .F., .F., .F.,
 ( 4, 3, 3, 3, 3, 3, 3, 3, 3, 3, 4 ),
 ( 2, 2 ),
 ( 0.000000000000000000, 0.1333490885032447282, 0.3007194338854389248, 0.4699862290245251373, 0.5844252810809574816, 0.6686540514502947730, 0.7354980260655736846, 0.8028463152565851191, 0.8633854507757401375, 0.9437142632667373521, 1.000000000000000000 ),
 ( 0.000000000000000000, 1.000000000000000000 ),
 .UNSPECIFIED. ) ;
#30209=CARTESIAN_POINT ( 'NONE',  ( 84.76617582037141574, 50.00026310130547813, -13.66906362199170921 ) ) ;
#30215=CARTESIAN_POINT ( 'NONE',  ( 73.30631488696991482, 69.89686749726290316, 9.630897265116471928 ) ) ;
#30216=CARTESIAN_POINT ( 'NONE',  ( 38.36533659613348846, 24.01110640527295104, 2.839279412974134775 ) ) ;
#30221=DIRECTION ( 'NONE',  ( -0.3940053768033626169, 0.6824373310787468228, 0.6156614753256509642 ) ) ;
#30226=EDGE_CURVE ( 'NONE', #29132, #50553, #39238, .T. ) ;
#30229=CARTESIAN_POINT ( 'NONE',  ( 34.13026518906141860, 41.74646525600392977, 2.839279412974139660 ) ) ;
#30231=CARTESIAN_POINT ( 'NONE',  ( 73.60933432321982650, 55.64367109616565443, 16.10230547196763595 ) ) ;
#30238=CARTESIAN_POINT ( 'NONE',  ( 72.13293662478744750, 72.32175006689249130, -1.141440976623812942 ) ) ;
#30239=CARTESIAN_POINT ( 'NONE',  ( 86.81641918289878390, 45.77657501471897916, -8.750901752256119437 ) ) ;
#30244=CARTESIAN_POINT ( 'NONE',  ( 77.29684513673267077, 59.91861738668672643, -15.97104762766038810 ) ) ;
#30255=CARTESIAN_POINT ( 'NONE',  ( 74.00349760290353629, 68.31608301643910863, -11.67389511724663009 ) ) ;
#30259=CARTESIAN_POINT ( 'NONE',  ( 16.38795500122288473, 25.16454794089041158, -10.00000000000000355 ) ) ;
#30271=CARTESIAN_POINT ( 'NONE',  ( 69.80192404618573221, 63.14541187278000223, -13.66695019165900149 ) ) ;
#30283=ADVANCED_FACE ( 'NONE', ( #16954 ), #53459, .T. ) ;
#30288=CARTESIAN_POINT ( 'NONE',  ( 82.64074333392795779, 53.51963485226765016, -15.73164264726942285 ) ) ;
#30300=CARTESIAN_POINT ( 'NONE',  ( 73.72691027005377862, 69.52791761355244660, -9.770281360779824453 ) ) ;
#30301=CARTESIAN_POINT ( 'NONE',  ( 76.58496548142363736, 51.27307132485643137, 16.05712343730097658 ) ) ;
#30302=CARTESIAN_POINT ( 'NONE',  ( 33.92686603480522223, 41.36126292948897998, 6.180339887498949913 ) ) ;
#30306=CARTESIAN_POINT ( 'NONE',  ( 71.88653196722606253, 72.25570330380722339, 3.269911192557288793 ) ) ;
#30312=CARTESIAN_POINT ( 'NONE',  ( 79.92971505533115817, 50.62409585498646436, -14.80966530455547847 ) ) ;
#30315=B_SPLINE_CURVE_WITH_KNOTS ( 'NONE', 3,
 ( #11437, #81353, #41795, #2836, #42290, #42780, #95570, #35702, #18024, #73714, #97052, #27620, #10417, #81843, #43286, #74232, #4818, #66601, #58969, #45284, #45770, #90454, #75215, #28591, #89941, #30093, #52390, #59977, #74730, #29599, #6298, #12927, #67591, #60471, #82358, #22492, #98521, #76692, #21023, #75713, #14880, #36682, #37189, #59473, #53384, #84334 ),
 .UNSPECIFIED., .F., .F.,
 ( 4, 1, 2, 2, 1, 2, 2, 1, 1, 2, 2, 1, 1, 2, 2, 1, 1, 2, 2, 1, 1, 1, 2, 2, 1, 1, 1, 2, 2, 4 ),
 ( 0.000000000000000000, 0.06250000000000309475, 0.09375000000000353884, 0.1250000000000039968, 0.1875000000000036637, 0.2187500000000034972, 0.2500000000000033307, 0.3125000000000037192, 0.3437500000000049960, 0.3593750000000063838, 0.3750000000000077161, 0.4375000000000158207, 0.4687500000000199285, 0.4843750000000218159, 0.5000000000000236478, 0.5625000000000337508, 0.5937500000000368594, 0.6093750000000365263, 0.6250000000000361933, 0.6875000000000408562, 0.7187500000000411893, 0.7343750000000422995, 0.7421875000000427436, 0.7500000000000434097, 0.8125000000000350830, 0.8437500000000320854, 0.8593750000000306422, 0.8671875000000300870, 0.8750000000000294209, 1.000000000000000000 ),
 .UNSPECIFIED. ) ;
#30316=CARTESIAN_POINT ( 'NONE',  ( 17.24455747906367264, 28.14336893147755347, 7.433330006724141015 ) ) ;
#30319=CARTESIAN_POINT ( 'NONE',  ( 6.194340351808173217, 26.68290643055185285, 3.479690158560446702E-15 ) ) ;
#30324=CARTESIAN_POINT ( 'NONE',  ( 72.42236640908883771, 60.72463564107695788, 14.97540514082750640 ) ) ;
#30331=CARTESIAN_POINT ( 'NONE',  ( 77.01122693365802263, 49.58419032010621663, 15.00892541147910286 ) ) ;
#30340=CARTESIAN_POINT ( 'NONE',  ( 73.10133336124690118, 70.55037490275843481, -7.932148607956638564 ) ) ;
#30343=EDGE_CURVE ( 'NONE', #27875, #91598, #22068, .T. ) ;
#30346=CARTESIAN_POINT ( 'NONE',  ( 17.52119783388728180, 25.51421378149919050, -9.188101187500004485 ) ) ;
#30347=CARTESIAN_POINT ( 'NONE',  ( 75.84489191139213915, 59.04817673520474131, 15.93577818499344545 ) ) ;
#30348=CARTESIAN_POINT ( 'NONE',  ( 67.11274794702013935, 69.23909389306264472, -1.736299782362168642 ) ) ;
#30350=ORIENTED_EDGE ( 'NONE', *, *, #77873, .T. ) ;
#30355=( BOUNDED_CURVE ( )  B_SPLINE_CURVE ( 2, ( #18244, #532, #24823, #39500, #16231, #93263, #54710, #78044, #95289, #33433, #94762, #64330, #56211 ),
 .UNSPECIFIED., .F., .T. ) 
 B_SPLINE_CURVE_WITH_KNOTS ( ( 3, 2, 2, 2, 2, 2, 3 ),
 ( 0.5625000000000000000, 0.5649999999999999467, 0.5699999999999999512, 0.5749999999999999556, 0.5799999999999999600, 0.5849999999999999645, 0.5875000000000000222 ),
 .UNSPECIFIED. ) 
 CURVE ( )  GEOMETRIC_REPRESENTATION_ITEM ( )  RATIONAL_B_SPLINE_CURVE ( ( 0.9755282581475768211, 0.9755282581475768211, 1.000000000000000000, 0.9510565162951535312, 1.000000000000000000, 0.9510565162951535312, 1.000000000000000000, 0.9510565162951535312, 1.000000000000000000, 0.9510565162951535312, 1.000000000000000000, 0.9755282581475761550, 0.9755282581475767101 ) ) 
 REPRESENTATION_ITEM ( '' )  );
#30357=CARTESIAN_POINT ( 'NONE',  ( 67.87119603988516303, 66.02582195971199042, -10.46564531199834924 ) ) ;
#30362=EDGE_CURVE ( 'NONE', #29851, #77944, #99307, .T. ) ;
#30376=CARTESIAN_POINT ( 'NONE',  ( 67.03472654747955062, 67.61602409160271066, 6.661883959231219343 ) ) ;
#30377=DIRECTION ( 'NONE',  ( 0.8660254037844339337, 0.5000000000000081046, -0.000000000000000000 ) ) ;
#30379=CARTESIAN_POINT ( 'NONE',  ( 81.19301662773271744, 55.65398007790845014, 16.37810844063417548 ) ) ;
#30386=CARTESIAN_POINT ( 'NONE',  ( 76.25939620287860521, 51.63842756541252044, -16.17602125672954116 ) ) ;
#30387=CARTESIAN_POINT ( 'NONE',  ( 76.03824915322937272, 65.38513206480712370, -14.40956150002899783 ) ) ;
#30392=ORIENTED_EDGE ( 'NONE', *, *, #79415, .F. ) ;
#30393=CARTESIAN_POINT ( 'NONE',  ( 88.22177397292790602, 44.42207723138842113, 4.484962078095955818 ) ) ;
#30397=CARTESIAN_POINT ( 'NONE',  ( 72.74690663434007831, 70.81824800135888154, 7.160589954729633000 ) ) ;
#30402=CARTESIAN_POINT ( 'NONE',  ( 82.10590413265644827, 40.80812859821141103, 1.532309608727412398 ) ) ;
#30405=CARTESIAN_POINT ( 'NONE',  ( 83.53052282221433700, 51.97849157102297113, 15.01265415031365436 ) ) ;
#30416=CARTESIAN_POINT ( 'NONE',  ( 22.87232021560678064, 28.90829794293881960, 10.00000000000000355 ) ) ;
#30419=CARTESIAN_POINT ( 'NONE',  ( 68.05994358318133663, 69.15766078933415884, -5.932084911600773225 ) ) ;
#30425=CARTESIAN_POINT ( 'NONE',  ( 67.15772368909351542, 67.74692886573922124, -6.548511843863578541 ) ) ;
#30426=CARTESIAN_POINT ( 'NONE',  ( 72.71813417941987723, 70.76084006159409512, -7.966439650937866546 ) ) ;
#30429=CARTESIAN_POINT ( 'NONE',  ( 28.31825578742223115, 28.30066082961423390, -10.00000000000000533 ) ) ;
#30432=PLANE ( 'NONE',  #23225 ) ;
#30438=CARTESIAN_POINT ( 'NONE',  ( 82.01460820302004606, 41.19402847427713255, 5.465372724684262273 ) ) ;
#30442=CARTESIAN_POINT ( 'NONE',  ( 66.43767850218320348, 67.94397599821699885, 6.523424134266977426 ) ) ;
#30444=CARTESIAN_POINT ( 'NONE',  ( 40.83172133312034191, 29.28920272979929962, -7.433330006724141015 ) ) ;
#30445=B_SPLINE_CURVE_WITH_KNOTS ( 'NONE', 3,
 ( #79744, #10808, #34591, #95947, #18919, #65990, #87867, #65490, #56388, #79248, #65004, #96439, #96943, #57386, #95461, #27509, #87384, #27003, #81240, #26508, #49792, #17391, #3711, #10306, #88360, #50287, #88866, #71619, #19431, #2215, #63992, #41178, #33096, #72114, #2718, #64501, #94934, #17913, #26013, #33606, #9820, #56884, #18413, #49304, #80755, #80241 ),
 .UNSPECIFIED., .F., .F.,
 ( 4, 1, 1, 1, 2, 2, 1, 1, 1, 2, 2, 1, 1, 2, 2, 1, 1, 2, 2, 1, 1, 2, 2, 1, 2, 2, 1, 2, 2, 4 ),
 ( 0.000000000000000000, 0.06249999999997297995, 0.09374999999995986544, 0.1093749999999537453, 0.1171874999999507477, 0.1249999999999477640, 0.1874999999999338307, 0.2187499999999278633, 0.2343749999999247824, 0.2421874999999236722, 0.2499999999999225064, 0.3124999999999218403, 0.3437499999999210631, 0.3593749999999211187, 0.3749999999999211742, 0.4374999999999245048, 0.4687499999999255040, 0.4843749999999260591, 0.4999999999999266143, 0.5624999999999341638, 0.5937499999999384936, 0.6093749999999407141, 0.6249999999999429345, 0.6874999999999559241, 0.7187499999999609201, 0.7499999999999659162, 0.8124999999999746869, 0.8437499999999790168, 0.8749999999999834577, 1.000000000000000000 ),
 .UNSPECIFIED. ) ;
#30452=CARTESIAN_POINT ( 'NONE',  ( 17.52119783388727825, 25.51421378149919050, -9.188101187500004485 ) ) ;
#30454=CARTESIAN_POINT ( 'NONE',  ( 71.59150237832598407, 59.07131284048556807, 15.33293140476554228 ) ) ;
#30455=EDGE_CURVE ( 'NONE', #17810, #65477, #66066, .T. ) ;
#30457=ORIENTED_EDGE ( 'NONE', *, *, #39740, .T. ) ;
#30459=CARTESIAN_POINT ( 'NONE',  ( 75.27202081363431319, 53.54715819699419654, -16.04939499529041669 ) ) ;
#30461=CARTESIAN_POINT ( 'NONE',  ( 81.88875743029853993, 42.19903267382473189, 7.633282463442304433 ) ) ;
#30463=FACE_OUTER_BOUND ( 'NONE', #23935, .T. ) ;
#30464=CARTESIAN_POINT ( 'NONE',  ( 72.61981592835454080, 71.39147990323394311, -5.869544098407574850 ) ) ;
#30465=CARTESIAN_POINT ( 'NONE',  ( 72.60664467684684098, 57.18896317022895914, 16.35683965500042802 ) ) ;
#30470=CARTESIAN_POINT ( 'NONE',  ( 83.36585540513543435, 42.45426523848973943, -5.297942810992300799 ) ) ;
#30475=CARTESIAN_POINT ( 'NONE',  ( 79.89992946763821635, 58.05382247932297446, 16.26787594119393532 ) ) ;
#30476=CARTESIAN_POINT ( 'NONE',  ( 67.09773762330524960, 69.34340978576997827, -3.906684184505462731 ) ) ;
#30488=CARTESIAN_POINT ( 'NONE',  ( 78.18897306460242191, 47.59851855797241171, -14.42851076044696335 ) ) ;
#30489=EDGE_LOOP ( 'NONE', ( #68714, #23584, #96579, #4458 ) ) ;
#30494=CARTESIAN_POINT ( 'NONE',  ( 41.21417716447173518, 24.76426979415093044, 3.090169943749476733 ) ) ;
#30495=ORIENTED_EDGE ( 'NONE', *, *, #89381, .T. ) ;
#30496=VERTEX_POINT ( 'NONE', #33422 ) ;
#30498=CARTESIAN_POINT ( 'NONE',  ( 86.64388902346107102, 46.39093904164906945, 9.083131486035911806 ) ) ;
#30506=CARTESIAN_POINT ( 'NONE',  ( 71.97959222828325210, 71.25346787330545340, 5.319870175860073935 ) ) ;
#30508=CARTESIAN_POINT ( 'NONE',  ( 66.99733635639957186, 66.90869551988777175, 8.780753403809187674 ) ) ;
#30510=CARTESIAN_POINT ( 'NONE',  ( 78.16621118571123361, 47.55685362076941658, 14.41442218299236622 ) ) ;
#30514=CARTESIAN_POINT ( 'NONE',  ( 75.72842597690201671, 54.31630180662983065, -16.10729176078631752 ) ) ;
#30517=CARTESIAN_POINT ( 'NONE',  ( 79.19657612229403298, 45.81917910958111406, 13.05272374772707700 ) ) ;
#30519=CARTESIAN_POINT ( 'NONE',  ( 82.00351712801760584, 53.66420159836799542, -15.87819945195018789 ) ) ;
#30525=CARTESIAN_POINT ( 'NONE',  ( 72.48412649147189768, 71.58981433514404102, 5.211472423265571585 ) ) ;
#30530=EDGE_CURVE ( 'NONE', #48310, #33772, #16220, .T. ) ;
#30536=CARTESIAN_POINT ( 'NONE',  ( 85.70574795423719650, 48.48025216897318046, -12.24584271313006312 ) ) ;
#30537=ORIENTED_EDGE ( 'NONE', *, *, #63705, .T. ) ;
#30538=CARTESIAN_POINT ( 'NONE',  ( 70.94537046311441486, 63.12358859840954040, 13.51887736991167621 ) ) ;
#30540=B_SPLINE_CURVE_WITH_KNOTS ( 'NONE', 3,
 ( #229, #31114, #75756, #99057, #60512, #22028, #23854, #86224, #94801, #95328, #18281, #94307, #24859, #16262, #17261, #48165, #63862, #40550, #1074, #25886, #78586, #71979, #86724, #2585 ),
 .UNSPECIFIED., .F., .F.,
 ( 4, 2, 2, 2, 2, 2, 2, 2, 2, 2, 2, 4 ),
 ( 0.000000000000000000, 0.1250000000000129896, 0.2500000000000259792, 0.3750000000000389688, 0.4375000000000411338, 0.5000000000000432987, 0.5625000000000454081, 0.6250000000000476286, 0.6875000000000497380, 0.7500000000000519584, 0.8750000000000259792, 1.000000000000000000 ),
 .UNSPECIFIED. ) ;
#30541=CARTESIAN_POINT ( 'NONE',  ( 74.37357505727348439, 67.95923626955014640, -11.68566301663373963 ) ) ;
#30553=AXIS2_PLACEMENT_3D ( 'NONE', #56632, #25753, #98522 ) ;
#30555=CARTESIAN_POINT ( 'NONE',  ( 84.88474621580253654, 46.65668362480882791, -11.06339629709468042 ) ) ;
#30556=AXIS2_PLACEMENT_3D ( 'NONE', #61407, #15807, #68516 ) ;
#30558=CARTESIAN_POINT ( 'NONE',  ( 7.350711452622367581, 26.01751292744054567, 6.180339887498949913 ) ) ;
#30560=CARTESIAN_POINT ( 'NONE',  ( 71.97397978244890737, 59.31999651994269840, -15.32424238813479889 ) ) ;
#30564=CARTESIAN_POINT ( 'NONE',  ( 12.74041337322552891, 7.759783934591623300, -1.583844403245364241 ) ) ;
#30566=CARTESIAN_POINT ( 'NONE',  ( 17.73406340791407843, 11.20801979619927558, -3.090169943749474069 ) ) ;
#30573=CARTESIAN_POINT ( 'NONE',  ( 37.13125039574066477, 23.29860640527294535, -2.839279412974138328 ) ) ;
#30575=CARTESIAN_POINT ( 'NONE',  ( 82.75711436980199665, 40.78606491925197730, -2.625374872848795782 ) ) ;
#30577=CARTESIAN_POINT ( 'NONE',  ( 69.02699102946681364, 64.47626555514762003, 12.46414397747164671 ) ) ;
#30579=CARTESIAN_POINT ( 'NONE',  ( 81.31146485538788227, 51.54224463187279071, 15.34331897028426717 ) ) ;
#30583=CARTESIAN_POINT ( 'NONE',  ( 6.569006713621681648, 25.83396525600388216, -2.839279412974133887 ) ) ;
#30589=CARTESIAN_POINT ( 'NONE',  ( 69.39586509779915957, 62.82256197253910557, 13.14397930765713163 ) ) ;
#30590=EDGE_CURVE ( 'NONE', #69830, #59778, #77416, .T. ) ;
#30596=ORIENTED_EDGE ( 'NONE', *, *, #81673, .T. ) ;
#30598=CARTESIAN_POINT ( 'NONE',  ( 72.49881181205529401, 70.63619014701561127, 7.225229806400220056 ) ) ;
#30602=CARTESIAN_POINT ( 'NONE',  ( 83.25213841147557048, 45.25846362796585964, -9.926727695915893435 ) ) ;
#30603=ORIENTED_EDGE ( 'NONE', *, *, #76353, .T. ) ;
#30604=EDGE_CURVE ( 'NONE', #17646, #39570, #32796, .T. ) ;
#30607=CARTESIAN_POINT ( 'NONE',  ( 15.49551970000783996, 14.11029122506293021, -8.090169943749478065 ) ) ;
#30609=CARTESIAN_POINT ( 'NONE',  ( 69.60809846375656207, 62.55097647278505235, 13.37551271588222690 ) ) ;
#30613=CARTESIAN_POINT ( 'NONE',  ( 73.27146650943220152, 69.63413511619549467, -9.919440617956860606 ) ) ;
#30619=EDGE_CURVE ( 'NONE', #25393, #16493, #63157, .T. ) ;
#30621=CARTESIAN_POINT ( 'NONE',  ( 81.41849629226379648, 50.07632656148466310, 14.25717219674097791 ) ) ;
#30622=VERTEX_POINT ( 'NONE', #78931 ) ;
#30623=CARTESIAN_POINT ( 'NONE',  ( 67.79074041082746760, 67.79995302995581596, 7.165554312747186572 ) ) ;
#30624=CARTESIAN_POINT ( 'NONE',  ( 87.89296955652562815, 44.95200477618789137, 6.297572492595292282 ) ) ;
#30631=CARTESIAN_POINT ( 'NONE',  ( 82.44310520575160695, 54.28011738120409291, -15.96781897959228758 ) ) ;
#30633=CARTESIAN_POINT ( 'NONE',  ( 15.73863525846626032, 14.80170272979925272, 7.433330006724137462 ) ) ;
#30642=DIRECTION ( 'NONE',  ( -0.8660254037844378194, -0.5000000000000014433, -0.000000000000000000 ) ) ;
#30643=CARTESIAN_POINT ( 'NONE',  ( 81.66383133520196225, 46.03416481792814352, -11.52458638852417572 ) ) ;
#30646=AXIS2_PLACEMENT_3D ( 'NONE', #22856, #36186, #76570 ) ;
#30651=CARTESIAN_POINT ( 'NONE',  ( 74.89378789817061488, 62.29972416502009480, -14.99401956569568561 ) ) ;
#30658=CARTESIAN_POINT ( 'NONE',  ( 72.87908800440395396, 70.94240749453250316, 7.824389999597029188 ) ) ;
#30660=CARTESIAN_POINT ( 'NONE',  ( 76.22741562560636908, 65.24129761985034293, 14.53304928680089958 ) ) ;
#30663=EDGE_LOOP ( 'NONE', ( #54894, #54906, #83862, #33710 ) ) ;
#30667=( BOUNDED_CURVE ( )  B_SPLINE_CURVE ( 2, ( #54831, #70032, #24446, #646, #31532, #15322, #22935 ),
 .UNSPECIFIED., .F., .T. ) 
 B_SPLINE_CURVE_WITH_KNOTS ( ( 3, 2, 2, 3 ),
 ( 0.9875000000000000444, 0.9899999999999999911, 0.9949999999999999956, 1.000000000000000000 ),
 .UNSPECIFIED. ) 
 CURVE ( )  GEOMETRIC_REPRESENTATION_ITEM ( )  RATIONAL_B_SPLINE_CURVE ( ( 0.9755282581475767101, 0.9755282581475772652, 1.000000000000000000, 0.9510565162951535312, 1.000000000000000000, 0.9510565162951535312, 1.000000000000000000 ) ) 
 REPRESENTATION_ITEM ( '' )  );
#30668=CARTESIAN_POINT ( 'NONE',  ( 84.02246009045383346, 46.28810143914654418, -10.58215992841521391 ) ) ;
#30671=CARTESIAN_POINT ( 'NONE',  ( 81.83475763163420424, 42.02284892325379673, 6.270888180158195269 ) ) ;
#30687=CARTESIAN_POINT ( 'NONE',  ( 71.33995758461628611, 71.62702440093282519, 2.627031368899047870 ) ) ;
#30688=CARTESIAN_POINT ( 'NONE',  ( 80.68240590561059378, 44.01878066398630551, 10.12792899481129894 ) ) ;
#30694=CARTESIAN_POINT ( 'NONE',  ( 20.18540868186541459, 12.44966523072493914, -2.296566073217252530E-15 ) ) ;
#30695=CARTESIAN_POINT ( 'NONE',  ( 77.56874017944556954, 59.32837778823116537, -16.45541604924300927 ) ) ;
#30696=VECTOR ( 'NONE', #64022, 1000.000000000000114 ) ;
#30705=CARTESIAN_POINT ( 'NONE',  ( 66.13428293896411958, 69.21728233722956247, 1.665249920595609501 ) ) ;
#30707=CARTESIAN_POINT ( 'NONE',  ( 24.06271987006732616, 35.93396525600390845, 2.839279412974139660 ) ) ;
#30720=CARTESIAN_POINT ( 'NONE',  ( 27.74993340135631215, 36.99752408145592852, 5.678558825948277544 ) ) ;
#30722=CARTESIAN_POINT ( 'NONE',  ( 66.57026871561890857, 68.76443072695623471, 4.738950751700697239 ) ) ;
#30725=EDGE_LOOP ( 'NONE', ( #65560, #40465, #29411, #16151, #92685, #77370 ) ) ;
#30727=CARTESIAN_POINT ( 'NONE',  ( 86.37995054896607883, 46.98508828575033647, -10.52062608394496479 ) ) ;
#30734=CARTESIAN_POINT ( 'NONE',  ( 81.63547489262985835, 55.73921394657421757, -16.35272683298455121 ) ) ;
#30743=CARTESIAN_POINT ( 'NONE',  ( 84.38175156668881982, 50.02035787987339432, 13.81135446509517628 ) ) ;
#30749=CARTESIAN_POINT ( 'NONE',  ( 71.19320197529700067, 61.90671673094616523, -14.21225849412795306 ) ) ;
#30750=CARTESIAN_POINT ( 'NONE',  ( 82.72861693379122983, 40.56744065827609802, 0.9164833145372243139 ) ) ;
#30752=CARTESIAN_POINT ( 'NONE',  ( 77.00376392975798012, 63.39239755058648029, -15.46687034352795109 ) ) ;
#30755=ORIENTED_EDGE ( 'NONE', *, *, #94882, .T. ) ;
#30757=CARTESIAN_POINT ( 'NONE',  ( 41.44395331530407844, 35.87878583063845639, -9.188101187500006262 ) ) ;
#30760=CARTESIAN_POINT ( 'NONE',  ( 74.15402199957247831, 68.42859570829774896, -11.65141325894000879 ) ) ;
#30761=CARTESIAN_POINT ( 'NONE',  ( 72.74506803476772632, 63.63576506029848190, -13.82193098727775649 ) ) ;
#30764=CARTESIAN_POINT ( 'NONE',  ( 72.85138575605425615, 64.91499728177296902, 13.16331341298753088 ) ) ;
#30794=CARTESIAN_POINT ( 'NONE',  ( 74.27315540778812419, 65.63952288200199803, -13.71985095672392774 ) ) ;
#30799=CARTESIAN_POINT ( 'NONE',  ( 78.75297625639956323, 47.66336229257159118, 14.29739783539339371 ) ) ;
#30801=CARTESIAN_POINT ( 'NONE',  ( 84.67010498191464762, 49.80963328464838469, -13.17095790170508174 ) ) ;
#30803=CARTESIAN_POINT ( 'NONE',  ( 73.36014537180697914, 69.17374614814826828, -9.939646048807338374 ) ) ;
#30804=CARTESIAN_POINT ( 'NONE',  ( 76.10825311040436247, 51.34890012828683581, 15.64337078650107671 ) ) ;
#30813=CARTESIAN_POINT ( 'NONE',  ( 87.94829491887652750, 43.95349485838026027, 0.4967466087338212044 ) ) ;
#30814=CARTESIAN_POINT ( 'NONE',  ( 76.47316661484272515, 51.61210842333346704, -15.65491330287230376 ) ) ;
#30816=CARTESIAN_POINT ( 'NONE',  ( 66.61806446105697432, 69.58935570732562326, -0.3124497180235544791 ) ) ;
#30818=CARTESIAN_POINT ( 'NONE',  ( 26.97531487256933858, 21.28920272979927830, -7.433330006724141015 ) ) ;
#30821=CARTESIAN_POINT ( 'NONE',  ( 10.03310832875943603, 27.83396525600388571, -2.839279412974133887 ) ) ;
#30823=CARTESIAN_POINT ( 'NONE',  ( 76.77756057274272905, 63.67496528870245243, 15.32214893988671101 ) ) ;
#30824=CARTESIAN_POINT ( 'NONE',  ( 76.19481306539471177, 60.31832523138206170, 16.18231617239213094 ) ) ;
#30827=CARTESIAN_POINT ( 'NONE',  ( 76.48733475582915275, 56.37564448157380781, -16.15952532856388046 ) ) ;
#30832=CARTESIAN_POINT ( 'NONE',  ( 77.13981730435806128, 49.50565677253940322, 14.95469319025198196 ) ) ;
#30837=CARTESIAN_POINT ( 'NONE',  ( 69.01668676381960665, 68.81684766018636878, -6.622719373402289555 ) ) ;
#30839=B_SPLINE_CURVE_WITH_KNOTS ( 'NONE', 3,
 ( #85982, #16509, #47404, #78331, #99136, #29722, #60596, #22120, #83966, #2843, #96062, #71739, #18530, #9418, #63112, #48924, #49413, #26621, #41297, #79367, #11444, #80360, #65114, #10424, #33733, #56508, #79861, #10931, #40793, #25624, #87497 ),
 .UNSPECIFIED., .F., .F.,
 ( 4, 3, 3, 3, 3, 3, 3, 3, 3, 3, 4 ),
 ( 0.000000000000000000, 0.1333490885032345696, 0.3007194338854333737, 0.4699862290245237495, 0.5844252810809289489, 0.6686540514502742338, 0.7354980260655397117, 0.8028463152565420424, 0.8633854507756993923, 0.9437142632667149256, 1.000000000000000000 ),
 .UNSPECIFIED. ) ;
#30843=ORIENTED_EDGE ( 'NONE', *, *, #2938, .T. ) ;
#30844=CARTESIAN_POINT ( 'NONE',  ( 23.93942162470478507, 34.79752408145593279, -5.678558825948271327 ) ) ;
#30845=CARTESIAN_POINT ( 'NONE',  ( 74.83966849089097195, 54.13869872289780005, 16.11807719370478864 ) ) ;
#30847=CARTESIAN_POINT ( 'NONE',  ( 74.93756780616696744, 67.42216207915814152, -12.80861374294490318 ) ) ;
#30848=ORIENTED_EDGE ( 'NONE', *, *, #48882, .T. ) ;
#30849=FACE_OUTER_BOUND ( 'NONE', #17763, .T. ) ;
#30856=CARTESIAN_POINT ( 'NONE',  ( 71.17266338141718052, 64.03727702359581997, 13.60747010924504607 ) ) ;
#30857=CARTESIAN_POINT ( 'NONE',  ( 67.96557359005117860, 65.23838819696450742, -10.59734309696486143 ) ) ;
#30874=CARTESIAN_POINT ( 'NONE',  ( 80.17557668363483003, 44.21690606740114049, -11.32705747359858073 ) ) ;
#30879=CARTESIAN_POINT ( 'NONE',  ( 71.34493322773809609, 66.48664206392754750, 11.31262581298163106 ) ) ;
#30884=CARTESIAN_POINT ( 'NONE',  ( 24.86476902620765728, 14.75978393459164373, -1.583844403245362020 ) ) ;
#30887=CARTESIAN_POINT ( 'NONE',  ( 83.72772921281246283, 41.65051315404114263, 0.2546602532276703301 ) ) ;
#30893=CARTESIAN_POINT ( 'NONE',  ( 82.27584197377750286, 43.65791533439266203, -8.572228566050736021 ) ) ;
#30895=CARTESIAN_POINT ( 'NONE',  ( 31.97641226934276659, 34.16454794089042935, -10.00000000000000355 ) ) ;
#30897=CARTESIAN_POINT ( 'NONE',  ( 72.67131491517322672, 70.78719139597193077, 7.139508363488885401 ) ) ;
#30903=CARTESIAN_POINT ( 'NONE',  ( 79.83962644441906775, 47.32072031626830722, 13.19797558408899008 ) ) ;
#30904=CARTESIAN_POINT ( 'NONE',  ( 83.78524573913310292, 52.15075186824800824, 14.63520302633205361 ) ) ;
#30912=CARTESIAN_POINT ( 'NONE',  ( 73.68661752955311783, 55.32924942141305280, 16.59143442441305538 ) ) ;
#30913=CARTESIAN_POINT ( 'NONE',  ( 23.20344070249937829, 32.13478043621388736, 8.090169943749478065 ) ) ;
#30923=CARTESIAN_POINT ( 'NONE',  ( 66.71451521809625262, 67.43874277882086687, -6.652223803815810577 ) ) ;
#30924=CARTESIAN_POINT ( 'NONE',  ( 72.86429505109983040, 70.96802964124921687, -7.768747002037665439 ) ) ;
#30925=CARTESIAN_POINT ( 'NONE',  ( 81.85952891566994083, 41.18668495682469910, 5.665119147071315808 ) ) ;
#30929=CARTESIAN_POINT ( 'NONE',  ( 25.81463925578599117, 37.83705186507755514, 3.090169943749475401 ) ) ;
#30930=CARTESIAN_POINT ( 'NONE',  ( 85.32181490816766711, 42.56115037135857904, -1.119015723361847181 ) ) ;
#30933=CARTESIAN_POINT ( 'NONE',  ( 82.08779928828076322, 42.49253994542575441, 7.931423503822311538 ) ) ;
#30938=CARTESIAN_POINT ( 'NONE',  ( 72.41389820116259557, 70.72247311216293042, 7.745007521649655224 ) ) ;
#30940=CARTESIAN_POINT ( 'NONE',  ( 72.62340041749851594, 70.70648146094340802, -7.965908336710430859 ) ) ;
#30941=CARTESIAN_POINT ( 'NONE',  ( 32.37774987120970849, 30.64441083166263269, -10.00000000000000533 ) ) ;
#30945=DIRECTION ( 'NONE',  ( -0.4999999999999982792, 0.8660254037844398178, 0.000000000000000000 ) ) ;
#30948=CARTESIAN_POINT ( 'NONE',  ( 24.30746885452586525, 16.96004757982090183, -5.678558825948276656 ) ) ;
#30950=CARTESIAN_POINT ( 'NONE',  ( 72.02510489751692546, 59.23144522310215621, 15.85746550207202077 ) ) ;
#30953=CARTESIAN_POINT ( 'NONE',  ( 3.154811933878272523, 22.79752408145589371, -5.678558825948271327 ) ) ;
#30954=CARTESIAN_POINT ( 'NONE',  ( 71.71174882302004505, 58.93038559421764688, -15.88944412480316970 ) ) ;
#30955=CARTESIAN_POINT ( 'NONE',  ( 88.24655134174822990, 44.28719395207696863, 2.070298746488927755 ) ) ;
#30960=CARTESIAN_POINT ( 'NONE',  ( 72.52865609843787809, 57.51546068812135815, 16.29679984377914437 ) ) ;
#30979=CARTESIAN_POINT ( 'NONE',  ( 33.05914333415502426, 24.80170272979928470, 7.433330006724137462 ) ) ;
#30981=CARTESIAN_POINT ( 'NONE',  ( 78.32728443519724237, 47.41824214893080836, -13.74674985590325171 ) ) ;
#30987=CARTESIAN_POINT ( 'NONE',  ( 31.59942275858663407, 40.01751292744058475, 6.180339887498949913 ) ) ;
#30992=CARTESIAN_POINT ( 'NONE',  ( 82.61830983956946284, 42.72265058836246254, -6.751676072530465866 ) ) ;
#30999=CARTESIAN_POINT ( 'NONE',  ( 69.50090580276174990, 66.60780273872985902, 10.14006215365368924 ) ) ;
#31001=CARTESIAN_POINT ( 'NONE',  ( 75.73213429733796431, 65.60614264062904510, 13.80850863069982992 ) ) ;
#31003=CARTESIAN_POINT ( 'NONE',  ( 78.46010992227571990, 47.82667959050288431, 13.91303883740862624 ) ) ;
#31005=ORIENTED_EDGE ( 'NONE', *, *, #6401, .T. ) ;
#31015=CARTESIAN_POINT ( 'NONE',  ( 72.46511837996447980, 71.56249752072032777, 6.234640293157911017 ) ) ;
#31024=CARTESIAN_POINT ( 'NONE',  ( 85.76025348255959102, 48.54612661500244997, -11.80603267945767954 ) ) ;
#31030=CARTESIAN_POINT ( 'NONE',  ( 72.94085775465440236, 59.22282884362820710, 16.00814023073137093 ) ) ;
#31037=CARTESIAN_POINT ( 'NONE',  ( 15.09101445147005727, 32.21091486745859811, -1.111400068045478839E-16 ) ) ;
#31039=EDGE_CURVE ( 'NONE', #93933, #51005, #78740, .T. ) ;
#31041=CARTESIAN_POINT ( 'NONE',  ( 86.46651626576456806, 46.39758167564458802, -9.828513499124806430 ) ) ;
#31043=CARTESIAN_POINT ( 'NONE',  ( 18.87072174683323666, 11.86426979415088745, -3.090169943749474069 ) ) ;
#31046=CARTESIAN_POINT ( 'NONE',  ( 73.21379494821863432, 69.78953872660252955, 9.103517464032861994 ) ) ;
#31050=CARTESIAN_POINT ( 'NONE',  ( 73.00502472597065662, 57.20524681399147227, 15.90417734607904876 ) ) ;
#31056=CARTESIAN_POINT ( 'NONE',  ( 30.58134869734400851, 35.84336893147758474, -7.433330006724137462 ) ) ;
#31060=CARTESIAN_POINT ( 'NONE',  ( 88.46324942983896733, 43.96425106107526659, 1.817931795122161631 ) ) ;
#31061=CARTESIAN_POINT ( 'NONE',  ( 65.81518118656045147, 68.94946510510605719, 2.247327669414935780 ) ) ;
#31065=CARTESIAN_POINT ( 'NONE',  ( 83.42542119994750749, 51.64995580955420706, -14.90072893730332027 ) ) ;
#31066=CARTESIAN_POINT ( 'NONE',  ( 17.35761498915574563, 12.94754757982088478, 5.678558825948272215 ) ) ;
#31071=CARTESIAN_POINT ( 'NONE',  ( 71.57943482431289794, 72.41997303871666247, 0.9858917062509267026 ) ) ;
#31077=EDGE_LOOP ( 'NONE', ( #65239, #10656, #53868, #74867 ) ) ;
#31081=CARTESIAN_POINT ( 'NONE',  ( 21.98544502579644799, 24.64441083166261137, -10.00000000000000533 ) ) ;
#31083=CARTESIAN_POINT ( 'NONE',  ( 86.94567315205141256, 44.99287267174491234, -6.599641438898517620 ) ) ;
#31087=FACE_OUTER_BOUND ( 'NONE', #50181, .T. ) ;
#31090=CARTESIAN_POINT ( 'NONE',  ( 69.89538980332476115, 62.79524207331544972, 13.90205096215579950 ) ) ;
#31094=CARTESIAN_POINT ( 'NONE',  ( 66.10228174255657052, 68.64626758096548542, 4.271897712742703135 ) ) ;
#31099=CARTESIAN_POINT ( 'NONE',  ( 74.50658829527574767, 66.53799963998996247, 12.80246580919608235 ) ) ;
#31101=CARTESIAN_POINT ( 'NONE',  ( 70.85244465605627795, 71.45066637977274127, 2.090713904591689598 ) ) ;
#31104=CARTESIAN_POINT ( 'NONE',  ( 81.47863721931979342, 44.48187038564707052, 10.12635968134262399 ) ) ;
#31108=CARTESIAN_POINT ( 'NONE',  ( 82.87162244869749372, 53.63483014063397292, -15.36256874745430245 ) ) ;
#31112=CARTESIAN_POINT ( 'NONE',  ( 17.90851666933368236, 18.84335787977762777, 9.188101187500006262 ) ) ;
#31114=CARTESIAN_POINT ( 'NONE',  ( 85.69555808373030459, 48.70564388484159224, 11.94729400084767157 ) ) ;
#31120=CARTESIAN_POINT ( 'NONE',  ( 82.21697353817442888, 45.95328030435120326, -11.18469232000785496 ) ) ;
#31129=CARTESIAN_POINT ( 'NONE',  ( 16.00201260034520345, 10.20801979619927380, -3.090169943749474069 ) ) ;
#31131=LINE ( 'NONE', #62024, #82406 ) ;
#31137=VERTEX_POINT ( 'NONE', #31999 ) ;
#31140=CARTESIAN_POINT ( 'NONE',  ( 82.17887713766984348, 46.62351855337478668, -11.80422335332041328 ) ) ;
#31148=ORIENTED_EDGE ( 'NONE', *, *, #80431, .T. ) ;
#31154=CARTESIAN_POINT ( 'NONE',  ( 34.10980067877857635, 31.64441083166263269, -10.00000000000000533 ) ) ;
#31158=CARTESIAN_POINT ( 'NONE',  ( 81.08332877246739656, 43.92371124442119168, 10.53733257259109735 ) ) ;
#31161=EDGE_CURVE ( 'NONE', #11833, #97853, #48596, .T. ) ;
#31165=CARTESIAN_POINT ( 'NONE',  ( 67.78251950854047436, 66.97470367889792442, 8.421653629368158533 ) ) ;
#31173=CARTESIAN_POINT ( 'NONE',  ( 14.76917458061509514, 17.03085787977762067, 9.188101187500006262 ) ) ;
#31183=CARTESIAN_POINT ( 'NONE',  ( 86.43642008611649885, 47.55668332166565904, 10.53568000035417995 ) ) ;
#31184=ORIENTED_EDGE ( 'NONE', *, *, #28905, .T. ) ;
#31186=CARTESIAN_POINT ( 'NONE',  ( 27.63686232447692603, 34.14336893147756768, 7.433330006724141015 ) ) ;
#31187=DIRECTION ( 'NONE',  ( 0.4493970231495826861, -0.7783784768652872721, -0.4383711467890751834 ) ) ;
#31192=B_SPLINE_CURVE_WITH_KNOTS ( 'NONE', 3,
 ( #40015, #63833, #55215, #33439, #87715, #18250, #1555, #86197, #80080, #39016, #538, #31423, #81086, #72467, #89203, #65335, #89684, #82081, #66333, #19751, #35922, #18749, #88197, #33958 ),
 .UNSPECIFIED., .F., .F.,
 ( 4, 2, 2, 2, 2, 2, 2, 2, 2, 2, 2, 4 ),
 ( 0.000000000000000000, 0.1250000000000164591, 0.2500000000000329181, 0.3750000000000494049, 0.4375000000000497935, 0.5000000000000501821, 0.5625000000000506262, 0.6250000000000510703, 0.6875000000000515143, 0.7500000000000519584, 0.8750000000000260902, 1.000000000000000000 ),
 .UNSPECIFIED. ) ;
#31194=CARTESIAN_POINT ( 'NONE',  ( 78.82603149318642011, 48.82109720856274748, 14.29823851343999941 ) ) ;
#31196=DIRECTION ( 'NONE',  ( -0.8660254037844377084, -0.5000000000000014433, -0.000000000000000000 ) ) ;
#31197=CARTESIAN_POINT ( 'NONE',  ( 74.90541669563339156, 53.37575215131342077, -16.53204517015438313 ) ) ;
#31199=EDGE_CURVE ( 'NONE', #31328, #44296, #61835, .T. ) ;
#31201=CARTESIAN_POINT ( 'NONE',  ( 73.36774340952439388, 69.90371635966560859, 9.665654898056800448 ) ) ;
#31202=CARTESIAN_POINT ( 'NONE',  ( 42.00264329202813229, 26.11110640527295601, -2.839279412974138328 ) ) ;
#31209=CARTESIAN_POINT ( 'NONE',  ( 86.23632586776285791, 46.97348825937578454, -10.05460913028329450 ) ) ;
#31213=CARTESIAN_POINT ( 'NONE',  ( 80.81722803126136512, 44.69323391722993932, -11.42900611749914219 ) ) ;
#31215=CARTESIAN_POINT ( 'NONE',  ( 81.62115332376640708, 55.85468755722441614, -16.37141313285761157 ) ) ;
#31221=CARTESIAN_POINT ( 'NONE',  ( 77.36600796148924530, 49.13692148722834929, -14.77749963168139935 ) ) ;
#31228=CARTESIAN_POINT ( 'NONE',  ( 67.70770923549420672, 67.39958653419566303, 8.673274222080605611 ) ) ;
#31230=CARTESIAN_POINT ( 'NONE',  ( 82.57037383359188709, 41.04081928364340115, 1.106021355371193282 ) ) ;
#31236=CARTESIAN_POINT ( 'NONE',  ( 42.85004829832550399, 33.24335787977766188, -9.188101187500008038 ) ) ;
#31240=CARTESIAN_POINT ( 'NONE',  ( 86.89657730260137214, 45.77512320498411214, -8.683907937581334835 ) ) ;
#31251=EDGE_LOOP ( 'NONE', ( #63547, #20393, #22560, #58374 ) ) ;
#31267=CARTESIAN_POINT ( 'NONE',  ( 72.85462391432039908, 67.11347816504185460, 11.56953996784876715 ) ) ;
#31276=CARTESIAN_POINT ( 'NONE',  ( 70.56242779276917076, 66.53244391737094077, -11.50149545576417864 ) ) ;
#31278=CARTESIAN_POINT ( 'NONE',  ( 67.35448364888117112, 66.58801464723161700, 8.610823906226203306 ) ) ;
#31285=CARTESIAN_POINT ( 'NONE',  ( 66.57026871561892278, 68.76443072695623471, 4.738950751700696351 ) ) ;
#31286=CARTESIAN_POINT ( 'NONE',  ( 73.72251996588057921, 69.48154048452748555, -9.822749744319873244 ) ) ;
#31287=CARTESIAN_POINT ( 'NONE',  ( 76.01988506423570868, 51.27439951277732177, 16.12938561522662440 ) ) ;
#31289=EDGE_CURVE ( 'NONE', #30119, #86428, #50906, .T. ) ;
#31299=CARTESIAN_POINT ( 'NONE',  ( 88.28592015977812935, 44.16006502160690417, -0.2344584660016976740 ) ) ;
#31302=CARTESIAN_POINT ( 'NONE',  ( 77.71695824120645568, 49.45779813244274692, 15.33409790704233977 ) ) ;
#31304=CARTESIAN_POINT ( 'NONE',  ( 31.21402144970675252, 20.94754757982090609, 5.678558825948272215 ) ) ;
#31305=CARTESIAN_POINT ( 'NONE',  ( 81.58050098450105736, 59.42274603127592769, -0.3830222215594929480 ) ) ;
#31306=CARTESIAN_POINT ( 'NONE',  ( 81.70770681640576072, 47.33369484184763820, -12.52618337250604519 ) ) ;
#31307=CARTESIAN_POINT ( 'NONE',  ( 9.658441966945924051, 28.68290643055185996, 3.479690158560446702E-15 ) ) ;
#31309=CARTESIAN_POINT ( 'NONE',  ( 77.20294869268629157, 63.53692916728167006, 15.07858399788869797 ) ) ;
#31312=CARTESIAN_POINT ( 'NONE',  ( 66.77376812102318127, 68.41195941748605946, -4.433129028897194068 ) ) ;
#31315=CARTESIAN_POINT ( 'NONE',  ( 81.12641806927595667, 54.67637760867621211, -15.82913326966788681 ) ) ;
#31322=CARTESIAN_POINT ( 'NONE',  ( 76.93135750435078535, 49.70919492771366777, 15.06818509151668195 ) ) ;
#31323=CARTESIAN_POINT ( 'NONE',  ( 82.62974588365311490, 53.86145749464595411, 15.83045060744369970 ) ) ;
#31324=EDGE_LOOP ( 'NONE', ( #37563, #99329, #87977, #94808 ) ) ;
#31327=CARTESIAN_POINT ( 'NONE',  ( 68.60042634697137487, 68.76562077347861646, -6.227687874156614178 ) ) ;
#31328=VERTEX_POINT ( 'NONE', #20696 ) ;
#31338=CARTESIAN_POINT ( 'NONE',  ( 19.72598728594001116, 34.49540643055188127, 3.479690158560446702E-15 ) ) ;
#31339=CARTESIAN_POINT ( 'NONE',  ( 75.04415442720188878, 55.04612442798951832, 16.14546943093221287 ) ) ;
#31341=CARTESIAN_POINT ( 'NONE',  ( 75.17086645518898536, 66.39979144248444243, -13.15673120748005154 ) ) ;
#31346=VERTEX_POINT ( 'NONE', #21686 ) ;
#31348=CARTESIAN_POINT ( 'NONE',  ( 67.78299301307349367, 65.68149062186182618, 10.02826371555679152 ) ) ;
#31349=CARTESIAN_POINT ( 'NONE',  ( 67.70479547160532263, 65.84759395738886667, -10.55275263577380862 ) ) ;
#31350=CARTESIAN_POINT ( 'NONE',  ( 81.63285811411603277, 55.18114913913488806, -15.91372994156266962 ) ) ;
#31365=CARTESIAN_POINT ( 'NONE',  ( 80.20857538931046804, 44.21345027830163588, -11.30608575784165026 ) ) ;
#31368=DIRECTION ( 'NONE',  ( -0.8660254037844378194, -0.5000000000000014433, -0.000000000000000000 ) ) ;
#31378=CARTESIAN_POINT ( 'NONE',  ( 76.01947567912945658, 65.31078134063972129, -14.44091581795174051 ) ) ;
#31384=CARTESIAN_POINT ( 'NONE',  ( 83.53255499166944276, 43.67462638228406036, -7.537004589607056104 ) ) ;
#31390=CARTESIAN_POINT ( 'NONE',  ( 68.89583508828081904, 67.43123359013807772, -8.727553619782785432 ) ) ;
#31391=ORIENTED_EDGE ( 'NONE', *, *, #36249, .F. ) ;
#31396=CARTESIAN_POINT ( 'NONE',  ( 83.78171082742430542, 51.97306301863908828, 14.95037678041455109 ) ) ;
#31404=CARTESIAN_POINT ( 'NONE',  ( 73.61770819056830817, 55.44860389765071318, 16.11080357623078640 ) ) ;
#31407=CARTESIAN_POINT ( 'NONE',  ( 31.17504386912796477, 20.12755873383627758, -6.180339887498949025 ) ) ;
#31409=CARTESIAN_POINT ( 'NONE',  ( 86.13879346367242817, 46.95025718893441535, -10.63009676298478823 ) ) ;
#31419=CARTESIAN_POINT ( 'NONE',  ( 31.58830253577720626, 26.43677371833803846, -10.00000000000000355 ) ) ;
#31420=CARTESIAN_POINT ( 'NONE',  ( 84.50369441069709353, 42.22801554421776160, -2.143854648006744856 ) ) ;
#31423=CARTESIAN_POINT ( 'NONE',  ( 87.17616255865019070, 46.12350222913486419, -8.288611607450606655 ) ) ;
#31426=CARTESIAN_POINT ( 'NONE',  ( 73.10444574000553075, 66.28578448752213603, -12.33233823302241028 ) ) ;
#31430=CARTESIAN_POINT ( 'NONE',  ( 70.50721453739950562, 70.25575512013267598, -6.612918012354620068 ) ) ;
#31433=CARTESIAN_POINT ( 'NONE',  ( 67.41248320326424448, 66.37693208286884783, -8.946798147498737919 ) ) ;
#31435=B_SPLINE_CURVE_WITH_KNOTS ( 'NONE', 3,
 ( #67317, #68314, #29823, #76913, #91656, #90680, #21236, #22728, #60697, #22221 ),
 .UNSPECIFIED., .F., .F.,
 ( 4, 2, 2, 2, 4 ),
 ( 0.000000000000000000, 0.2499999999999997780, 0.4999999999999998890, 0.7500000000000000000, 1.000000000000000000 ),
 .UNSPECIFIED. ) ;
#31439=CARTESIAN_POINT ( 'NONE',  ( 16.63655203261577498, 31.64646525600389637, -2.839279412974133887 ) ) ;
#31441=CARTESIAN_POINT ( 'NONE',  ( 71.66445348058819320, 59.04578686578420132, 15.35137124261116348 ) ) ;
#31444=CARTESIAN_POINT ( 'NONE',  ( 39.30595310148520838, 34.64441083166263979, -10.00000000000000533 ) ) ;
#31445=CARTESIAN_POINT ( 'NONE',  ( 9.401013375279877238, 17.37878583063838889, 9.188101187500006262 ) ) ;
#31446=CARTESIAN_POINT ( 'NONE',  ( 75.35748313534503495, 53.53391244244795644, -16.04435529155647089 ) ) ;
#31447=CARTESIAN_POINT ( 'NONE',  ( 74.69440617789626913, 59.37262990323052492, -15.74149122071481699 ) ) ;
#31448=CARTESIAN_POINT ( 'NONE',  ( 88.22748190676185231, 44.35111709898976784, 2.597852402453839638 ) ) ;
#31451=CARTESIAN_POINT ( 'NONE',  ( 72.56229913925623976, 71.29878675843531255, -6.010006885656266284 ) ) ;
#31453=CARTESIAN_POINT ( 'NONE',  ( 87.63170318219837895, 44.36446170533411504, -4.079950490519347106 ) ) ;
#31457=CARTESIAN_POINT ( 'NONE',  ( 67.11110063547383220, 69.33978020239571549, 3.973669838717296177 ) ) ;
#31458=CARTESIAN_POINT ( 'NONE',  ( 84.26179751283029873, 42.61849302290659836, -4.369886972103340206 ) ) ;
#31461=CARTESIAN_POINT ( 'NONE',  ( 72.41389820116259557, 70.72247311216293042, 7.745007521649655224 ) ) ;
#31462=CARTESIAN_POINT ( 'NONE',  ( 72.85370133302119200, 56.82307610116442476, -15.94993432694561619 ) ) ;
#31463=CARTESIAN_POINT ( 'NONE',  ( 76.62859868508415673, 63.47930858090246176, 15.36151106740648409 ) ) ;
#31468=DIRECTION ( 'NONE',  ( 0.5000000000000014433, -0.8660254037844378194, 0.000000000000000000 ) ) ;
#31471=CARTESIAN_POINT ( 'NONE',  ( 25.29680607046014984, 36.64646525600391413, -2.839279412974133887 ) ) ;
#31473=CARTESIAN_POINT ( 'NONE',  ( 78.23551423149454820, 47.47004208817780579, -13.80088926432411078 ) ) ;
#31475=FACE_OUTER_BOUND ( 'NONE', #87869, .T. ) ;
#31478=CARTESIAN_POINT ( 'NONE',  ( 83.80070905581447960, 52.11257540518899134, 14.61422408426159514 ) ) ;
#31481=CARTESIAN_POINT ( 'NONE',  ( 72.24154989827734141, 59.25143648895021897, -15.38920633486964462 ) ) ;
#31491=CARTESIAN_POINT ( 'NONE',  ( 71.27261462778223233, 70.10394064289017990, 6.818682661097508202 ) ) ;
#31493=CARTESIAN_POINT ( 'NONE',  ( 67.47735244041156477, 66.63445412725755546, 8.643438539336665727 ) ) ;
#31494=CARTESIAN_POINT ( 'NONE',  ( 71.45656473000614994, 65.30002271808615433, -12.31008476486731418 ) ) ;
#31495=CARTESIAN_POINT ( 'NONE',  ( 78.23831993261968876, 47.47892751676445755, 14.35468016619520881 ) ) ;
#31499=CARTESIAN_POINT ( 'NONE',  ( 83.81364139273995306, 41.70719278157028498, -0.8692552194661639087 ) ) ;
#31503=CARTESIAN_POINT ( 'NONE',  ( 83.82917762730355093, 51.97629592023758249, -14.94018958758825022 ) ) ;
#31506=DIRECTION ( 'NONE',  ( 0.6758705274779382988, 0.2489746672676192429, 0.6936934806855775681 ) ) ;
#31507=CARTESIAN_POINT ( 'NONE',  ( 72.29720748969889144, 71.75793896413090067, 5.568862843245728556 ) ) ;
#31514=B_SPLINE_CURVE_WITH_KNOTS ( 'NONE', 3,
 ( #25823, #93749, #57186, #55674, #64304, #16701, #95255, #18713, #94241, #86661, #56699, #72933, #71919, #64811, #17193, #87680, #33403, #9627, #62792, #18215, #40973, #80550, #41487, #40488, #72433, #49107, #87177, #17713, #71418, #80044, #70915, #47593, #9106, #63801, #10611, #33926, #48614, #95759, #32894, #26311, #41997, #32402, #88165, #49595, #63299, #94735 ),
 .UNSPECIFIED., .F., .F.,
 ( 4, 1, 2, 2, 1, 2, 2, 1, 1, 2, 2, 1, 1, 2, 2, 1, 1, 2, 2, 1, 1, 1, 2, 2, 1, 1, 1, 2, 2, 4 ),
 ( 0.000000000000000000, 0.06249999999998799571, 0.09374999999998243072, 0.1249999999999768796, 0.1874999999999684974, 0.2187499999999658606, 0.2499999999999632516, 0.3124999999999567013, 0.3437499999999547029, 0.3593749999999529821, 0.3749999999999512057, 0.4374999999999458766, 0.4687499999999430456, 0.4843749999999430456, 0.4999999999999430456, 0.5624999999999473754, 0.5937499999999509281, 0.6093749999999535927, 0.6249999999999562572, 0.6874999999999649170, 0.7187499999999702460, 0.7343749999999733546, 0.7421874999999749090, 0.7499999999999764633, 0.8124999999999785727, 0.8437499999999796829, 0.8593749999999792388, 0.8671874999999796829, 0.8749999999999800160, 1.000000000000000000 ),
 .UNSPECIFIED. ) ;
#31516=CARTESIAN_POINT ( 'NONE',  ( 69.37251848561912482, 66.28420332388499503, -10.39712879372465437 ) ) ;
#31519=CARTESIAN_POINT ( 'NONE',  ( 87.70233365940427461, 44.37954158847006170, -4.000613605175061593 ) ) ;
#31523=CARTESIAN_POINT ( 'NONE',  ( 82.13606007655464225, 41.45974715720112869, -5.928773293604740147 ) ) ;
#31528=( BOUNDED_CURVE ( )  B_SPLINE_CURVE ( 2, ( #48292, #87374, #93425, #2204, #70070, #9810, #685, #48800, #32586, #79238, #92913, #71607, #23977 ),
 .UNSPECIFIED., .F., .T. ) 
 B_SPLINE_CURVE_WITH_KNOTS ( ( 3, 2, 2, 2, 2, 2, 3 ),
 ( 0.5875000000000000222, 0.5899999999999999689, 0.5949999999999999734, 0.5999999999999999778, 0.6049999999999999822, 0.6099999999999999867, 0.6125000000000000444 ),
 .UNSPECIFIED. ) 
 CURVE ( )  GEOMETRIC_REPRESENTATION_ITEM ( )  RATIONAL_B_SPLINE_CURVE ( ( 0.9755282581475767101, 0.9755282581475772652, 1.000000000000000000, 0.9510565162951535312, 1.000000000000000000, 0.9510565162951535312, 1.000000000000000000, 0.9510565162951535312, 1.000000000000000000, 0.9510565162951535312, 1.000000000000000000, 0.9755282581475761550, 0.9755282581475767101 ) ) 
 REPRESENTATION_ITEM ( '' )  );
#31532=CARTESIAN_POINT ( 'NONE',  ( 43.80372508975956691, 30.45404122711137163, -8.090169943749478065 ) ) ;
#31538=CARTESIAN_POINT ( 'NONE',  ( 15.30702494462977370, 17.03677371833801146, 10.00000000000000533 ) ) ;
#31539=CARTESIAN_POINT ( 'NONE',  ( 72.52865609843787809, 57.51546068812135815, 16.29679984377914437 ) ) ;
#31545=CARTESIAN_POINT ( 'NONE',  ( 73.15257707569458034, 57.27860612637811499, 16.38974116562414451 ) ) ;
#31546=LINE ( 'NONE', #60443, #29448 ) ;
#31547=CARTESIAN_POINT ( 'NONE',  ( 19.02883662497902861, 11.39040679176981996, 1.333680081654574804E-15 ) ) ;
#31548=ORIENTED_EDGE ( 'NONE', *, *, #34475, .T. ) ;
#31552=CARTESIAN_POINT ( 'NONE',  ( 25.38519627463738715, 32.84336893147757053, -7.433330006724137462 ) ) ;
#31557=CARTESIAN_POINT ( 'NONE',  ( 65.82094082657513923, 68.94627234734062426, 2.288258256726706907 ) ) ;
#31562=CARTESIAN_POINT ( 'NONE',  ( 14.98925625915878435, 9.449665230724930254, -2.296566073217252530E-15 ) ) ;
#31564=CARTESIAN_POINT ( 'NONE',  ( 71.90400658755810070, 72.53437165389429708, 1.750395423964772990 ) ) ;
#31575=CARTESIAN_POINT ( 'NONE',  ( 73.06786641563543583, 70.68483820275014295, 7.671292531139269677 ) ) ;
#31579=VERTEX_POINT ( 'NONE', #37126 ) ;
#31581=DIRECTION ( 'NONE',  ( -0.4924038765061016787, 0.8528685319524424990, -0.1736481776669404342 ) ) ;
#31584=CARTESIAN_POINT ( 'NONE',  ( 21.35627990119762032, 12.73415679381821519, 1.333680081654574804E-15 ) ) ;
#31588=CARTESIAN_POINT ( 'NONE',  ( 33.26462506102002692, 34.90829794293883026, 10.00000000000000355 ) ) ;
#31590=EDGE_LOOP ( 'NONE', ( #5000, #63608, #30495, #74661 ) ) ;
#31592=CARTESIAN_POINT ( 'NONE',  ( 72.81511981781955001, 58.90692562186728765, 15.57534130551175799 ) ) ;
#31598=CARTESIAN_POINT ( 'NONE',  ( 81.98982836076474712, 58.71377021865833257, 0.05226423163382854647 ) ) ;
#31603=CARTESIAN_POINT ( 'NONE',  ( 82.37373412059557154, 53.49834611899161985, -15.77010555883211929 ) ) ;
#31604=CARTESIAN_POINT ( 'NONE',  ( 87.10115137904762150, 45.28340438443854055, 6.995308688534716879 ) ) ;
#31606=CARTESIAN_POINT ( 'NONE',  ( 75.08189823614961256, 56.99527856207666332, -16.54286807313852137 ) ) ;
#31607=CARTESIAN_POINT ( 'NONE',  ( 9.333682440526761326, 28.49540643055185640, 3.479690158560446702E-15 ) ) ;
#31615=CARTESIAN_POINT ( 'NONE',  ( 81.70878797397156745, 46.02746657646116546, -11.49744158306595310 ) ) ;
#31624=CARTESIAN_POINT ( 'NONE',  ( 82.16355652963139278, 40.77362396971211922, -0.6832070566406561740 ) ) ;
#31629=CARTESIAN_POINT ( 'NONE',  ( 75.60765592493140730, 65.32810859375902623, 14.31319638027754593 ) ) ;
#31633=DIRECTION ( 'NONE',  ( 0.8660254037844341557, 0.5000000000000082157, -0.000000000000000000 ) ) ;
#31636=CARTESIAN_POINT ( 'NONE',  ( 83.55900032775279840, 46.36886482531775044, -10.91248212791196615 ) ) ;
#31640=CARTESIAN_POINT ( 'NONE',  ( 74.43794370846053710, 68.05007506763284653, -11.63842094426022555 ) ) ;
#31643=VERTEX_POINT ( 'NONE', #75158 ) ;
#31648=CARTESIAN_POINT ( 'NONE',  ( 35.64779661956466583, 28.78052372038643369, -10.00000000000000355 ) ) ;
#31666=CARTESIAN_POINT ( 'NONE',  ( 8.474262601947446072, 26.93396525600388713, 2.839279412974139660 ) ) ;
#31668=CARTESIAN_POINT ( 'NONE',  ( 73.52895665835218608, 59.09902088736443915, -16.10230406680008741 ) ) ;
#31676=CARTESIAN_POINT ( 'NONE',  ( 86.46502256137985398, 47.49784904624871729, 10.45499499417849876 ) ) ;
#31680=CARTESIAN_POINT ( 'NONE',  ( 82.67070653882738895, 41.17429230206336399, 4.398717897525028064 ) ) ;
#31685=CARTESIAN_POINT ( 'NONE',  ( 73.17900167297862879, 69.84980244707995212, 9.598651498403647508 ) ) ;
#31686=CARTESIAN_POINT ( 'NONE',  ( 33.80247542503471436, 34.91421378149921395, 9.188101187500008038 ) ) ;
#31692=CARTESIAN_POINT ( 'NONE',  ( 79.58917286194427732, 59.33460254692537461, 16.56081879078485741 ) ) ;
#31695=CARTESIAN_POINT ( 'NONE',  ( 19.73933908736162124, 30.13478043621388380, 8.090169943749478065 ) ) ;
#31698=CARTESIAN_POINT ( 'NONE',  ( 85.07340834217973224, 44.94014711221131364, -9.007945491601892840 ) ) ;
#31701=EDGE_CURVE ( 'NONE', #73884, #41027, #92859, .T. ) ;
#31706=CARTESIAN_POINT ( 'NONE',  ( 77.16425012238860859, 49.51985965088922370, -15.46725698127323945 ) ) ;
#31707=ORIENTED_EDGE ( 'NONE', *, *, #39513, .T. ) ;
#31708=CARTESIAN_POINT ( 'NONE',  ( 86.89657730260137214, 45.77512320498411214, -8.683907937581334835 ) ) ;
#31715=CARTESIAN_POINT ( 'NONE',  ( 79.49951204047911801, 46.37032438487753438, 12.70281872619212926 ) ) ;
#31717=ADVANCED_FACE ( 'NONE', ( #60410 ), #45225, .T. ) ;
#31721=CARTESIAN_POINT ( 'NONE',  ( 70.80322137413750738, 60.50400129575321984, -14.70302039727341636 ) ) ;
#31722=CARTESIAN_POINT ( 'NONE',  ( 33.58239374649102871, 42.49540643055189548, 3.479690158560446702E-15 ) ) ;
#31724=DIRECTION ( 'NONE',  ( 0.2633726137851616911, 0.9634420117996742583, 0.04913609882121805494 ) ) ;
#31731=CARTESIAN_POINT ( 'NONE',  ( 71.41016749218992743, 59.45273978182970609, 15.19346469599747174 ) ) ;
#31734=EDGE_CURVE ( 'NONE', #2508, #96690, #25632, .T. ) ;
#31736=CARTESIAN_POINT ( 'NONE',  ( 26.07871176553302917, 38.55466486950701466, 7.012934429366973338E-14 ) ) ;
#31737=CARTESIAN_POINT ( 'NONE',  ( 77.97212537282862854, 53.69847124008602890, -16.36973322202745607 ) ) ;
#31753=EDGE_CURVE ( 'NONE', #28265, #86867, #40110, .T. ) ;
#31762=CARTESIAN_POINT ( 'NONE',  ( 73.76584831522595209, 68.38082682530665579, 10.99424229391075514 ) ) ;
#31763=CARTESIAN_POINT ( 'NONE',  ( 69.65059073173789272, 70.85594054465668989, -0.7120434053404213204 ) ) ;
#31784=CARTESIAN_POINT ( 'NONE',  ( 72.87540168778714644, 56.79582781200069519, -15.95562737981789603 ) ) ;
#31787=PLANE ( 'NONE',  #67679 ) ;
#31788=CARTESIAN_POINT ( 'NONE',  ( 88.17148522932362198, 43.68169873549415883, 0.1729226289268753214 ) ) ;
#31789=CARTESIAN_POINT ( 'NONE',  ( 84.86738834342773430, 49.16326195102271868, -12.63241503557467205 ) ) ;
#31792=CARTESIAN_POINT ( 'NONE',  ( 68.97600843347925093, 70.62407868326711480, -3.116157198528183514 ) ) ;
#31794=CARTESIAN_POINT ( 'NONE',  ( 34.04181514241641793, 20.44966523072496400, -2.296566073217252530E-15 ) ) ;
#31795=DIRECTION ( 'NONE',  ( -0.8660254037844379305, -0.5000000000000014433, -0.000000000000000000 ) ) ;
#31796=CARTESIAN_POINT ( 'NONE',  ( 83.56384804551235845, 46.97371956187362940, -11.44051147514629818 ) ) ;
#31797=CARTESIAN_POINT ( 'NONE',  ( 15.62556418158687244, 11.94754757982088123, 5.678558825948272215 ) ) ;
#31803=CARTESIAN_POINT ( 'NONE',  ( 69.43616476765555490, 62.98053158445969757, -13.63934076488703795 ) ) ;
#31811=CARTESIAN_POINT ( 'NONE',  ( 77.29015577573032658, 49.49666603636313766, 14.91995587329190798 ) ) ;
#31816=CARTESIAN_POINT ( 'NONE',  ( 68.58230928772361779, 68.76319458306602428, -6.210401753971947159 ) ) ;
#31826=CARTESIAN_POINT ( 'NONE',  ( 32.96772289237024012, 21.96004757982091959, -5.678558825948275768 ) ) ;
#31828=CARTESIAN_POINT ( 'NONE',  ( 74.97941504220045772, 66.36908880787137832, -13.10375872137871767 ) ) ;
#31835=CARTESIAN_POINT ( 'NONE',  ( 68.00841086724713591, 65.44229140645596488, 10.41124389034581199 ) ) ;
#31836=CARTESIAN_POINT ( 'NONE',  ( 68.03198790762533577, 66.08726303867234719, -10.49906168697004816 ) ) ;
#31839=CARTESIAN_POINT ( 'NONE',  ( 32.56963740530460427, 41.73705186507756082, -3.090169943749475845 ) ) ;
#31855=CARTESIAN_POINT ( 'NONE',  ( 80.16587651742513287, 44.65728575280898127, -11.72747585068735887 ) ) ;
#31859=B_SPLINE_SURFACE_WITH_KNOTS ( 'NONE', 3, 1, ( 
 ( #74922, #28801 ),
 ( #61182, #74432 ),
 ( #59682, #90654 ),
 ( #53090, #21212 ),
 ( #91137, #44984 ),
 ( #77490, #85109 ),
 ( #14679, #22272 ),
 ( #8084, #99294 ),
 ( #14185, #23758 ),
 ( #76009, #68861 ),
 ( #84614, #61759 ),
 ( #91710, #92708 ),
 ( #54145, #38457 ),
 ( #45560, #29386 ),
 ( #23258, #69863 ),
 ( #60253, #29875 ),
 ( #100290, #53656 ),
 ( #93202, #46051 ),
 ( #53176, #99786 ),
 ( #38958, #60747 ),
 ( #15659, #22779 ),
 ( #85627, #52663 ),
 ( #91211, #30376 ),
 ( #46555, #15153 ),
 ( #84130, #61259 ),
 ( #76489, #6587 ),
 ( #76966, #68370 ),
 ( #92229, #7068 ),
 ( #21773, #37952 ),
 ( #83617, #7567 ),
 ( #69371, #475 ) ),
 .UNSPECIFIED., .F., .F., .F.,
 ( 4, 3, 3, 3, 3, 3, 3, 3, 3, 3, 4 ),
 ( 2, 2 ),
 ( 0.000000000000000000, 0.1122669598086762505, 0.2243161639709597699, 0.3396355846219117347, 0.4553962076585177376, 0.5677860799922461732, 0.6749047109689493285, 0.7773884377078335017, 0.8775581155834230040, 0.9782364162377888972, 1.000000000000000000 ),
 ( 0.000000000000000000, 1.000000000000000000 ),
 .UNSPECIFIED. ) ;
#31861=CARTESIAN_POINT ( 'NONE',  ( 84.55469670542369443, 47.34764971695675229, -11.32901942273590379 ) ) ;
#31874=CARTESIAN_POINT ( 'NONE',  ( 87.64772643527687990, 44.68358544867225390, 5.012156274856216953 ) ) ;
#31880=CARTESIAN_POINT ( 'NONE',  ( 71.88281838930642209, 59.56282477439597045, -15.74156321294393024 ) ) ;
#31887=CARTESIAN_POINT ( 'NONE',  ( 82.08475017950465258, 40.77228884684495824, 1.269038889852737384 ) ) ;
#31889=CARTESIAN_POINT ( 'NONE',  ( 83.75118553669710764, 52.20252726632157447, 14.66647926495056886 ) ) ;
#31891=B_SPLINE_CURVE_WITH_KNOTS ( 'NONE', 3,
 ( #97076, #12445, #81379, #26139, #3838, #19057, #49931, #72767, #64643, #11946 ),
 .UNSPECIFIED., .F., .F.,
 ( 4, 2, 2, 2, 4 ),
 ( 0.000000000000000000, 0.2500000000000000000, 0.5000000000000000000, 0.7500000000000000000, 1.000000000000000000 ),
 .UNSPECIFIED. ) ;
#31901=CARTESIAN_POINT ( 'NONE',  ( 26.41003172443570790, 38.18080186712595037, 3.090169943749475401 ) ) ;
#31907=DIRECTION ( 'NONE',  ( 0.06958655048003267729, -0.1205274409548735270, -0.9902680687415703620 ) ) ;
#31910=CARTESIAN_POINT ( 'NONE',  ( 26.23682664367882111, 38.08080186712594184, -3.090169943749475845 ) ) ;
#31916=CARTESIAN_POINT ( 'NONE',  ( 28.13532114344886992, 38.01751292744058475, 6.180339887498949913 ) ) ;
#31917=CARTESIAN_POINT ( 'NONE',  ( 85.18851589652911116, 42.50252688496647835, -1.291714491316064306 ) ) ;
#31920=CARTESIAN_POINT ( 'NONE',  ( 81.50416045441870949, 56.04869296950724333, 16.05856639404321129 ) ) ;
#31925=CARTESIAN_POINT ( 'NONE',  ( 68.42498683509937507, 66.83623499972065929, -9.111695128013669986 ) ) ;
#31928=CARTESIAN_POINT ( 'NONE',  ( 71.39067424117821759, 70.28756797341888785, -7.485097133833798821 ) ) ;
#31931=CARTESIAN_POINT ( 'NONE',  ( 77.46075950540223687, 49.77948894799936852, -14.98483444581543722 ) ) ;
#31937=CARTESIAN_POINT ( 'NONE',  ( 18.21401815691482895, 25.91421378149918198, 9.188101187500008038 ) ) ;
#31943=CARTESIAN_POINT ( 'NONE',  ( 35.31250668086031652, 42.16126292948898424, -6.180339887498951690 ) ) ;
#31944=CARTESIAN_POINT ( 'NONE',  ( 10.26703877906431472, 17.87878583063839599, -9.188101187500006262 ) ) ;
#31945=CARTESIAN_POINT ( 'NONE',  ( 75.25614561676577807, 53.63511853603917956, -16.53665762988984511 ) ) ;
#31947=CARTESIAN_POINT ( 'NONE',  ( 71.91251904240313308, 72.63095699448832931, -0.6620033135626105514 ) ) ;
#31948=CARTESIAN_POINT ( 'NONE',  ( 36.20694410119924811, 43.83705186507757645, 3.090169943749475401 ) ) ;
#31949=ORIENTED_EDGE ( 'NONE', *, *, #83937, .F. ) ;
#31950=DIRECTION ( 'NONE',  ( -0.6355427771210634402, 0.000000000000000000, 0.7720656568254065100 ) ) ;
#31951=CARTESIAN_POINT ( 'NONE',  ( 72.52074056358647169, 71.25752213848458894, -6.049989122658143259 ) ) ;
#31956=CARTESIAN_POINT ( 'NONE',  ( 79.14312167556931854, 57.64441083166269664, 0.000000000000000000 ) ) ;
#31957=CARTESIAN_POINT ( 'NONE',  ( 86.45348570349138129, 43.24264366923927838, -1.738868482183878239 ) ) ;
#31959=CARTESIAN_POINT ( 'NONE',  ( 65.86357856937301847, 68.93032387894690771, -2.527662978207743549 ) ) ;
#31960=CARTESIAN_POINT ( 'NONE',  ( 71.76465953926796715, 72.09915442159702081, -3.621776363507912766 ) ) ;
#31961=CARTESIAN_POINT ( 'NONE',  ( 79.93705350559073963, 58.08899977657839031, 16.26815128937695576 ) ) ;
#31962=CARTESIAN_POINT ( 'NONE',  ( 76.92045831404706746, 63.69682018499118925, 15.34400990693822564 ) ) ;
#31971=CARTESIAN_POINT ( 'NONE',  ( 24.92213970864663963, 37.49540643055189548, 3.479690158560446702E-15 ) ) ;
#31973=CARTESIAN_POINT ( 'NONE',  ( 78.28749215422203633, 47.38001368514189693, -14.28996306490787482 ) ) ;
#31977=CARTESIAN_POINT ( 'NONE',  ( 74.40608543823466903, 68.34271654374390437, 11.85151599582642312 ) ) ;
#31981=EDGE_CURVE ( 'NONE', #35343, #69104, #7105, .T. ) ;
#31993=CARTESIAN_POINT ( 'NONE',  ( 76.18925827497564285, 65.27842891210502785, 14.09988157931024766 ) ) ;
#31994=CARTESIAN_POINT ( 'NONE',  ( 76.32413911534708006, 63.96060367144042402, -14.71169841249486332 ) ) ;
#31999=CARTESIAN_POINT ( 'NONE',  ( 84.55537670905214043, 50.62155581810768012, -14.09136642048690291 ) ) ;
#32000=CARTESIAN_POINT ( 'NONE',  ( 70.61866190243357266, 66.21379322135312862, 11.18361157626617874 ) ) ;
#32003=CARTESIAN_POINT ( 'NONE',  ( 83.83319469606612984, 52.06770183867002544, -14.58843048856406099 ) ) ;
#32006=CARTESIAN_POINT ( 'NONE',  ( 80.15404930735283529, 58.24487849859603017, -16.60713908503102232 ) ) ;
#32008=CARTESIAN_POINT ( 'NONE',  ( 85.83574890286925552, 44.62951015086210305, -6.991694815152513343 ) ) ;
#32018=CARTESIAN_POINT ( 'NONE',  ( 85.55975315002648074, 48.35019831671618817, -12.20940535940758842 ) ) ;
#32024=LINE ( 'NONE', #93885, #61175 ) ;
#32025=CARTESIAN_POINT ( 'NONE',  ( 67.79725476218452229, 65.71048819351143777, 10.00598338191753101 ) ) ;
#32032=CARTESIAN_POINT ( 'NONE',  ( 88.05223289789027774, 44.73115413622458902, 4.436861541472143067 ) ) ;
#32034=CARTESIAN_POINT ( 'NONE',  ( 8.320926099340340443, 27.73705186507752174, -3.090169943749475845 ) ) ;
#32036=CARTESIAN_POINT ( 'NONE',  ( 71.87556436007473337, 59.56477266904413881, -15.73977692506605486 ) ) ;
#32037=CARTESIAN_POINT ( 'NONE',  ( 66.76060919205468736, 68.13847131232218146, -6.506754398145753626 ) ) ;
#32040=CARTESIAN_POINT ( 'NONE',  ( 12.53791098520745173, 8.208019796199266693, -3.090169943749474069 ) ) ;
#32043=CARTESIAN_POINT ( 'NONE',  ( 16.70795526530605457, 14.81029122506293483, 8.090169943749479842 ) ) ;
#32051=CARTESIAN_POINT ( 'NONE',  ( 27.52682148520507965, 37.93396525600392266, 2.839279412974139660 ) ) ;
#32058=AXIS2_PLACEMENT_3D ( 'NONE', #49269, #18373, #88323 ) ;
#32059=CARTESIAN_POINT ( 'NONE',  ( 66.03987969823486992, 68.56027586650085937, 2.028142095923215482 ) ) ;
#32061=CARTESIAN_POINT ( 'NONE',  ( 82.87596643829704135, 41.15858874971023340, 0.1873015203630768732 ) ) ;
#32065=CARTESIAN_POINT ( 'NONE',  ( 14.44138481658839090, 10.19860640527290663, 2.839279412974134775 ) ) ;
#32075=VERTEX_POINT ( 'NONE', #24800 ) ;
#32080=ORIENTED_EDGE ( 'NONE', *, *, #60011, .F. ) ;
#32085=CARTESIAN_POINT ( 'NONE',  ( 79.08643767721619611, 59.41746268492353522, -16.53334974603829366 ) ) ;
#32088=CARTESIAN_POINT ( 'NONE',  ( 80.85195420596313909, 43.03173977397389649, 9.658905536921107426 ) ) ;
#32098=CARTESIAN_POINT ( 'NONE',  ( 73.54926982385974554, 62.06432499625495325, 14.76512139019120973 ) ) ;
#32105=CARTESIAN_POINT ( 'NONE',  ( 81.87257924523440522, 45.31425140043580768, 10.75858732970988108 ) ) ;
#32108=EDGE_CURVE ( 'NONE', #184, #44213, #66739, .T. ) ;
#32110=CARTESIAN_POINT ( 'NONE',  ( 82.70749068191635445, 53.29046182800484388, -15.29114564428902234 ) ) ;
#32113=CARTESIAN_POINT ( 'NONE',  ( 14.52983486323338802, 31.49540643055186706, 3.479690158560446702E-15 ) ) ;
#32124=CARTESIAN_POINT ( 'NONE',  ( 85.51176157151247992, 45.57569484508597668, -8.758718004448168060 ) ) ;
#32127=ORIENTED_EDGE ( 'NONE', *, *, #53625, .F. ) ;
#32129=( BOUNDED_CURVE ( )  B_SPLINE_CURVE ( 2, ( #15221, #7638, #92288, #53721, #46631, #77557, #44625, #67950, #36537, #84681, #46116, #77032, #53 ),
 .UNSPECIFIED., .F., .T. ) 
 B_SPLINE_CURVE_WITH_KNOTS ( ( 3, 2, 2, 2, 2, 2, 3 ),
 ( 0.9125000000000000888, 0.9150000000000000355, 0.9200000000000000400, 0.9250000000000000444, 0.9300000000000000488, 0.9350000000000000533, 0.9375000000000000000 ),
 .UNSPECIFIED. ) 
 CURVE ( )  GEOMETRIC_REPRESENTATION_ITEM ( )  RATIONAL_B_SPLINE_CURVE ( ( 0.9755282581475767101, 0.9755282581475772652, 1.000000000000000000, 0.9510565162951535312, 1.000000000000000000, 0.9510565162951535312, 1.000000000000000000, 0.9510565162951535312, 1.000000000000000000, 0.9510565162951535312, 1.000000000000000000, 0.9755282581475768211, 0.9755282581475768211 ) ) 
 REPRESENTATION_ITEM ( '' )  );
#32132=CARTESIAN_POINT ( 'NONE',  ( 66.47763888060634940, 67.99612994687967671, 6.463816603905427449 ) ) ;
#32135=CARTESIAN_POINT ( 'NONE',  ( 82.37597161381533795, 40.39206419195442521, -1.284498707061657585 ) ) ;
#32141=CARTESIAN_POINT ( 'NONE',  ( 75.64798029740516938, 65.57340602677163588, 13.80036590763650750 ) ) ;
#32150=CARTESIAN_POINT ( 'NONE',  ( 28.04762285228751395, 28.14441083166262203, 10.00000000000000533 ) ) ;
#32154=CARTESIAN_POINT ( 'NONE',  ( 74.21225604557145061, 68.54784490154126786, -11.57567064299385784 ) ) ;
#32163=DIRECTION ( 'NONE',  ( 0.8503781557569302096, -0.05328141121993811014, 0.5234673661555743207 ) ) ;
#32164=CARTESIAN_POINT ( 'NONE',  ( 80.58798105445690396, 57.19556934344895183, -16.22990577884235108 ) ) ;
#32165=CARTESIAN_POINT ( 'NONE',  ( 68.87153398673127924, 63.79608234936608113, -12.28269806760821936 ) ) ;
#32177=B_SPLINE_CURVE_WITH_KNOTS ( 'NONE', 3,
 ( #91897, #44243, #14845, #59939, #36645, #46223, #45731, #38123, #76653, #69040, #67551, #30555, #7750, #69547, #31041, #25444 ),
 .UNSPECIFIED., .F., .F.,
 ( 4, 1, 2, 2, 2, 1, 2, 2, 4 ),
 ( 0.000000000000000000, 0.1249999999999992506, 0.1875000000000008604, 0.2500000000000024980, 0.5000000000000014433, 0.6250000000000024425, 0.6875000000000014433, 0.7500000000000003331, 1.000000000000000000 ),
 .UNSPECIFIED. ) ;
#32180=CARTESIAN_POINT ( 'NONE',  ( 12.13982549814181411, 27.98502408145591502, -5.678558825948271327 ) ) ;
#32182=CARTESIAN_POINT ( 'NONE',  ( 73.93788252295223629, 58.97677190194296770, -16.17750573964183403 ) ) ;
#32190=CARTESIAN_POINT ( 'NONE',  ( 76.26946404230704957, 64.97317754398874001, 14.67006731301515998 ) ) ;
#32193=CARTESIAN_POINT ( 'NONE',  ( 71.98264401366868981, 72.39816763649429276, -2.869464145551841039 ) ) ;
#32196=CARTESIAN_POINT ( 'NONE',  ( 72.09021951009610518, 72.27625441170016529, 1.322546034541348225 ) ) ;
#32198=B_SPLINE_CURVE_WITH_KNOTS ( 'NONE', 3,
 ( #55292, #53791, #84753, #61896, #40093, #24909, #71036, #54288, #31499, #92357, #93861, #86273, #62391, #55784, #7712, #54806, #15292, #93348, #86776, #46191, #85783, #9742 ),
 .UNSPECIFIED., .F., .F.,
 ( 4, 1, 1, 2, 2, 1, 1, 2, 2, 1, 1, 2, 2, 4 ),
 ( 0.5972366333919344461, 0.6475820542179384631, 0.6727547646309413043, 0.6853411198374419477, 0.6979274750439424801, 0.7482728958699466082, 0.7734456062829488943, 0.7860319614894499818, 0.7986183166959511803, 0.8489637375219629689, 0.8741364479349700289, 0.8867228031414734479, 0.8993091583479768669, 1.000000000000000000 ),
 .UNSPECIFIED. ) ;
#32199=CARTESIAN_POINT ( 'NONE',  ( 83.90043522580160129, 51.91099903043517827, -14.50837359699251294 ) ) ;
#32204=CARTESIAN_POINT ( 'NONE',  ( 30.66616357392367220, 39.74646525600392977, 2.839279412974139660 ) ) ;
#32205=CARTESIAN_POINT ( 'NONE',  ( 83.56516159190486803, 41.02999554113897318, 0.5818837730058337154 ) ) ;
#32212=CARTESIAN_POINT ( 'NONE',  ( 86.43064670831508067, 47.06455762112943120, -10.03233545160486706 ) ) ;
#32218=VECTOR ( 'NONE', #73289, 1000.000000000000000 ) ;
#32219=LINE ( 'NONE', #1836, #48569 ) ;
#32221=ORIENTED_EDGE ( 'NONE', *, *, #35498, .T. ) ;
#32225=CARTESIAN_POINT ( 'NONE',  ( 77.13583932239204444, 49.51254683941623824, -14.95790760833234678 ) ) ;
#32229=CARTESIAN_POINT ( 'NONE',  ( 79.44876042842709296, 54.60773761053498987, 15.97065083431682275 ) ) ;
#32235=CARTESIAN_POINT ( 'NONE',  ( 82.70122523897394728, 40.55072272859479909, 0.9023291622205993345 ) ) ;
#32245=CARTESIAN_POINT ( 'NONE',  ( 22.60804823384966156, 31.79103043416549923, 8.090169943749478065 ) ) ;
#32246=ORIENTED_EDGE ( 'NONE', *, *, #93627, .F. ) ;
#32251=CARTESIAN_POINT ( 'NONE',  ( 73.66446749447686670, 67.99659565248040849, 11.28331122821951560 ) ) ;
#32260=CYLINDRICAL_SURFACE ( 'NONE', #33826, 15.60714546451156970 ) ;
#32270=CARTESIAN_POINT ( 'NONE',  ( 73.78372473906969731, 65.88421683824888930, 13.39692504310327692 ) ) ;
#32275=CARTESIAN_POINT ( 'NONE',  ( 74.20995892610953604, 68.60058487300136676, 11.52733404855581867 ) ) ;
#32276=CARTESIAN_POINT ( 'NONE',  ( 73.90039612685991699, 68.57416616861503655, 10.88887154151077397 ) ) ;
#32277=CARTESIAN_POINT ( 'NONE',  ( 70.70154975520648577, 71.34200407928535981, -2.184243020790304524 ) ) ;
#32285=CARTESIAN_POINT ( 'NONE',  ( 78.19980343102787401, 47.50132803318881258, 14.37731510607409646 ) ) ;
#32288=CARTESIAN_POINT ( 'NONE',  ( 78.02231740044358332, 54.72928692317312027, 16.06689032128053896 ) ) ;
#32290=CARTESIAN_POINT ( 'NONE',  ( 77.77623215880998941, 62.01577911499505547, 15.64215120907620005 ) ) ;
#32292=CARTESIAN_POINT ( 'NONE',  ( 76.24073292652140310, 51.11943835579473472, 16.06739483476730967 ) ) ;
#32301=EDGE_CURVE ( 'NONE', #16291, #5537, #53580, .T. ) ;
#32304=FACE_OUTER_BOUND ( 'NONE', #57665, .T. ) ;
#32305=CARTESIAN_POINT ( 'NONE',  ( 84.36110011788976237, 49.31626265921352115, -12.91867116132553761 ) ) ;
#32306=CARTESIAN_POINT ( 'NONE',  ( 86.69305172099772960, 43.39454550306078318, -4.013483749032378256 ) ) ;
#32307=CARTESIAN_POINT ( 'NONE',  ( 72.69493809724967548, 71.16443809380129437, -7.267007365939472052 ) ) ;
#32310=CARTESIAN_POINT ( 'NONE',  ( 31.93509797303403630, 20.29860640527293825, -2.839279412974138328 ) ) ;
#32311=CARTESIAN_POINT ( 'NONE',  ( 72.44129552685039641, 70.67501955208014408, -7.848061272651224662 ) ) ;
#32312=CARTESIAN_POINT ( 'NONE',  ( 81.98039554206116009, 47.27905221821983162, -12.37811565305940142 ) ) ;
#32313=CARTESIAN_POINT ( 'NONE',  ( 9.022134044517839513, 26.18502408145589655, 5.678558825948277544 ) ) ;
#32321=CARTESIAN_POINT ( 'NONE',  ( 80.19044581452921250, 55.04695057392905255, -15.97072302619556261 ) ) ;
#32322=CARTESIAN_POINT ( 'NONE',  ( 87.52040938742109688, 45.06780532364838621, -6.102424753035670335 ) ) ;
#32327=CARTESIAN_POINT ( 'NONE',  ( 77.07045653762983761, 49.53584601179438351, 14.97980822837095793 ) ) ;
#32337=B_SPLINE_CURVE_WITH_KNOTS ( 'NONE', 3,
 ( #75869, #6448, #99652, #92095, #30238, #43044, #53526, #37327, #81613, #73988, #68228, #4572, #67745, #98670, #99151, #75186, #82813, #51358, #20486, #40877, #58936, #12388, #71823, #32797 ),
 .UNSPECIFIED., .F., .F.,
 ( 4, 2, 2, 2, 2, 2, 2, 2, 2, 2, 2, 4 ),
 ( 0.000000000000000000, 0.1249999999999957534, 0.2499999999999915068, 0.3749999999999872324, 0.4374999999999828471, 0.4999999999999784617, 0.5624999999999741318, 0.6249999999999698019, 0.6874999999999654721, 0.7499999999999611422, 0.8749999999999805711, 1.000000000000000000 ),
 .UNSPECIFIED. ) ;
#32340=VERTEX_POINT ( 'NONE', #99209 ) ;
#32341=CARTESIAN_POINT ( 'NONE',  ( 25.52954022263673295, 23.24335787977764056, -9.188101187500008038 ) ) ;
#32342=CARTESIAN_POINT ( 'NONE',  ( 66.60594655232844730, 69.00361448147799592, -1.130437426683872149 ) ) ;
#32343=CARTESIAN_POINT ( 'NONE',  ( 74.82458239918585718, 66.79921256097772186, -13.19236156228707024 ) ) ;
#32344=CARTESIAN_POINT ( 'NONE',  ( 85.04986998970780121, 47.88075954187213767, -11.53627252243822099 ) ) ;
#32352=CARTESIAN_POINT ( 'NONE',  ( 68.04192742210889833, 65.44532392020195743, 10.42765866839662081 ) ) ;
#32353=CARTESIAN_POINT ( 'NONE',  ( 68.33289931102945047, 65.68983735164607651, -10.34968271987537669 ) ) ;
#32360=ADVANCED_FACE ( 'NONE', ( #43979 ), #31859, .T. ) ;
#32366=CARTESIAN_POINT ( 'NONE',  ( 78.17116731237634042, 61.83023861435394508, -16.09040300007290725 ) ) ;
#32368=CARTESIAN_POINT ( 'NONE',  ( 75.98104421109889017, 51.53574906954564483, 16.18761828508177203 ) ) ;
#32370=CARTESIAN_POINT ( 'NONE',  ( 80.08699412898864978, 44.58265640332982116, -11.70218130687201885 ) ) ;
#32371=ADVANCED_FACE ( 'NONE', ( #45070 ), #69866, .T. ) ;
#32372=DIRECTION ( 'NONE',  ( 0.000000000000000000, -0.3470917258701496921, 0.9378311862123591691 ) ) ;
#32374=CARTESIAN_POINT ( 'NONE',  ( 81.03183881876289263, 56.09329797361272085, 16.10623978537670098 ) ) ;
#32375=CARTESIAN_POINT ( 'NONE',  ( 85.27864792750219181, 47.17654793273538161, -10.80350663618311557 ) ) ;
#32380=ORIENTED_EDGE ( 'NONE', *, *, #18984, .F. ) ;
#32386=CARTESIAN_POINT ( 'NONE',  ( 76.23159145087653599, 64.83013986238610471, -14.34096891692713704 ) ) ;
#32392=CARTESIAN_POINT ( 'NONE',  ( 85.39547059847991761, 43.80125623371271359, -5.793701783558419471 ) ) ;
#32402=CARTESIAN_POINT ( 'NONE',  ( 82.91132241635402522, 41.41978976119851552, 2.605981997472240241 ) ) ;
#32404=CARTESIAN_POINT ( 'NONE',  ( 83.54394669835052412, 52.38488257041225182, 14.79586828322707071 ) ) ;
#32407=VERTEX_POINT ( 'NONE', #18181 ) ;
#32414=CARTESIAN_POINT ( 'NONE',  ( 73.67502235716121106, 55.34260408957710808, 16.11561656089581973 ) ) ;
#32417=CARTESIAN_POINT ( 'NONE',  ( 33.41142024434631708, 24.45404122711135386, -8.090169943749478065 ) ) ;
#32423=( BOUNDED_CURVE ( )  B_SPLINE_CURVE ( 2, ( #76877, #385, #62161, #7473, #29788, #91617, #22188, #47964, #19965, #87049, #97003, #9996, #8980 ),
 .UNSPECIFIED., .F., .T. ) 
 B_SPLINE_CURVE_WITH_KNOTS ( ( 3, 2, 2, 2, 2, 2, 3 ),
 ( 0.3375000000000000222, 0.3400000000000000244, 0.3449999999999999734, 0.3499999999999999778, 0.3549999999999999822, 0.3599999999999999867, 0.3624999999999999889 ),
 .UNSPECIFIED. ) 
 CURVE ( )  GEOMETRIC_REPRESENTATION_ITEM ( )  RATIONAL_B_SPLINE_CURVE ( ( 0.9755282581475768211, 0.9755282581475768211, 1.000000000000000000, 0.9510565162951535312, 1.000000000000000000, 0.9510565162951535312, 1.000000000000000000, 0.9510565162951535312, 1.000000000000000000, 0.9510565162951535312, 1.000000000000000000, 0.9755282581475768211, 0.9755282581475768211 ) ) 
 REPRESENTATION_ITEM ( '' )  );
#32425=CARTESIAN_POINT ( 'NONE',  ( 82.44703276532530367, 48.69185277918708721, 13.19452699896754133 ) ) ;
#32426=ORIENTED_EDGE ( 'NONE', *, *, #72641, .T. ) ;
#32428=FACE_OUTER_BOUND ( 'NONE', #65288, .T. ) ;
#32433=CARTESIAN_POINT ( 'NONE',  ( 26.95805898326085170, 39.65659080271453263, -1.878358725466461243E-16 ) ) ;
#32434=CARTESIAN_POINT ( 'NONE',  ( 84.45526090851787160, 42.21020478296429701, -2.202011278587945320 ) ) ;
#32436=CARTESIAN_POINT ( 'NONE',  ( 73.06766668685415311, 65.73470164174882768, 13.24181784610626522 ) ) ;
#32448=CARTESIAN_POINT ( 'NONE',  ( 67.53003662305086152, 66.80518130314699476, -8.448892015563799873 ) ) ;
#32457=CARTESIAN_POINT ( 'NONE',  ( 29.59504171901726366, 22.80170272979927759, 7.433330006724137462 ) ) ;
#32462=CARTESIAN_POINT ( 'NONE',  ( 34.89708068152319242, 43.08080186712595605, -3.090169943749475845 ) ) ;
#32463=CARTESIAN_POINT ( 'NONE',  ( 11.06209807803029221, 12.10170272979924988, -7.433330006724141015 ) ) ;
#32464=CARTESIAN_POINT ( 'NONE',  ( 80.07551378063752168, 57.23092041213119074, -16.24140625160306683 ) ) ;
#32465=CARTESIAN_POINT ( 'NONE',  ( 71.51903464973995028, 72.36264346112822921, -1.271393898589449512 ) ) ;
#32466=ADVANCED_FACE ( 'NONE', ( #4982 ), #6747, .T. ) ;
#32475=EDGE_CURVE ( 'NONE', #75378, #71488, #14568, .T. ) ;
#32478=ORIENTED_EDGE ( 'NONE', *, *, #73533, .F. ) ;
#32480=CARTESIAN_POINT ( 'NONE',  ( 71.65684213956077997, 72.06054752937143348, -3.528960205221522095 ) ) ;
#32482=CARTESIAN_POINT ( 'NONE',  ( 76.77756057274272905, 63.67496528870245243, 15.32214893988671101 ) ) ;
#32494=CARTESIAN_POINT ( 'NONE',  ( 30.11465696128792757, 23.10170272979928541, -7.433330006724141015 ) ) ;
#32496=CARTESIAN_POINT ( 'NONE',  ( 66.90449132437942126, 69.67812219415840502, -1.620417471643094798 ) ) ;
#32499=CARTESIAN_POINT ( 'NONE',  ( 74.10605571268695257, 68.62492193873490010, 10.95106078344675637 ) ) ;
#32505=CARTESIAN_POINT ( 'NONE',  ( 86.15569456219643030, 43.34566298074329893, -3.128694683549113176 ) ) ;
#32516=CARTESIAN_POINT ( 'NONE',  ( 67.48492722593299220, 67.03479993418675065, 8.993132823606122983 ) ) ;
#32517=CARTESIAN_POINT ( 'NONE',  ( 74.81986938884084282, 64.47242206951092669, -14.05694895914753673 ) ) ;
#32522=CARTESIAN_POINT ( 'NONE',  ( 69.87353541051622585, 64.19244626969324941, 12.43200581978026342 ) ) ;
#32525=CARTESIAN_POINT ( 'NONE',  ( 83.74768966023471251, 52.21580090503303495, -15.05827679895701898 ) ) ;
#32529=CARTESIAN_POINT ( 'NONE',  ( 80.61477260300527803, 57.23824740812084144, -16.23096960288277302 ) ) ;
#32540=CARTESIAN_POINT ( 'NONE',  ( 85.62748912975605720, 48.34643938460052937, -11.70855452506934391 ) ) ;
#32541=CARTESIAN_POINT ( 'NONE',  ( 87.95999259833929784, 44.52227941376569476, -3.981728561935235611 ) ) ;
#32548=CARTESIAN_POINT ( 'NONE',  ( 80.44948470589578449, 51.95659882761868431, -15.19047218006325650 ) ) ;
#32554=CARTESIAN_POINT ( 'NONE',  ( 8.494131180097229006, 27.83705186507752671, 3.090169943749475401 ) ) ;
#32555=CARTESIAN_POINT ( 'NONE',  ( 79.17566594283800896, 50.17566997415585206, -15.28976903731980741 ) ) ;
#32557=CARTESIAN_POINT ( 'NONE',  ( 72.21281551018738298, 72.08933296411181857, 3.049783143056646662 ) ) ;
#32565=EDGE_LOOP ( 'NONE', ( #21147, #71839, #26406, #4943 ) ) ;
#32569=B_SPLINE_CURVE_WITH_KNOTS ( 'NONE', 3,
 ( #9535, #40889, #94654, #2436, #25209, #56612, #40396, #69807, #70822, #77930, #86574, #55591, #48526, #46496, #77432, #70307, #417, #31306, #1431, #47507, #32312, #16117, #24708, #62194, #93145, #47015, #8521, #39390, #31796, #86087, #66702, #28202, #72344, #57600, #18122, #49024, #65213, #95675, #89090, #26222, #96155, #19639, #81948, #35808, #89563, #80463 ),
 .UNSPECIFIED., .F., .F.,
 ( 4, 1, 1, 1, 2, 2, 1, 1, 1, 2, 2, 1, 1, 2, 2, 1, 1, 2, 2, 1, 1, 2, 2, 1, 2, 2, 1, 2, 2, 4 ),
 ( 0.000000000000000000, 0.06249999999998910594, 0.09374999999998365197, 0.1093749999999809319, 0.1171874999999812095, 0.1249999999999814870, 0.1874999999999751310, 0.2187499999999721612, 0.2343749999999688860, 0.2421874999999692468, 0.2499999999999695799, 0.3124999999999819034, 0.3437499999999878986, 0.3593749999999907296, 0.3749999999999935052, 0.4374999999999977796, 0.4687499999999999445, 0.4843750000000010547, 0.5000000000000021094, 0.5625000000000041078, 0.5937500000000052180, 0.6093750000000056621, 0.6250000000000063283, 0.6875000000000054401, 0.7187500000000034417, 0.7500000000000013323, 0.8124999999999976685, 0.8437499999999973355, 0.8749999999999970024, 1.000000000000000000 ),
 .UNSPECIFIED. ) ;
#32572=CARTESIAN_POINT ( 'NONE',  ( 42.70206918026080700, 25.44966523072497822, -2.296566073217252530E-15 ) ) ;
#32576=CARTESIAN_POINT ( 'NONE',  ( 68.35453417343931903, 65.67399229982113695, 10.37910612949749911 ) ) ;
#32578=CARTESIAN_POINT ( 'NONE',  ( 66.11564498168849013, 69.06652558778995399, 2.579580841645931599 ) ) ;
#32583=CARTESIAN_POINT ( 'NONE',  ( 4.462289544239298245, 25.68290643055184930, 3.479690158560446702E-15 ) ) ;
#32586=CARTESIAN_POINT ( 'NONE',  ( 25.55253460671674759, 33.49103043416550918, -8.090169943749479842 ) ) ;
#32588=CARTESIAN_POINT ( 'NONE',  ( 66.30954113569532637, 68.28728378170325186, 3.992301261007319191 ) ) ;
#32595=CARTESIAN_POINT ( 'NONE',  ( 86.32568876638555366, 47.65221178568590688, 10.70297444941600418 ) ) ;
#32601=CARTESIAN_POINT ( 'NONE',  ( 85.35443477132466228, 48.30880629543902671, -11.80360700664790663 ) ) ;
#32608=LINE ( 'NONE', #70602, #76875 ) ;
#32614=ORIENTED_EDGE ( 'NONE', *, *, #63678, .F. ) ;
#32615=CARTESIAN_POINT ( 'NONE',  ( 73.11277796669548934, 60.16616684050868002, 15.29999328649868851 ) ) ;
#32619=CARTESIAN_POINT ( 'NONE',  ( 82.37905398250840960, 46.52165906567139331, 11.60550393209069320 ) ) ;
#32620=CARTESIAN_POINT ( 'NONE',  ( 69.74653821704758627, 65.80766725781488447, 11.05544688728975622 ) ) ;
#32622=CARTESIAN_POINT ( 'NONE',  ( 82.49110201129202835, 53.29505896912813512, -15.32863176240265268 ) ) ;
#32624=ORIENTED_EDGE ( 'NONE', *, *, #68098, .F. ) ;
#32626=CARTESIAN_POINT ( 'NONE',  ( 23.10466909204031083, 21.84335787977762777, 9.188101187500006262 ) ) ;
#32645=CARTESIAN_POINT ( 'NONE',  ( 82.41933087065974917, 40.38430946149325962, -0.8419157720437354664 ) ) ;
#32649=CARTESIAN_POINT ( 'NONE',  ( 75.78086150065365700, 65.61082703666508564, 13.82051080074114502 ) ) ;
#32651=ORIENTED_EDGE ( 'NONE', *, *, #56017, .F. ) ;
#32655=CARTESIAN_POINT ( 'NONE',  ( 88.02757723400505085, 43.99990312156534600, 0.5524629566968192185 ) ) ;
#32656=CARTESIAN_POINT ( 'NONE',  ( 32.56068451518306262, 20.92755873383627829, 6.180339887498953466 ) ) ;
#32659=CARTESIAN_POINT ( 'NONE',  ( 74.38673974678103207, 68.41474614631960094, -11.27947015944677212 ) ) ;
#32664=B_SPLINE_CURVE_WITH_KNOTS ( 'NONE', 3,
 ( #68807, #99735, #45993, #76911, #69318, #36411, #100240, #44001, #36963, #29378, #23253, #76959, #45062, #6580, #68362, #6069 ),
 .UNSPECIFIED., .F., .F.,
 ( 4, 1, 2, 2, 2, 1, 2, 2, 4 ),
 ( 0.000000000000000000, 0.1249999999999942268, 0.1874999999999933109, 0.2499999999999923950, 0.4999999999999982236, 0.6250000000000007772, 0.6875000000000017764, 0.7500000000000027756, 1.000000000000000000 ),
 .UNSPECIFIED. ) ;
#32665=CARTESIAN_POINT ( 'NONE',  ( 82.90600853043393670, 44.75983668713269026, 9.542372462439493219 ) ) ;
#32671=CARTESIAN_POINT ( 'NONE',  ( 74.14312167556930433, 66.30466486950707861, 1.224646799147354045E-15 ) ) ;
#32675=ADVANCED_FACE ( 'NONE', ( #2252 ), #47321, .T. ) ;
#32682=CARTESIAN_POINT ( 'NONE',  ( 14.85095921958720666, 14.28920272979925699, -7.433330006724141015 ) ) ;
#32683=CARTESIAN_POINT ( 'NONE',  ( 72.83042459652598666, 60.89494529775108589, -15.49726665856611163 ) ) ;
#32688=CARTESIAN_POINT ( 'NONE',  ( 20.83817183295411013, 35.52903772873357724, -1.583844403245363575 ) ) ;
#32690=CARTESIAN_POINT ( 'NONE',  ( 81.94814304414562400, 41.00889934599905473, -3.213059439476845913 ) ) ;
#32698=ORIENTED_EDGE ( 'NONE', *, *, #95424, .F. ) ;
#32699=B_SPLINE_SURFACE_WITH_KNOTS ( 'NONE', 3, 1, ( 
 ( #78365, #31721 ),
 ( #1857, #32739 ),
 ( #24147, #61634 ),
 ( #23623, #63644 ),
 ( #347, #70236 ),
 ( #840, #93580 ),
 ( #63142, #94087 ),
 ( #92586, #25136 ),
 ( #76842, #23129 ),
 ( #54024, #55032 ),
 ( #84979, #62121 ),
 ( #93069, #54517 ),
 ( #85495, #19576 ),
 ( #80905, #27157 ),
 ( #49441, #79395 ),
 ( #72271, #80396 ),
 ( #33770, #64657 ),
 ( #88510, #25660 ),
 ( #95606, #2366 ),
 ( #58044, #89026 ),
 ( #19073, #57031 ),
 ( #48451, #96594 ),
 ( #26155, #33244 ),
 ( #9962, #57533 ),
 ( #64145, #88014 ),
 ( #42820, #18563 ),
 ( #34248, #10965 ),
 ( #48957, #73750 ),
 ( #71767, #41838 ),
 ( #72783, #95096 ),
 ( #11958, #56539 ) ),
 .UNSPECIFIED., .F., .F., .F.,
 ( 4, 3, 3, 3, 3, 3, 3, 3, 3, 3, 4 ),
 ( 2, 2 ),
 ( 0.000000000000000000, 0.1122669598086760978, 0.2243161639709538580, 0.3396355846219034635, 0.4553962076585165719, 0.5677860799922357371, 0.6749047109689572110, 0.7773884377078412733, 0.8775581155834328850, 0.9782364162377978900, 1.000000000000000000 ),
 ( 0.000000000000000000, 1.000000000000000000 ),
 .UNSPECIFIED. ) ;
#32700=CARTESIAN_POINT ( 'NONE',  ( 79.47297740959983514, 51.20435970566347095, 15.10662661765129222 ) ) ;
#32701=CARTESIAN_POINT ( 'NONE',  ( 83.61754957953866096, 52.24592005514148951, -14.70745080183156972 ) ) ;
#32702=LINE ( 'NONE', #70703, #24217 ) ;
#32707=CARTESIAN_POINT ( 'NONE',  ( 35.38177548881301249, 32.37878583063844218, 9.188101187500006262 ) ) ;
#32714=CARTESIAN_POINT ( 'NONE',  ( 86.35458572345136474, 46.97350791603361131, -10.52386536561718700 ) ) ;
#32718=CARTESIAN_POINT ( 'NONE',  ( 73.98570270871887544, 68.92876820612472955, -11.10152750440661862 ) ) ;
#32725=CARTESIAN_POINT ( 'NONE',  ( 81.27629932712225980, 55.76935796986149541, 16.38776540150240990 ) ) ;
#32728=CARTESIAN_POINT ( 'NONE',  ( 78.99356797199125424, 52.14063585753078911, 15.48230155875487135 ) ) ;
#32731=CARTESIAN_POINT ( 'NONE',  ( 27.80420065655628648, 34.79103043416550634, 8.090169943749478065 ) ) ;
#32734=CARTESIAN_POINT ( 'NONE',  ( 82.51641340783935163, 40.44452228410568040, 0.9102053940968845014 ) ) ;
#32736=CARTESIAN_POINT ( 'NONE',  ( 76.67567146729663818, 63.34086528488000312, -15.41964329106467346 ) ) ;
#32739=CARTESIAN_POINT ( 'NONE',  ( 70.76698439857202061, 60.51306593283057111, -14.69096287377648657 ) ) ;
#32740=CARTESIAN_POINT ( 'NONE',  ( 36.38853680410606728, 41.98502408145596121, -5.678558825948271327 ) ) ;
#32743=FACE_OUTER_BOUND ( 'NONE', #72359, .T. ) ;
#32744=ORIENTED_EDGE ( 'NONE', *, *, #96915, .F. ) ;
#32749=CARTESIAN_POINT ( 'NONE',  ( 73.27264618352865000, 66.51157917954436982, 12.27253699350153404 ) ) ;
#32754=ORIENTED_EDGE ( 'NONE', *, *, #11844, .F. ) ;
#32758=CARTESIAN_POINT ( 'NONE',  ( 71.86256228778262312, 72.60615528678950170, -0.5650332253009007211 ) ) ;
#32773=CARTESIAN_POINT ( 'NONE',  ( 85.14411491811664234, 46.97365546850126350, 10.63533560768400044 ) ) ;
#32775=CARTESIAN_POINT ( 'NONE',  ( 67.87252889196815886, 69.68634872786070389, 1.786884576500594068 ) ) ;
#32779=CARTESIAN_POINT ( 'NONE',  ( 88.05007481205849729, 44.74915561242152506, -4.497590196485170999 ) ) ;
#32784=CARTESIAN_POINT ( 'NONE',  ( 78.45861607683767147, 57.52921583862547550, 16.22413336569833220 ) ) ;
#32785=CARTESIAN_POINT ( 'NONE',  ( 84.80383116528092557, 49.89350275441562843, -13.17492736023872091 ) ) ;
#32786=CARTESIAN_POINT ( 'NONE',  ( 78.02488749478023067, 61.97397559377148468, 15.68332185870741036 ) ) ;
#32794=CARTESIAN_POINT ( 'NONE',  ( 78.65123893946785927, 54.86935689443330944, -16.05544503379834964 ) ) ;
#32796=LINE ( 'NONE', #56078, #10910 ) ;
#32797=CARTESIAN_POINT ( 'NONE',  ( 71.66369827319218189, 72.02185750324218816, -1.551229696566573502 ) ) ;
#32800=CARTESIAN_POINT ( 'NONE',  ( 76.99381129068922291, 63.91386138922637628, -15.28064156999390732 ) ) ;
#32801=ADVANCED_FACE ( 'NONE', ( #37967 ), #14691, .T. ) ;
#32802=ADVANCED_FACE ( 'NONE', ( #76021 ), #9239, .T. ) ;
#32804=CARTESIAN_POINT ( 'NONE',  ( 88.19107160583139660, 43.69314304319705400, 0.1842422985582090333 ) ) ;
#32805=CARTESIAN_POINT ( 'NONE',  ( 83.40455683621979688, 49.60330724181036999, -13.41979453150748114 ) ) ;
#32809=CARTESIAN_POINT ( 'NONE',  ( 25.99623195869282100, 35.98502408145594700, -5.678558825948271327 ) ) ;
#32813=CARTESIAN_POINT ( 'NONE',  ( 24.83368966200164607, 16.19860640527292261, 2.839279412974134775 ) ) ;
#32815=CARTESIAN_POINT ( 'NONE',  ( 76.64464310018406934, 63.53199411942404851, 15.34601863127964627 ) ) ;
#32828=CARTESIAN_POINT ( 'NONE',  ( 67.68514482100736984, 66.83340866827894899, -8.536435324610977204 ) ) ;
#32829=CARTESIAN_POINT ( 'NONE',  ( 66.77376812102318127, 68.41195941748605946, -4.433129028897194068 ) ) ;
#32832=CARTESIAN_POINT ( 'NONE',  ( 72.48454840684568978, 71.59325672763723958, 6.192859277029556075 ) ) ;
#32836=EDGE_LOOP ( 'NONE', ( #17257, #26664, #44037, #6183 ) ) ;
#32838=CARTESIAN_POINT ( 'NONE',  ( 21.83270445532239989, 34.64646525600390703, -2.839279412974133887 ) ) ;
#32839=CARTESIAN_POINT ( 'NONE',  ( 75.12194974421997529, 66.37886708184480256, -13.15189938993499830 ) ) ;
#32840=CARTESIAN_POINT ( 'NONE',  ( 84.55133599061954897, 48.00037868907449479, -11.86301670575332068 ) ) ;
#32847=CARTESIAN_POINT ( 'NONE',  ( 68.04555932152995013, 65.72381589692875536, 10.88124144663173354 ) ) ;
#32854=CARTESIAN_POINT ( 'NONE',  ( 71.78107986572921106, 62.71246368623720002, -14.51539090988953440 ) ) ;
#32855=EDGE_CURVE ( 'NONE', #14695, #68463, #15539, .T. ) ;
#32861=CARTESIAN_POINT ( 'NONE',  ( 78.14027010749673252, 61.52421145379764766, -16.15198519767693242 ) ) ;
#32866=CARTESIAN_POINT ( 'NONE',  ( 80.31236711830932506, 44.94079046180152659, -11.22303980454576333 ) ) ;
#32868=DIRECTION ( 'NONE',  ( 0.8660254037844377084, 0.5000000000000015543, 0.000000000000000000 ) ) ;
#32870=CARTESIAN_POINT ( 'NONE',  ( 81.15909907030567183, 48.17545335780159377, -13.29838471746604966 ) ) ;
#32874=EDGE_LOOP ( 'NONE', ( #52622, #67880, #22903, #62083 ) ) ;
#32879=CARTESIAN_POINT ( 'NONE',  ( 19.48182849416020090, 34.18080186712593616, 3.090169943749475401 ) ) ;
#32882=CARTESIAN_POINT ( 'NONE',  ( 87.74222765753326314, 44.73834681983743877, 5.012736470890956753 ) ) ;
#32894=CARTESIAN_POINT ( 'NONE',  ( 83.08910943491284229, 41.56722408657803669, 2.852113461528766880 ) ) ;
#32896=CARTESIAN_POINT ( 'NONE',  ( 83.44503355366286712, 51.91352208420825320, 15.00625484349790284 ) ) ;
#32904=ADVANCED_FACE ( 'NONE', ( #25804 ), #40957, .T. ) ;
#32905=CARTESIAN_POINT ( 'NONE',  ( 33.22292548896825082, 27.38052372038642801, 10.00000000000000533 ) ) ;
#32920=CARTESIAN_POINT ( 'NONE',  ( 81.97536373108215457, 41.18676643964585793, 5.503149011488202902 ) ) ;
#32923=CARTESIAN_POINT ( 'NONE',  ( 39.22461576370143632, 27.81029122506297568, 8.090169943749479842 ) ) ;
#32929=PRODUCT ( 'Center Base Mounting Screw', 'Center Base Mounting Screw', '', ( #75570 ) ) ;
#32933=CARTESIAN_POINT ( 'NONE',  ( 74.40040945360185276, 65.95912601619707516, -13.09620949053549666 ) ) ;
#32946=CARTESIAN_POINT ( 'NONE',  ( 22.11595037535113661, 30.95586893147756413, 7.433330006724141015 ) ) ;
#32951=CARTESIAN_POINT ( 'NONE',  ( 7.668962567711002265, 16.37878583063838533, 9.188101187500006262 ) ) ;
#32953=CARTESIAN_POINT ( 'NONE',  ( 72.06083603792721703, 60.17315645985856065, -15.09511454206493042 ) ) ;
#32957=FACE_OUTER_BOUND ( 'NONE', #74283, .T. ) ;
#32964=ORIENTED_EDGE ( 'NONE', *, *, #72781, .F. ) ;
#32966=CARTESIAN_POINT ( 'NONE',  ( 72.06656620204616104, 72.31304997165260318, -3.465063205002326452 ) ) ;
#32967=CARTESIAN_POINT ( 'NONE',  ( 68.88004550269626236, 70.89535253697187045, -0.8688780715835217050 ) ) ;
#32968=CARTESIAN_POINT ( 'NONE',  ( 3.124773676633713748, 24.73705186507751463, -3.090169943749475845 ) ) ;
#32975=ADVANCED_FACE ( 'NONE', ( #98701 ), #66775, .T. ) ;
#32979=CARTESIAN_POINT ( 'NONE',  ( 28.30082151474694641, 24.84335787977763843, 9.188101187500006262 ) ) ;
#32981=CARTESIAN_POINT ( 'NONE',  ( 70.93672144898081910, 70.68531007502453178, -6.225600342418550426 ) ) ;
#32984=CARTESIAN_POINT ( 'NONE',  ( 73.93840856004327122, 68.59252082510937498, 11.39217114877861547 ) ) ;
#32990=CARTESIAN_POINT ( 'NONE',  ( 73.47351968716873216, 58.90398476228797620, -15.65848594678527839 ) ) ;
#33003=CARTESIAN_POINT ( 'NONE',  ( 88.05246585649720714, 43.65063640626211594, -1.233213520688016374 ) ) ;
#33004=CARTESIAN_POINT ( 'NONE',  ( 67.52528295890758159, 67.08866990654458107, 8.951888472663769747 ) ) ;
#33005=CARTESIAN_POINT ( 'NONE',  ( 73.19903135511377457, 64.92610867417256770, -13.26410356664282553 ) ) ;
#33006=CARTESIAN_POINT ( 'NONE',  ( 5.530962353892125094, 15.14441083166257584, 0.000000000000000000 ) ) ;
#33010=CARTESIAN_POINT ( 'NONE',  ( 83.29340746618338187, 41.55334719867666848, 2.042985643346537206 ) ) ;
#33015=CARTESIAN_POINT ( 'NONE',  ( 83.90892505094211629, 51.89215068963646615, -14.49862402916220461 ) ) ;
#33023=CARTESIAN_POINT ( 'NONE',  ( 73.55652807945510574, 69.73106060664957795, -9.395567069825068174 ) ) ;
#33028=CARTESIAN_POINT ( 'NONE',  ( 73.41965926039753754, 61.58357384648181920, -15.38293892878691160 ) ) ;
#33030=CARTESIAN_POINT ( 'NONE',  ( 88.04743768874705268, 44.61440943640608481, -4.110277753786412802 ) ) ;
#33032=CARTESIAN_POINT ( 'NONE',  ( 71.56516262931459949, 71.04936870583668451, -5.185425663852958778 ) ) ;
#33046=CARTESIAN_POINT ( 'NONE',  ( 15.34872451668155868, 24.56454794089041016, 10.00000000000000355 ) ) ;
#33047=CARTESIAN_POINT ( 'NONE',  ( 67.97219646607847210, 65.51810466360356600, -10.31124141321363830 ) ) ;
#33048=CARTESIAN_POINT ( 'NONE',  ( 76.28872632190459058, 51.00282802105012081, -16.03419075268624994 ) ) ;
#33050=CARTESIAN_POINT ( 'NONE',  ( 66.60908278236352942, 68.04996951702554497, -6.508824207629166914 ) ) ;
#33052=CARTESIAN_POINT ( 'NONE',  ( 5.551812139918021138, 18.90829794293878408, 10.00000000000000355 ) ) ;
#33066=CARTESIAN_POINT ( 'NONE',  ( 34.28181963472369631, 41.83396525600392835, -2.839279412974133887 ) ) ;
#33070=CARTESIAN_POINT ( 'NONE',  ( 30.35763184873497877, 26.03085787977764198, 9.188101187500006262 ) ) ;
#33074=CARTESIAN_POINT ( 'NONE',  ( 65.88310562884009869, 69.02589174572793240, 1.996831191910242609 ) ) ;
#33075=ORIENTED_EDGE ( 'NONE', *, *, #62355, .T. ) ;
#33078=CARTESIAN_POINT ( 'NONE',  ( 7.601631632957884577, 27.49540643055185285, 3.479690158560446702E-15 ) ) ;
#33080=CARTESIAN_POINT ( 'NONE',  ( 19.25205234332785764, 23.06628583063841020, -9.188101187500006262 ) ) ;
#33082=CARTESIAN_POINT ( 'NONE',  ( 17.41845772768865075, 33.55466486950699334, -1.111400068045478839E-16 ) ) ;
#33083=CARTESIAN_POINT ( 'NONE',  ( 88.22249780726667723, 44.22164796532466369, -1.816046898853142855 ) ) ;
#33087=B_SPLINE_CURVE_WITH_KNOTS ( 'NONE', 3,
 ( #45072, #83117, #84615, #53658, #99297, #54149, #98807, #45562, #44560, #84133, #77492, #36973, #76011, #15156, #6589 ),
 .UNSPECIFIED., .F., .F.,
 ( 4, 2, 2, 2, 1, 2, 2, 4 ),
 ( 0.007447265025110824666, 0.1315163568969734964, 0.2555854487688362653, 0.5037236325125593606, 0.6277927243844221294, 0.6898272703203521816, 0.7518618162562823448, 1.000000000000000000 ),
 .UNSPECIFIED. ) ;
#33094=CARTESIAN_POINT ( 'NONE',  ( 86.30241807085522510, 47.23217017718856425, 10.82197119102028893 ) ) ;
#33096=CARTESIAN_POINT ( 'NONE',  ( 77.80689875040398817, 57.80620150817188829, 16.17428301622781461 ) ) ;
#33099=CARTESIAN_POINT ( 'NONE',  ( 78.39455052809223901, 61.40085115147536499, -15.85312059573208998 ) ) ;
#33100=CARTESIAN_POINT ( 'NONE',  ( 79.05300200689268308, 59.41537015362479224, -16.53193985632130847 ) ) ;
#33101=B_SPLINE_CURVE_WITH_KNOTS ( 'NONE', 3,
 ( #4834, #51921, #89475, #52403, #35715, #81369, #97544, #11937, #43301, #73727 ),
 .UNSPECIFIED., .F., .F.,
 ( 4, 2, 2, 2, 4 ),
 ( 0.000000000000000000, 0.2500000000000000000, 0.5000000000000000000, 0.7500000000000000000, 1.000000000000000000 ),
 .UNSPECIFIED. ) ;
#33112=ORIENTED_EDGE ( 'NONE', *, *, #43878, .F. ) ;
#33116=VERTEX_POINT ( 'NONE', #80929 ) ;
#33117=CARTESIAN_POINT ( 'NONE',  ( 77.56105267981614304, 49.72783448595330924, -15.46007777815280981 ) ) ;
#33119=CARTESIAN_POINT ( 'NONE',  ( 70.82976944384030560, 68.20446162899281717, 9.207867830786081953 ) ) ;
#33126=CARTESIAN_POINT ( 'NONE',  ( 15.27916758686040488, 29.79752408145592568, -5.678558825948271327 ) ) ;
#33133=CARTESIAN_POINT ( 'NONE',  ( 45.00959873851216031, 26.39040679176986970, 1.333680081654574804E-15 ) ) ;
#33142=CARTESIAN_POINT ( 'NONE',  ( 5.867642952189432215, 25.16126292948893450, -6.180339887498951690 ) ) ;
#33148=CARTESIAN_POINT ( 'NONE',  ( 82.39049329420826950, 40.94913840096306501, -1.238713965289769181 ) ) ;
#33149=CARTESIAN_POINT ( 'NONE',  ( 22.75701074986381656, 14.10801979619928659, 3.090169943749476733 ) ) ;
#33161=CARTESIAN_POINT ( 'NONE',  ( 74.21927401529055146, 68.62113723208385352, -11.51360559050239374 ) ) ;
#33167=CARTESIAN_POINT ( 'NONE',  ( 82.63346302021976442, 44.24771747269379318, 9.093021782927767305 ) ) ;
#33169=ADVANCED_FACE ( 'NONE', ( #20083 ), #89049, .T. ) ;
#33172=DIRECTION ( 'NONE',  ( 0.5242119900219359696, 0.000000000000000000, -0.8515878049368965641 ) ) ;
#33174=CARTESIAN_POINT ( 'NONE',  ( 69.11330294371380489, 64.33813860942547080, -11.97090107321349883 ) ) ;
#33187=CARTESIAN_POINT ( 'NONE',  ( 19.96532700332172183, 20.03085787977762422, 9.188101187500006262 ) ) ;
#33188=CARTESIAN_POINT ( 'NONE',  ( 75.15246256102729205, 67.05878861674010238, 13.14576163508979612 ) ) ;
#33189=CARTESIAN_POINT ( 'NONE',  ( 83.53204454370724363, 52.39401912150450613, -15.17729711222452416 ) ) ;
#33202=CARTESIAN_POINT ( 'NONE',  ( 71.90400658755808649, 72.53437165389429708, 1.750395423964768993 ) ) ;
#33211=CARTESIAN_POINT ( 'NONE',  ( 43.73469409959700016, 27.11110640527295956, -2.839279412974138328 ) ) ;
#33219=CARTESIAN_POINT ( 'NONE',  ( 79.29399852950436411, 59.91530550262321242, 16.14991020500348284 ) ) ;
#33220=DIRECTION ( 'NONE',  ( -0.2837547813814349507, -0.9281390619545439868, -0.2409172175609568534 ) ) ;
#33222=CARTESIAN_POINT ( 'NONE',  ( 75.20389695419315501, 52.88180760346911313, -15.99093876381489920 ) ) ;
#33228=CARTESIAN_POINT ( 'NONE',  ( 77.34702598425042197, 49.11609959051940422, -15.28751209942174860 ) ) ;
#33229=VERTEX_POINT ( 'NONE', #53923 ) ;
#33231=CARTESIAN_POINT ( 'NONE',  ( 78.67033018268951139, 50.72589383312638489, 15.10119772252972403 ) ) ;
#33239=B_SPLINE_CURVE_WITH_KNOTS ( 'NONE', 3,
 ( #83361, #68613, #30624, #36714, #53895, #98550, #44313, #7821, #17808, #48709, #75500, #12711, #28895, #66879, #44064, #52669, #36475, #74516, #6084, #6593, #60753, #22279, #37959, #52173, #45076, #13691, #89738, #83626, #36977, #45567, #68867 ),
 .UNSPECIFIED., .F., .F.,
 ( 4, 3, 3, 3, 3, 3, 3, 3, 3, 3, 4 ),
 ( 0.000000000000000000, 0.1333490885032321271, 0.3007194338854310423, 0.4699862290245110930, 0.5844252810809297261, 0.6686540514502729016, 0.7354980260655470392, 0.8028463152565559202, 0.8633854507757028340, 0.9437142632666930542, 1.000000000000000000 ),
 .UNSPECIFIED. ) ;
#33244=CARTESIAN_POINT ( 'NONE',  ( 70.79441317036970815, 61.10405584021994940, -14.44842289594245166 ) ) ;
#33245=CARTESIAN_POINT ( 'NONE',  ( 5.396842180905148112, 18.51421378149916563, -9.188101187500004485 ) ) ;
#33248=CARTESIAN_POINT ( 'NONE',  ( 85.67146519243034675, 48.43225591334719837, -12.22341872913517591 ) ) ;
#33257=CARTESIAN_POINT ( 'NONE',  ( 79.58936028502597537, 59.22294857574252802, 16.56770033466462166 ) ) ;
#33273=ORIENTED_EDGE ( 'NONE', *, *, #31734, .F. ) ;
#33276=CARTESIAN_POINT ( 'NONE',  ( 78.41477381122238910, 47.32040575024743134, -14.22103711499937617 ) ) ;
#33277=CARTESIAN_POINT ( 'NONE',  ( 73.38945809345867133, 65.55744267816019999, -12.97487857549163870 ) ) ;
#33278=VECTOR ( 'NONE', #88669, 1000.000000000000114 ) ;
#33286=CARTESIAN_POINT ( 'NONE',  ( 88.19523698511710563, 44.46804064255652378, -4.670053027270656187 ) ) ;
#33288=DIRECTION ( 'NONE',  ( 0.4996954135095463823, -0.8654978445076774163, -0.03489949670249753444 ) ) ;
#33289=CARTESIAN_POINT ( 'NONE',  ( 77.63260553344707660, 52.78140009998875115, 15.78914038458534641 ) ) ;
#33291=CARTESIAN_POINT ( 'NONE',  ( 67.49618919058045208, 67.03867160555277849, 8.996887788448240997 ) ) ;
#33292=CARTESIAN_POINT ( 'NONE',  ( 76.48237539624216197, 51.57453071699011105, 15.64553330800477404 ) ) ;
#33300=CARTESIAN_POINT ( 'NONE',  ( 66.37865437376702005, 68.04852424368543495, -4.838310726055023991 ) ) ;
#33302=CARTESIAN_POINT ( 'NONE',  ( 76.91165928263828278, 63.32913628365751180, -15.47028109333149715 ) ) ;
#33305=CARTESIAN_POINT ( 'NONE',  ( 83.88838745027602783, 50.86303177257806141, -14.42977140412262216 ) ) ;
#33307=CARTESIAN_POINT ( 'NONE',  ( 83.33117328246518696, 42.97812013064149284, -7.544556126886196701 ) ) ;
#33312=CARTESIAN_POINT ( 'NONE',  ( 31.76189289227714951, 20.19860640527293683, 2.839279412974134775 ) ) ;
#33316=CARTESIAN_POINT ( 'NONE',  ( 19.25205234332785764, 23.06628583063841020, -9.188101187500006262 ) ) ;
#33318=CARTESIAN_POINT ( 'NONE',  ( 76.60814547930165475, 63.80470055869116663, 14.86801040537077867 ) ) ;
#33323=( BOUNDED_CURVE ( )  B_SPLINE_CURVE ( 2, ( #42452, #88638, #51053, #19695, #81511, #12081, #80520, #65759, #27281, #20186, #27775, #4985, #73386 ),
 .UNSPECIFIED., .F., .T. ) 
 B_SPLINE_CURVE_WITH_KNOTS ( ( 3, 2, 2, 2, 2, 2, 3 ),
 ( 0.1625000000000000056, 0.1650000000000000078, 0.1700000000000000122, 0.1749999999999999889, 0.1799999999999999933, 0.1849999999999999978, 0.1875000000000000000 ),
 .UNSPECIFIED. ) 
 CURVE ( )  GEOMETRIC_REPRESENTATION_ITEM ( )  RATIONAL_B_SPLINE_CURVE ( ( 0.9755282581475768211, 0.9755282581475768211, 1.000000000000000000, 0.9510565162951535312, 1.000000000000000000, 0.9510565162951535312, 1.000000000000000000, 0.9510565162951535312, 1.000000000000000000, 0.9510565162951535312, 1.000000000000000000, 0.9755282581475768211, 0.9755282581475768211 ) ) 
 REPRESENTATION_ITEM ( '' )  );
#33324=AXIS2_PLACEMENT_3D ( 'NONE', #86167, #1522, #79036 ) ;
#33325=CARTESIAN_POINT ( 'NONE',  ( 86.67919437798869353, 47.13106718819364716, 10.49222478779208068 ) ) ;
#33330=CARTESIAN_POINT ( 'NONE',  ( 75.35067983306640826, 53.14245299146813295, 16.48596124111078609 ) ) ;
#33344=CARTESIAN_POINT ( 'NONE',  ( 36.80649086932150027, 23.11110640527294535, -2.839279412974138328 ) ) ;
#33346=CARTESIAN_POINT ( 'NONE',  ( 84.76146393123151768, 50.45989236026047564, -13.93701821937661833 ) ) ;
#33347=CARTESIAN_POINT ( 'NONE',  ( 79.61387698796545465, 49.22643846628885456, -14.28797054368582486 ) ) ;
#33349=CARTESIAN_POINT ( 'NONE',  ( 83.10776606998568639, 40.75710275334526500, -2.573362665496658816E-06 ) ) ;
#33354=CARTESIAN_POINT ( 'NONE',  ( 67.66477494606748166, 65.93994996600352465, 10.43000743018374621 ) ) ;
#33359=CARTESIAN_POINT ( 'NONE',  ( 70.94055981774539532, 61.07284667920529131, 15.02700796178418408 ) ) ;
#33366=CARTESIAN_POINT ( 'NONE',  ( 77.96869982513443631, 61.39881034122267778, -16.15742658069109439 ) ) ;
#33369=ORIENTED_EDGE ( 'NONE', *, *, #74862, .T. ) ;
#33370=CARTESIAN_POINT ( 'NONE',  ( 79.90914067555259237, 44.54479442172742409, -11.07812196971692842 ) ) ;
#33371=CARTESIAN_POINT ( 'NONE',  ( 66.69061599261269180, 67.49838889342164805, 6.509093489976348401 ) ) ;
#33373=CARTESIAN_POINT ( 'NONE',  ( 83.71040786192132543, 41.77199054155873625, -1.945830175533111106 ) ) ;
#33374=CARTESIAN_POINT ( 'NONE',  ( 85.97400624412107106, 47.01443177752299363, -10.25505571482220013 ) ) ;
#33380=ORIENTED_EDGE ( 'NONE', *, *, #24798, .T. ) ;
#33384=ADVANCED_FACE ( 'NONE', ( #77123 ), #36623, .T. ) ;
#33386=CARTESIAN_POINT ( 'NONE',  ( 70.27108337839371188, 69.38421209371701082, -7.013144159806405931 ) ) ;
#33387=CARTESIAN_POINT ( 'NONE',  ( 87.65075002439434115, 44.95127668719692338, -6.583683359477274344 ) ) ;
#33389=CARTESIAN_POINT ( 'NONE',  ( 88.04001560340805099, 44.77405568574921091, 4.599260828767079978 ) ) ;
#33390=ORIENTED_EDGE ( 'NONE', *, *, #5142, .F. ) ;
#33392=CARTESIAN_POINT ( 'NONE',  ( 87.96802319852463370, 44.26031603380329926, -2.803967949215167454 ) ) ;
#33403=CARTESIAN_POINT ( 'NONE',  ( 85.33118850621276863, 44.02131733009327519, 6.393353383217204033 ) ) ;
#33404=CARTESIAN_POINT ( 'NONE',  ( 14.87430715154758687, 30.36126292948894445, 6.180339887498949913 ) ) ;
#33405=CARTESIAN_POINT ( 'NONE',  ( 77.82408648432202369, 62.02431454202515226, 15.64647534684074692 ) ) ;
#33415=CARTESIAN_POINT ( 'NONE',  ( 31.41726478770819853, 19.10801979619930435, 3.090169943749476733 ) ) ;
#33420=AXIS2_PLACEMENT_3D ( 'NONE', #56594, #72329, #88564 ) ;
#33422=CARTESIAN_POINT ( 'NONE',  ( 72.69493809724967548, 71.16443809380129437, -7.267007365939472052 ) ) ;
#33424=CARTESIAN_POINT ( 'NONE',  ( 81.55349978670373901, 45.99021204074624336, 11.55842612056192387 ) ) ;
#33428=CARTESIAN_POINT ( 'NONE',  ( 26.03432425566073150, 38.52903772873360566, -1.583844403245329602 ) ) ;
#33429=CARTESIAN_POINT ( 'NONE',  ( 72.13898424358956163, 72.32266849676254594, -1.187258607322207560 ) ) ;
#33431=EDGE_CURVE ( 'NONE', #51277, #23145, #77152, .T. ) ;
#33433=CARTESIAN_POINT ( 'NONE',  ( 31.96529204653334588, 20.58380873178789017, 6.180339887498953466 ) ) ;
#33434=CARTESIAN_POINT ( 'NONE',  ( 34.40128339993918871, 35.56454794089043503, 10.00000000000000355 ) ) ;
#33437=CARTESIAN_POINT ( 'NONE',  ( 72.57818625921403566, 63.87955903443374694, 14.16064695466623213 ) ) ;
#33438=CARTESIAN_POINT ( 'NONE',  ( 81.79443437784206594, 42.09912225842974465, 7.556739885930086054 ) ) ;
#33439=CARTESIAN_POINT ( 'NONE',  ( 87.11381950699171739, 46.35653380776409449, -8.652283511631230439 ) ) ;
#33440=CARTESIAN_POINT ( 'NONE',  ( 83.58343668721781228, 51.99607003748921841, 15.00733587213922426 ) ) ;
#33442=DIRECTION ( 'NONE',  ( -0.9532659690011954234, 0.2314883312386637471, 0.1941575258509202206 ) ) ;
#33451=DIRECTION ( 'NONE',  ( 0.5000000000000013323, -0.8660254037844378194, 0.000000000000000000 ) ) ;
#33457=CARTESIAN_POINT ( 'NONE',  ( 20.82173017108080515, 32.99752408145591431, 5.678558825948277544 ) ) ;
#33460=AXIS2_PLACEMENT_3D ( 'NONE', #35284, #19621, #49993 ) ;
#33463=VECTOR ( 'NONE', #95330, 1000.000000000000114 ) ;
#33464=CARTESIAN_POINT ( 'NONE',  ( 16.02188117849498639, 11.11110640527290983, -2.839279412974138328 ) ) ;
#33473=CARTESIAN_POINT ( 'NONE',  ( 84.14312167556933275, 48.98415679381830756, 0.000000000000000000 ) ) ;
#33481=CARTESIAN_POINT ( 'NONE',  ( 72.79456978488967422, 56.87432143794737982, -15.93777291093744708 ) ) ;
#33488=ORIENTED_EDGE ( 'NONE', *, *, #92930, .F. ) ;
#33489=AXIS2_PLACEMENT_3D ( 'NONE', #13844, #44228, #44721 ) ;
#33493=CARTESIAN_POINT ( 'NONE',  ( 33.10965510200716722, 34.51421378149920827, -9.188101187500004485 ) ) ;
#33495=CARTESIAN_POINT ( 'NONE',  ( 78.59318410106391184, 47.91850279518009614, -14.47096384754294363 ) ) ;
#33497=CARTESIAN_POINT ( 'NONE',  ( 73.96424987833113107, 68.60250435897062005, 11.39670188853133048 ) ) ;
#33503=CARTESIAN_POINT ( 'NONE',  ( 73.21300331465644717, 58.97917566933716671, -15.60506319839823064 ) ) ;
#33504=CARTESIAN_POINT ( 'NONE',  ( 85.72508672120996209, 43.23034436632222111, -3.633758481124208295 ) ) ;
#33507=ORIENTED_EDGE ( 'NONE', *, *, #97007, .F. ) ;
#33512=CARTESIAN_POINT ( 'NONE',  ( 81.65975360897576252, 52.35792944948207861, -15.54859200978484601 ) ) ;
#33518=B_SPLINE_CURVE_WITH_KNOTS ( 'NONE', 3,
 ( #39683, #47307, #81976, #50527, #73354, #27747, #98658, #13061, #4955, #19664, #13549, #82496, #59611, #67735, #58133, #42905, #90077, #29242, #81480, #12053, #73846, #58616, #65725, #4435, #66243, #27250, #5442, #35333, #11562, #89115, #28231 ),
 .UNSPECIFIED., .F., .F.,
 ( 4, 3, 3, 3, 3, 3, 3, 3, 3, 3, 4 ),
 ( 0.000000000000000000, 0.1333490885032416196, 0.3007194338854398130, 0.4699862290245220287, 0.5844252810809438259, 0.6686540514502733457, 0.7354980260655562541, 0.8028463152565635808, 0.8633854507757173780, 0.9437142632667323561, 1.000000000000000000 ),
 .UNSPECIFIED. ) ;
#33525=CARTESIAN_POINT ( 'NONE',  ( 83.83095627921952087, 51.88776739408810812, -14.90233955705620694 ) ) ;
#33526=CARTESIAN_POINT ( 'NONE',  ( 76.22397158102836556, 50.99593462407597855, -15.55193810795204179 ) ) ;
#33528=CARTESIAN_POINT ( 'NONE',  ( 80.34499676519902778, 57.43793486056498665, -16.58883017036144381 ) ) ;
#33532=CARTESIAN_POINT ( 'NONE',  ( 74.59892996465779902, 66.99479792721430726, 12.53190758343627031 ) ) ;
#33542=B_SPLINE_SURFACE_WITH_KNOTS ( 'NONE', 3, 1, ( 
 ( #98, #39558 ),
 ( #91828, #30981 ),
 ( #6695, #70482 ),
 ( #588, #54259 ),
 ( #31973, #31473 ),
 ( #76122, #68479 ),
 ( #62364, #85230 ),
 ( #38065, #77083 ),
 ( #99409, #68979 ),
 ( #38577, #61868 ),
 ( #93321, #99901 ),
 ( #30488, #61378 ),
 ( #92333, #3127 ),
 ( #65383, #10201 ),
 ( #80135, #26398 ),
 ( #10698, #96326 ),
 ( #79635, #95843 ),
 ( #73013, #41065 ),
 ( #48187, #48701 ),
 ( #94327, #78605 ),
 ( #71510, #79133 ),
 ( #56781, #34012 ),
 ( #72002, #55263 ),
 ( #64897, #55757 ),
 ( #86749, #87271 ),
 ( #57275, #41577 ),
 ( #40570, #11214 ),
 ( #1610, #2607 ),
 ( #33495, #71008 ),
 ( #80637, #17283 ),
 ( #9191, #86245 ) ),
 .UNSPECIFIED., .F., .F., .F.,
 ( 4, 3, 3, 3, 3, 3, 3, 3, 3, 3, 4 ),
 ( 2, 2 ),
 ( 0.000000000000000000, 0.1122669598086731141, 0.2243161639709448096, 0.3396355846218966912, 0.4553962076584983087, 0.5677860799922205270, 0.6749047109689384483, 0.7773884377078154051, 0.8775581155834121239, 0.9782364162377549244, 1.000000000000000000 ),
 ( 0.000000000000000000, 1.000000000000000000 ),
 .UNSPECIFIED. ) ;
#33551=CARTESIAN_POINT ( 'NONE',  ( 79.26853152882971187, 52.33679484845949759, -15.48194681045292320 ) ) ;
#33554=CARTESIAN_POINT ( 'NONE',  ( 18.44000607287492954, 15.81029122506293838, 8.090169943749479842 ) ) ;
#33557=CARTESIAN_POINT ( 'NONE',  ( 17.92595094200897776, 22.30066082961421259, -10.00000000000000533 ) ) ;
#33558=CARTESIAN_POINT ( 'NONE',  ( 68.02798755508815987, 65.19179537507288558, -10.68069436451683352 ) ) ;
#33559=CARTESIAN_POINT ( 'NONE',  ( 65.76829148152603466, 69.09872882758028823, 0.1165290730599739394 ) ) ;
#33562=CARTESIAN_POINT ( 'NONE',  ( 66.90909321525144549, 68.17756947874360662, -6.600776075497404527 ) ) ;
#33564=DIRECTION ( 'NONE',  ( -0.7235470741700504860, -0.1663964660674512042, 0.6699192843471690750 ) ) ;
#33569=CARTESIAN_POINT ( 'NONE',  ( 6.396987757676594555, 15.64441083166260427, 0.000000000000000000 ) ) ;
#33576=CARTESIAN_POINT ( 'NONE',  ( 32.54976882715482134, 40.83396525600392835, -2.839279412974133887 ) ) ;
#33581=CARTESIAN_POINT ( 'NONE',  ( 32.54976882715482134, 40.83396525600392835, -2.839279412974133887 ) ) ;
#33586=CARTESIAN_POINT ( 'NONE',  ( 11.99908958663318970, 18.87878583063839955, -9.188101187500006262 ) ) ;
#33588=CARTESIAN_POINT ( 'NONE',  ( 15.22926075146606273, 30.83396525600389637, -2.839279412974133887 ) ) ;
#33591=CARTESIAN_POINT ( 'NONE',  ( 84.83002093244189723, 50.29676582423640241, -13.82165720535206788 ) ) ;
#33597=CARTESIAN_POINT ( 'NONE',  ( 66.25889107252001509, 68.18093703880344947, 4.235875044229025832 ) ) ;
#33598=CARTESIAN_POINT ( 'NONE',  ( 87.62362232749241286, 45.09856358269391308, 6.901305344596342373 ) ) ;
#33603=CARTESIAN_POINT ( 'NONE',  ( 86.65390046659096868, 47.16758140886460637, 10.54653844973484489 ) ) ;
#33605=AXIS2_PLACEMENT_3D ( 'NONE', #43883, #43384, #4914 ) ;
#33606=CARTESIAN_POINT ( 'NONE',  ( 78.08056911966330915, 59.58490249653190318, 16.06997153095679209 ) ) ;
#33610=CARTESIAN_POINT ( 'NONE',  ( 84.46782944188609576, 48.58092674594113447, -12.38698248680477221 ) ) ;
#33612=CARTESIAN_POINT ( 'NONE',  ( 80.48572449743757318, 43.55285070694157668, 9.722916489287488417 ) ) ;
#33626=EDGE_LOOP ( 'NONE', ( #58757, #91419, #9916, #16321 ) ) ;
#33633=CARTESIAN_POINT ( 'NONE',  ( 72.01212875430924498, 70.46278977997356208, 6.938461426218038852 ) ) ;
#33639=VERTEX_POINT ( 'NONE', #63432 ) ;
#33641=CARTESIAN_POINT ( 'NONE',  ( 26.41418602390824333, 17.11110640527292759, -2.839279412974138328 ) ) ;
#33647=VECTOR ( 'NONE', #37461, 1000.000000000000114 ) ;
#33654=CARTESIAN_POINT ( 'NONE',  ( 79.14312167556931854, 57.64441083166269664, 0.000000000000000000 ) ) ;
#33663=CARTESIAN_POINT ( 'NONE',  ( 82.10040256005657966, 40.74948492577103565, -0.8666556322613548913 ) ) ;
#33664=CARTESIAN_POINT ( 'NONE',  ( 84.65919635822490363, 50.58401048434825498, 13.62798742565141907 ) ) ;
#33672=CARTESIAN_POINT ( 'NONE',  ( 88.16428468221791093, 44.07872432484457903, 0.5427949595267680394 ) ) ;
#33675=CARTESIAN_POINT ( 'NONE',  ( 86.32721218574307898, 47.55264674982593931, -11.12316258729871699 ) ) ;
#33676=CARTESIAN_POINT ( 'NONE',  ( 74.11446612904798315, 67.86722427140298919, -11.63493275082046452 ) ) ;
#33682=CARTESIAN_POINT ( 'NONE',  ( 82.17579637593928510, 43.45516270846064089, 8.362656290713127660 ) ) ;
#33686=EDGE_CURVE ( 'NONE', #30496, #50515, #85799, .T. ) ;
#33688=VECTOR ( 'NONE', #31368, 1000.000000000000114 ) ;
#33689=CARTESIAN_POINT ( 'NONE',  ( 68.70265395645864714, 63.99518547148130665, -12.05469093682469328 ) ) ;
#33694=CARTESIAN_POINT ( 'NONE',  ( 72.21141513960786540, 68.08919752073838083, -10.92203768660748153 ) ) ;
#33703=CARTESIAN_POINT ( 'NONE',  ( 17.52000153575897912, 22.06628583063841020, -9.188101187500006262 ) ) ;
#33705=EDGE_CURVE ( 'NONE', #66239, #7719, #45001, .T. ) ;
#33710=ORIENTED_EDGE ( 'NONE', *, *, #14539, .T. ) ;
#33715=CARTESIAN_POINT ( 'NONE',  ( 81.62115332376640708, 55.85468755722441614, -16.37141313285761512 ) ) ;
#33723=CARTESIAN_POINT ( 'NONE',  ( 80.24736013087236586, 55.07173234547738616, 15.97097506978094650 ) ) ;
#33724=CARTESIAN_POINT ( 'NONE',  ( 83.51092623577891061, 51.50185674319120466, -14.43088262691036583 ) ) ;
#33725=CARTESIAN_POINT ( 'NONE',  ( 72.11718761729461846, 71.53392678631075796, -5.852761162471809442 ) ) ;
#33730=CARTESIAN_POINT ( 'NONE',  ( 14.68538779211344902, 8.288480858562296660, 1.475505719884397138E-15 ) ) ;
#33733=CARTESIAN_POINT ( 'NONE',  ( 77.77576245277342082, 61.68761876588025217, 16.07113493600747844 ) ) ;
#33735=CARTESIAN_POINT ( 'NONE',  ( 87.13707957584176711, 44.08023128113844535, -5.302241763375429073 ) ) ;
#33737=CARTESIAN_POINT ( 'NONE',  ( 79.04010335995445757, 59.81086823702358402, 16.49488376190979722 ) ) ;
#33741=AXIS2_PLACEMENT_3D ( 'NONE', #28673, #36766, #97134 ) ;
#33745=APPLICATION_CONTEXT ( 'automotive_design' ) ;
#33748=ORIENTED_EDGE ( 'NONE', *, *, #35572, .F. ) ;
#33750=ORIENTED_EDGE ( 'NONE', *, *, #81599, .T. ) ;
#33751=CYLINDRICAL_SURFACE ( 'NONE', #67584, 16.60714546451156792 ) ;
#33757=CARTESIAN_POINT ( 'NONE',  ( 82.27971551521895321, 41.21092863865097655, 3.244910409712729926 ) ) ;
#33758=CARTESIAN_POINT ( 'NONE',  ( 80.89042375233061932, 43.66431198654377965, -9.574497798402536120 ) ) ;
#33761=VECTOR ( 'NONE', #46216, 1000.000000000000000 ) ;
#33770=CARTESIAN_POINT ( 'NONE',  ( 70.45109164464976459, 61.27252908298403611, -14.82318262686264987 ) ) ;
#33772=VERTEX_POINT ( 'NONE', #34049 ) ;
#33775=CARTESIAN_POINT ( 'NONE',  ( 82.59110617328815351, 43.40291750172000462, -8.843653439107631797 ) ) ;
#33780=CARTESIAN_POINT ( 'NONE',  ( 75.87525401958798454, 64.72722897157592570, -14.29033900848947169 ) ) ;
#33786=CARTESIAN_POINT ( 'NONE',  ( 76.46584302315547177, 51.61417680368897010, -15.65621440425051603 ) ) ;
#33789=ORIENTED_EDGE ( 'NONE', *, *, #87685, .F. ) ;
#33791=CARTESIAN_POINT ( 'NONE',  ( 66.31491329446379268, 68.86277721778741068, 0.1110262474478811850 ) ) ;
#33792=ORIENTED_EDGE ( 'NONE', *, *, #44896, .F. ) ;
#33802=B_SPLINE_SURFACE_WITH_KNOTS ( 'NONE', 3, 1, ( 
 ( #47647, #16261 ),
 ( #68956, #54745 ),
 ( #85732, #47153 ),
 ( #78584, #61848 ),
 ( #1072, #29966 ),
 ( #91805, #38552 ),
 ( #568, #53263 ),
 ( #92796, #61356 ),
 ( #23350, #54236 ),
 ( #14765, #30464 ),
 ( #8171, #85206 ),
 ( #92311, #22861 ),
 ( #53745, #46141 ),
 ( #39041, #31451 ),
 ( #84704, #8664 ),
 ( #39536, #31951 ),
 ( #62853, #71484 ),
 ( #11681, #79105 ),
 ( #26373, #19294 ),
 ( #9688, #63861 ),
 ( #49655, #42054 ),
 ( #95820, #95327 ),
 ( #57250, #10176 ),
 ( #48164, #72990 ),
 ( #64874, #57748 ),
 ( #11188, #56251 ),
 ( #41551, #79612 ),
 ( #50161, #2584 ),
 ( #3582, #94799 ),
 ( #70984, #48679 ),
 ( #34462, #10674 ) ),
 .UNSPECIFIED., .F., .F., .F.,
 ( 4, 3, 3, 3, 3, 3, 3, 3, 3, 3, 4 ),
 ( 2, 2 ),
 ( 0.000000000000000000, 0.1333490885032317108, 0.3007194338854392579, 0.4699862290245125918, 0.5844252810809411613, 0.6686540514502808952, 0.7354980260655639146, 0.8028463152565747940, 0.8633854507757208196, 0.9437142632667219200, 1.000000000000000000 ),
 ( 0.000000000000000000, 1.000000000000000000 ),
 .UNSPECIFIED. ) ;
#33803=CARTESIAN_POINT ( 'NONE',  ( 70.51282955450930956, 62.70216424510687148, -13.59275263340693130 ) ) ;
#33805=CARTESIAN_POINT ( 'NONE',  ( 75.20365466289253220, 64.98199045542118313, -13.95732831142939467 ) ) ;
#33807=CARTESIAN_POINT ( 'NONE',  ( 80.77766742949400225, 43.16040824514890772, -9.863399489045445279 ) ) ;
#33808=CARTESIAN_POINT ( 'NONE',  ( 66.99589590513352277, 68.94589010804261875, 3.022793341730511063 ) ) ;
#33811=CARTESIAN_POINT ( 'NONE',  ( 88.07382696622103424, 44.71549268748395889, -4.363432358687163060 ) ) ;
#33814=CARTESIAN_POINT ( 'NONE',  ( 75.13760321359936256, 55.20964237971745803, -16.13749542340338294 ) ) ;
#33820=CARTESIAN_POINT ( 'NONE',  ( 75.53863029606473845, 55.96446735458120969, -16.15547972021748180 ) ) ;
#33821=CARTESIAN_POINT ( 'NONE',  ( 74.15479259499207387, 55.62765001666249276, -16.59030973340311022 ) ) ;
#33823=CARTESIAN_POINT ( 'NONE',  ( 73.53729735990698657, 69.85633680769765874, 9.839233502311348190 ) ) ;
#33825=CARTESIAN_POINT ( 'NONE',  ( 76.69634485559663517, 63.33187278031594758, -15.42689205524521157 ) ) ;
#33826=AXIS2_PLACEMENT_3D ( 'NONE', #38350, #63161, #24166 ) ;
#33834=CIRCLE ( 'NONE', #51603, 0.5000000000000004441 ) ;
#33836=CARTESIAN_POINT ( 'NONE',  ( 37.28583507901048222, 30.03085787977765975, 9.188101187500006262 ) ) ;
#33840=CARTESIAN_POINT ( 'NONE',  ( 18.38602693954342371, 22.56628583063840310, 9.188101187500006262 ) ) ;
#33842=DIRECTION ( 'NONE',  ( 0.2938926261462335709, -0.5090369604551240323, 0.8090169943749504489 ) ) ;
#33849=EDGE_CURVE ( 'NONE', #25515, #29839, #13123, .T. ) ;
#33852=CARTESIAN_POINT ( 'NONE',  ( 72.51472823790616928, 71.58500209747694498, 5.264689056060205097 ) ) ;
#33854=CARTESIAN_POINT ( 'NONE',  ( 87.27117856089937220, 44.98890866680353895, -6.231534082530008511 ) ) ;
#33857=CARTESIAN_POINT ( 'NONE',  ( 74.99170170892071496, 53.13635499159778419, 16.50622363577149443 ) ) ;
#33860=EDGE_LOOP ( 'NONE', ( #937, #46517, #51814, #14412 ) ) ;
#33864=ORIENTED_EDGE ( 'NONE', *, *, #17444, .F. ) ;
#33872=CARTESIAN_POINT ( 'NONE',  ( 26.65419051621551461, 38.49540643055189548, 3.479690158560446702E-15 ) ) ;
#33873=CARTESIAN_POINT ( 'NONE',  ( 83.24863284446355749, 48.31717972554097429, -12.63386792366998534 ) ) ;
#33874=CARTESIAN_POINT ( 'NONE',  ( 74.14312167556930433, 66.30466486950707861, 1.224646799147354045E-15 ) ) ;
#33877=ORIENTED_EDGE ( 'NONE', *, *, #6422, .T. ) ;
#33880=CARTESIAN_POINT ( 'NONE',  ( 68.13224077221879327, 65.78494403969656901, 10.87017445448774033 ) ) ;
#33882=CARTESIAN_POINT ( 'NONE',  ( 85.29362735876655677, 48.41412782346650800, 12.38048700662147716 ) ) ;
#33888=CARTESIAN_POINT ( 'NONE',  ( 79.19335676987149952, 59.81345803429233143, 16.50342877771832661 ) ) ;
#33893=B_SPLINE_CURVE_WITH_KNOTS ( 'NONE', 3,
 ( #83394, #75778, #6365, #99074, #91487, #22050, #52950, #14462, #45344, #92005, #84389, #45826, #7342, #38225, #69141, #1131, #88787, #17838, #64426, #41609, #2137, #42112, #73046, #49717 ),
 .UNSPECIFIED., .F., .F.,
 ( 4, 2, 2, 2, 2, 2, 2, 2, 2, 2, 2, 4 ),
 ( 0.000000000000000000, 0.1249999999999997780, 0.2499999999999995559, 0.3749999999999987788, 0.4374999999999988898, 0.4999999999999990008, 0.5624999999999991118, 0.6249999999999992228, 0.6874999999999993339, 0.7499999999999994449, 0.8749999999999996669, 1.000000000000000000 ),
 .UNSPECIFIED. ) ;
#33898=EDGE_CURVE ( 'NONE', #749, #42575, #55189, .T. ) ;
#33904=ORIENTED_EDGE ( 'NONE', *, *, #26037, .F. ) ;
#33907=CARTESIAN_POINT ( 'NONE',  ( 24.41587626779758580, 32.83478043621389020, -8.090169943749479842 ) ) ;
#33908=CARTESIAN_POINT ( 'NONE',  ( 72.72501144050022504, 69.27512644744767556, -9.364870738290214547 ) ) ;
#33911=CARTESIAN_POINT ( 'NONE',  ( 87.98321614449201888, 44.37542847539244661, 4.756797044073171499 ) ) ;
#33914=CARTESIAN_POINT ( 'NONE',  ( 87.73337331461395650, 44.19923036242353476, -3.116042966821523041 ) ) ;
#33916=CARTESIAN_POINT ( 'NONE',  ( 82.32665380160997870, 40.35341351610614424, -1.168632817617336839 ) ) ;
#33924=( BOUNDED_CURVE ( )  B_SPLINE_CURVE ( 2, ( #17183, #62269, #61782, #10, #23786, #62781, #38480, #93225, #78511, #76508, #92729, #54671, #39464 ),
 .UNSPECIFIED., .F., .T. ) 
 B_SPLINE_CURVE_WITH_KNOTS ( ( 3, 2, 2, 2, 2, 2, 3 ),
 ( 0.8625000000000000444, 0.8649999999999999911, 0.8699999999999999956, 0.8750000000000000000, 0.8800000000000000044, 0.8850000000000000089, 0.8875000000000000666 ),
 .UNSPECIFIED. ) 
 CURVE ( )  GEOMETRIC_REPRESENTATION_ITEM ( )  RATIONAL_B_SPLINE_CURVE ( ( 0.9755282581475767101, 0.9755282581475772652, 1.000000000000000000, 0.9510565162951535312, 1.000000000000000000, 0.9510565162951535312, 1.000000000000000000, 0.9510565162951535312, 1.000000000000000000, 0.9510565162951535312, 1.000000000000000000, 0.9755282581475761550, 0.9755282581475767101 ) ) 
 REPRESENTATION_ITEM ( '' )  );
#33926=CARTESIAN_POINT ( 'NONE',  ( 83.57754660192708229, 42.00176330557154358, 3.549989893534491792 ) ) ;
#33927=CARTESIAN_POINT ( 'NONE',  ( 13.95435611255089725, 31.55466486950698268, -1.111400068045478839E-16 ) ) ;
#33928=CARTESIAN_POINT ( 'NONE',  ( 78.17938457032805388, 61.84587351074209494, 15.72953426550225942 ) ) ;
#33932=CARTESIAN_POINT ( 'NONE',  ( 76.73689447628605365, 63.01357867417375758, -15.17253155338367954 ) ) ;
#33935=CARTESIAN_POINT ( 'NONE',  ( 38.51867309874058520, 23.20801979619931643, -3.090169943749474069 ) ) ;
#33936=CARTESIAN_POINT ( 'NONE',  ( 78.33040301246538206, 47.74919695098484596, 13.91169181636929864 ) ) ;
#33944=CARTESIAN_POINT ( 'NONE',  ( 83.07383449898573247, 51.69909393465605518, 14.61845402798252636 ) ) ;
#33946=CARTESIAN_POINT ( 'NONE',  ( 86.82730862513506054, 46.47781937394018570, 9.057350913429045747 ) ) ;
#33948=CARTESIAN_POINT ( 'NONE',  ( 82.00582843356828278, 41.75518532697849139, 5.420714220595918675 ) ) ;
#33950=CARTESIAN_POINT ( 'NONE',  ( 87.19358828159984398, 46.06351791880832991, 8.846884648199045742 ) ) ;
#33952=CARTESIAN_POINT ( 'NONE',  ( 40.97195624589149077, 25.78380873178790011, -6.180339887498949025 ) ) ;
#33957=CARTESIAN_POINT ( 'NONE',  ( 81.37766082491019404, 41.99711756777615079, 7.787696445709868520 ) ) ;
#33958=CARTESIAN_POINT ( 'NONE',  ( 86.76444126019433156, 45.86660341771495553, -8.261827951889216592 ) ) ;
#33959=DIRECTION ( 'NONE',  ( 0.000000000000000000, 0.000000000000000000, -1.000000000000000000 ) ) ;
#33961=EDGE_CURVE ( 'NONE', #3380, #20756, #56383, .T. ) ;
#33964=CARTESIAN_POINT ( 'NONE',  ( 75.66892512706360208, 65.56297878460881634, -13.78772485324686237 ) ) ;
#33965=LINE ( 'NONE', #50625, #46586 ) ;
#33972=CIRCLE ( 'NONE', #24264, 15.60714546451156970 ) ;
#33973=CARTESIAN_POINT ( 'NONE',  ( 67.57495667756568025, 66.81435014269607109, -8.472947009434754762 ) ) ;
#33974=ORIENTED_EDGE ( 'NONE', *, *, #78367, .F. ) ;
#33979=CARTESIAN_POINT ( 'NONE',  ( 23.19008890107777177, 36.49540643055188838, 3.479690158560446702E-15 ) ) ;
#33984=CARTESIAN_POINT ( 'NONE',  ( 17.47068606603513530, 15.80170272979925628, 7.433330006724137462 ) ) ;
#33987=ORIENTED_EDGE ( 'NONE', *, *, #30144, .F. ) ;
#34001=CARTESIAN_POINT ( 'NONE',  ( 72.61487623500035227, 57.17883103660691546, -16.35891038744556525 ) ) ;
#34002=CARTESIAN_POINT ( 'NONE',  ( 78.40116303218597693, 61.34120641638568827, -15.86691968629957650 ) ) ;
#34009=EDGE_LOOP ( 'NONE', ( #44802, #23494, #13649, #62769 ) ) ;
#34010=CARTESIAN_POINT ( 'NONE',  ( 36.08541434599421649, 23.76004757982091320, 5.678558825948272215 ) ) ;
#34012=CARTESIAN_POINT ( 'NONE',  ( 78.33244564584110492, 47.97788310747041152, -14.02544125455132651 ) ) ;
#34014=CARTESIAN_POINT ( 'NONE',  ( 74.13497556468038852, 68.62018799133311120, 11.47049235834078296 ) ) ;
#34020=CARTESIAN_POINT ( 'NONE',  ( 77.89397139995216435, 52.97378536012750061, 16.25196429188360625 ) ) ;
#34022=CARTESIAN_POINT ( 'NONE',  ( 70.16674147172682297, 69.76683255227192149, -6.105712478908892571 ) ) ;
#34024=CARTESIAN_POINT ( 'NONE',  ( 79.77196807731678518, 53.06786404022832215, -16.06017792100006503 ) ) ;
#34037=CARTESIAN_POINT ( 'NONE',  ( 79.50492434327871649, 59.51147149025595695, -16.19819612084857496 ) ) ;
#34038=CARTESIAN_POINT ( 'NONE',  ( 74.27219104505947200, 58.60180873485686703, 15.82987398880578134 ) ) ;
#34040=ORIENTED_EDGE ( 'NONE', *, *, #53901, .F. ) ;
#34041=CARTESIAN_POINT ( 'NONE',  ( 80.48345259418954356, 57.73457509892514139, -16.59664598758602949 ) ) ;
#34047=AXIS2_PLACEMENT_3D ( 'NONE', #78774, #17456, #3770 ) ;
#34049=CARTESIAN_POINT ( 'NONE',  ( 66.46320885748656337, 68.94986384069261476, 0.01364106734875079018 ) ) ;
#34052=CARTESIAN_POINT ( 'NONE',  ( 15.92326719930538204, 21.14441083166260071, 10.00000000000000533 ) ) ;
#34060=CARTESIAN_POINT ( 'NONE',  ( 77.75060393840874440, 52.81207349147976515, -15.76950510618580203 ) ) ;
#34063=CARTESIAN_POINT ( 'NONE',  ( 66.49206384107228018, 67.79058194764397172, -6.885858948892061626 ) ) ;
#34068=CARTESIAN_POINT ( 'NONE',  ( 15.24912932961584744, 31.73705186507753950, -3.090169943749475845 ) ) ;
#34071=CARTESIAN_POINT ( 'NONE',  ( 72.30187851786844533, 71.99614501073629924, -3.638213215807910572 ) ) ;
#34073=CARTESIAN_POINT ( 'NONE',  ( 73.74125571288574577, 55.30219098885146423, -16.59355670855032372 ) ) ;
#34085=CARTESIAN_POINT ( 'NONE',  ( 29.80674373534435162, 38.18502408145592852, 5.678558825948277544 ) ) ;
#34089=CARTESIAN_POINT ( 'NONE',  ( 38.14222467998226307, 24.94754757982092386, 5.678558825948272215 ) ) ;
#34094=CARTESIAN_POINT ( 'NONE',  ( 4.137530017820134631, 25.49540643055185285, 3.479690158560446702E-15 ) ) ;
#34096=CARTESIAN_POINT ( 'NONE',  ( 19.52749640002317122, 16.98920272979925628, 7.433330006724137462 ) ) ;
#34105=CARTESIAN_POINT ( 'NONE',  ( 66.31578965481824639, 68.16347547130251883, 4.387282884348506329 ) ) ;
#34106=CARTESIAN_POINT ( 'NONE',  ( 87.60007719130888404, 45.49888764405456953, 6.854024160836727830 ) ) ;
#34108=ORIENTED_EDGE ( 'NONE', *, *, #74921, .F. ) ;
#34110=CARTESIAN_POINT ( 'NONE',  ( 86.50957498950597824, 47.24826369376732771, 10.71680696257866394 ) ) ;
#34111=ORIENTED_EDGE ( 'NONE', *, *, #86371, .T. ) ;
#34115=CARTESIAN_POINT ( 'NONE',  ( 36.35590661721340666, 26.15404122711136026, 8.090169943749479842 ) ) ;
#34116=CARTESIAN_POINT ( 'NONE',  ( 83.18584357961942999, 48.96896753446518602, -13.12400861552115572 ) ) ;
#34117=CARTESIAN_POINT ( 'NONE',  ( 80.77639761371902694, 43.06272340307192792, 9.748640195465013036 ) ) ;
#34126=EDGE_LOOP ( 'NONE', ( #9402, #93672, #14842, #26288, #60744 ) ) ;
#34128=VECTOR ( 'NONE', #59867, 1000.000000000000227 ) ;
#34132=CARTESIAN_POINT ( 'NONE',  ( 71.04820796358482937, 68.65144407467539622, 8.809617914912280412 ) ) ;
#34134=CARTESIAN_POINT ( 'NONE',  ( 86.35121876318000034, 43.08468197994678661, 0.3078304325362931637 ) ) ;
#34138=CARTESIAN_POINT ( 'NONE',  ( 20.27385872851041526, 33.74646525600390135, 2.839279412974139660 ) ) ;
#34145=CARTESIAN_POINT ( 'NONE',  ( 69.86972952878745957, 62.75331692225537239, 13.91736506036380661 ) ) ;
#34147=CARTESIAN_POINT ( 'NONE',  ( 19.07322413485131563, 11.41603393254324139, -1.583844403245362020 ) ) ;
#34152=CARTESIAN_POINT ( 'NONE',  ( 70.02414138031360835, 62.78214778883172187, 13.38063900663788885 ) ) ;
#34153=PLANE ( 'NONE',  #59244 ) ;
#34163=ORIENTED_EDGE ( 'NONE', *, *, #65299, .T. ) ;
#34166=CARTESIAN_POINT ( 'NONE',  ( 88.07432094012324342, 44.02706539047903789, 0.5635391379978663684 ) ) ;
#34167=CARTESIAN_POINT ( 'NONE',  ( 84.35036076898174429, 44.10653668295481822, 7.536754518051668406 ) ) ;
#34169=CARTESIAN_POINT ( 'NONE',  ( 14.42807667092211865, 8.734156793818204534, -7.779800476318352071E-15 ) ) ;
#34174=EDGE_LOOP ( 'NONE', ( #64734, #71750, #11945, #21446 ) ) ;
#34175=CARTESIAN_POINT ( 'NONE',  ( 84.34447119165866980, 48.35867903125333100, 12.23554050903201151 ) ) ;
#34178=CARTESIAN_POINT ( 'NONE',  ( 69.00853799725599913, 64.33131446021079114, -11.92797522396560872 ) ) ;
#34180=CARTESIAN_POINT ( 'NONE',  ( 79.96162642484517846, 48.81434648651384833, 14.52309195649116269 ) ) ;
#34187=ORIENTED_EDGE ( 'NONE', *, *, #90035, .T. ) ;
#34193=CARTESIAN_POINT ( 'NONE',  ( 19.25205234332785764, 23.06628583063841020, -9.188101187500006262 ) ) ;
#34194=CARTESIAN_POINT ( 'NONE',  ( 74.92662977279880465, 67.20364597524810790, 12.51845076170456572 ) ) ;
#34200=VERTEX_POINT ( 'NONE', #39062 ) ;
#34205=CARTESIAN_POINT ( 'NONE',  ( 81.62646408706272894, 55.64454924624774890, -16.33875670839028871 ) ) ;
#34206=ORIENTED_EDGE ( 'NONE', *, *, #16957, .F. ) ;
#34211=CARTESIAN_POINT ( 'NONE',  ( 83.91531380489591641, 51.74629119495582330, -14.43556620278794611 ) ) ;
#34214=( BOUNDED_SURFACE ( )  B_SPLINE_SURFACE ( 1, 2, ( 
 ( #29560, #36151, #90913, #52848, #74693, #14847, #21462, #38126, #82810, #68053, #7244, #59436, #84299, #5757, #43749, #97978, #6759, #61442, #22941, #28554, #83295, #12893, #90418, #13859, #13378, #75672, #44247, #6257, #67553, #37637, #98486, #29077, #37154, #60434, #91390, #83798, #14362, #45248, #45733, #53349, #76656, #68548, #99473, #60939, #91899, #69043, #99973, #30558, #61930, #8751, #23940, #93896, #8259, #9258, #24450, #86308, #62427, #23436, #54840, #46749, #55331, #85821, #16350, #15331, #32034, #39124, #32554, #24941, #40130, #84790, #46226, #31538, #92882, #47244, #77148, #93388, #31043, #71070, #155, #54325, #53830, #78164, #85296, #7752, #651, #15840, #55819, #86812, #17344, #39622, #38645, #62946, #69550, #78667, #1671, #77675, #70038, #70544, #1160, #16843, #47733, #63452, #94388, #48252, #79199, #9772, #40634, #71569, #2165, #33046, #63945, #94884, #3667, #80193, #4140, #96893, #81195, #34545, #50730, #81685, #33557, #2666, #48764, #11764, #64959, #73556, #73069, #64452, #65443, #35542, #96388, #26952, #35035, #95412, #57338, #12258, #65939, #87823, #27463, #11277, #56838, #10761, #42627, #79697, #34068, #26462, #25968, #25446, #43116, #58333, #56336, #95904, #87335, #88312, #57835, #18362, #41128, #19382, #88816, #18866, #50241, #49748, #41635, #89309, #19863, #17867, #74060, #49257, #4649, #72579, #10259, #72066, #80701, #3185, #82195, #37031, #13734, #20357, #75057, #67939, #89781, #29930, #5634, #53231, #97859, #83172, #22332, #74570, #99352, #20861, #58819, #51227, #21834, #76544, #38007, #12766, #67428, #28430, #43631, #91269, #75549, #28948, #98860, #21343, #51752, #29437, #60807, #7123, #52719, #90291, #45126, #36029, #97371, #37519, #59826, #98359, #5148, #60311, #44614, #66929, #36527, #83679, #59312, #91767, #90791, #84183, #82694, #6134, #14732, #13260, #45615, #44120, #52227, #14240, #76064, #27937, #6644, #68424, #39013, #99846, #30429, #46619, #77022, #69919, #92281, #8138, #46108, #24334, #15213, #38519, #68920, #533, #69429, #61320, #15718, #7628, #70946, #40007, #1550, #31419, #22828, #47122, #53713, #93776, #16729, #45, #30929, #23819, #62308, #8634, #23318, #55211, #39501, #1037, #77549, #61813, #93264, #92763, #70428, #54711, #85693, #84671, #78045, #54206, #47620, #32433, #86193, #31916, #94269, #24824, #85174, #16232, #62820, #78547, #9135, #63328, #55699, #86687, #17219, #79070, #48126, #9655, #19262, #10140, #72461, #96772, #50129, #2549, #11647, #26340, #71947, #25850, #26834, #94763, #49138, #41517, #41005, #81565, #27338, #42507, #71448, #80072, #50611, #3066, #11158, #10643, #40513, #79579, #64839, #33434, #87209, #2037, #32923, #58219, #42025, #18245, #89198, #33952, #88692, #73443, #81081, #18740, #95786, #57216, #19746, #88191, #72959, #64331, #63827, #48644, #49624, #56212, #25326, #17744, #80578, #95290, #56726, #87709, #3551, #34429, #4027, #65329, #34913, #96268, #57712, #65811, #44505, #13631, #75434, #66328, #36409, #74454, #66817, #60193, #91650, #14124, #6527, #97745, #52603, #4522, #98241, #13142, #67313, #43999, #83560, #60692, #29818, #59191, #27827, #97260, #59710, #42998, #98747, #53114, #28827, #83058, #36912, #45005, #5034, #67825, #51110 ),
 ( #58703, #75951, #37403, #68309, #74941, #35423, #90676, #12136, #29327, #91153, #12645, #20238, #21232, #82579, #52111, #28313, #21719, #6018, #99232, #20740, #82075, #5525, #35916, #22217, #73936, #89677, #43515, #90167, #51627, #62699, #55101, #39391, #93146, #9016, #39888, #92173, #61206, #7011, #70308, #23203, #54094, #84071, #22723, #8031, #53602, #30319, #94156, #24709, #1432, #85574, #61701, #70823, #77433, #31797, #86088, #93656, #62195, #38904, #92653, #63214, #85050, #54592, #7505, #37896, #84560, #69808, #99732, #32313, #14624, #418, #15099, #45990, #76436, #68804, #76907, #24221, #38402, #16612, #15597, #69315, #100237, #16118, #47016, #77931, #30821, #31307, #46497, #23697, #47508, #45503, #78435, #8522, #921, #96157, #48005, #41402, #56614, #79959, #87598, #26720, #3918, #73331, #2438, #71335, #9537, #2951, #86575, #41913, #96657, #72346, #26224, #80465, #57602, #48528, #11036, #94656, #34317, #25211, #34801, #57100, #50018, #65703, #88582, #79465, #10527, #78949, #56095, #40891, #63718, #17108, #33840, #64215, #10029, #88082, #87088, #40398, #72848, #3440, #17624, #19144, #33316, #64728, #95677, #95166, #55592, #25734, #49511, #65215, #80972, #11537, #42397, #18124, #71840, #1927, #32813, #35810, #35307, #28204, #60086, #4931, #50501, #98637, #59080, #13036, #66219, #67204, #67710, #81950, #28710, #5908, #97158, #90051, #83444, #36798, #89565, #29219, #43898, #58592, #12527, #13526, #81455, #66704, #20623, #27724, #68194, #14011, #91049, #58110, #97639, #37297, #51507, #98126, #20127, #42883, #21133, #5418, #82474, #59588, #74838, #43399, #90564, #21616, #27227, #52010, #50999, #75329, #74342, #89092, #52496, #36300, #82953, #12027, #44394, #44889, #73819, #75830, #6416, #19641, #4411, #7392, #56359, #99622, #84935, #25469, #76324, #2187, #22603, #60582, #91538, #24961, #79717, #41150, #83949, #69193, #29705, #22102, #76799, #6899, #100122, #52998, #38282, #37788, #55839, #45394, #68689, #99123, #30707, #30200, #14511, #45875, #61086, #33070, #71592, #63964, #61587, #92057, #77306, #53491, #86834, #48274, #84443, #14988, #53977, #92538, #38788, #23085, #17367, #69694, #31186, #15481, #46376, #7913, #299, #62077, #94408, #79220, #9794, #40654, #94907, #87358, #17887, #48786, #10280, #97385, #27953, #80214, #49277, #95436, #27482, #11298, #19881, #19401, #10782, #88837, #82213, #50260, #41657, #89800, #73575, #66460, #20374, #74078, #64978, #65465, #25988, #72600, #57357, #3204, #2689, #81213, #80724, #26482, #4158, #34089, #56857, #89328, #58350, #95921, #4668, #18888, #11787, #57857, #49768, #51245, #42157, #42644, #35053, #65961, #96911, #50751, #73092, #88333, #81703, #58834, #3685, #34564, #96406, #35559, #26975, #87843, #43137, #12276, #12783, #72088, #33581, #64475, #18382, #13750, #43648, #82710, #67954, #13277, #90308, #53727, #84686, #61334, #45143, #21361, #30444, #37046, #91783, #45628, #53245, #21850, #98874, #52246, #22844, #44631, #14255, #67449, #66946, #51768, #29452, #59328, #92293, #74587, #60328, #44139, #20879, #36044, #97875, #75073, #84201, #98377, #14747, #83190, #5653, #36542, #76082, #6657, #37534, #28449, #91284, #28965, #59844, #22349, #5165, #76557, #38023, #90806, #7136 ) ),
 .UNSPECIFIED., .F., .F., .T. ) 
 B_SPLINE_SURFACE_WITH_KNOTS ( ( 2, 2 ),
 ( 3, 2, 2, 2, 2, 2, 2, 2, 2, 2, 2, 2, 2, 2, 2, 2, 2, 2, 2, 2, 2, 2, 2, 2, 2, 2, 2, 2, 2, 2, 2, 2, 2, 2, 2, 2, 2, 2, 2, 2, 2, 2, 2, 2, 2, 2, 2, 2, 2, 2, 2, 2, 2, 2, 2, 2, 2, 2, 2, 2, 2, 2, 2, 2, 2, 2, 2, 2, 2, 2, 2, 2, 2, 2, 2, 2, 2, 2, 2, 2, 2, 2, 2, 2, 2, 2, 2, 2, 2, 2, 2, 2, 2, 2, 2, 2, 2, 2, 2, 2, 2, 2, 2, 2, 2, 2, 2, 2, 2, 2, 2, 2, 2, 2, 2, 2, 2, 2, 2, 2, 2, 2, 2, 2, 2, 2, 2, 2, 2, 2, 2, 2, 2, 2, 2, 2, 2, 2, 2, 2, 2, 2, 2, 2, 2, 2, 2, 2, 2, 2, 2, 2, 2, 2, 2, 2, 2, 2, 2, 2, 2, 2, 2, 2, 2, 2, 2, 2, 2, 2, 2, 2, 2, 2, 2, 2, 2, 2, 2, 2, 2, 2, 2, 2, 2, 2, 2, 2, 2, 2, 2, 2, 2, 2, 2, 2, 2, 2, 2, 2, 3 ),
 ( 0.000000000000000000, 1.000000000000000000 ),
 ( 0.000000000000000000, 0.005000000000000000104, 0.01000000000000000021, 0.01499999999999999944, 0.02000000000000000042, 0.02500000000000000139, 0.02999999999999999889, 0.03500000000000000333, 0.04000000000000000083, 0.04499999999999999833, 0.05000000000000000278, 0.05500000000000000028, 0.05999999999999999778, 0.06500000000000000222, 0.07000000000000000666, 0.07499999999999999722, 0.08000000000000000167, 0.08500000000000000611, 0.08999999999999999667, 0.09500000000000000111, 0.1000000000000000056, 0.1049999999999999961, 0.1100000000000000006, 0.1150000000000000050, 0.1199999999999999956, 0.1250000000000000000, 0.1300000000000000044, 0.1350000000000000089, 0.1400000000000000133, 0.1449999999999999900, 0.1499999999999999944, 0.1549999999999999989, 0.1600000000000000033, 0.1650000000000000078, 0.1700000000000000122, 0.1749999999999999889, 0.1799999999999999933, 0.1849999999999999978, 0.1900000000000000022, 0.1950000000000000067, 0.2000000000000000111, 0.2049999999999999878, 0.2099999999999999922, 0.2149999999999999967, 0.2200000000000000011, 0.2250000000000000056, 0.2300000000000000100, 0.2349999999999999867, 0.2399999999999999911, 0.2449999999999999956, 0.2500000000000000000, 0.2550000000000000044, 0.2600000000000000089, 0.2650000000000000133, 0.2700000000000000178, 0.2750000000000000222, 0.2800000000000000266, 0.2849999999999999756, 0.2899999999999999800, 0.2949999999999999845, 0.2999999999999999889, 0.3049999999999999933, 0.3099999999999999978, 0.3150000000000000022, 0.3200000000000000067, 0.3250000000000000111, 0.3300000000000000155, 0.3350000000000000200, 0.3400000000000000244, 0.3449999999999999734, 0.3499999999999999778, 0.3549999999999999822, 0.3599999999999999867, 0.3649999999999999911, 0.3699999999999999956, 0.3750000000000000000, 0.3800000000000000044, 0.3850000000000000089, 0.3900000000000000133, 0.3950000000000000178, 0.4000000000000000222, 0.4050000000000000266, 0.4099999999999999756, 0.4149999999999999800, 0.4199999999999999845, 0.4249999999999999889, 0.4299999999999999933, 0.4349999999999999978, 0.4400000000000000022, 0.4450000000000000067, 0.4500000000000000111, 0.4550000000000000155, 0.4600000000000000200, 0.4650000000000000244, 0.4699999999999999734, 0.4749999999999999778, 0.4799999999999999822, 0.4849999999999999867, 0.4899999999999999911, 0.4949999999999999956, 0.5000000000000000000, 0.5050000000000000044, 0.5100000000000000089, 0.5150000000000000133, 0.5200000000000000178, 0.5250000000000000222, 0.5300000000000000266, 0.5350000000000000311, 0.5400000000000000355, 0.5450000000000000400, 0.5500000000000000444, 0.5550000000000000488, 0.5600000000000000533, 0.5649999999999999467, 0.5699999999999999512, 0.5749999999999999556, 0.5799999999999999600, 0.5849999999999999645, 0.5899999999999999689, 0.5949999999999999734, 0.5999999999999999778, 0.6049999999999999822, 0.6099999999999999867, 0.6149999999999999911, 0.6199999999999999956, 0.6250000000000000000, 0.6300000000000000044, 0.6350000000000000089, 0.6400000000000000133, 0.6450000000000000178, 0.6500000000000000222, 0.6550000000000000266, 0.6600000000000000311, 0.6650000000000000355, 0.6700000000000000400, 0.6750000000000000444, 0.6800000000000000488, 0.6850000000000000533, 0.6899999999999999467, 0.6949999999999999512, 0.6999999999999999556, 0.7049999999999999600, 0.7099999999999999645, 0.7149999999999999689, 0.7199999999999999734, 0.7249999999999999778, 0.7299999999999999822, 0.7349999999999999867, 0.7399999999999999911, 0.7449999999999999956, 0.7500000000000000000, 0.7550000000000000044, 0.7600000000000000089, 0.7650000000000000133, 0.7700000000000000178, 0.7750000000000000222, 0.7800000000000000266, 0.7850000000000000311, 0.7900000000000000355, 0.7950000000000000400, 0.8000000000000000444, 0.8050000000000000488, 0.8100000000000000533, 0.8149999999999999467, 0.8199999999999999512, 0.8249999999999999556, 0.8299999999999999600, 0.8349999999999999645, 0.8399999999999999689, 0.8449999999999999734, 0.8499999999999999778, 0.8549999999999999822, 0.8599999999999999867, 0.8649999999999999911, 0.8699999999999999956, 0.8750000000000000000, 0.8800000000000000044, 0.8850000000000000089, 0.8900000000000000133, 0.8950000000000000178, 0.9000000000000000222, 0.9050000000000000266, 0.9100000000000000311, 0.9150000000000000355, 0.9200000000000000400, 0.9250000000000000444, 0.9300000000000000488, 0.9350000000000000533, 0.9399999999999999467, 0.9449999999999999512, 0.9499999999999999556, 0.9549999999999999600, 0.9599999999999999645, 0.9649999999999999689, 0.9699999999999999734, 0.9749999999999999778, 0.9799999999999999822, 0.9849999999999999867, 0.9899999999999999911, 0.9949999999999999956, 1.000000000000000000 ),
 .UNSPECIFIED. ) 
 GEOMETRIC_REPRESENTATION_ITEM ( )  RATIONAL_B_SPLINE_SURFACE ( (
 ( 1.000000000000000000, 0.9510565162951535312, 1.000000000000000000, 0.9510565162951535312, 1.000000000000000000, 0.9510565162951535312, 1.000000000000000000, 0.9510565162951535312, 1.000000000000000000, 0.9510565162951535312, 1.000000000000000000, 0.9510565162951535312, 1.000000000000000000, 0.9510565162951535312, 1.000000000000000000, 0.9510565162951535312, 1.000000000000000000, 0.9510565162951535312, 1.000000000000000000, 0.9510565162951535312, 1.000000000000000000, 0.9510565162951535312, 1.000000000000000000, 0.9510565162951535312, 1.000000000000000000, 0.9510565162951535312, 1.000000000000000000, 0.9510565162951535312, 1.000000000000000000, 0.9510565162951535312, 1.000000000000000000, 0.9510565162951535312, 1.000000000000000000, 0.9510565162951535312, 1.000000000000000000, 0.9510565162951535312, 1.000000000000000000, 0.9510565162951535312, 1.000000000000000000, 0.9510565162951535312, 1.000000000000000000, 0.9510565162951535312, 1.000000000000000000, 0.9510565162951535312, 1.000000000000000000, 0.9510565162951535312, 1.000000000000000000, 0.9510565162951535312, 1.000000000000000000, 0.9510565162951535312, 1.000000000000000000, 0.9510565162951535312, 1.000000000000000000, 0.9510565162951535312, 1.000000000000000000, 0.9510565162951535312, 1.000000000000000000, 0.9510565162951535312, 1.000000000000000000, 0.9510565162951535312, 1.000000000000000000, 0.9510565162951535312, 1.000000000000000000, 0.9510565162951535312, 1.000000000000000000, 0.9510565162951535312, 1.000000000000000000, 0.9510565162951535312, 1.000000000000000000, 0.9510565162951535312, 1.000000000000000000, 0.9510565162951535312, 1.000000000000000000, 0.9510565162951535312, 1.000000000000000000, 0.9510565162951535312, 1.000000000000000000, 0.9510565162951535312, 1.000000000000000000, 0.9510565162951535312, 1.000000000000000000, 0.9510565162951535312, 1.000000000000000000, 0.9510565162951535312, 1.000000000000000000, 0.9510565162951535312, 1.000000000000000000, 0.9510565162951535312, 1.000000000000000000, 0.9510565162951535312, 1.000000000000000000, 0.9510565162951535312, 1.000000000000000000, 0.9510565162951535312, 1.000000000000000000, 0.9510565162951535312, 1.000000000000000000, 0.9510565162951535312, 1.000000000000000000, 0.9510565162951535312, 1.000000000000000000, 0.9510565162951535312, 1.000000000000000000, 0.9510565162951535312, 1.000000000000000000, 0.9510565162951535312, 1.000000000000000000, 0.9510565162951535312, 1.000000000000000000, 0.9510565162951535312, 1.000000000000000000, 0.9510565162951535312, 1.000000000000000000, 0.9510565162951535312, 1.000000000000000000, 0.9510565162951535312, 1.000000000000000000, 0.9510565162951535312, 1.000000000000000000, 0.9510565162951535312, 1.000000000000000000, 0.9510565162951535312, 1.000000000000000000, 0.9510565162951535312, 1.000000000000000000, 0.9510565162951535312, 1.000000000000000000, 0.9510565162951535312, 1.000000000000000000, 0.9510565162951535312, 1.000000000000000000, 0.9510565162951535312, 1.000000000000000000, 0.9510565162951535312, 1.000000000000000000, 0.9510565162951535312, 1.000000000000000000, 0.9510565162951535312, 1.000000000000000000, 0.9510565162951535312, 1.000000000000000000, 0.9510565162951535312, 1.000000000000000000, 0.9510565162951535312, 1.000000000000000000, 0.9510565162951535312, 1.000000000000000000, 0.9510565162951535312, 1.000000000000000000, 0.9510565162951535312, 1.000000000000000000, 0.9510565162951535312, 1.000000000000000000, 0.9510565162951535312, 1.000000000000000000, 0.9510565162951535312, 1.000000000000000000, 0.9510565162951535312, 1.000000000000000000, 0.9510565162951535312, 1.000000000000000000, 0.9510565162951535312, 1.000000000000000000, 0.9510565162951535312, 1.000000000000000000, 0.9510565162951535312, 1.000000000000000000, 0.9510565162951535312, 1.000000000000000000, 0.9510565162951535312, 1.000000000000000000, 0.9510565162951535312, 1.000000000000000000, 0.9510565162951535312, 1.000000000000000000, 0.9510565162951535312, 1.000000000000000000, 0.9510565162951535312, 1.000000000000000000, 0.9510565162951535312, 1.000000000000000000, 0.9510565162951535312, 1.000000000000000000, 0.9510565162951535312, 1.000000000000000000, 0.9510565162951535312, 1.000000000000000000, 0.9510565162951535312, 1.000000000000000000, 0.9510565162951535312, 1.000000000000000000, 0.9510565162951535312, 1.000000000000000000, 0.9510565162951535312, 1.000000000000000000, 0.9510565162951535312, 1.000000000000000000, 0.9510565162951535312, 1.000000000000000000, 0.9510565162951535312, 1.000000000000000000, 0.9510565162951535312, 1.000000000000000000, 0.9510565162951535312, 1.000000000000000000, 0.9510565162951535312, 1.000000000000000000, 0.9510565162951535312, 1.000000000000000000, 0.9510565162951535312, 1.000000000000000000, 0.9510565162951535312, 1.000000000000000000, 0.9510565162951535312, 1.000000000000000000, 0.9510565162951535312, 1.000000000000000000, 0.9510565162951535312, 1.000000000000000000, 0.9510565162951535312, 1.000000000000000000, 0.9510565162951535312, 1.000000000000000000, 0.9510565162951535312, 1.000000000000000000, 0.9510565162951535312, 1.000000000000000000, 0.9510565162951535312, 1.000000000000000000, 0.9510565162951535312, 1.000000000000000000, 0.9510565162951535312, 1.000000000000000000, 0.9510565162951535312, 1.000000000000000000, 0.9510565162951535312, 1.000000000000000000, 0.9510565162951535312, 1.000000000000000000, 0.9510565162951535312, 1.000000000000000000, 0.9510565162951535312, 1.000000000000000000, 0.9510565162951535312, 1.000000000000000000, 0.9510565162951535312, 1.000000000000000000, 0.9510565162951535312, 1.000000000000000000, 0.9510565162951535312, 1.000000000000000000, 0.9510565162951535312, 1.000000000000000000, 0.9510565162951535312, 1.000000000000000000, 0.9510565162951535312, 1.000000000000000000, 0.9510565162951535312, 1.000000000000000000, 0.9510565162951535312, 1.000000000000000000, 0.9510565162951535312, 1.000000000000000000, 0.9510565162951535312, 1.000000000000000000, 0.9510565162951535312, 1.000000000000000000, 0.9510565162951535312, 1.000000000000000000, 0.9510565162951535312, 1.000000000000000000, 0.9510565162951535312, 1.000000000000000000, 0.9510565162951535312, 1.000000000000000000, 0.9510565162951535312, 1.000000000000000000, 0.9510565162951535312, 1.000000000000000000, 0.9510565162951535312, 1.000000000000000000, 0.9510565162951535312, 1.000000000000000000, 0.9510565162951535312, 1.000000000000000000, 0.9510565162951535312, 1.000000000000000000, 0.9510565162951535312, 1.000000000000000000, 0.9510565162951535312, 1.000000000000000000, 0.9510565162951535312, 1.000000000000000000, 0.9510565162951535312, 1.000000000000000000, 0.9510565162951535312, 1.000000000000000000, 0.9510565162951535312, 1.000000000000000000, 0.9510565162951535312, 1.000000000000000000, 0.9510565162951535312, 1.000000000000000000, 0.9510565162951535312, 1.000000000000000000, 0.9510565162951535312, 1.000000000000000000, 0.9510565162951535312, 1.000000000000000000, 0.9510565162951535312, 1.000000000000000000, 0.9510565162951535312, 1.000000000000000000, 0.9510565162951535312, 1.000000000000000000, 0.9510565162951535312, 1.000000000000000000, 0.9510565162951535312, 1.000000000000000000, 0.9510565162951535312, 1.000000000000000000, 0.9510565162951535312, 1.000000000000000000, 0.9510565162951535312, 1.000000000000000000, 0.9510565162951535312, 1.000000000000000000, 0.9510565162951535312, 1.000000000000000000, 0.9510565162951535312, 1.000000000000000000, 0.9510565162951535312, 1.000000000000000000, 0.9510565162951535312, 1.000000000000000000, 0.9510565162951535312, 1.000000000000000000, 0.9510565162951535312, 1.000000000000000000, 0.9510565162951535312, 1.000000000000000000, 0.9510565162951535312, 1.000000000000000000, 0.9510565162951535312, 1.000000000000000000, 0.9510565162951535312, 1.000000000000000000, 0.9510565162951535312, 1.000000000000000000, 0.9510565162951535312, 1.000000000000000000, 0.9510565162951535312, 1.000000000000000000, 0.9510565162951535312, 1.000000000000000000, 0.9510565162951535312, 1.000000000000000000, 0.9510565162951535312, 1.000000000000000000, 0.9510565162951535312, 1.000000000000000000, 0.9510565162951535312, 1.000000000000000000, 0.9510565162951535312, 1.000000000000000000, 0.9510565162951535312, 1.000000000000000000, 0.9510565162951535312, 1.000000000000000000, 0.9510565162951535312, 1.000000000000000000, 0.9510565162951535312, 1.000000000000000000, 0.9510565162951535312, 1.000000000000000000, 0.9510565162951535312, 1.000000000000000000, 0.9510565162951535312, 1.000000000000000000, 0.9510565162951535312, 1.000000000000000000, 0.9510565162951535312, 1.000000000000000000, 0.9510565162951535312, 1.000000000000000000, 0.9510565162951535312, 1.000000000000000000, 0.9510565162951535312, 1.000000000000000000, 0.9510565162951535312, 1.000000000000000000, 0.9510565162951535312, 1.000000000000000000, 0.9510565162951535312, 1.000000000000000000, 0.9510565162951535312, 1.000000000000000000, 0.9510565162951535312, 1.000000000000000000, 0.9510565162951535312, 1.000000000000000000),
 ( 1.000000000000000000, 0.9510565162951535312, 1.000000000000000000, 0.9510565162951535312, 1.000000000000000000, 0.9510565162951535312, 1.000000000000000000, 0.9510565162951535312, 1.000000000000000000, 0.9510565162951535312, 1.000000000000000000, 0.9510565162951535312, 1.000000000000000000, 0.9510565162951535312, 1.000000000000000000, 0.9510565162951535312, 1.000000000000000000, 0.9510565162951535312, 1.000000000000000000, 0.9510565162951535312, 1.000000000000000000, 0.9510565162951535312, 1.000000000000000000, 0.9510565162951535312, 1.000000000000000000, 0.9510565162951535312, 1.000000000000000000, 0.9510565162951535312, 1.000000000000000000, 0.9510565162951535312, 1.000000000000000000, 0.9510565162951535312, 1.000000000000000000, 0.9510565162951535312, 1.000000000000000000, 0.9510565162951535312, 1.000000000000000000, 0.9510565162951535312, 1.000000000000000000, 0.9510565162951535312, 1.000000000000000000, 0.9510565162951535312, 1.000000000000000000, 0.9510565162951535312, 1.000000000000000000, 0.9510565162951535312, 1.000000000000000000, 0.9510565162951535312, 1.000000000000000000, 0.9510565162951535312, 1.000000000000000000, 0.9510565162951535312, 1.000000000000000000, 0.9510565162951535312, 1.000000000000000000, 0.9510565162951535312, 1.000000000000000000, 0.9510565162951535312, 1.000000000000000000, 0.9510565162951535312, 1.000000000000000000, 0.9510565162951535312, 1.000000000000000000, 0.9510565162951535312, 1.000000000000000000, 0.9510565162951535312, 1.000000000000000000, 0.9510565162951535312, 1.000000000000000000, 0.9510565162951535312, 1.000000000000000000, 0.9510565162951535312, 1.000000000000000000, 0.9510565162951535312, 1.000000000000000000, 0.9510565162951535312, 1.000000000000000000, 0.9510565162951535312, 1.000000000000000000, 0.9510565162951535312, 1.000000000000000000, 0.9510565162951535312, 1.000000000000000000, 0.9510565162951535312, 1.000000000000000000, 0.9510565162951535312, 1.000000000000000000, 0.9510565162951535312, 1.000000000000000000, 0.9510565162951535312, 1.000000000000000000, 0.9510565162951535312, 1.000000000000000000, 0.9510565162951535312, 1.000000000000000000, 0.9510565162951535312, 1.000000000000000000, 0.9510565162951535312, 1.000000000000000000, 0.9510565162951535312, 1.000000000000000000, 0.9510565162951535312, 1.000000000000000000, 0.9510565162951535312, 1.000000000000000000, 0.9510565162951535312, 1.000000000000000000, 0.9510565162951535312, 1.000000000000000000, 0.9510565162951535312, 1.000000000000000000, 0.9510565162951535312, 1.000000000000000000, 0.9510565162951535312, 1.000000000000000000, 0.9510565162951535312, 1.000000000000000000, 0.9510565162951535312, 1.000000000000000000, 0.9510565162951535312, 1.000000000000000000, 0.9510565162951535312, 1.000000000000000000, 0.9510565162951535312, 1.000000000000000000, 0.9510565162951535312, 1.000000000000000000, 0.9510565162951535312, 1.000000000000000000, 0.9510565162951535312, 1.000000000000000000, 0.9510565162951535312, 1.000000000000000000, 0.9510565162951535312, 1.000000000000000000, 0.9510565162951535312, 1.000000000000000000, 0.9510565162951535312, 1.000000000000000000, 0.9510565162951535312, 1.000000000000000000, 0.9510565162951535312, 1.000000000000000000, 0.9510565162951535312, 1.000000000000000000, 0.9510565162951535312, 1.000000000000000000, 0.9510565162951535312, 1.000000000000000000, 0.9510565162951535312, 1.000000000000000000, 0.9510565162951535312, 1.000000000000000000, 0.9510565162951535312, 1.000000000000000000, 0.9510565162951535312, 1.000000000000000000, 0.9510565162951535312, 1.000000000000000000, 0.9510565162951535312, 1.000000000000000000, 0.9510565162951535312, 1.000000000000000000, 0.9510565162951535312, 1.000000000000000000, 0.9510565162951535312, 1.000000000000000000, 0.9510565162951535312, 1.000000000000000000, 0.9510565162951535312, 1.000000000000000000, 0.9510565162951535312, 1.000000000000000000, 0.9510565162951535312, 1.000000000000000000, 0.9510565162951535312, 1.000000000000000000, 0.9510565162951535312, 1.000000000000000000, 0.9510565162951535312, 1.000000000000000000, 0.9510565162951535312, 1.000000000000000000, 0.9510565162951535312, 1.000000000000000000, 0.9510565162951535312, 1.000000000000000000, 0.9510565162951535312, 1.000000000000000000, 0.9510565162951535312, 1.000000000000000000, 0.9510565162951535312, 1.000000000000000000, 0.9510565162951535312, 1.000000000000000000, 0.9510565162951535312, 1.000000000000000000, 0.9510565162951535312, 1.000000000000000000, 0.9510565162951535312, 1.000000000000000000, 0.9510565162951535312, 1.000000000000000000, 0.9510565162951535312, 1.000000000000000000, 0.9510565162951535312, 1.000000000000000000, 0.9510565162951535312, 1.000000000000000000, 0.9510565162951535312, 1.000000000000000000, 0.9510565162951535312, 1.000000000000000000, 0.9510565162951535312, 1.000000000000000000, 0.9510565162951535312, 1.000000000000000000, 0.9510565162951535312, 1.000000000000000000, 0.9510565162951535312, 1.000000000000000000, 0.9510565162951535312, 1.000000000000000000, 0.9510565162951535312, 1.000000000000000000, 0.9510565162951535312, 1.000000000000000000, 0.9510565162951535312, 1.000000000000000000, 0.9510565162951535312, 1.000000000000000000, 0.9510565162951535312, 1.000000000000000000, 0.9510565162951535312, 1.000000000000000000, 0.9510565162951535312, 1.000000000000000000, 0.9510565162951535312, 1.000000000000000000, 0.9510565162951535312, 1.000000000000000000, 0.9510565162951535312, 1.000000000000000000, 0.9510565162951535312, 1.000000000000000000, 0.9510565162951535312, 1.000000000000000000, 0.9510565162951535312, 1.000000000000000000, 0.9510565162951535312, 1.000000000000000000, 0.9510565162951535312, 1.000000000000000000, 0.9510565162951535312, 1.000000000000000000, 0.9510565162951535312, 1.000000000000000000, 0.9510565162951535312, 1.000000000000000000, 0.9510565162951535312, 1.000000000000000000, 0.9510565162951535312, 1.000000000000000000, 0.9510565162951535312, 1.000000000000000000, 0.9510565162951535312, 1.000000000000000000, 0.9510565162951535312, 1.000000000000000000, 0.9510565162951535312, 1.000000000000000000, 0.9510565162951535312, 1.000000000000000000, 0.9510565162951535312, 1.000000000000000000, 0.9510565162951535312, 1.000000000000000000, 0.9510565162951535312, 1.000000000000000000, 0.9510565162951535312, 1.000000000000000000, 0.9510565162951535312, 1.000000000000000000, 0.9510565162951535312, 1.000000000000000000, 0.9510565162951535312, 1.000000000000000000, 0.9510565162951535312, 1.000000000000000000, 0.9510565162951535312, 1.000000000000000000, 0.9510565162951535312, 1.000000000000000000, 0.9510565162951535312, 1.000000000000000000, 0.9510565162951535312, 1.000000000000000000, 0.9510565162951535312, 1.000000000000000000, 0.9510565162951535312, 1.000000000000000000, 0.9510565162951535312, 1.000000000000000000, 0.9510565162951535312, 1.000000000000000000, 0.9510565162951535312, 1.000000000000000000, 0.9510565162951535312, 1.000000000000000000, 0.9510565162951535312, 1.000000000000000000, 0.9510565162951535312, 1.000000000000000000, 0.9510565162951535312, 1.000000000000000000, 0.9510565162951535312, 1.000000000000000000, 0.9510565162951535312, 1.000000000000000000, 0.9510565162951535312, 1.000000000000000000, 0.9510565162951535312, 1.000000000000000000, 0.9510565162951535312, 1.000000000000000000, 0.9510565162951535312, 1.000000000000000000, 0.9510565162951535312, 1.000000000000000000, 0.9510565162951535312, 1.000000000000000000, 0.9510565162951535312, 1.000000000000000000, 0.9510565162951535312, 1.000000000000000000, 0.9510565162951535312, 1.000000000000000000, 0.9510565162951535312, 1.000000000000000000, 0.9510565162951535312, 1.000000000000000000, 0.9510565162951535312, 1.000000000000000000, 0.9510565162951535312, 1.000000000000000000, 0.9510565162951535312, 1.000000000000000000, 0.9510565162951535312, 1.000000000000000000, 0.9510565162951535312, 1.000000000000000000, 0.9510565162951535312, 1.000000000000000000, 0.9510565162951535312, 1.000000000000000000, 0.9510565162951535312, 1.000000000000000000, 0.9510565162951535312, 1.000000000000000000, 0.9510565162951535312, 1.000000000000000000, 0.9510565162951535312, 1.000000000000000000, 0.9510565162951535312, 1.000000000000000000, 0.9510565162951535312, 1.000000000000000000, 0.9510565162951535312, 1.000000000000000000, 0.9510565162951535312, 1.000000000000000000, 0.9510565162951535312, 1.000000000000000000, 0.9510565162951535312, 1.000000000000000000, 0.9510565162951535312, 1.000000000000000000, 0.9510565162951535312, 1.000000000000000000, 0.9510565162951535312, 1.000000000000000000, 0.9510565162951535312, 1.000000000000000000, 0.9510565162951535312, 1.000000000000000000, 0.9510565162951535312, 1.000000000000000000, 0.9510565162951535312, 1.000000000000000000, 0.9510565162951535312, 1.000000000000000000, 0.9510565162951535312, 1.000000000000000000, 0.9510565162951535312, 1.000000000000000000, 0.9510565162951535312, 1.000000000000000000, 0.9510565162951535312, 1.000000000000000000, 0.9510565162951535312, 1.000000000000000000) ) ) 
 REPRESENTATION_ITEM ( '' )  SURFACE ( )  );
#34216=CARTESIAN_POINT ( 'NONE',  ( 9.861089372814316079, 17.64441083166259006, -10.00000000000000533 ) ) ;
#34223=CARTESIAN_POINT ( 'NONE',  ( 78.93453705340030524, 60.10095773708777500, 16.11389061908799647 ) ) ;
#34227=CARTESIAN_POINT ( 'NONE',  ( 83.29773739198154203, 50.25459149593829267, -13.85366754400191525 ) ) ;
#34228=CARTESIAN_POINT ( 'NONE',  ( 73.37704433742356969, 70.12506801342537699, -9.398789138188929471 ) ) ;
#34229=CARTESIAN_POINT ( 'NONE',  ( 81.27906948385655994, 42.22991039144485370, -7.243114465301290217 ) ) ;
#34230=ORIENTED_EDGE ( 'NONE', *, *, #38751, .T. ) ;
#34231=EDGE_LOOP ( 'NONE', ( #65721, #34606, #55479, #91176 ) ) ;
#34240=CARTESIAN_POINT ( 'NONE',  ( 82.17778236580524265, 40.63545381150629510, 3.437353603792591805 ) ) ;
#34241=PLANE ( 'NONE',  #78043 ) ;
#34245=CARTESIAN_POINT ( 'NONE',  ( 87.17876410986579572, 43.10751584725982610, -0.2475519180087527027 ) ) ;
#34248=CARTESIAN_POINT ( 'NONE',  ( 70.75845742388486315, 61.42534300271167069, -14.83394790560162413 ) ) ;
#34250=ADVANCED_FACE ( 'NONE', ( #45669 ), #78099, .T. ) ;
#34251=CARTESIAN_POINT ( 'NONE',  ( 85.58533047404948491, 48.36141062822003533, -12.20656690058574689 ) ) ;
#34254=ADVANCED_FACE ( 'NONE', ( #69974 ), #33542, .T. ) ;
#34255=CARTESIAN_POINT ( 'NONE',  ( 76.26495795533084276, 64.90087152775714685, -14.31572824905659935 ) ) ;
#34262=CARTESIAN_POINT ( 'NONE',  ( 88.19053702688614749, 44.32527345396093921, -2.493626234014362009 ) ) ;
#34263=ORIENTED_EDGE ( 'NONE', *, *, #29795, .T. ) ;
#34265=CARTESIAN_POINT ( 'NONE',  ( 65.97951220193175459, 68.67161866859687791, -0.1777484692489773310 ) ) ;
#34268=EDGE_CURVE ( 'NONE', #48220, #41092, #83298, .T. ) ;
#34271=CARTESIAN_POINT ( 'NONE',  ( 81.33896983113768897, 44.83237125196090034, -10.57384344836858325 ) ) ;
#34274=CARTESIAN_POINT ( 'NONE',  ( 88.28217478145764119, 43.95791727297697804, 2.470383038495642669 ) ) ;
#34278=CARTESIAN_POINT ( 'NONE',  ( 80.12217583349386985, 58.13818462438354828, 16.26693196410659326 ) ) ;
#34283=CARTESIAN_POINT ( 'NONE',  ( 80.85183824906197003, 42.96989659668948747, -9.583637002236184088 ) ) ;
#34293=CARTESIAN_POINT ( 'NONE',  ( 77.55539304566268299, 52.43243923690647534, 15.72493065762432174 ) ) ;
#34300=CARTESIAN_POINT ( 'NONE',  ( 80.95010002000924487, 53.96101425250913763, -15.71262299032070331 ) ) ;
#34303=CARTESIAN_POINT ( 'NONE',  ( 75.37662461738884190, 53.50075842301595230, 16.04033158989234309 ) ) ;
#34306=CARTESIAN_POINT ( 'NONE',  ( 72.47345658542111835, 57.49201715091417952, 15.81387984723518159 ) ) ;
#34313=CARTESIAN_POINT ( 'NONE',  ( 35.77386594998528579, 21.44966523072496756, -2.296566073217252530E-15 ) ) ;
#34314=CARTESIAN_POINT ( 'NONE',  ( 79.77267820561851863, 49.16024335904899090, -14.73473614307763846 ) ) ;
#34315=CARTESIAN_POINT ( 'NONE',  ( 74.32283972735670829, 55.33658384534070507, 16.60204640374922036 ) ) ;
#34317=CARTESIAN_POINT ( 'NONE',  ( 21.54279312762077936, 14.29860640527291871, -2.839279412974138328 ) ) ;
#34324=CARTESIAN_POINT ( 'NONE',  ( 86.30241807085522510, 47.23217017718856425, 10.82197119102028893 ) ) ;
#34329=B_SPLINE_CURVE_WITH_KNOTS ( 'NONE', 3,
 ( #10011, #40875, #3425, #89076, #88065, #80956, #71820, #34300, #18614, #64197, #78930, #65200, #26208, #3904, #27207, #58093, #96142, #49493, #32794, #56593, #18107, #26702, #49008, #1911, #79942, #10503, #57585, #41385, #72328, #2931, #25192, #63701, #11522, #50001, #33820, #88563, #19626, #95659, #64708, #57085, #19127, #42380, #73312, #9519, #40379, #94637 ),
 .UNSPECIFIED., .F., .F.,
 ( 4, 1, 2, 2, 1, 2, 2, 1, 1, 2, 2, 1, 1, 2, 2, 1, 1, 2, 2, 1, 1, 1, 2, 2, 1, 1, 1, 2, 2, 4 ),
 ( 0.000000000000000000, 0.06250000000000385803, 0.09375000000000578704, 0.1250000000000077161, 0.1875000000000154876, 0.2187500000000190681, 0.2500000000000226485, 0.3125000000000335287, 0.3437500000000370259, 0.3593750000000391354, 0.3750000000000411893, 0.4375000000000595080, 0.4687500000000667244, 0.4843750000000707767, 0.5000000000000747180, 0.5625000000000771605, 0.5937500000000761613, 0.6093750000000776046, 0.6250000000000790479, 0.6875000000000812683, 0.7187500000000821565, 0.7343750000000806022, 0.7421875000000799361, 0.7500000000000791589, 0.8125000000000575096, 0.8437500000000466294, 0.8593750000000411893, 0.8671875000000386358, 0.8750000000000360822, 1.000000000000000000 ),
 .UNSPECIFIED. ) ;
#34330=CARTESIAN_POINT ( 'NONE',  ( 74.74299343307386323, 53.49955268462365865, 16.07385381711848638 ) ) ;
#34333=ORIENTED_EDGE ( 'NONE', *, *, #83301, .F. ) ;
#34346=CARTESIAN_POINT ( 'NONE',  ( 24.92213970864663963, 37.49540643055189548, 3.479690158560446702E-15 ) ) ;
#34347=CARTESIAN_POINT ( 'NONE',  ( 83.02699437693422624, 48.37159093816767808, -12.75497678487218600 ) ) ;
#34348=DIRECTION ( 'NONE',  ( 0.8116583814955277143, 0.01378320505840788246, -0.5839697723396121143 ) ) ;
#34355=CARTESIAN_POINT ( 'NONE',  ( 85.56715572150820037, 48.66046822832736041, 12.44852408270450184 ) ) ;
#34365=CARTESIAN_POINT ( 'NONE',  ( 73.91024718746507460, 55.00110737226054880, -16.60404657609226575 ) ) ;
#34370=CARTESIAN_POINT ( 'NONE',  ( 87.18059948837544937, 46.13477641244298155, -8.300795534149866484 ) ) ;
#34372=B_SPLINE_SURFACE_WITH_KNOTS ( 'NONE', 3, 1, ( 
 ( #27930, #82190 ),
 ( #57333, #43626 ),
 ( #28425, #11270 ),
 ( #90287, #20856 ),
 ( #78787, #40253 ),
 ( #34063, #64954 ),
 ( #88307, #45122 ),
 ( #68420, #99347 ),
 ( #91760, #52222 ),
 ( #29431, #84663 ),
 ( #14727, #30923 ),
 ( #83167, #44116 ),
 ( #51748, #7118 ),
 ( #60307, #92758 ),
 ( #45608, #21828 ),
 ( #67423, #84178 ),
 ( #76540, #82690 ),
 ( #98355, #13256 ),
 ( #28943, #44608 ),
 ( #98855, #38003 ),
 ( #60801, #61808 ),
 ( #38512, #91264 ),
 ( #75053, #83672 ),
 ( #52714, #77017 ),
 ( #5629, #68916 ),
 ( #59820, #6638 ),
 ( #69424, #37 ),
 ( #22325, #36523 ),
 ( #75543, #99841 ),
 ( #67934, #90786 ),
 ( #53226, #30425 ) ),
 .UNSPECIFIED., .F., .F., .F.,
 ( 4, 3, 3, 3, 3, 3, 3, 3, 3, 3, 4 ),
 ( 2, 2 ),
 ( 0.000000000000000000, 0.1122669598086788734, 0.2243161639709606303, 0.3396355846219134000, 0.4553962076585122976, 0.5677860799922305191, 0.6749047109689531032, 0.7773884377078198460, 0.8775581155834139002, 0.9782364162377853445, 1.000000000000000000 ),
 ( 0.000000000000000000, 1.000000000000000000 ),
 .UNSPECIFIED. ) ;
#34373=CARTESIAN_POINT ( 'NONE',  ( 30.93718178480143521, 33.56454794089042082, 10.00000000000000355 ) ) ;
#34383=CARTESIAN_POINT ( 'NONE',  ( 75.72636783681542738, 65.12249353091223725, -14.45027308884206718 ) ) ;
#34387=CARTESIAN_POINT ( 'NONE',  ( 69.45603412936870313, 62.99601925590414453, -13.63678823767287973 ) ) ;
#34396=EDGE_CURVE ( 'NONE', #26854, #44175, #39625, .T. ) ;
#34397=DIRECTION ( 'NONE',  ( -0.3782958374750524655, 0.000000000000000000, -0.9256847516023197775 ) ) ;
#34400=CARTESIAN_POINT ( 'NONE',  ( 78.86219776201926379, 59.55369065033507070, 16.50996775951928086 ) ) ;
#34406=CARTESIAN_POINT ( 'NONE',  ( 34.54807858326547176, 25.11029122506296929, -8.090169943749478065 ) ) ;
#34407=CARTESIAN_POINT ( 'NONE',  ( 72.12429762571967728, 64.53244924666101667, -13.11970522421019503 ) ) ;
#34409=CARTESIAN_POINT ( 'NONE',  ( 74.25393038840245197, 55.45593832152543712, 16.12141555578006447 ) ) ;
#34411=CARTESIAN_POINT ( 'NONE',  ( 35.14347105191519205, 25.45404122711135741, -8.090169943749478065 ) ) ;
#34416=CARTESIAN_POINT ( 'NONE',  ( 87.39545338979795019, 43.86517562418462290, -2.489615843231432368 ) ) ;
#34419=CARTESIAN_POINT ( 'NONE',  ( 83.03097277809888510, 51.42467778882387819, 14.50400025335057208 ) ) ;
#34422=CARTESIAN_POINT ( 'NONE',  ( 87.25346308258933448, 46.04525953206349698, 8.773708642049088624 ) ) ;
#34423=EDGE_CURVE ( 'NONE', #92377, #25562, #95722, .T. ) ;
#34425=CARTESIAN_POINT ( 'NONE',  ( 81.92146693744936670, 41.17928938369797009, 5.561051477722002367 ) ) ;
#34429=CARTESIAN_POINT ( 'NONE',  ( 40.24855657362158468, 31.43677371833804912, -10.00000000000000355 ) ) ;
#34433=CARTESIAN_POINT ( 'NONE',  ( 5.618660645053492608, 25.01751292744054211, 6.180339887498949913 ) ) ;
#34438=CARTESIAN_POINT ( 'NONE',  ( 83.98894966577088894, 51.79070771454841804, 14.82098776213804392 ) ) ;
#34446=CARTESIAN_POINT ( 'NONE',  ( 67.00965166525888606, 66.88736477923252721, -8.820170631815919648 ) ) ;
#34452=CARTESIAN_POINT ( 'NONE',  ( 26.56877070717806788, 23.84335787977763843, 9.188101187500006262 ) ) ;
#34453=CARTESIAN_POINT ( 'NONE',  ( 73.09359486087168989, 70.66713452829003472, -7.730905117165903562 ) ) ;
#34456=VERTEX_POINT ( 'NONE', #48571 ) ;
#34457=CARTESIAN_POINT ( 'NONE',  ( 13.54711677929152636, 28.79752408145591858, -5.678558825948271327 ) ) ;
#34458=CARTESIAN_POINT ( 'NONE',  ( 76.08054936894747300, 60.44165029396862820, 15.72172349425854065 ) ) ;
#34460=CARTESIAN_POINT ( 'NONE',  ( 13.42817895373461390, 26.49103043416548076, -8.090169943749479842 ) ) ;
#34462=CARTESIAN_POINT ( 'NONE',  ( 71.96639307748559133, 71.49757472301891426, -5.734781593071442529 ) ) ;
#34465=CARTESIAN_POINT ( 'NONE',  ( 74.73869185334548604, 64.10010416581232562, -14.66605532835945880 ) ) ;
#34466=VERTEX_POINT ( 'NONE', #87140 ) ;
#34471=CARTESIAN_POINT ( 'NONE',  ( 66.17812102814201580, 68.61244640036318287, -2.189447319278969406 ) ) ;
#34474=CARTESIAN_POINT ( 'NONE',  ( 78.08890065365325484, 61.45839965263433413, -16.15943835942215756 ) ) ;
#34475=EDGE_CURVE ( 'NONE', #33229, #26719, #25258, .T. ) ;
#34482=CARTESIAN_POINT ( 'NONE',  ( 38.16387531507685793, 24.96004757982092315, -5.678558825948276656 ) ) ;
#34494=ORIENTED_EDGE ( 'NONE', *, *, #51324, .F. ) ;
#34495=CARTESIAN_POINT ( 'NONE',  ( 72.19109158906036328, 71.10838548458626462, -5.953967166465967686 ) ) ;
#34498=CARTESIAN_POINT ( 'NONE',  ( 84.14312167556933275, 48.98415679381830756, 0.000000000000000000 ) ) ;
#34516=CARTESIAN_POINT ( 'NONE',  ( 74.14611568627913130, 58.01609043150301659, 15.90920405299479157 ) ) ;
#34518=ORIENTED_EDGE ( 'NONE', *, *, #5142, .T. ) ;
#34519=CARTESIAN_POINT ( 'NONE',  ( 80.26984573713558291, 57.41310870600725025, -16.58958131739138508 ) ) ;
#34529=CARTESIAN_POINT ( 'NONE',  ( 14.87430715154758687, 30.36126292948894800, 6.180339887498949913 ) ) ;
#34533=B_SPLINE_CURVE_WITH_KNOTS ( 'NONE', 3,
 ( #55765, #31481, #14795, #45677, #76603, #88259, #33503, #88757, #32990, #49210, #79142, #18311, #11711, #71518, #48712, #18807, #10209, #25394, #26407, #42088, #40578, #80142, #2108, #87773, #64398, #94830, #95362, #72525, #3613, #56788, #63893, #73020, #56281, #10707, #87280, #49689, #26903, #86757, #17291, #27405, #57285, #80644, #11222, #17811, #42573, #79643 ),
 .UNSPECIFIED., .F., .F.,
 ( 4, 1, 1, 1, 2, 2, 1, 1, 1, 2, 2, 1, 1, 2, 2, 1, 1, 2, 2, 1, 1, 2, 2, 1, 2, 2, 1, 2, 2, 4 ),
 ( 0.000000000000000000, 0.06249999999998676059, 0.09374999999998205602, 0.1093749999999796968, 0.1171874999999787531, 0.1249999999999777955, 0.1874999999999881206, 0.2187499999999913958, 0.2343749999999911460, 0.2421874999999893974, 0.2499999999999876210, 0.3124999999999739098, 0.3437499999999689138, 0.3593749999999641953, 0.3749999999999594213, 0.4374999999999457656, 0.4687499999999393263, 0.4843749999999361622, 0.4999999999999329425, 0.5624999999999296119, 0.5937499999999259481, 0.6093749999999263922, 0.6249999999999268363, 0.6874999999999357181, 0.7187499999999398259, 0.7499999999999438227, 0.8124999999999519273, 0.8437499999999579225, 0.8749999999999639178, 1.000000000000000000 ),
 .UNSPECIFIED. ) ;
#34545=CARTESIAN_POINT ( 'NONE',  ( 21.91939736263385541, 14.78380873178786636, -6.180339887498949025 ) ) ;
#34547=CARTESIAN_POINT ( 'NONE',  ( 69.03518170984699509, 64.49507618471645287, 12.45339560606362461 ) ) ;
#34548=CARTESIAN_POINT ( 'NONE',  ( 72.08021828965947009, 72.40975849880194914, -3.082927075499598324 ) ) ;
#34550=CARTESIAN_POINT ( 'NONE',  ( 73.83283565865448850, 55.23351700259583197, -16.12091336794239638 ) ) ;
#34553=CARTESIAN_POINT ( 'NONE',  ( 74.58922631747108767, 66.95469429158355013, 12.55546573254311937 ) ) ;
#34554=CARTESIAN_POINT ( 'NONE',  ( 23.75126848931443746, 37.21091486745861943, 7.012934429366973338E-14 ) ) ;
#34555=FACE_OUTER_BOUND ( 'NONE', #22119, .T. ) ;
#34561=CARTESIAN_POINT ( 'NONE',  ( 39.87427548755113804, 25.94754757982092741, 5.678558825948272215 ) ) ;
#34564=CARTESIAN_POINT ( 'NONE',  ( 40.97001837269192492, 24.44966523072497822, -2.296566073217252530E-15 ) ) ;
#34565=CARTESIAN_POINT ( 'NONE',  ( 26.76913962382671386, 17.58380873178787951, 6.180339887498953466 ) ) ;
#34571=CARTESIAN_POINT ( 'NONE',  ( 14.66449673273962340, 9.262165230724928477, -2.296566073217252530E-15 ) ) ;
#34572=CARTESIAN_POINT ( 'NONE',  ( 71.97141114645216931, 72.59821799906345063, 1.534520970786794836 ) ) ;
#34573=CARTESIAN_POINT ( 'NONE',  ( 20.18540868186541459, 12.44966523072493914, -2.296566073217252530E-15 ) ) ;
#34574=CIRCLE ( 'NONE', #60362, 16.10714546451156082 ) ;
#34582=CARTESIAN_POINT ( 'NONE',  ( 29.46552898026456546, 17.41603393254326093, -1.583844403245362020 ) ) ;
#34583=CARTESIAN_POINT ( 'NONE',  ( 87.83187315495058556, 45.09740525803774602, 6.666720864128770074 ) ) ;
#34591=CARTESIAN_POINT ( 'NONE',  ( 76.62142590937760644, 52.12176499430435683, 15.74697333657635134 ) ) ;
#34595=CARTESIAN_POINT ( 'NONE',  ( 77.61054570139664577, 50.60100434898155441, -15.24042138154272763 ) ) ;
#34606=ORIENTED_EDGE ( 'NONE', *, *, #6611, .F. ) ;
#34614=CARTESIAN_POINT ( 'NONE',  ( 70.06962527880796188, 66.55497806833156460, 10.52730242420649631 ) ) ;
#34620=CARTESIAN_POINT ( 'NONE',  ( 27.26159103020561147, 24.24335787977764767, -9.188101187500008038 ) ) ;
#34624=EDGE_LOOP ( 'NONE', ( #20276, #86415, #99647, #59263 ) ) ;
#34627=CARTESIAN_POINT ( 'NONE',  ( 69.71681968175923316, 62.66721131071562212, 13.91613743701406491 ) ) ;
#34629=CARTESIAN_POINT ( 'NONE',  ( 18.87072174683323666, 11.86426979415088745, -3.090169943749474069 ) ) ;
#34630=EDGE_CURVE ( 'NONE', #17546, #2384, #14182, .T. ) ;
#34651=CARTESIAN_POINT ( 'NONE',  ( 79.58119954245727001, 47.14750477878121160, -13.19237880149493769 ) ) ;
#34657=CARTESIAN_POINT ( 'NONE',  ( 74.17426598413138095, 67.86558882176393581, -11.66684587328573031 ) ) ;
#34661=CARTESIAN_POINT ( 'NONE',  ( 79.04869528564928771, 60.22382082520469737, -16.44980649040590492 ) ) ;
#34665=CARTESIAN_POINT ( 'NONE',  ( 68.60506951895222016, 64.61196645306745268, -12.16704851705999957 ) ) ;
#34667=CARTESIAN_POINT ( 'NONE',  ( 80.77040970686135779, 52.39315937341162055, 15.73168746087837810 ) ) ;
#34678=CARTESIAN_POINT ( 'NONE',  ( 16.80672687576512203, 25.10171378149917842, 9.188101187500008038 ) ) ;
#34679=CARTESIAN_POINT ( 'NONE',  ( 75.28650001057752661, 66.67572118895705557, 13.44401380721711270 ) ) ;
#34683=CARTESIAN_POINT ( 'NONE',  ( 15.34872451668155868, 24.56454794089041016, 10.00000000000000355 ) ) ;
#34690=CARTESIAN_POINT ( 'NONE',  ( 81.78242120570297402, 55.48469546634665761, -15.94821833579707437 ) ) ;
#34692=DIRECTION ( 'NONE',  ( 0.1039558454088763267, -0.1800568059919503139, 0.9781476007338069101 ) ) ;
#34694=CARTESIAN_POINT ( 'NONE',  ( 82.53715491520738112, 41.41892551179127935, 3.500865685413612205 ) ) ;
#34695=CARTESIAN_POINT ( 'NONE',  ( 80.15082809947642772, 54.47608182991538683, 15.87478864171170123 ) ) ;
#34701=CARTESIAN_POINT ( 'NONE',  ( 4.150881819241740267, 21.13478043621385538, 8.090169943749478065 ) ) ;
#34709=CARTESIAN_POINT ( 'NONE',  ( 78.89591602029014439, 59.68745106357756924, 16.49891905133565473 ) ) ;
#34711=CARTESIAN_POINT ( 'NONE',  ( 75.15191903148871688, 52.97183600646508239, -16.48001256418180915 ) ) ;
#34713=ORIENTED_EDGE ( 'NONE', *, *, #55837, .T. ) ;
#34715=CARTESIAN_POINT ( 'NONE',  ( 82.76821771688562990, 50.44192209291004048, -14.09389759779402063 ) ) ;
#34716=CARTESIAN_POINT ( 'NONE',  ( 73.46468938206548671, 69.84266834477836028, -9.805732075891272714 ) ) ;
#34717=CARTESIAN_POINT ( 'NONE',  ( 84.65536491870415148, 49.91664468313385328, -13.65730316586987669 ) ) ;
#34722=ORIENTED_EDGE ( 'NONE', *, *, #22284, .F. ) ;
#34726=CARTESIAN_POINT ( 'NONE',  ( 75.80447387303706819, 62.76703707744994887, 15.01739634675713830 ) ) ;
#34736=CARTESIAN_POINT ( 'NONE',  ( 75.66673835297086725, 54.72918191672597743, 16.12085908788240474 ) ) ;
#34738=CARTESIAN_POINT ( 'NONE',  ( 10.59299460361177125, 21.51421378149917274, -9.188101187500004485 ) ) ;
#34744=CARTESIAN_POINT ( 'NONE',  ( 76.04051017601332774, 65.42867741054584485, -13.97686685444981336 ) ) ;
#34748=CARTESIAN_POINT ( 'NONE',  ( 86.90457605785044848, 44.29542909698827202, 4.965724379175460612 ) ) ;
#34749=CARTESIAN_POINT ( 'NONE',  ( 88.44601041138486153, 44.07807065378580802, -2.614235559790803798 ) ) ;
#34752=CARTESIAN_POINT ( 'NONE',  ( 65.92267706577344200, 69.18571671596606620, 0.2487269089564623503 ) ) ;
#34758=CARTESIAN_POINT ( 'NONE',  ( 45.00959873851216031, 26.39040679176986970, 1.333680081654574804E-15 ) ) ;
#34761=CARTESIAN_POINT ( 'NONE',  ( 88.29163947745264807, 44.34544895456824065, 2.315384907525153135 ) ) ;
#34765=B_SPLINE_CURVE_WITH_KNOTS ( 'NONE', 3,
 ( #91812, #38050, #77591, #9696, #39047, #8178, #93304, #8673, #86230, #24376, #85214, #31957, #77065, #69959, #61854, #54752, #62860, #68963, #15759, #46148, #93817, #55248, #16765, #78084, #92803, #39543, #23861, #31458, #16267, #1079, #54241, #574, #24866, #30470, #47656, #85738, #47160, #7673, #69468, #79114, #70465, #46664, #78591, #9176, #40050, #70990 ),
 .UNSPECIFIED., .F., .F.,
 ( 4, 1, 2, 2, 1, 2, 2, 1, 1, 2, 2, 1, 1, 2, 2, 1, 1, 2, 2, 1, 1, 1, 2, 2, 1, 1, 1, 2, 2, 4 ),
 ( 0.007499696492506968508, 0.06953096546172284065, 0.1005465999463296539, 0.1315622344309364811, 0.1935935034001495803, 0.2246091378847561715, 0.2556247723693627072, 0.3176560413385787207, 0.3486716758231865332, 0.3641794930654918550, 0.3796873103077972322, 0.4417185792770212394, 0.4727342137616331597, 0.4882420310039392031, 0.5037498482462451355, 0.5657811172154665336, 0.5967967517000785094, 0.6123045689423857185, 0.6278123861846929277, 0.6898436551539256500, 0.7208592896385420667, 0.7363671068808488318, 0.7441210155020008266, 0.7518749241231527103, 0.8139061930923631172, 0.8449218275769683206, 0.8604296448192708668, 0.8681835534404220844, 0.8759374620615733020, 1.000000000000000000 ),
 .UNSPECIFIED. ) ;
#34766=LINE ( 'NONE', #48986, #32218 ) ;
#34768=CARTESIAN_POINT ( 'NONE',  ( 72.01549410641601412, 65.88731131220951909, -12.15293914534650277 ) ) ;
#34770=CARTESIAN_POINT ( 'NONE',  ( 80.76710472214251979, 43.07881916343166750, -9.774221331374631561 ) ) ;
#34777=DIRECTION ( 'NONE',  ( 0.5000000000000014433, -0.8660254037844378194, 0.000000000000000000 ) ) ;
#34778=CARTESIAN_POINT ( 'NONE',  ( 77.27856866401023694, 51.25232217808265034, 15.47710953478911655 ) ) ;
#34783=CARTESIAN_POINT ( 'NONE',  ( 85.01541621076924571, 50.02003410940323391, 13.59443226853714926 ) ) ;
#34785=CARTESIAN_POINT ( 'NONE',  ( 79.19548319422065674, 46.07689622240576455, -13.22575811200356810 ) ) ;
#34791=DIRECTION ( 'NONE',  ( -0.8660254037844379305, -0.5000000000000014433, -0.000000000000000000 ) ) ;
#34794=CARTESIAN_POINT ( 'NONE',  ( 76.03019726450892790, 65.44783958900880805, 14.37600347258595690 ) ) ;
#34797=CARTESIAN_POINT ( 'NONE',  ( 34.67812306484451312, 22.94754757982092030, 5.678558825948272215 ) ) ;
#34798=CARTESIAN_POINT ( 'NONE',  ( 79.57665710957374472, 49.21012782547803965, -14.80730596066503679 ) ) ;
#34799=CARTESIAN_POINT ( 'NONE',  ( 74.71948287562122459, 57.03696899136454590, 16.52214785348690285 ) ) ;
#34800=ORIENTED_EDGE ( 'NONE', *, *, #1818, .T. ) ;
#34801=CARTESIAN_POINT ( 'NONE',  ( 20.04711164229383513, 17.28920272979926764, -7.433330006724141015 ) ) ;
#34806=CARTESIAN_POINT ( 'NONE',  ( 86.11363163537949106, 47.05074959952599301, 10.74854466831323840 ) ) ;
#34809=CARTESIAN_POINT ( 'NONE',  ( 87.38898754588738882, 44.84176836479306871, -6.666552467508535251 ) ) ;
#34812=CARTESIAN_POINT ( 'NONE',  ( 74.82756539338009816, 53.47993334157433765, 16.54385625414931837 ) ) ;
#34813=EDGE_LOOP ( 'NONE', ( #34957, #25643, #53028, #67841 ) ) ;
#34814=CARTESIAN_POINT ( 'NONE',  ( 85.50503765007894685, 46.43143530048178036, 9.878743384447044917 ) ) ;
#34823=CARTESIAN_POINT ( 'NONE',  ( 3.011046308360212809, 25.23654200823200355, 1.583844403245364241 ) ) ;
#34828=CARTESIAN_POINT ( 'NONE',  ( 29.04415360562664361, 34.95586893147757479, 7.433330006724141015 ) ) ;
#34829=CARTESIAN_POINT ( 'NONE',  ( 76.29760026105621762, 59.55922990308604170, -15.89113754366026576 ) ) ;
#34830=CARTESIAN_POINT ( 'NONE',  ( 74.25393038840245197, 55.45593832152543712, 16.12141555578006091 ) ) ;
#34831=EDGE_CURVE ( 'NONE', #19903, #67514, #25940, .T. ) ;
#34833=ORIENTED_EDGE ( 'NONE', *, *, #46245, .F. ) ;
#34836=CARTESIAN_POINT ( 'NONE',  ( 68.33081780576208075, 65.63013816376739840, 10.40955482511126107 ) ) ;
#34838=CARTESIAN_POINT ( 'NONE',  ( 85.51062282364698319, 48.96702101389664108, -12.23238128493630583 ) ) ;
#34841=CARTESIAN_POINT ( 'NONE',  ( 70.47590555702623760, 60.94424470842204755, 14.96950124546868111 ) ) ;
#34846=VERTEX_POINT ( 'NONE', #74765 ) ;
#34852=CARTESIAN_POINT ( 'NONE',  ( 87.23676543452685905, 46.07418070687454303, -8.827152287545313669 ) ) ;
#34858=ORIENTED_EDGE ( 'NONE', *, *, #55939, .T. ) ;
#34869=CARTESIAN_POINT ( 'NONE',  ( 71.39421488629903934, 69.39266753417868472, -8.110451711237608663 ) ) ;
#34871=CARTESIAN_POINT ( 'NONE',  ( 69.79245252017108214, 62.76958509742000558, -13.30825049901474344 ) ) ;
#34876=EDGE_CURVE ( 'NONE', #77470, #10592, #896, .T. ) ;
#34877=CARTESIAN_POINT ( 'NONE',  ( 81.53053605624106126, 48.05823170493817287, 13.08105315416342052 ) ) ;
#34878=CARTESIAN_POINT ( 'NONE',  ( 81.95798892854801920, 41.01614721200600400, -3.218282653241920865 ) ) ;
#34879=ADVANCED_FACE ( 'NONE', ( #84861 ), #39110, .T. ) ;
#34883=CARTESIAN_POINT ( 'NONE',  ( 82.63281508726200286, 40.94328431233920895, -3.617117793111280122 ) ) ;
#34886=B_SPLINE_CURVE_WITH_KNOTS ( 'NONE', 3,
 ( #28310, #3549, #50609, #97742, #49622, #74451, #51624, #81563, #88189, #42995, #82576, #33950, #57214, #42505, #95784, #26338, #50127, #65327, #4519, #96266, #11645, #66325, #88690, #34911, #35913, #97257, #27824, #58700, #89674, #20235, #51107 ),
 .UNSPECIFIED., .F., .F.,
 ( 4, 3, 3, 3, 3, 3, 3, 3, 3, 3, 4 ),
 ( 0.000000000000000000, 0.1333490885032313222, 0.3007194338854242699, 0.4699862290244929963, 0.5844252810809240639, 0.6686540514502682386, 0.7354980260655500368, 0.8028463152565734617, 0.8633854507757154906, 0.9437142632667211428, 1.000000000000000000 ),
 .UNSPECIFIED. ) ;
#34887=CARTESIAN_POINT ( 'NONE',  ( 70.46185687578375223, 70.52818721896052523, -4.697131730717588383 ) ) ;
#34889=CARTESIAN_POINT ( 'NONE',  ( 83.20726942458908582, 52.32534163598141674, 14.85174634631042423 ) ) ;
#34895=CARTESIAN_POINT ( 'NONE',  ( 40.66614990564659138, 23.28848085856234817, 1.475505719884397138E-15 ) ) ;
#34898=CARTESIAN_POINT ( 'NONE',  ( 71.70501702668993005, 58.75402291411430156, -15.44053495759504457 ) ) ;
#34904=CARTESIAN_POINT ( 'NONE',  ( 86.54292033101232562, 46.25028892199807729, 8.970843135639706034 ) ) ;
#34907=CARTESIAN_POINT ( 'NONE',  ( 82.16658848853110442, 41.26547592452066482, 5.424318534973775030 ) ) ;
#34909=B_SPLINE_CURVE_WITH_KNOTS ( 'NONE', 3,
 ( #92473, #93476, #30136, #47326, #22542, #100056, #238, #77235, #23515, #39210, #91990, #7842, #30643, #31615, #53428, #1241, #31120, #729, #84377, #62511, #14924, #45813, #8831, #62010, #85905, #92962, #85383, #46834, #78252, #8340, #24028, #54927, #16430, #39700, #70631, #32124, #82224, #51260, #90820, #60340, #52746, #83707, #21862, #68947, #97889, #84212 ),
 .UNSPECIFIED., .F., .F.,
 ( 4, 1, 1, 1, 2, 2, 1, 1, 1, 2, 2, 1, 1, 2, 2, 1, 1, 2, 2, 1, 1, 2, 2, 1, 2, 2, 1, 2, 2, 4 ),
 ( 0.000000000000000000, 0.06249999999998029354, 0.09374999999997030153, 0.1093749999999655692, 0.1171874999999649586, 0.1249999999999643618, 0.1874999999999631128, 0.2187499999999606426, 0.2343749999999612532, 0.2421874999999597267, 0.2499999999999581446, 0.3124999999999589773, 0.3437499999999574229, 0.3593749999999568678, 0.3749999999999562572, 0.4374999999999509837, 0.4687499999999500955, 0.4843749999999513722, 0.4999999999999525935, 0.5624999999999675815, 0.5937499999999736877, 0.6093749999999763522, 0.6249999999999791278, 0.6874999999999837907, 0.7187499999999863443, 0.7499999999999887867, 0.8124999999999932276, 0.8437499999999955591, 0.8749999999999977796, 1.000000000000000000 ),
 .UNSPECIFIED. ) ;
#34911=CARTESIAN_POINT ( 'NONE',  ( 86.88058850597731464, 45.96296635460476665, 8.956153083123110648 ) ) ;
#34913=CARTESIAN_POINT ( 'NONE',  ( 35.94483945213000453, 39.49103043416551628, -8.090169943749479842 ) ) ;
#34919=CARTESIAN_POINT ( 'NONE',  ( 70.29670215996473814, 67.87645915626477233, -9.215380671816021163 ) ) ;
#34925=DIRECTION ( 'NONE',  ( -0.8660254037844379305, -0.5000000000000014433, -0.000000000000000000 ) ) ;
#34933=CARTESIAN_POINT ( 'NONE',  ( 67.24893291460693945, 66.51310417600045355, -8.632834435144324914 ) ) ;
#34938=CARTESIAN_POINT ( 'NONE',  ( 35.31080938399455249, 26.10170272979929607, -7.433330006724141015 ) ) ;
#34943=CARTESIAN_POINT ( 'NONE',  ( 13.01786573420820403, 22.91421378149917842, 9.188101187500008038 ) ) ;
#34952=ORIENTED_EDGE ( 'NONE', *, *, #62897, .F. ) ;
#34957=ORIENTED_EDGE ( 'NONE', *, *, #57791, .F. ) ;
#34958=CARTESIAN_POINT ( 'NONE',  ( 66.38567292659833186, 68.74021793980560346, -2.134846014654135704 ) ) ;
#34961=DIRECTION ( 'NONE',  ( -0.8660254037844377084, -0.5000000000000014433, -0.000000000000000000 ) ) ;
#34971=CARTESIAN_POINT ( 'NONE',  ( 29.04415360562664361, 34.95586893147757479, 7.433330006724141015 ) ) ;
#34982=CARTESIAN_POINT ( 'NONE',  ( 79.70677143361787387, 46.01134058561531504, 12.98241517792750699 ) ) ;
#34984=ORIENTED_EDGE ( 'NONE', *, *, #35995, .T. ) ;
#34989=EDGE_CURVE ( 'NONE', #55973, #46528, #25116, .T. ) ;
#34992=DIRECTION ( 'NONE',  ( -0.7691052716734865236, -0.08748735329024208418, 0.6331058711608359424 ) ) ;
#35007=VERTEX_POINT ( 'NONE', #74139 ) ;
#35008=CARTESIAN_POINT ( 'NONE',  ( 77.33081455423041461, 59.48262537591812560, 16.03249298943872603 ) ) ;
#35015=CARTESIAN_POINT ( 'NONE',  ( 69.40490131253574191, 70.33133358430262660, 3.195916881608930726 ) ) ;
#35018=CARTESIAN_POINT ( 'NONE',  ( 21.09856983598611535, 20.38052372038641025, 10.00000000000000533 ) ) ;
#35035=CARTESIAN_POINT ( 'NONE',  ( 21.90410768801267949, 17.81029122506294726, 8.090169943749479842 ) ) ;
#35036=CARTESIAN_POINT ( 'NONE',  ( 67.91095298726213514, 65.32202572000780094, -10.47973064602391524 ) ) ;
#35040=CARTESIAN_POINT ( 'NONE',  ( 73.86299659849926513, 55.57419400639425788, -16.58552430813258027 ) ) ;
#35043=CARTESIAN_POINT ( 'NONE',  ( 77.23305886468027381, 62.39039902364388723, 15.82877784703884672 ) ) ;
#35053=CARTESIAN_POINT ( 'NONE',  ( 30.99092310034283315, 39.93396525600392977, 2.839279412974139660 ) ) ;
#35061=CARTESIAN_POINT ( 'NONE',  ( 7.821713311501573784, 19.91421378149916421, 9.188101187500008038 ) ) ;
#35063=CARTESIAN_POINT ( 'NONE',  ( 23.64951029700316099, 14.44966523072494802, -2.296566073217252530E-15 ) ) ;
#35067=ORIENTED_EDGE ( 'NONE', *, *, #8669, .F. ) ;
#35068=AXIS2_PLACEMENT_3D ( 'NONE', #77869, #40828, #63650 ) ;
#35076=CARTESIAN_POINT ( 'NONE',  ( 66.58223749524904633, 68.25836364787168975, 4.558095512795234505 ) ) ;
#35077=EDGE_CURVE ( 'NONE', #11388, #81557, #49330, .T. ) ;
#35078=CARTESIAN_POINT ( 'NONE',  ( 87.33294734268929460, 44.88192199842170282, 6.808005391826769781 ) ) ;
#35080=( BOUNDED_CURVE ( )  B_SPLINE_CURVE ( 2, ( #33927, #26312, #43484, #33404, #57187, #18714, #27804, #64305, #95257, #42481, #25824, #49108, #58677 ),
 .UNSPECIFIED., .F., .T. ) 
 B_SPLINE_CURVE_WITH_KNOTS ( ( 3, 2, 2, 2, 2, 2, 3 ),
 ( 0.3624999999999999889, 0.3649999999999999911, 0.3699999999999999956, 0.3750000000000000000, 0.3800000000000000044, 0.3850000000000000089, 0.3875000000000000111 ),
 .UNSPECIFIED. ) 
 CURVE ( )  GEOMETRIC_REPRESENTATION_ITEM ( )  RATIONAL_B_SPLINE_CURVE ( ( 0.9755282581475768211, 0.9755282581475768211, 1.000000000000000000, 0.9510565162951535312, 1.000000000000000000, 0.9510565162951535312, 1.000000000000000000, 0.9510565162951535312, 1.000000000000000000, 0.9510565162951535312, 1.000000000000000000, 0.9755282581475768211, 0.9755282581475768211 ) ) 
 REPRESENTATION_ITEM ( '' )  );
#35085=VERTEX_POINT ( 'NONE', #84742 ) ;
#35090=CARTESIAN_POINT ( 'NONE',  ( 88.50942844660002606, 43.88426665780151836, -0.4971503815960297556 ) ) ;
#35107=CARTESIAN_POINT ( 'NONE',  ( 82.78422215508307147, 53.78621188977053436, 15.78456841880229078 ) ) ;
#35113=CARTESIAN_POINT ( 'NONE',  ( 78.11054252755917560, 56.59592749652284027, -16.20240047345659207 ) ) ;
#35116=CARTESIAN_POINT ( 'NONE',  ( 77.50559704200234989, 49.73895437837127531, -15.47469949631416952 ) ) ;
#35118=CARTESIAN_POINT ( 'NONE',  ( 84.49887340489608789, 41.63797158674129406, -1.523898730005905255 ) ) ;
#35119=AXIS2_PLACEMENT_3D ( 'NONE', #15254, #76110, #77068 ) ;
#35122=CARTESIAN_POINT ( 'NONE',  ( 69.95523204135938045, 62.90150226501648234, 13.86126985460704297 ) ) ;
#35130=VECTOR ( 'NONE', #95370, 1000.000000000000114 ) ;
#35138=CARTESIAN_POINT ( 'NONE',  ( 72.56680254073344827, 71.38637538794351656, 5.777867564336608197 ) ) ;
#35153=CARTESIAN_POINT ( 'NONE',  ( 84.60735463175657856, 50.53152741511170376, -13.60229262012000184 ) ) ;
#35162=CARTESIAN_POINT ( 'NONE',  ( 68.53472279406327061, 64.53069240858096123, -12.19966557917646988 ) ) ;
#35168=CARTESIAN_POINT ( 'NONE',  ( 70.82736078104210264, 70.74693773775240402, 4.782910273999081419 ) ) ;
#35175=CARTESIAN_POINT ( 'NONE',  ( 24.28581821943125263, 16.94754757982090254, 5.678558825948272215 ) ) ;
#35177=CARTESIAN_POINT ( 'NONE',  ( 74.68693990639053482, 67.13232622275778283, 12.47216552256462840 ) ) ;
#35180=CARTESIAN_POINT ( 'NONE',  ( 74.64154962151783934, 66.95428888261444911, 13.01658699031521671 ) ) ;
#35181=CARTESIAN_POINT ( 'NONE',  ( 21.57298720112008894, 14.58380873178786885, 6.180339887498953466 ) ) ;
#35188=CARTESIAN_POINT ( 'NONE',  ( 81.68367041701041842, 55.79078710209740422, -16.00088945688137443 ) ) ;
#35190=CARTESIAN_POINT ( 'NONE',  ( 69.51993594036143520, 67.94519450850054909, 8.515667477277720110 ) ) ;
#35192=CARTESIAN_POINT ( 'NONE',  ( 71.76139268086217271, 72.52520824035065061, 0.9833505332507517238 ) ) ;
#35195=DIRECTION ( 'NONE',  ( 0.4145187862775202015, -0.7179675985244525771, -0.5591929034707450175 ) ) ;
#35198=ADVANCED_FACE ( 'NONE', ( #18812 ), #49697, .T. ) ;
#35199=CARTESIAN_POINT ( 'NONE',  ( 72.23468229527969697, 71.59820328793978206, -5.860928441596811922 ) ) ;
#35204=CARTESIAN_POINT ( 'NONE',  ( 8.129038565245441106, 16.64441083166258650, -10.00000000000000533 ) ) ;
#35207=CYLINDRICAL_SURFACE ( 'NONE', #99927, 10.00000000000001066 ) ;
#35211=VERTEX_POINT ( 'NONE', #76500 ) ;
#35212=CARTESIAN_POINT ( 'NONE',  ( 78.78511898078654951, 60.03407184738823332, 16.11193227242592840 ) ) ;
#35213=CARTESIAN_POINT ( 'NONE',  ( 79.14312167556931854, 57.64441083166269664, 0.000000000000000000 ) ) ;
#35218=CARTESIAN_POINT ( 'NONE',  ( 81.38866437292413991, 50.91805390661637176, -14.64230100137327284 ) ) ;
#35220=CARTESIAN_POINT ( 'NONE',  ( 84.63506747414010079, 49.80695396426073529, -13.18143026763655534 ) ) ;
#35226=CARTESIAN_POINT ( 'NONE',  ( 78.14015596324891533, 47.79605781560269406, 14.53813849190288465 ) ) ;
#35228=CARTESIAN_POINT ( 'NONE',  ( 75.03406391020887156, 58.89278341677606221, 15.85403548772932503 ) ) ;
#35233=CARTESIAN_POINT ( 'NONE',  ( 81.90650872946123684, 41.09198023048384840, 3.645612064814079734 ) ) ;
#35237=CARTESIAN_POINT ( 'NONE',  ( 72.50222618693952370, 68.22314101123330943, -10.37516697382647024 ) ) ;
#35240=CARTESIAN_POINT ( 'NONE',  ( 75.80125281519391933, 55.32059395707344152, 16.14277639286700605 ) ) ;
#35241=CARTESIAN_POINT ( 'NONE',  ( 14.28983037092611319, 10.11110640527290627, -2.839279412974138328 ) ) ;
#35244=CARTESIAN_POINT ( 'NONE',  ( 85.39636071719610300, 48.32640963909398124, -12.26545443191636586 ) ) ;
#35247=CARTESIAN_POINT ( 'NONE',  ( 78.38215086339779702, 48.00876806938738639, -14.02649451357657995 ) ) ;
#35252=CARTESIAN_POINT ( 'NONE',  ( 85.20757786915602594, 42.65106006787098636, 2.242368550657015902 ) ) ;
#35253=CARTESIAN_POINT ( 'NONE',  ( 88.14497077207560949, 43.82233299356100531, -2.120619512623201253 ) ) ;
#35256=CARTESIAN_POINT ( 'NONE',  ( 66.07714878694351057, 69.27459742504910878, 0.2655349905647865771 ) ) ;
#35257=ORIENTED_EDGE ( 'NONE', *, *, #39262, .F. ) ;
#35262=CARTESIAN_POINT ( 'NONE',  ( 80.32560484147226987, 44.93948968179056180, -11.21518412823304800 ) ) ;
#35264=ADVANCED_FACE ( 'NONE', ( #82655 ), #77988, .T. ) ;
#35267=CARTESIAN_POINT ( 'NONE',  ( 88.47364309043327069, 44.01569472767099001, 2.145854971186514693 ) ) ;
#35270=VECTOR ( 'NONE', #41821, 1000.000000000000114 ) ;
#35273=CARTESIAN_POINT ( 'NONE',  ( 80.56697878876413199, 57.58860379435336796, 16.23401761274853428 ) ) ;
#35274=CARTESIAN_POINT ( 'NONE',  ( 70.71537437633379852, 66.12099867655061303, -11.31749738359454760 ) ) ;
#35278=CARTESIAN_POINT ( 'NONE',  ( 81.11567069824683074, 43.42565969520126856, -9.945124925201680455 ) ) ;
#35282=CARTESIAN_POINT ( 'NONE',  ( 87.70182765261645841, 44.38038868594539110, -4.004158056545790600 ) ) ;
#35284=CARTESIAN_POINT ( 'NONE',  ( 79.14312167556931854, 57.64441083166269664, 0.000000000000000000 ) ) ;
#35289=CARTESIAN_POINT ( 'NONE',  ( 71.86256228778262312, 72.60615528678950170, -0.5650332253009007211 ) ) ;
#35290=CARTESIAN_POINT ( 'NONE',  ( 84.66363459063573771, 50.58495542193022487, 13.62716051735802836 ) ) ;
#35292=CARTESIAN_POINT ( 'NONE',  ( 80.63310098719156827, 53.50240974728008325, -16.03299162280124435 ) ) ;
#35303=CARTESIAN_POINT ( 'NONE',  ( 36.84800447571193160, 26.98920272979929180, 7.433330006724137462 ) ) ;
#35307=CARTESIAN_POINT ( 'NONE',  ( 25.00689474275853286, 16.29860640527292759, -2.839279412974138328 ) ) ;
#35312=CARTESIAN_POINT ( 'NONE',  ( 86.12260107077111115, 47.06852444819536885, 10.76136662946663947 ) ) ;
#35314=EDGE_CURVE ( 'NONE', #98353, #65113, #51956, .T. ) ;
#35318=CARTESIAN_POINT ( 'NONE',  ( 22.17949989257922283, 28.50829794293881037, -10.00000000000000355 ) ) ;
#35321=CARTESIAN_POINT ( 'NONE',  ( 85.80882896958009098, 47.30052720894016716, 10.64875693516724908 ) ) ;
#35324=CARTESIAN_POINT ( 'NONE',  ( 84.79859407451725417, 42.50768657221069446, 2.813679082869662285 ) ) ;
#35328=ORIENTED_EDGE ( 'NONE', *, *, #58199, .F. ) ;
#35333=CARTESIAN_POINT ( 'NONE',  ( 87.79556561918005286, 44.17086485108952587, -4.468589225908877971 ) ) ;
#35337=CARTESIAN_POINT ( 'NONE',  ( 35.92184506804998279, 29.24335787977765833, -9.188101187500008038 ) ) ;
#35343=VERTEX_POINT ( 'NONE', #23773 ) ;
#35344=CARTESIAN_POINT ( 'NONE',  ( 81.09996276884294275, 42.55047014966801555, 7.932854448062508723 ) ) ;
#35346=CARTESIAN_POINT ( 'NONE',  ( 68.35453417343933324, 65.67399229982113695, 10.37910612949749023 ) ) ;
#35356=VERTEX_POINT ( 'NONE', #79903 ) ;
#35357=CARTESIAN_POINT ( 'NONE',  ( 73.73249371147525721, 55.30366856558931232, -16.59341848673177111 ) ) ;
#35362=CARTESIAN_POINT ( 'NONE',  ( 87.04122873496829982, 46.31593380912286051, -9.298662157179396814 ) ) ;
#35375=CARTESIAN_POINT ( 'NONE',  ( 83.05052185759683425, 46.42945747414138680, 11.22551205484409564 ) ) ;
#35382=CARTESIAN_POINT ( 'NONE',  ( 81.97334639510765442, 41.04379167472870193, -3.293735024885245721 ) ) ;
#35391=CARTESIAN_POINT ( 'NONE',  ( 79.98636212202836759, 50.06317686608937834, 14.58694793862931327 ) ) ;
#35392=CARTESIAN_POINT ( 'NONE',  ( 67.02271111079838306, 69.26504780342379775, -0.6689381131363330013 ) ) ;
#35399=CARTESIAN_POINT ( 'NONE',  ( 33.32035334334607057, 27.43677371833803846, -10.00000000000000355 ) ) ;
#35401=CARTESIAN_POINT ( 'NONE',  ( 70.73808989031111594, 70.90155945549474836, -4.160261088369678006 ) ) ;
#35403=CARTESIAN_POINT ( 'NONE',  ( 5.294102074706517058, 26.55466486950697558, -1.111400068045478839E-16 ) ) ;
#35404=CARTESIAN_POINT ( 'NONE',  ( 39.11189823470242999, 30.78052372038643725, -10.00000000000000355 ) ) ;
#35405=CARTESIAN_POINT ( 'NONE',  ( 72.55490714944258457, 58.69537080386778172, -16.07943689878887739 ) ) ;
#35411=CARTESIAN_POINT ( 'NONE',  ( 87.88902802526534686, 43.91876200309240375, 0.4180276961671919311 ) ) ;
#35413=CARTESIAN_POINT ( 'NONE',  ( 86.85818799200686158, 46.48416747087964751, 9.041777841573095387 ) ) ;
#35416=CARTESIAN_POINT ( 'NONE',  ( 71.75124654091098364, 72.49002453570855664, -1.344699539992842752 ) ) ;
#35418=B_SPLINE_CURVE_WITH_KNOTS ( 'NONE', 3,
 ( #69886, #64297, #96736, #89168, #19715, #57180, #95750, #66295, #56689, #17703 ),
 .UNSPECIFIED., .F., .F.,
 ( 4, 2, 2, 2, 4 ),
 ( 0.000000000000000000, 0.2500000000000000000, 0.5000000000000000000, 0.7500000000000000000, 1.000000000000000000 ),
 .UNSPECIFIED. ) ;
#35423=CARTESIAN_POINT ( 'NONE',  ( 2.730238736670422384, 24.68290643055184574, 3.479690158560446702E-15 ) ) ;
#35427=LINE ( 'NONE', #66332, #8841 ) ;
#35429=EDGE_CURVE ( 'NONE', #45858, #99079, #55166, .T. ) ;
#35435=EDGE_LOOP ( 'NONE', ( #26892, #23990, #98141, #24093 ) ) ;
#35440=CARTESIAN_POINT ( 'NONE',  ( 67.63792478863227586, 66.83026407364596366, -8.502183981914797073 ) ) ;
#35446=CARTESIAN_POINT ( 'NONE',  ( 34.18979426048110781, 28.24335787977765122, -9.188101187500008038 ) ) ;
#35450=ORIENTED_EDGE ( 'NONE', *, *, #75734, .F. ) ;
#35451=CARTESIAN_POINT ( 'NONE',  ( 17.99030130830579566, 16.10170272979926054, -7.433330006724141015 ) ) ;
#35452=CARTESIAN_POINT ( 'NONE',  ( 68.79254404386716715, 64.26810367574286431, 12.51937741639473245 ) ) ;
#35454=CARTESIAN_POINT ( 'NONE',  ( 17.73189607522619582, 18.43677371833801359, -10.00000000000000355 ) ) ;
#35455=VERTEX_POINT ( 'NONE', #26662 ) ;
#35456=CARTESIAN_POINT ( 'NONE',  ( 77.47728950214126087, 59.35671389659360386, 16.44570396066454521 ) ) ;
#35464=CARTESIAN_POINT ( 'NONE',  ( 66.07037714390584426, 68.51423597247097064, -2.421109949964840524 ) ) ;
#35468=CARTESIAN_POINT ( 'NONE',  ( 77.91510949599519620, 62.18724900762369856, -15.97225761198294691 ) ) ;
#35471=CARTESIAN_POINT ( 'NONE',  ( 79.14312167556931854, 57.64441083166269664, 0.000000000000000000 ) ) ;
#35476=ORIENTED_EDGE ( 'NONE', *, *, #93191, .F. ) ;
#35479=CARTESIAN_POINT ( 'NONE',  ( 75.30099715557209095, 66.83639500800819633, -12.91230939377402542 ) ) ;
#35481=ORIENTED_EDGE ( 'NONE', *, *, #80665, .T. ) ;
#35488=CARTESIAN_POINT ( 'NONE',  ( 76.11542371522575934, 62.61180736277591308, -15.13754670253717194 ) ) ;
#35490=ORIENTED_EDGE ( 'NONE', *, *, #59890, .F. ) ;
#35492=CARTESIAN_POINT ( 'NONE',  ( 81.89930626873778863, 42.21375885382297355, 7.647715624843501203 ) ) ;
#35498=EDGE_CURVE ( 'NONE', #24001, #47421, #21347, .T. ) ;
#35506=CARTESIAN_POINT ( 'NONE',  ( 85.48944666241685297, 43.63848491286618980, 5.277307547990027103 ) ) ;
#35510=CARTESIAN_POINT ( 'NONE',  ( 73.95048969143448403, 57.13095431899427723, 16.00405266783817027 ) ) ;
#35513=CARTESIAN_POINT ( 'NONE',  ( 76.59400919359040927, 55.08999672436397788, 16.14094864937774787 ) ) ;
#35526=CARTESIAN_POINT ( 'NONE',  ( 15.84452179826556417, 32.08080186712592763, -3.090169943749475845 ) ) ;
#35541=CARTESIAN_POINT ( 'NONE',  ( 83.76030657582204242, 41.96383438897017726, 4.835547397684552884 ) ) ;
#35542=CARTESIAN_POINT ( 'NONE',  ( 17.08077532425043543, 25.56454794089041727, 10.00000000000000355 ) ) ;
#35543=CARTESIAN_POINT ( 'NONE',  ( 85.23821057327256767, 49.07543163279748910, 12.45235422365945510 ) ) ;
#35546=CARTESIAN_POINT ( 'NONE',  ( 73.83032011078108781, 55.08034924954741740, -16.60147083384191902 ) ) ;
#35559=CARTESIAN_POINT ( 'NONE',  ( 40.22068564906490451, 26.14754757982093381, -5.678558825948276656 ) ) ;
#35567=CARTESIAN_POINT ( 'NONE',  ( 16.48196734934595753, 24.91421378149918198, 9.188101187500008038 ) ) ;
#35568=CARTESIAN_POINT ( 'NONE',  ( 71.53080809438635868, 72.38941617099001746, 1.021674839914414878 ) ) ;
#35569=CARTESIAN_POINT ( 'NONE',  ( 82.17887732911846399, 54.20604701261002845, 15.63465942432049083 ) ) ;
#35571=CARTESIAN_POINT ( 'NONE',  ( 71.63453813518020752, 72.07236434383467838, 0.7172108931481352423 ) ) ;
#35572=EDGE_CURVE ( 'NONE', #89714, #73699, #83385, .T. ) ;
#35583=CARTESIAN_POINT ( 'NONE',  ( 66.31130943496550856, 68.58487545890584158, 4.825481589580086883 ) ) ;
#35591=CARTESIAN_POINT ( 'NONE',  ( 88.30455217607853058, 43.91915848855261828, -2.151936166193182398 ) ) ;
#35592=CARTESIAN_POINT ( 'NONE',  ( 80.56743834928197145, 57.59328067535012252, 16.23428813468583698 ) ) ;
#35595=CARTESIAN_POINT ( 'NONE',  ( 82.37376302093576896, 49.21181299837914480, -13.53283297697456966 ) ) ;
#35596=CARTESIAN_POINT ( 'NONE',  ( 81.28581595673009019, 43.24335794003573596, 9.611647108222669544 ) ) ;
#35600=CARTESIAN_POINT ( 'NONE',  ( 73.71617248606330008, 59.79991374540308868, 15.48773420481832730 ) ) ;
#35619=B_SPLINE_CURVE_WITH_KNOTS ( 'NONE', 3,
 ( #73973, #58735, #27368, #98276, #58251, #35456, #44535, #66359, #97292, #90710, #66850, #89711, #20272, #67859, #97778, #21266 ),
 .UNSPECIFIED., .F., .F.,
 ( 4, 1, 2, 2, 2, 1, 2, 2, 4 ),
 ( 0.000000000000000000, 0.1250000000000005551, 0.1875000000000007494, 0.2500000000000009437, 0.4999999999999994449, 0.6249999999999976685, 0.6874999999999981126, 0.7499999999999986677, 1.000000000000000000 ),
 .UNSPECIFIED. ) ;
#35628=CARTESIAN_POINT ( 'NONE',  ( 83.51092623577891061, 51.50185674319120466, -14.43088262691036583 ) ) ;
#35630=CARTESIAN_POINT ( 'NONE',  ( 14.46184932687122604, 20.30066082961420904, -10.00000000000000533 ) ) ;
#35647=ORIENTED_EDGE ( 'NONE', *, *, #37351, .T. ) ;
#35649=CARTESIAN_POINT ( 'NONE',  ( 74.46690696312865043, 68.23757356209769398, -11.48548186069604782 ) ) ;
#35651=CARTESIAN_POINT ( 'NONE',  ( 70.94579913988255271, 71.56585977893712425, -1.408710708485262586 ) ) ;
#35654=CARTESIAN_POINT ( 'NONE',  ( 81.98471768757296729, 41.36544628577401994, -5.913068783389250349 ) ) ;
#35667=CARTESIAN_POINT ( 'NONE',  ( 73.22997076551303053, 69.87431308930813145, 9.604659174840600500 ) ) ;
#35672=CARTESIAN_POINT ( 'NONE',  ( 66.35038720663168021, 68.05568594965032503, -4.770468563139677265 ) ) ;
#35675=ADVANCED_FACE ( 'NONE', ( #54292 ), #98944, .T. ) ;
#35680=CARTESIAN_POINT ( 'NONE',  ( 28.70736568013821355, 22.28920272979928185, -7.433330006724141015 ) ) ;
#35682=CARTESIAN_POINT ( 'NONE',  ( 83.53204454370724363, 52.39401912150450613, -15.17729711222452416 ) ) ;
#35694=CARTESIAN_POINT ( 'NONE',  ( 3.479571460297436136, 22.98502408145589726, -5.678558825948271327 ) ) ;
#35696=CARTESIAN_POINT ( 'NONE',  ( 70.74552968606906234, 69.97318964771673677, 6.399120444304696953 ) ) ;
#35699=CARTESIAN_POINT ( 'NONE',  ( 85.04775486883579561, 44.40351755419373347, 7.355666434035634360 ) ) ;
#35702=CARTESIAN_POINT ( 'NONE',  ( 70.78531041105927102, 71.56694630268400203, -0.1705850445758182454 ) ) ;
#35706=CARTESIAN_POINT ( 'NONE',  ( 3.304740145946305052, 26.00034080476288167, -1.878358725466461243E-16 ) ) ;
#35715=CARTESIAN_POINT ( 'NONE',  ( 74.88534510618254103, 53.30470171424536829, 16.04906050052737498 ) ) ;
#35719=CARTESIAN_POINT ( 'NONE',  ( 80.33508072308799797, 44.92307697338561923, 11.19555900290710149 ) ) ;
#35720=CARTESIAN_POINT ( 'NONE',  ( 84.57060543673907205, 49.80382465363337019, -13.20176661028953546 ) ) ;
#35730=CARTESIAN_POINT ( 'NONE',  ( 75.85732906438254020, 63.05884040557971559, 14.92899268908093013 ) ) ;
#35734=CARTESIAN_POINT ( 'NONE',  ( 82.46767041311871083, 40.74398673389430314, 3.187025703938450416 ) ) ;
#35739=CARTESIAN_POINT ( 'NONE',  ( 20.87599742628078303, 30.79103043416549568, 8.090169943749478065 ) ) ;
#35742=CARTESIAN_POINT ( 'NONE',  ( 75.95592525424871155, 56.02552295162529816, 16.15038119120977100 ) ) ;
#35743=CARTESIAN_POINT ( 'NONE',  ( 14.52619969316804394, 14.10170272979925699, -7.433330006724141015 ) ) ;
#35749=CARTESIAN_POINT ( 'NONE',  ( 76.20329143637185609, 64.79007453736731748, -14.35255403285628795 ) ) ;
#35758=CARTESIAN_POINT ( 'NONE',  ( 77.28846913097220295, 61.37098587332354072, -15.71112316387479879 ) ) ;
#35772=CARTESIAN_POINT ( 'NONE',  ( 79.83821995607597444, 57.92396234388704102, 16.26578674484267495 ) ) ;
#35774=CARTESIAN_POINT ( 'NONE',  ( 85.76569060431222624, 48.58547048772101107, -11.83440413304170846 ) ) ;
#35779=CARTESIAN_POINT ( 'NONE',  ( 81.03696130064014369, 43.68575652313568725, -9.501319341590960477 ) ) ;
#35785=CARTESIAN_POINT ( 'NONE',  ( 79.12246707933677214, 57.02010426323071357, 16.20246513760482543 ) ) ;
#35786=CARTESIAN_POINT ( 'NONE',  ( 81.53115339410010165, 41.92267797703283350, -7.515177224638171616 ) ) ;
#35789=CARTESIAN_POINT ( 'NONE',  ( 84.80172950927561715, 50.19486025153376829, 13.34007759942640803 ) ) ;
#35793=B_SPLINE_CURVE_WITH_KNOTS ( 'NONE', 3,
 ( #50940, #65151, #27164, #4868, #43836, #19079, #58052, #35247, #96098, #81890 ),
 .UNSPECIFIED., .F., .F.,
 ( 4, 2, 2, 2, 4 ),
 ( 0.000000000000000000, 0.2500000000000000000, 0.5000000000000000000, 0.7500000000000000000, 1.000000000000000000 ),
 .UNSPECIFIED. ) ;
#35798=CARTESIAN_POINT ( 'NONE',  ( 3.825981621811214151, 23.18502408145589300, 5.678558825948277544 ) ) ;
#35804=CARTESIAN_POINT ( 'NONE',  ( 75.64192366613818308, 65.38353595949358521, 14.29496885373930226 ) ) ;
#35806=CARTESIAN_POINT ( 'NONE',  ( 30.99092310034283315, 39.93396525600392977, 2.839279412974139660 ) ) ;
#35808=CARTESIAN_POINT ( 'NONE',  ( 86.41066968851905017, 46.49022025137010417, -9.329619672313064882 ) ) ;
#35810=CARTESIAN_POINT ( 'NONE',  ( 25.38156110457203241, 15.44966523072494624, -2.296566073217252530E-15 ) ) ;
#35815=CARTESIAN_POINT ( 'NONE',  ( 70.33479273767041207, 61.15449313193268210, 14.84539183123301775 ) ) ;
#35819=CARTESIAN_POINT ( 'NONE',  ( 85.69563749947228359, 42.25122789774620458, -8.045052972278457832E-08 ) ) ;
#35823=CARTESIAN_POINT ( 'NONE',  ( 82.63766857847271297, 46.45602455969778788, -12.04605856197770031 ) ) ;
#35827=CARTESIAN_POINT ( 'NONE',  ( 81.66745758616980311, 42.31905251298808679, -8.034357111095493664 ) ) ;
#35829=CARTESIAN_POINT ( 'NONE',  ( 77.30903763899321746, 63.28101462763900997, -15.19399449308598804 ) ) ;
#35830=EDGE_LOOP ( 'NONE', ( #41221, #1809, #75107, #10231 ) ) ;
#35832=CARTESIAN_POINT ( 'NONE',  ( 2.966658798487924908, 25.21091486745858035, 1.000260061240931054E-15 ) ) ;
#35838=CARTESIAN_POINT ( 'NONE',  ( 40.42517716772906056, 31.84335787977767041, 9.188101187500006262 ) ) ;
#35839=CARTESIAN_POINT ( 'NONE',  ( 76.00075513927814086, 59.66202446853887409, -15.83865532722460578 ) ) ;
#35845=CARTESIAN_POINT ( 'NONE',  ( 81.61509234124716272, 42.58397340471713477, 7.503678272258770043 ) ) ;
#35849=CARTESIAN_POINT ( 'NONE',  ( 85.48805828002734586, 48.64268271054365300, 12.46980397201070900 ) ) ;
#35852=CARTESIAN_POINT ( 'NONE',  ( 82.36398727104865713, 40.36718183008564154, 1.065671972821284230 ) ) ;
#35861=CARTESIAN_POINT ( 'NONE',  ( 87.08174047714162214, 46.31017841404310786, -9.261312696178791271 ) ) ;
#35865=CARTESIAN_POINT ( 'NONE',  ( 73.67824366217406862, 55.52431661998092238, 16.58293631993679540 ) ) ;
#35877=ORIENTED_EDGE ( 'NONE', *, *, #22608, .F. ) ;
#35879=CARTESIAN_POINT ( 'NONE',  ( 81.86216086620987653, 49.16130738973323844, 13.63634663801094327 ) ) ;
#35880=CARTESIAN_POINT ( 'NONE',  ( 82.33378460754960315, 40.34433662615649041, -0.9934756154102190040 ) ) ;
#35881=DIRECTION ( 'NONE',  ( 0.4924038765061026779, -0.8528685319524446085, -0.1736481776669273058 ) ) ;
#35884=CARTESIAN_POINT ( 'NONE',  ( 71.93253201618666992, 72.27632922802737880, 3.295383250428975064 ) ) ;
#35886=EDGE_CURVE ( 'NONE', #16015, #24489, #66031, .T. ) ;
#35888=CARTESIAN_POINT ( 'NONE',  ( 80.60695466096186124, 53.05637191785592677, 15.52015733122538244 ) ) ;
#35889=CARTESIAN_POINT ( 'NONE',  ( 67.58545467128371342, 69.55077376957733293, -1.347700640191054289 ) ) ;
#35893=CARTESIAN_POINT ( 'NONE',  ( 77.61092910917922438, 61.85833765720148847, 15.65612403738310476 ) ) ;
#35897=CARTESIAN_POINT ( 'NONE',  ( 73.70226580840751751, 69.60776679690043522, -9.655525091778702773 ) ) ;
#35899=CARTESIAN_POINT ( 'NONE',  ( 15.82880751958831667, 10.10801979619927415, 3.090169943749476733 ) ) ;
#35900=CARTESIAN_POINT ( 'NONE',  ( 35.84185148634745843, 32.64441083166263979, -10.00000000000000533 ) ) ;
#35902=CARTESIAN_POINT ( 'NONE',  ( 82.07265110639774264, 53.99302234254209054, 15.59308437138325587 ) ) ;
#35903=CARTESIAN_POINT ( 'NONE',  ( 71.66453512356649469, 72.11062924793525042, 3.341973230705647335 ) ) ;
#35905=CARTESIAN_POINT ( 'NONE',  ( 70.73562432741556449, 71.76670644637469820, 2.397384686151506905 ) ) ;
#35908=CARTESIAN_POINT ( 'NONE',  ( 87.05137182546295094, 46.44927321608544446, 8.839680459623687980 ) ) ;
#35911=CARTESIAN_POINT ( 'NONE',  ( 35.84185148634745843, 32.64441083166263979, -10.00000000000000533 ) ) ;
#35913=CARTESIAN_POINT ( 'NONE',  ( 86.86399242946149002, 45.94634269538593685, 8.946615921987719489 ) ) ;
#35916=CARTESIAN_POINT ( 'NONE',  ( 6.332637391379750014, 21.84336893147753855, -7.433330006724137462 ) ) ;
#35920=CARTESIAN_POINT ( 'NONE',  ( 72.90981660445726220, 62.57208767169331054, 14.37557442138605523 ) ) ;
#35921=CARTESIAN_POINT ( 'NONE',  ( 72.29738803710162642, 67.68364943355766172, -10.75058748413067633 ) ) ;
#35922=CARTESIAN_POINT ( 'NONE',  ( 86.93590031418035835, 45.88516064952855089, -8.148499982929045871 ) ) ;
#35923=CARTESIAN_POINT ( 'NONE',  ( 81.96547941067910870, 41.17040324926905015, 3.814626384468428721 ) ) ;
#35925=CARTESIAN_POINT ( 'NONE',  ( 74.98858861178062796, 53.12804837913225953, 16.50569088578514254 ) ) ;
#35932=CARTESIAN_POINT ( 'NONE',  ( 67.36400621912697773, 67.24424126167714633, -8.606104698649938101 ) ) ;
#35937=CARTESIAN_POINT ( 'NONE',  ( 25.67147243227365294, 35.79752408145593989, -5.678558825948271327 ) ) ;
#35940=ADVANCED_FACE ( 'NONE', ( #59792 ), #62582, .T. ) ;
#35943=ORIENTED_EDGE ( 'NONE', *, *, #1510, .T. ) ;
#35944=CARTESIAN_POINT ( 'NONE',  ( 13.73114039420206645, 19.87878583063839955, -9.188101187500006262 ) ) ;
#35946=CARTESIAN_POINT ( 'NONE',  ( 66.90480444531253568, 69.14389213734473572, -1.488062147591796114 ) ) ;
#35954=FACE_OUTER_BOUND ( 'NONE', #40942, .T. ) ;
#35957=CARTESIAN_POINT ( 'NONE',  ( 66.07036783887816966, 68.50746885787836504, -2.462010881573316823 ) ) ;
#35963=DIRECTION ( 'NONE',  ( 0.2033683215378999376, -0.3522442655536480172, -0.9135454576426004225 ) ) ;
#35964=VERTEX_POINT ( 'NONE', #10104 ) ;
#35973=CARTESIAN_POINT ( 'NONE',  ( 81.76364840784469834, 55.63774643643142781, 16.32517576395870407 ) ) ;
#35978=CARTESIAN_POINT ( 'NONE',  ( 77.73560472764970086, 61.98338471776878578, -15.62265401182667546 ) ) ;
#35979=CARTESIAN_POINT ( 'NONE',  ( 66.26615415756170080, 68.24338033411152082, 4.053640967902321535 ) ) ;
#35983=CARTESIAN_POINT ( 'NONE',  ( 76.23362574048000795, 51.00037424386685814, -15.55159192653386846 ) ) ;
#35993=CARTESIAN_POINT ( 'NONE',  ( 88.08546139208640113, 44.41188104239807188, 4.690966480777963632 ) ) ;
#35995=EDGE_CURVE ( 'NONE', #60500, #30119, #47090, .T. ) ;
#35996=CARTESIAN_POINT ( 'NONE',  ( 79.89568642616896454, 44.56385848865007659, -11.10247427051291957 ) ) ;
#36001=CARTESIAN_POINT ( 'NONE',  ( 77.29002174012607895, 59.18083051215872814, 16.06399558427829888 ) ) ;
#36005=CARTESIAN_POINT ( 'NONE',  ( 73.53265170616339219, 69.21111818949283645, -10.01235007243518282 ) ) ;
#36014=CARTESIAN_POINT ( 'NONE',  ( 16.78929260308981952, 21.64441083166260427, -10.00000000000000533 ) ) ;
#36018=CARTESIAN_POINT ( 'NONE',  ( 72.24373504362831966, 72.05182877291241539, -3.239030724485916224 ) ) ;
#36019=B_SPLINE_CURVE_WITH_KNOTS ( 'NONE', 3,
 ( #32601, #48815, #63499, #24991, #55867, #33610, #64506, #26017, #56888, #22250, #27986, #34116, #89359, #68348, #50291, #35595, #26512, #19913, #49796, #74113, #19436, #82246, #99273, #29856, #60726, #45046, #73124, #91688, #50784, #42189, #27007, #53153, #6565, #37437, #20410, #3715, #89834, #10812, #81245, #57893, #18923, #34595, #81734, #80760, #4706, #65494 ),
 .UNSPECIFIED., .F., .F.,
 ( 4, 1, 2, 2, 1, 2, 2, 1, 1, 2, 2, 1, 1, 2, 2, 1, 1, 2, 2, 1, 1, 1, 2, 2, 1, 1, 1, 2, 2, 4 ),
 ( 0.000000000000000000, 0.06249999999998788469, 0.09374999999998182010, 0.1249999999999757694, 0.1874999999999677758, 0.2187499999999636402, 0.2499999999999595324, 0.3124999999999504841, 0.3437499999999476530, 0.3593749999999477085, 0.3749999999999477640, 0.4374999999999529265, 0.4687499999999537037, 0.4843749999999523159, 0.4999999999999509281, 0.5624999999999494849, 0.5937499999999465983, 0.6093749999999452660, 0.6249999999999439337, 0.6874999999999414912, 0.7187499999999403810, 0.7343749999999413802, 0.7421874999999418243, 0.7499999999999422684, 0.8124999999999472644, 0.8437499999999513722, 0.8593749999999534817, 0.8671874999999562572, 0.8749999999999590328, 1.000000000000000000 ),
 .UNSPECIFIED. ) ;
#36028=CARTESIAN_POINT ( 'NONE',  ( 86.70911053808110580, 46.89117940024963360, 10.21290512048939547 ) ) ;
#36029=CARTESIAN_POINT ( 'NONE',  ( 27.43138059761189496, 24.03677371833802923, 10.00000000000000533 ) ) ;
#36036=CARTESIAN_POINT ( 'NONE',  ( 75.12850925987632422, 67.10442048360499712, 12.66444045603761026 ) ) ;
#36044=CARTESIAN_POINT ( 'NONE',  ( 41.44275701717577221, 32.43085787977767609, -9.188101187500008038 ) ) ;
#36047=CARTESIAN_POINT ( 'NONE',  ( 21.39005255714673126, 24.30066082961421969, -10.00000000000000533 ) ) ;
#36051=CARTESIAN_POINT ( 'NONE',  ( 14.44441505419593064, 16.84335787977761711, 9.188101187500006262 ) ) ;
#36052=CARTESIAN_POINT ( 'NONE',  ( 71.64147408072076928, 72.45736481867631085, 0.9627058344235117637 ) ) ;
#36057=ORIENTED_EDGE ( 'NONE', *, *, #67447, .T. ) ;
#36062=CARTESIAN_POINT ( 'NONE',  ( 81.35882998133553201, 42.02707565754876384, 7.853547620083842773 ) ) ;
#36065=CARTESIAN_POINT ( 'NONE',  ( 72.26191451101281871, 71.91445694603925176, -5.118044210176698527 ) ) ;
#36067=CARTESIAN_POINT ( 'NONE',  ( 66.46432511499183704, 68.67385870075324306, 4.823677987632845721 ) ) ;
#36075=CARTESIAN_POINT ( 'NONE',  ( 88.23959751488011705, 43.87687695675944610, -2.120018653157903721 ) ) ;
#36076=CARTESIAN_POINT ( 'NONE',  ( 80.42870892512175374, 57.78063267130219316, 16.59889063300756717 ) ) ;
#36080=CARTESIAN_POINT ( 'NONE',  ( 87.54964925812681997, 45.08772413541393576, -6.108523167108508289 ) ) ;
#36090=CARTESIAN_POINT ( 'NONE',  ( 34.99667586858890900, 35.90829794293883737, 10.00000000000000355 ) ) ;
#36092=VERTEX_POINT ( 'NONE', #64299 ) ;
#36103=CARTESIAN_POINT ( 'NONE',  ( 74.16082345638017159, 57.99061582411809468, -15.91439080673301731 ) ) ;
#36112=CARTESIAN_POINT ( 'NONE',  ( 71.31535561598460049, 67.97248318114000654, 9.859851264107916791 ) ) ;
#36113=EDGE_CURVE ( 'NONE', #7411, #84127, #19226, .T. ) ;
#36114=CARTESIAN_POINT ( 'NONE',  ( 84.02521314179199408, 41.77600783192887945, 3.730838443793543568 ) ) ;
#36119=EDGE_CURVE ( 'NONE', #65992, #66239, #33834, .T. ) ;
#36120=CARTESIAN_POINT ( 'NONE',  ( 84.67893657527464768, 44.90132223245755227, 9.238919453567655538 ) ) ;
#36137=CARTESIAN_POINT ( 'NONE',  ( 69.57285913202781558, 70.79546693701125548, 0.5177190112630815078 ) ) ;
#36139=CARTESIAN_POINT ( 'NONE',  ( 81.86430770026659332, 41.23265223418440684, -5.767287080406577893 ) ) ;
#36140=CARTESIAN_POINT ( 'NONE',  ( 10.70626499057286196, 14.38052372038638893, 10.00000000000000533 ) ) ;
#36151=CARTESIAN_POINT ( 'NONE',  ( 5.995650155809630455, 19.16454794089039382, -10.00000000000000355 ) ) ;
#36152=CARTESIAN_POINT ( 'NONE',  ( 80.95016728299943054, 53.58696901841446447, 16.00970915675678796 ) ) ;
#36153=CARTESIAN_POINT ( 'NONE',  ( 71.80310585937155565, 59.28703135751661790, -15.30483328490166706 ) ) ;
#36154=CARTESIAN_POINT ( 'NONE',  ( 73.63016447670500497, 69.73264996670253879, 9.457047152984245031 ) ) ;
#36159=CARTESIAN_POINT ( 'NONE',  ( 66.36918592400230921, 68.05458625204849454, -4.804853499357824020 ) ) ;
#36160=ORIENTED_EDGE ( 'NONE', *, *, #20042, .T. ) ;
#36163=VECTOR ( 'NONE', #52380, 1000.000000000000000 ) ;
#36165=CARTESIAN_POINT ( 'NONE',  ( 18.69336236660381090, 32.83396525600390703, -2.839279412974133887 ) ) ;
#36168=DIRECTION ( 'NONE',  ( -0.7235470741700464892, -0.1663964660674591423, -0.6699192843471715175 ) ) ;
#36169=VECTOR ( 'NONE', #158, 1000.000000000000000 ) ;
#36171=CARTESIAN_POINT ( 'NONE',  ( 74.76437051368166919, 67.10386306624577912, 12.96231939749656270 ) ) ;
#36172=CARTESIAN_POINT ( 'NONE',  ( 69.11514122063265120, 64.27165015964561690, 12.02313996166621024 ) ) ;
#36176=CARTESIAN_POINT ( 'NONE',  ( 68.82950249375011254, 67.23871426837432352, -9.720984335491779760 ) ) ;
#36180=CARTESIAN_POINT ( 'NONE',  ( 71.11409818138567118, 70.51317934531886067, 5.732207205114195681 ) ) ;
#36182=CARTESIAN_POINT ( 'NONE',  ( 83.03454124716056128, 41.89555541620175205, 4.196031385176040018 ) ) ;
#36186=DIRECTION ( 'NONE',  ( -0.8660254037844377084, -0.5000000000000014433, -0.000000000000000000 ) ) ;
#36189=CARTESIAN_POINT ( 'NONE',  ( 10.64836937555893570, 29.08080186712591697, -3.090169943749475845 ) ) ;
#36193=CARTESIAN_POINT ( 'NONE',  ( 86.50731970396800818, 47.43598145919347786, -10.90780039058066997 ) ) ;
#36202=VERTEX_POINT ( 'NONE', #3519 ) ;
#36205=CARTESIAN_POINT ( 'NONE',  ( 73.29675513422920119, 69.64584746942686877, -9.922798968680028864 ) ) ;
#36209=ADVANCED_FACE ( 'NONE', ( #74421 ), #5006, .T. ) ;
#36215=CARTESIAN_POINT ( 'NONE',  ( 81.76857307223471594, 51.79620215026877617, 14.92011331900278925 ) ) ;
#36216=ORIENTED_EDGE ( 'NONE', *, *, #24872, .F. ) ;
#36217=CARTESIAN_POINT ( 'NONE',  ( 75.40712543759373432, 60.69022127545543555, 15.54263831071833479 ) ) ;
#36219=VERTEX_POINT ( 'NONE', #11615 ) ;
#36221=DIRECTION ( 'NONE',  ( -0.2837547813814367825, -0.9281390619545411003, 0.2409172175609656796 ) ) ;
#36224=CARTESIAN_POINT ( 'NONE',  ( 71.50952208868150706, 68.35890179303125080, -9.555329829617408066 ) ) ;
#36227=CARTESIAN_POINT ( 'NONE',  ( 76.18443605400364049, 57.11110936434808849, 16.13045278074740452 ) ) ;
#36228=CARTESIAN_POINT ( 'NONE',  ( 8.534987971495436199, 16.87878583063839599, -9.188101187500006262 ) ) ;
#36229=ORIENTED_EDGE ( 'NONE', *, *, #64011, .T. ) ;
#36240=CARTESIAN_POINT ( 'NONE',  ( 85.58674419670936118, 42.96232126506118476, 2.800701338658758921 ) ) ;
#36241=CARTESIAN_POINT ( 'NONE',  ( 88.44819812734249354, 44.06706281553302773, -2.545729839345954204 ) ) ;
#36245=CARTESIAN_POINT ( 'NONE',  ( 71.28447224701196205, 63.33288523720543850, -13.51654472431917497 ) ) ;
#36249=EDGE_CURVE ( 'NONE', #39006, #49112, #49169, .T. ) ;
#36252=CARTESIAN_POINT ( 'NONE',  ( 87.69503266575394207, 44.73314950816818936, -5.003925075596086458 ) ) ;
#36255=CARTESIAN_POINT ( 'NONE',  ( 88.03161368674544462, 43.80918251920726902, 2.446934266190721186 ) ) ;
#36264=ADVANCED_FACE ( 'NONE', ( #10606 ), #83028, .T. ) ;
#36265=CARTESIAN_POINT ( 'NONE',  ( 85.74281436412356072, 48.57633205417285893, -12.30481470458759929 ) ) ;
#36268=( BOUNDED_CURVE ( )  B_SPLINE_CURVE ( 2, ( #1504, #24291, #32879, #55168, #25805, #47577, #90115, #42951, #43466, #96725, #65767, #58173, #73890 ),
 .UNSPECIFIED., .F., .T. ) 
 B_SPLINE_CURVE_WITH_KNOTS ( ( 3, 2, 2, 2, 2, 2, 3 ),
 ( 0.5125000000000000666, 0.5150000000000000133, 0.5200000000000000178, 0.5250000000000000222, 0.5300000000000000266, 0.5350000000000000311, 0.5375000000000000888 ),
 .UNSPECIFIED. ) 
 CURVE ( )  GEOMETRIC_REPRESENTATION_ITEM ( )  RATIONAL_B_SPLINE_CURVE ( ( 0.9755282581475767101, 0.9755282581475772652, 1.000000000000000000, 0.9510565162951535312, 1.000000000000000000, 0.9510565162951535312, 1.000000000000000000, 0.9510565162951535312, 1.000000000000000000, 0.9510565162951535312, 1.000000000000000000, 0.9755282581475761550, 0.9755282581475767101 ) ) 
 REPRESENTATION_ITEM ( '' )  );
#36269=CARTESIAN_POINT ( 'NONE',  ( 81.19656099882028855, 43.43094936609876555, -9.896970666369856673 ) ) ;
#36275=CARTESIAN_POINT ( 'NONE',  ( 78.44929255208916175, 53.32820552639820733, 15.80390961651161419 ) ) ;
#36277=CARTESIAN_POINT ( 'NONE',  ( 78.96891143551646053, 53.97097611525893512, -15.87805625008014943 ) ) ;
#36282=CARTESIAN_POINT ( 'NONE',  ( 84.38707503008889432, 50.04123336203296901, 13.82163251822127670 ) ) ;
#36290=CARTESIAN_POINT ( 'NONE',  ( 14.98925625915878079, 9.449665230724930254, -2.296566073217252530E-15 ) ) ;
#36297=CARTESIAN_POINT ( 'NONE',  ( 39.17063663036994114, 34.56628583063844928, 9.188101187500006262 ) ) ;
#36299=DIRECTION ( 'NONE',  ( 0.3978777116982076811, 0.7304723483372488335, -0.5550706935593547886 ) ) ;
#36300=CARTESIAN_POINT ( 'NONE',  ( 23.73493010604062192, 29.10171378149919974, 9.188101187500008038 ) ) ;
#36305=CARTESIAN_POINT ( 'NONE',  ( 67.53167658295855347, 67.09922345392760690, 8.942594108559754673 ) ) ;
#36311=CARTESIAN_POINT ( 'NONE',  ( 69.99818716782885986, 62.70504339187703380, 13.41613852849032362 ) ) ;
#36316=CARTESIAN_POINT ( 'NONE',  ( 82.90570422835274655, 41.17580535834989064, 0.2246636192497151185 ) ) ;
#36323=CARTESIAN_POINT ( 'NONE',  ( 13.78829669240011135, 8.364779650996389648, 1.583844403245363130 ) ) ;
#36328=CARTESIAN_POINT ( 'NONE',  ( 39.38594668318775405, 31.24335787977766188, -9.188101187500008038 ) ) ;
#36334=ORIENTED_EDGE ( 'NONE', *, *, #72781, .T. ) ;
#36336=CARTESIAN_POINT ( 'NONE',  ( 87.17963343274935539, 46.25680430639528140, -9.118192349661992324 ) ) ;
#36341=CARTESIAN_POINT ( 'NONE',  ( 78.94131938193116582, 59.19540273697393928, -16.19806489488007983 ) ) ;
#36344=CARTESIAN_POINT ( 'NONE',  ( 76.80517106979452535, 63.30872754350402687, -15.45635652541256455 ) ) ;
#36358=ORIENTED_EDGE ( 'NONE', *, *, #13240, .F. ) ;
#36363=DIRECTION ( 'NONE',  ( 0.000000000000000000, 0.4385670422228000742, -0.8986984752829754175 ) ) ;
#36367=CARTESIAN_POINT ( 'NONE',  ( 69.60454156778966706, 62.55713719731701161, -13.37071440263582112 ) ) ;
#36368=CARTESIAN_POINT ( 'NONE',  ( 67.86860378221429357, 65.58690806574966814, -10.91583492536020472 ) ) ;
#36371=CARTESIAN_POINT ( 'NONE',  ( 82.78345634833958400, 53.69061190982763776, 15.38144188222361386 ) ) ;
#36372=CARTESIAN_POINT ( 'NONE',  ( 82.56326814738740438, 40.91834736438271136, -3.675696166060102854 ) ) ;
#36373=EDGE_CURVE ( 'NONE', #18632, #34200, #10414, .T. ) ;
#36376=CARTESIAN_POINT ( 'NONE',  ( 72.06396613292808695, 72.31755342346831128, 3.440598478083111367 ) ) ;
#36384=CARTESIAN_POINT ( 'NONE',  ( 77.60205039494942980, 61.82655112718389034, 15.66204818029991941 ) ) ;
#36389=CARTESIAN_POINT ( 'NONE',  ( 66.86272913223326952, 69.17654172454702177, 0.7859538092876443560 ) ) ;
#36390=CARTESIAN_POINT ( 'NONE',  ( 73.37704433742356969, 70.12506801342537699, -9.398789138188929471 ) ) ;
#36391=FACE_OUTER_BOUND ( 'NONE', #91968, .T. ) ;
#36396=CARTESIAN_POINT ( 'NONE',  ( 72.06501183224497709, 72.04686745563701322, 2.871359202350765472 ) ) ;
#36402=CARTESIAN_POINT ( 'NONE',  ( 71.79363655647949827, 72.51690322118082577, -1.318798153274830076 ) ) ;
#36406=CARTESIAN_POINT ( 'NONE',  ( 17.13451663979182626, 31.93396525600390135, 2.839279412974139660 ) ) ;
#36409=CARTESIAN_POINT ( 'NONE',  ( 39.57658603661993624, 34.80066082961425877, 10.00000000000000533 ) ) ;
#36411=CARTESIAN_POINT ( 'NONE',  ( 78.05817343695024135, 58.35059340816943774, -16.56781068415745750 ) ) ;
#36414=CARTESIAN_POINT ( 'NONE',  ( 71.04687822819680321, 67.82841818693096059, -9.805517038057930179 ) ) ;
#36416=CARTESIAN_POINT ( 'NONE',  ( 82.37267291861169838, 41.27180535394074923, 3.277253532406301684 ) ) ;
#36417=CARTESIAN_POINT ( 'NONE',  ( 87.53583079710631409, 45.45925790797146249, -6.823327534849012110 ) ) ;
#36423=ORIENTED_EDGE ( 'NONE', *, *, #17236, .T. ) ;
#36430=CARTESIAN_POINT ( 'NONE',  ( 79.15324990756228374, 45.89422231479612435, -13.12042404536878237 ) ) ;
#36433=DIRECTION ( 'NONE',  ( -0.8660254037844378194, -0.5000000000000014433, -0.000000000000000000 ) ) ;
#36436=CARTESIAN_POINT ( 'NONE',  ( 27.42516030814983807, 18.76004757982090609, 5.678558825948272215 ) ) ;
#36437=CARTESIAN_POINT ( 'NONE',  ( 76.35345023940182330, 62.28244966075228461, 15.31341552635249137 ) ) ;
#36438=CARTESIAN_POINT ( 'NONE',  ( 70.44627411417100404, 70.20050130344810668, -5.575475040495237344 ) ) ;
#36447=EDGE_LOOP ( 'NONE', ( #26275, #47678, #52174, #10053 ) ) ;
#36448=ORIENTED_EDGE ( 'NONE', *, *, #41229, .F. ) ;
#36451=CARTESIAN_POINT ( 'NONE',  ( 70.07987635803645787, 71.18405689213730625, -3.399692208177651942 ) ) ;
#36452=CARTESIAN_POINT ( 'NONE',  ( 65.86595443870683653, 68.98825277307732051, -2.186046751764159080 ) ) ;
#36455=CARTESIAN_POINT ( 'NONE',  ( 81.83839218517164227, 55.52280113860526711, 16.29901351018851230 ) ) ;
#36475=CARTESIAN_POINT ( 'NONE',  ( 87.59998515009166908, 45.09196136326726645, 6.914658723149491593 ) ) ;
#36477=DIRECTION ( 'NONE',  ( 0.5295078238379054003, 0.5024823063053049932, 0.6834712842135706179 ) ) ;
#36479=CARTESIAN_POINT ( 'NONE',  ( 66.12762260262825009, 68.48100856943257497, -4.819680968675389643 ) ) ;
#36482=CARTESIAN_POINT ( 'NONE',  ( 76.14419419685665957, 51.07260177014754987, -15.57971481703006766 ) ) ;
#36484=B_SPLINE_CURVE_WITH_KNOTS ( 'NONE', 3,
 ( #83124, #12205, #73022, #12715, #96336, #59262, #3614, #44069 ),
 .UNSPECIFIED., .F., .F.,
 ( 4, 2, 2, 4 ),
 ( 0.4743034264391701171, 0.7371517132195847255, 0.8685758566097923072, 1.000000000000000000 ),
 .UNSPECIFIED. ) ;
#36485=CARTESIAN_POINT ( 'NONE',  ( 79.65227431844175499, 50.82673930868438816, 15.43633079355379145 ) ) ;
#36494=ORIENTED_EDGE ( 'NONE', *, *, #70780, .T. ) ;
#36495=CARTESIAN_POINT ( 'NONE',  ( 88.24246443646677562, 44.29974554292944333, 4.047255302186847814 ) ) ;
#36496=CARTESIAN_POINT ( 'NONE',  ( 85.22637764667558713, 43.33431299993616648, 4.849872636722851738 ) ) ;
#36499=CARTESIAN_POINT ( 'NONE',  ( 79.51018340840847998, 59.27997616101576028, -16.21944250808304133 ) ) ;
#36502=CARTESIAN_POINT ( 'NONE',  ( 76.17916984540215708, 53.15653679037458801, 15.96716164428893947 ) ) ;
#36505=CARTESIAN_POINT ( 'NONE',  ( 81.48851436888811861, 54.04920842346697896, 15.64857177594916315 ) ) ;
#36506=CARTESIAN_POINT ( 'NONE',  ( 73.71556180253553237, 69.43794663908232678, -9.869968096196300777 ) ) ;
#36508=CARTESIAN_POINT ( 'NONE',  ( 70.46332345186002044, 71.25533206547748932, 1.570548084703874858 ) ) ;
#36513=CARTESIAN_POINT ( 'NONE',  ( 21.14026940803790566, 27.90829794293880539, 10.00000000000000355 ) ) ;
#36518=CARTESIAN_POINT ( 'NONE',  ( 72.30516432241840619, 72.03273627914288113, -3.489044445822598650 ) ) ;
#36523=CARTESIAN_POINT ( 'NONE',  ( 67.14020853625015661, 67.74426869623036396, -6.533592144312494909 ) ) ;
#36527=CARTESIAN_POINT ( 'NONE',  ( 26.58620497985335973, 27.30066082961423035, -10.00000000000000533 ) ) ;
#36537=CARTESIAN_POINT ( 'NONE',  ( 42.68871737883920048, 29.81029122506298634, 8.090169943749479842 ) ) ;
#36542=CARTESIAN_POINT ( 'NONE',  ( 36.73494696561986217, 42.18502408145594984, 5.678558825948277544 ) ) ;
#36546=LINE ( 'NONE', #67453, #91386 ) ;
#36549=CARTESIAN_POINT ( 'NONE',  ( 11.28581492663933084, 21.91421378149917487, 9.188101187500008038 ) ) ;
#36551=CARTESIAN_POINT ( 'NONE',  ( 83.01487341893997041, 53.35419878647658720, 15.61608225115200987 ) ) ;
#36552=CARTESIAN_POINT ( 'NONE',  ( 72.97386446981147401, 70.68132344495337804, 8.316175787459499702 ) ) ;
#36557=CARTESIAN_POINT ( 'NONE',  ( 2.780145572064765425, 23.64646525600387506, -2.839279412974133887 ) ) ;
#36562=CARTESIAN_POINT ( 'NONE',  ( 66.66465390997532836, 68.91090369052673736, 2.096634673789778969 ) ) ;
#36563=LINE ( 'NONE', #44160, #93073 ) ;
#36570=ORIENTED_EDGE ( 'NONE', *, *, #19714, .T. ) ;
#36571=CARTESIAN_POINT ( 'NONE',  ( 88.42385336119198769, 44.01808410483894107, -2.342466917228906098 ) ) ;
#36572=CARTESIAN_POINT ( 'NONE',  ( 80.14460775109067470, 57.42271260518928244, -16.59269094194095473 ) ) ;
#36573=CARTESIAN_POINT ( 'NONE',  ( 28.94742091202107304, 40.21091486745862653, 7.012934429366973338E-14 ) ) ;
#36575=CARTESIAN_POINT ( 'NONE',  ( 87.27117856089937220, 44.98890866680353895, -6.231534082530021834 ) ) ;
#36577=CARTESIAN_POINT ( 'NONE',  ( 81.20226410207193624, 43.14699957628030802, 9.552668276955921911 ) ) ;
#36581=CARTESIAN_POINT ( 'NONE',  ( 74.34749166363997119, 62.52556080777176106, 14.76429959425114546 ) ) ;
#36587=CARTESIAN_POINT ( 'NONE',  ( 39.82000823235115661, 28.15404122711136736, 8.090169943749479842 ) ) ;
#36592=CARTESIAN_POINT ( 'NONE',  ( 73.27173416076851709, 69.81779851018656302, 9.109861862100318675 ) ) ;
#36595=CARTESIAN_POINT ( 'NONE',  ( 82.53276180672601470, 53.86864964727562466, 15.84768121842076916 ) ) ;
#36604=CARTESIAN_POINT ( 'NONE',  ( 67.31000428200415797, 66.58791411670934224, 8.576130451932648668 ) ) ;
#36606=CARTESIAN_POINT ( 'NONE',  ( 86.81972942635061941, 43.51551237735639432, 4.206298849977907039 ) ) ;
#36609=CARTESIAN_POINT ( 'NONE',  ( 80.43292161432816556, 52.70566313880177489, -15.44327005087032134 ) ) ;
#36611=CARTESIAN_POINT ( 'NONE',  ( 79.32679490348121476, 45.77422221639383082, 12.97016535827635408 ) ) ;
#36616=DIRECTION ( 'NONE',  ( 0.5000000000000014433, -0.8660254037844378194, 0.000000000000000000 ) ) ;
#36623=CYLINDRICAL_SURFACE ( 'NONE', #23968, 16.60714546451156792 ) ;
#36634=CARTESIAN_POINT ( 'NONE',  ( 76.61888230025124358, 51.35972145274618583, 16.07233720520855158 ) ) ;
#36635=CARTESIAN_POINT ( 'NONE',  ( 81.67228854796844928, 59.26376530784745711, -0.4806308479691611679 ) ) ;
#36642=ADVANCED_FACE ( 'NONE', ( #58564 ), #81422, .T. ) ;
#36643=CARTESIAN_POINT ( 'NONE',  ( 78.92023586790456591, 59.45316570216661489, -16.52216786098995982 ) ) ;
#36645=CARTESIAN_POINT ( 'NONE',  ( 80.57044917996766742, 47.48882946736131316, -13.61647149455460060 ) ) ;
#36649=CARTESIAN_POINT ( 'NONE',  ( 71.54138597657106402, 59.45382740952452849, -15.71570434403627914 ) ) ;
#36654=CARTESIAN_POINT ( 'NONE',  ( 70.08103292479646029, 69.71338913789749370, 6.159423539454167873 ) ) ;
#36661=CARTESIAN_POINT ( 'NONE',  ( 27.74991983456899902, 18.94754757982090254, 5.678558825948272215 ) ) ;
#36663=CARTESIAN_POINT ( 'NONE',  ( 87.97782240006738164, 43.76496563450898236, 2.369043524150744595 ) ) ;
#36667=CARTESIAN_POINT ( 'NONE',  ( 68.72121773276600720, 64.08709895911447063, 11.99045797092632526 ) ) ;
#36669=CARTESIAN_POINT ( 'NONE',  ( 80.04149297081583825, 46.93512272770157523, 13.46944761230850141 ) ) ;
#36672=CYLINDRICAL_SURFACE ( 'NONE', #15955, 16.60714546451156792 ) ;
#36675=DIRECTION ( 'NONE',  ( 0.3037402332698211915, 0.8935232438716343983, -0.3306933373297781809 ) ) ;
#36676=CARTESIAN_POINT ( 'NONE',  ( 84.07593154235651411, 41.67012449508333560, -3.184661558897835310 ) ) ;
#36678=EDGE_CURVE ( 'NONE', #50208, #93313, #41905, .T. ) ;
#36679=DIRECTION ( 'NONE',  ( -0.8660254037844377084, -0.5000000000000014433, -0.000000000000000000 ) ) ;
#36681=LINE ( 'NONE', #98520, #20234 ) ;
#36682=CARTESIAN_POINT ( 'NONE',  ( 67.29718787697062510, 68.46426409671040858, 5.180099965221677927 ) ) ;
#36686=CARTESIAN_POINT ( 'NONE',  ( 9.347034241948367850, 24.13478043621386604, 8.090169943749478065 ) ) ;
#36690=CARTESIAN_POINT ( 'NONE',  ( 86.47758924397189162, 47.47278051051635117, -10.96120693267980784 ) ) ;
#36691=CARTESIAN_POINT ( 'NONE',  ( 85.66574015724606284, 45.04611075343164117, -7.902063309705260608 ) ) ;
#36702=CARTESIAN_POINT ( 'NONE',  ( 73.24862708662814725, 69.62355710376385787, -9.916407523326116191 ) ) ;
#36705=EDGE_CURVE ( 'NONE', #84611, #7688, #77128, .T. ) ;
#36706=ORIENTED_EDGE ( 'NONE', *, *, #65851, .F. ) ;
#36709=CARTESIAN_POINT ( 'NONE',  ( 88.30697365647166919, 43.76017805630483792, 0.1929712240254211064 ) ) ;
#36711=CARTESIAN_POINT ( 'NONE',  ( 81.71781958264638490, 51.51165968475822865, 14.81913671552966782 ) ) ;
#36712=ORIENTED_EDGE ( 'NONE', *, *, #37351, .F. ) ;
#36713=CARTESIAN_POINT ( 'NONE',  ( 75.46810260959550476, 60.99596198493017596, 15.47750355691660928 ) ) ;
#36714=CARTESIAN_POINT ( 'NONE',  ( 87.89611104468033886, 44.97730679797474806, 6.346758332113888734 ) ) ;
#36721=CARTESIAN_POINT ( 'NONE',  ( 68.17914949951172332, 68.35117902963239089, -6.585394223376196621 ) ) ;
#36724=CARTESIAN_POINT ( 'NONE',  ( 66.10925264684654223, 68.74481801009629578, 0.07444925924169307208 ) ) ;
#36725=CARTESIAN_POINT ( 'NONE',  ( 7.128892988474023085, 19.51421378149916563, -9.188101187500004485 ) ) ;
#36726=ORIENTED_EDGE ( 'NONE', *, *, #8783, .F. ) ;
#36728=DIRECTION ( 'NONE',  ( -0.8660254037844378194, -0.5000000000000014433, -0.000000000000000000 ) ) ;
#36736=CARTESIAN_POINT ( 'NONE',  ( 84.19323161989967730, 41.93389703806564484, 0.8519107653881009545 ) ) ;
#36741=CARTESIAN_POINT ( 'NONE',  ( 71.33397847007799442, 63.32150720262168164, -13.53983176248328313 ) ) ;
#36748=CARTESIAN_POINT ( 'NONE',  ( 86.26929602985893553, 44.64143340914854718, -6.561271146724712011 ) ) ;
#36754=ORIENTED_EDGE ( 'NONE', *, *, #15155, .T. ) ;
#36759=CARTESIAN_POINT ( 'NONE',  ( 67.07192012151503491, 67.07552343309768617, -8.606452331924455024 ) ) ;
#36760=CARTESIAN_POINT ( 'NONE',  ( 20.28716687417668751, 35.21091486745861232, 7.012934429366973338E-14 ) ) ;
#36766=DIRECTION ( 'NONE',  ( -0.9634819383873037824, 0.2491829092639717136, 0.09803281150812255540 ) ) ;
#36768=ADVANCED_FACE ( 'NONE', ( #38621 ), #47232, .T. ) ;
#36776=CARTESIAN_POINT ( 'NONE',  ( 81.80713581745879992, 45.61783045263506864, 11.73987135276072280 ) ) ;
#36778=EDGE_CURVE ( 'NONE', #77944, #96074, #17693, .T. ) ;
#36779=CARTESIAN_POINT ( 'NONE',  ( 84.54065070028998718, 50.22889876405420040, 13.87834917160721737 ) ) ;
#36785=CARTESIAN_POINT ( 'NONE',  ( 84.14312167556933275, 48.98415679381830756, 0.000000000000000000 ) ) ;
#36787=CARTESIAN_POINT ( 'NONE',  ( 5.558032429380089567, 24.18502408145590010, 5.678558825948277544 ) ) ;
#36794=CARTESIAN_POINT ( 'NONE',  ( 45.07042791025775585, 28.94754757982093452, 5.678558825948272215 ) ) ;
#36796=DIRECTION ( 'NONE',  ( 0.5000000000000014433, -0.8660254037844378194, 0.000000000000000000 ) ) ;
#36798=CARTESIAN_POINT ( 'NONE',  ( 26.01786902700012405, 17.94754757982089899, 5.678558825948272215 ) ) ;
#36805=CARTESIAN_POINT ( 'NONE',  ( 70.42108267803217814, 60.99865500005843444, 14.93332735863378780 ) ) ;
#36810=EDGE_CURVE ( 'NONE', #58510, #55501, #44834, .T. ) ;
#36817=VERTEX_POINT ( 'NONE', #57614 ) ;
#36818=CARTESIAN_POINT ( 'NONE',  ( 87.92095387379619353, 44.55545140323351205, 4.092705293591274440 ) ) ;
#36823=ADVANCED_FACE ( 'NONE', ( #64741 ), #95051, .T. ) ;
#36830=CARTESIAN_POINT ( 'NONE',  ( 38.30580752471379213, 37.51421378149922958, -9.188101187500004485 ) ) ;
#36831=CARTESIAN_POINT ( 'NONE',  ( 78.59762652305811059, 58.68933280073064651, -16.17866137717102148 ) ) ;
#36832=EDGE_CURVE ( 'NONE', #62465, #94177, #87808, .T. ) ;
#36835=VERTEX_POINT ( 'NONE', #26212 ) ;
#36838=CARTESIAN_POINT ( 'NONE',  ( 87.23676543452685905, 46.07418070687454303, -8.827152287545313669 ) ) ;
#36844=CARTESIAN_POINT ( 'NONE',  ( 82.40498086807166089, 40.38612597002704518, 0.9999930885993705276 ) ) ;
#36845=VECTOR ( 'NONE', #97230, 1000.000000000000114 ) ;
#36847=CARTESIAN_POINT ( 'NONE',  ( 77.30322683057316624, 63.13261582766239854, -15.24451728302370235 ) ) ;
#36848=CARTESIAN_POINT ( 'NONE',  ( 78.89591602029014439, 59.68745106357756924, 16.49891905133565118 ) ) ;
#36851=CARTESIAN_POINT ( 'NONE',  ( 35.38177548881301249, 32.37878583063844218, 9.188101187500006262 ) ) ;
#36856=CARTESIAN_POINT ( 'NONE',  ( 74.21225604557145061, 68.54784490154126786, -11.57567064299385784 ) ) ;
#36858=B_SPLINE_SURFACE_WITH_KNOTS ( 'NONE', 3, 1, ( 
 ( #82866, #13439 ),
 ( #81862, #44305 ),
 ( #3353, #66122 ),
 ( #12439, #34229 ),
 ( #43306, #97071 ),
 ( #28613, #74253 ),
 ( #65124, #28116 ),
 ( #59497, #89959 ),
 ( #20538, #51417 ),
 ( #99034, #45305 ),
 ( #14424, #60491 ),
 ( #75733, #98541 ),
 ( #83858, #60994 ),
 ( #7305, #13920 ),
 ( #83354, #53887 ),
 ( #38186, #29131 ),
 ( #46282, #6318 ),
 ( #85352, #75235 ),
 ( #76240, #22011 ),
 ( #21525, #37695 ),
 ( #6814, #208 ),
 ( #84847, #69604 ),
 ( #44798, #37209 ),
 ( #92450, #68606 ),
 ( #99529, #52907 ),
 ( #68110, #29618 ),
 ( #30112, #59998 ),
 ( #91449, #52408 ),
 ( #91962, #5816 ),
 ( #22510, #69102 ),
 ( #90967, #53404 ) ),
 .UNSPECIFIED., .F., .F., .F.,
 ( 4, 3, 3, 3, 3, 3, 3, 3, 3, 3, 4 ),
 ( 2, 2 ),
 ( 0.000000000000000000, 0.1122669598086762227, 0.2243161639709647659, 0.3396355846219160091, 0.4553962076585160723, 0.5677860799922405111, 0.6749047109689648716, 0.7773884377078511543, 0.8775581155834262237, 0.9782364162378021089, 1.000000000000000000 ),
 ( 0.000000000000000000, 1.000000000000000000 ),
 .UNSPECIFIED. ) ;
#36861=CARTESIAN_POINT ( 'NONE',  ( 73.81768256443291421, 55.15394748217288878, -16.12362769555734943 ) ) ;
#36867=EDGE_LOOP ( 'NONE', ( #6928, #90987, #19374, #84015 ) ) ;
#36872=CARTESIAN_POINT ( 'NONE',  ( 83.12870697588047619, 46.63866199349129715, 11.37677525845150406 ) ) ;
#36880=CARTESIAN_POINT ( 'NONE',  ( 82.00520898190409014, 41.07855118830696028, -3.357997168065204541 ) ) ;
#36884=CARTESIAN_POINT ( 'NONE',  ( 84.20320819077289798, 44.90490820053396703, 8.816900774186109402 ) ) ;
#36886=CARTESIAN_POINT ( 'NONE',  ( 71.24663194959873636, 70.66145086035419354, -5.577829393062136099 ) ) ;
#36889=CARTESIAN_POINT ( 'NONE',  ( 77.82724693974202523, 61.74329194277088106, 16.06526602017299865 ) ) ;
#36893=CARTESIAN_POINT ( 'NONE',  ( 65.75540090923432501, 69.08964119695666284, -0.2331724888047134736 ) ) ;
#36894=CARTESIAN_POINT ( 'NONE',  ( 73.31376544620394498, 70.15701068496694859, -9.311920139903870464 ) ) ;
#36897=CARTESIAN_POINT ( 'NONE',  ( 45.44687632901609931, 27.20801979619932709, -3.090169943749474069 ) ) ;
#36899=CARTESIAN_POINT ( 'NONE',  ( 82.36286381532451628, 54.25719919591043805, 15.61971488265658792 ) ) ;
#36900=CARTESIAN_POINT ( 'NONE',  ( 71.83801353683954005, 72.23051172126305630, 3.257724734605899730 ) ) ;
#36901=ADVANCED_FACE ( 'NONE', ( #4396 ), #67187, .T. ) ;
#36905=CARTESIAN_POINT ( 'NONE',  ( 77.61091722901258549, 51.28954777400819864, -15.42868554443497153 ) ) ;
#36906=CARTESIAN_POINT ( 'NONE',  ( 71.68975264095180933, 72.03364086010030576, -1.589174013277645958 ) ) ;
#36909=CARTESIAN_POINT ( 'NONE',  ( 24.83368966200164607, 16.19860640527292261, 2.839279412974134775 ) ) ;
#36912=CARTESIAN_POINT ( 'NONE',  ( 46.58353466793526110, 27.86426979415093896, -3.090169943749474069 ) ) ;
#36916=VECTOR ( 'NONE', #98041, 1000.000000000000000 ) ;
#36918=CARTESIAN_POINT ( 'NONE',  ( 72.35426931885450585, 60.46654658139856053, 15.04702401992514282 ) ) ;
#36919=CARTESIAN_POINT ( 'NONE',  ( 71.29849878737984170, 67.80657138214567681, -10.00003097478887959 ) ) ;
#36936=CARTESIAN_POINT ( 'NONE',  ( 79.32306449657336600, 46.19060395113251616, -13.25186856088700615 ) ) ;
#36939=CARTESIAN_POINT ( 'NONE',  ( 86.84624261559693537, 44.08215787897474058, 5.733795036492094432 ) ) ;
#36942=CARTESIAN_POINT ( 'NONE',  ( 28.52090319329062851, 17.26216523072495690, -2.296566073217252530E-15 ) ) ;
#36943=CARTESIAN_POINT ( 'NONE',  ( 69.43213248134874505, 70.01719979072606748, -4.434620404520505765 ) ) ;
#36945=EDGE_CURVE ( 'NONE', #45639, #75490, #54606, .T. ) ;
#36949=ORIENTED_EDGE ( 'NONE', *, *, #14689, .F. ) ;
#36957=CARTESIAN_POINT ( 'NONE',  ( 81.66071111044179531, 55.73219010195405332, 16.34934455148813370 ) ) ;
#36963=CARTESIAN_POINT ( 'NONE',  ( 75.12366170154771794, 59.47066623895606341, -16.21752462648118964 ) ) ;
#36968=EDGE_LOOP ( 'NONE', ( #72749, #80, #91580, #48060 ) ) ;
#36970=CARTESIAN_POINT ( 'NONE',  ( 76.19402696226363503, 65.29190987809512592, 14.49924708549197128 ) ) ;
#36973=CARTESIAN_POINT ( 'NONE',  ( 83.61477352437640320, 42.16507195651136897, -5.583216967882105308 ) ) ;
#36974=CARTESIAN_POINT ( 'NONE',  ( 81.37395530686723077, 56.14341791244839186, 16.08471380636200365 ) ) ;
#36976=CARTESIAN_POINT ( 'NONE',  ( 72.80787385069068307, 70.05095376960370857, 8.379579475240937825 ) ) ;
#36977=CARTESIAN_POINT ( 'NONE',  ( 87.34977546134365411, 44.90968568749349288, 6.842696035241853103 ) ) ;
#36979=CARTESIAN_POINT ( 'NONE',  ( 16.25994779760268827, 31.16126292948894871, -6.180339887498951690 ) ) ;
#36983=ORIENTED_EDGE ( 'NONE', *, *, #54186, .T. ) ;
#36995=CARTESIAN_POINT ( 'NONE',  ( 88.26872550477153823, 44.38513711945522289, 4.282355379009171514 ) ) ;
#36996=CARTESIAN_POINT ( 'NONE',  ( 86.66434744208947905, 45.32692126891454620, 7.428864611774582905 ) ) ;
#36997=CARTESIAN_POINT ( 'NONE',  ( 80.16100348863038505, 44.92770494338710563, -11.28789370626155097 ) ) ;
#36998=CARTESIAN_POINT ( 'NONE',  ( 79.11723855630626190, 59.11194703662724237, -16.21433712332713029 ) ) ;
#36999=CARTESIAN_POINT ( 'NONE',  ( 74.02530730923707836, 66.66790563868377717, -12.50284404751719691 ) ) ;
#37004=CARTESIAN_POINT ( 'NONE',  ( 72.60568633014737827, 71.36030734738318415, -5.924380567679106591 ) ) ;
#37005=CARTESIAN_POINT ( 'NONE',  ( 81.53074493407929424, 54.33667322198162708, 15.71405181651475047 ) ) ;
#37013=EDGE_CURVE ( 'NONE', #22248, #59341, #27712, .T. ) ;
#37014=CARTESIAN_POINT ( 'NONE',  ( 26.80974344509558449, 15.28848085856231798, 1.475505719884397138E-15 ) ) ;
#37017=CARTESIAN_POINT ( 'NONE',  ( 26.55243232390424879, 15.73415679381822585, 1.333680081654574804E-15 ) ) ;
#37025=DIRECTION ( 'NONE',  ( -0.5000000000000014433, 0.8660254037844378194, 0.000000000000000000 ) ) ;
#37026=CARTESIAN_POINT ( 'NONE',  ( 72.69592421641888791, 70.74456683587563077, -7.971905174712497377 ) ) ;
#37031=CARTESIAN_POINT ( 'NONE',  ( 27.94640178401474273, 15.94473085651393340, 1.475505719884397138E-15 ) ) ;
#37032=CARTESIAN_POINT ( 'NONE',  ( 85.88643775857894980, 48.50416193104786799, 12.18167088616390537 ) ) ;
#37034=DIRECTION ( 'NONE',  ( 0.9659258262890695335, -0.2588190451025159655, 8.659560562354867531E-17 ) ) ;
#37039=CARTESIAN_POINT ( 'NONE',  ( 82.24832262017582707, 41.31296476174959764, 5.425068656990536198 ) ) ;
#37046=CARTESIAN_POINT ( 'NONE',  ( 39.71070620960689723, 31.43085787977766898, -9.188101187500008038 ) ) ;
#37055=CARTESIAN_POINT ( 'NONE',  ( 13.34565549823491004, 29.74646525600389424, 2.839279412974139660 ) ) ;
#37057=CARTESIAN_POINT ( 'NONE',  ( 71.44576612263118420, 59.19700591949954571, 15.27431131414821586 ) ) ;
#37063=CARTESIAN_POINT ( 'NONE',  ( 75.05139128669955539, 53.58935898396480724, -16.54232114207730930 ) ) ;
#37066=DIRECTION ( 'NONE',  ( -0.5000000000000013323, 0.8660254037844379305, 0.000000000000000000 ) ) ;
#37067=CARTESIAN_POINT ( 'NONE',  ( 68.67636306517070466, 70.25541593756011594, -0.5330109424154759745 ) ) ;
#37070=EDGE_LOOP ( 'NONE', ( #18921, #66390, #84222, #74508 ) ) ;
#37075=ORIENTED_EDGE ( 'NONE', *, *, #4862, .F. ) ;
#37076=CARTESIAN_POINT ( 'NONE',  ( 88.35080703960181836, 43.95228889933407856, -2.194260235337642140 ) ) ;
#37077=DIRECTION ( 'NONE',  ( 0.000000000000000000, 0.5247752241694969566, -0.8512408378936329179 ) ) ;
#37078=CARTESIAN_POINT ( 'NONE',  ( 80.37878231636271664, 58.00653726389809606, 16.25895090469026627 ) ) ;
#37079=CARTESIAN_POINT ( 'NONE',  ( 67.99156343939851865, 69.54710374710430187, -4.850653214453461537 ) ) ;
#37082=EDGE_CURVE ( 'NONE', #48590, #59818, #14102, .T. ) ;
#37086=EDGE_LOOP ( 'NONE', ( #40687, #23091, #67461, #2352 ) ) ;
#37097=CARTESIAN_POINT ( 'NONE',  ( 78.08015083193882333, 52.07315780664882254, -16.04342292210628784 ) ) ;
#37103=CARTESIAN_POINT ( 'NONE',  ( 66.10228174255657052, 68.64626758096548542, 4.271897712742705799 ) ) ;
#37107=CARTESIAN_POINT ( 'NONE',  ( 72.84093999290328725, 56.97456911652175648, -16.40692799624908815 ) ) ;
#37115=CARTESIAN_POINT ( 'NONE',  ( 79.62260391557677508, 45.88305127798363259, 12.92706424833072631 ) ) ;
#37121=CARTESIAN_POINT ( 'NONE',  ( 72.46567298678348834, 71.74231227323613780, 5.836615459846361098 ) ) ;
#37126=CARTESIAN_POINT ( 'NONE',  ( 88.02796755599807454, 43.59779901362369259, -1.172627947537940913E-07 ) ) ;
#37130=CARTESIAN_POINT ( 'NONE',  ( 75.84856439504059722, 51.76521084193598909, 15.76359423700355755 ) ) ;
#37133=CARTESIAN_POINT ( 'NONE',  ( 72.80948310655894318, 68.89414242203731931, 9.865878564760034664 ) ) ;
#37154=CARTESIAN_POINT ( 'NONE',  ( 13.24385365016830107, 12.81029122506292772, 8.090169943749479842 ) ) ;
#37161=CARTESIAN_POINT ( 'NONE',  ( 73.13293788966299758, 57.38693783170513996, 15.88898962805959947 ) ) ;
#37163=CARTESIAN_POINT ( 'NONE',  ( 66.31927393682876470, 68.07635084991424890, -4.657035190530372404 ) ) ;
#37164=( BOUNDED_CURVE ( )  B_SPLINE_CURVE ( 2, ( #18186, #10085, #63273, #40948, #24769, #34373, #3008, #71895, #25793, #94215, #11592, #49567, #25270 ),
 .UNSPECIFIED., .F., .T. ) 
 B_SPLINE_CURVE_WITH_KNOTS ( ( 3, 2, 2, 2, 2, 2, 3 ),
 ( 0.7125000000000000222, 0.7149999999999999689, 0.7199999999999999734, 0.7249999999999999778, 0.7299999999999999822, 0.7349999999999999867, 0.7375000000000000444 ),
 .UNSPECIFIED. ) 
 CURVE ( )  GEOMETRIC_REPRESENTATION_ITEM ( )  RATIONAL_B_SPLINE_CURVE ( ( 0.9755282581475767101, 0.9755282581475772652, 1.000000000000000000, 0.9510565162951535312, 1.000000000000000000, 0.9510565162951535312, 1.000000000000000000, 0.9510565162951535312, 1.000000000000000000, 0.9510565162951535312, 1.000000000000000000, 0.9755282581475761550, 0.9755282581475767101 ) ) 
 REPRESENTATION_ITEM ( '' )  );
#37169=CARTESIAN_POINT ( 'NONE',  ( 22.71615395846560759, 25.06628583063842086, -9.188101187500006262 ) ) ;
#37171=CARTESIAN_POINT ( 'NONE',  ( 83.61062943468348863, 51.62670160475642689, -14.84472182808584328 ) ) ;
#37173=CARTESIAN_POINT ( 'NONE',  ( 71.22741938756782076, 71.63657105851643792, 4.191086611024891440 ) ) ;
#37175=CARTESIAN_POINT ( 'NONE',  ( 68.92286145178795209, 64.34567850579628612, 12.51761414217151014 ) ) ;
#37181=CARTESIAN_POINT ( 'NONE',  ( 5.120201826081539842, 21.14336893147752861, 7.433330006724141015 ) ) ;
#37182=VERTEX_POINT ( 'NONE', #70679 ) ;
#37183=DIRECTION ( 'NONE',  ( 0.000000000000000000, 0.3470917258701589625, 0.9378311862123557274 ) ) ;
#37185=CARTESIAN_POINT ( 'NONE',  ( 75.46326934582160106, 53.27636971386139209, 16.49311846759427524 ) ) ;
#37189=CARTESIAN_POINT ( 'NONE',  ( 67.28342065528214277, 68.44788263265014905, 5.200797640023791857 ) ) ;
#37192=CARTESIAN_POINT ( 'NONE',  ( 7.599693759758306300, 26.16126292948893806, -6.180339887498951690 ) ) ;
#37196=CARTESIAN_POINT ( 'NONE',  ( 86.32721218574307898, 47.55264674982593931, -11.12316258729871699 ) ) ;
#37201=CARTESIAN_POINT ( 'NONE',  ( 79.04869528564927350, 60.22382082520471158, -16.44980649040591913 ) ) ;
#37204=CARTESIAN_POINT ( 'NONE',  ( 69.34550779939547738, 62.84827203527775197, 13.68706312608789410 ) ) ;
#37209=CARTESIAN_POINT ( 'NONE',  ( 81.47434785457708983, 42.60586634565555642, -7.670369333657699684 ) ) ;
#37211=EDGE_LOOP ( 'NONE', ( #82648, #51281, #28106, #78224 ) ) ;
#37213=CARTESIAN_POINT ( 'NONE',  ( 81.48310626213188357, 50.36142246172222769, 14.37505545833610654 ) ) ;
#37214=EDGE_LOOP ( 'NONE', ( #51649, #61984, #40811, #30154 ) ) ;
#37216=CARTESIAN_POINT ( 'NONE',  ( 68.92177428303565989, 69.37112163852187052, 5.346089011964235027 ) ) ;
#37220=CARTESIAN_POINT ( 'NONE',  ( 82.41510281465942001, 41.30975657737747753, 3.334936686815145546 ) ) ;
#37224=CARTESIAN_POINT ( 'NONE',  ( 70.54788803024760568, 68.42927960339889637, -8.732180548009763399 ) ) ;
#37228=CARTESIAN_POINT ( 'NONE',  ( 16.32921660555538423, 21.37878583063840310, 9.188101187500006262 ) ) ;
#37231=CARTESIAN_POINT ( 'NONE',  ( 80.28041774221068749, 57.81736701477464635, 16.60186235868146909 ) ) ;
#37237=CARTESIAN_POINT ( 'NONE',  ( 77.13638489036750912, 49.40795610031250362, -15.43467937247702793 ) ) ;
#37240=LINE ( 'NONE', #67644, #6208 ) ;
#37243=CARTESIAN_POINT ( 'NONE',  ( 69.30281931169795939, 63.72880281195976693, -12.52001448712189635 ) ) ;
#37249=CARTESIAN_POINT ( 'NONE',  ( 86.69791442786498692, 44.65922259563325269, -6.119518264180448419 ) ) ;
#37252=CARTESIAN_POINT ( 'NONE',  ( 76.16027975956328078, 65.34306562879338287, 14.46508190410747119 ) ) ;
#37255=ORIENTED_EDGE ( 'NONE', *, *, #69608, .T. ) ;
#37267=CARTESIAN_POINT ( 'NONE',  ( 65.96731655693133689, 68.98875292917840341, 2.536705629638577264 ) ) ;
#37268=VECTOR ( 'NONE', #49518, 1000.000000000000114 ) ;
#37281=CARTESIAN_POINT ( 'NONE',  ( 76.47316661484272515, 51.61210842333346704, -15.65491330287230376 ) ) ;
#37286=CARTESIAN_POINT ( 'NONE',  ( 5.010160986809694350, 24.93396525600388003, 2.839279412974139660 ) ) ;
#37289=CARTESIAN_POINT ( 'NONE',  ( 66.04604627343364598, 68.55213889972618801, 2.102432527703944842 ) ) ;
#37290=CARTESIAN_POINT ( 'NONE',  ( 82.10523990517461357, 41.85707133252695655, -5.529865280922476423 ) ) ;
#37296=ORIENTED_EDGE ( 'NONE', *, *, #68616, .F. ) ;
#37297=CARTESIAN_POINT ( 'NONE',  ( 22.00287929847174695, 28.10171378149919263, 9.188101187500008038 ) ) ;
#37301=CARTESIAN_POINT ( 'NONE',  ( 70.36883328969454965, 61.20268388249620273, 14.30258033183015520 ) ) ;
#37303=CARTESIAN_POINT ( 'NONE',  ( 73.97068428376778115, 60.66754191651645556, 15.78374986018236292 ) ) ;
#37305=CARTESIAN_POINT ( 'NONE',  ( 75.01560251667935120, 53.04709277412393220, -16.49609794243962213 ) ) ;
#37308=CARTESIAN_POINT ( 'NONE',  ( 73.06086572573603632, 69.73927861498383152, 9.650215327041465230 ) ) ;
#37309=ORIENTED_EDGE ( 'NONE', *, *, #41876, .F. ) ;
#37310=CARTESIAN_POINT ( 'NONE',  ( 66.30443171339169339, 68.57764064706508123, 4.834780342003228704 ) ) ;
#37314=CARTESIAN_POINT ( 'NONE',  ( 86.50731970396800818, 47.43598145919347786, -10.90780039058068063 ) ) ;
#37316=CARTESIAN_POINT ( 'NONE',  ( 85.04793144752866851, 49.76842598555752772, 13.42690168825988550 ) ) ;
#37319=EDGE_CURVE ( 'NONE', #84261, #42053, #61275, .T. ) ;
#37320=CARTESIAN_POINT ( 'NONE',  ( 43.36002773778349706, 27.96004757982094446, -5.678558825948275768 ) ) ;
#37321=CARTESIAN_POINT ( 'NONE',  ( 81.62004238798716926, 55.61031524971931361, -16.33394531952002637 ) ) ;
#37324=CARTESIAN_POINT ( 'NONE',  ( 87.52763816747332726, 45.51472861705721584, 6.966552648612967857 ) ) ;
#37327=CARTESIAN_POINT ( 'NONE',  ( 72.12695820614409570, 72.30325941021428093, -1.374247448237438718 ) ) ;
#37333=CARTESIAN_POINT ( 'NONE',  ( 75.58192994435955825, 60.58255967155832877, -15.61553270740560961 ) ) ;
#37342=CARTESIAN_POINT ( 'NONE',  ( 40.57792791151964451, 35.37878583063844218, 9.188101187500006262 ) ) ;
#37344=ORIENTED_EDGE ( 'NONE', *, *, #47287, .T. ) ;
#37345=ADVANCED_FACE ( 'NONE', ( #73200 ), #74207, .T. ) ;
#37350=CARTESIAN_POINT ( 'NONE',  ( 17.92595094200897776, 22.30066082961421259, -10.00000000000000533 ) ) ;
#37351=EDGE_CURVE ( 'NONE', #77062, #6177, #3311, .T. ) ;
#37355=ORIENTED_EDGE ( 'NONE', *, *, #75270, .T. ) ;
#37361=CARTESIAN_POINT ( 'NONE',  ( 67.57228314452760287, 68.96594721286149365, -4.233564566667188167 ) ) ;
#37365=ORIENTED_EDGE ( 'NONE', *, *, #52092, .F. ) ;
#37368=EDGE_CURVE ( 'NONE', #96468, #71854, #58945, .T. ) ;
#37372=CARTESIAN_POINT ( 'NONE',  ( 71.74723311883084875, 72.17470677413867008, 3.272391839458885343 ) ) ;
#37377=CARTESIAN_POINT ( 'NONE',  ( 82.62542648728522465, 54.14492212412226024, -15.90696914271029883 ) ) ;
#37380=CARTESIAN_POINT ( 'NONE',  ( 77.87494449001893315, 61.77424058857110367, 16.06449337301376090 ) ) ;
#37385=CARTESIAN_POINT ( 'NONE',  ( 73.68336374684922419, 69.35704589951700427, -9.943571445751130611 ) ) ;
#37390=CARTESIAN_POINT ( 'NONE',  ( 42.07167428219069905, 29.45404122711137163, -8.090169943749478065 ) ) ;
#37391=CARTESIAN_POINT ( 'NONE',  ( 74.63183655046933040, 58.04581334265427728, -16.40266346922720686 ) ) ;
#37392=CARTESIAN_POINT ( 'NONE',  ( 82.50768696284946202, 54.20953915494273190, 15.58343736883158037 ) ) ;
#37393=CARTESIAN_POINT ( 'NONE',  ( 71.99480943628985585, 72.01367526706704325, 2.839808199187065174 ) ) ;
#37397=CARTESIAN_POINT ( 'NONE',  ( 77.00202394376545101, 51.46254985920837299, -15.55718584050375597 ) ) ;
#37398=CARTESIAN_POINT ( 'NONE',  ( 71.94004515418134815, 72.62285878051592647, -1.062404765500833070 ) ) ;
#37400=CARTESIAN_POINT ( 'NONE',  ( 28.09632999608277615, 19.14754757982091604, -5.678558825948275768 ) ) ;
#37403=CARTESIAN_POINT ( 'NONE',  ( 4.600586583810874153, 20.84336893147753500, -7.433330006724137462 ) ) ;
#37404=CARTESIAN_POINT ( 'NONE',  ( 64.77737111682259297, 68.52662068827328312, 2.033788753608857291E-15 ) ) ;
#37405=CARTESIAN_POINT ( 'NONE',  ( 76.65021695619097386, 63.83748121254656382, 14.86493802743865977 ) ) ;
#37408=CARTESIAN_POINT ( 'NONE',  ( 72.27530749108618124, 60.16728400709956759, 15.12809549573886514 ) ) ;
#37411=CARTESIAN_POINT ( 'NONE',  ( 73.12133584826474930, 57.41764960941905116, -15.88333458976553381 ) ) ;
#37423=CARTESIAN_POINT ( 'NONE',  ( 79.15951963630969601, 45.96312243709959944, -13.16404013888753433 ) ) ;
#37425=CARTESIAN_POINT ( 'NONE',  ( 72.67905965592419193, 70.26320000030698054, -8.002569769838684621 ) ) ;
#37428=CARTESIAN_POINT ( 'NONE',  ( 18.36860284018464995, 32.64646525600389992, -2.839279412974133887 ) ) ;
#37429=CARTESIAN_POINT ( 'NONE',  ( 75.11677177402179950, 55.37571795895599536, 16.15001063157648176 ) ) ;
#37430=CARTESIAN_POINT ( 'NONE',  ( 68.66514842125685902, 69.81561067240546947, -3.556167530028313983 ) ) ;
#37431=CARTESIAN_POINT ( 'NONE',  ( 75.07659682177997240, 67.19019193167021342, -13.02721601185334244 ) ) ;
#37432=ORIENTED_EDGE ( 'NONE', *, *, #51816, .F. ) ;
#37437=CARTESIAN_POINT ( 'NONE',  ( 78.89069071477848638, 50.23289766025146008, -14.88438564644514805 ) ) ;
#37443=CARTESIAN_POINT ( 'NONE',  ( 81.87367770298098435, 58.91494905927235948, -0.4240240480782126453 ) ) ;
#37450=ORIENTED_EDGE ( 'NONE', *, *, #19591, .F. ) ;
#37452=CARTESIAN_POINT ( 'NONE',  ( 79.15982281496793860, 45.83852568395352023, 13.08051851333009807 ) ) ;
#37456=ORIENTED_EDGE ( 'NONE', *, *, #6965, .T. ) ;
#37458=CARTESIAN_POINT ( 'NONE',  ( 79.97565766777488250, 44.45602524408276679, -10.96263857390526120 ) ) ;
#37461=DIRECTION ( 'NONE',  ( -0.8660254037844378194, -0.5000000000000013323, -0.000000000000000000 ) ) ;
#37463=CARTESIAN_POINT ( 'NONE',  ( 81.19855876245502202, 56.17955710756607601, 16.10481241976900080 ) ) ;
#37464=LINE ( 'NONE', #91716, #25675 ) ;
#37466=CARTESIAN_POINT ( 'NONE',  ( 72.25937237857473860, 68.78397272217405600, 9.561999692830665865 ) ) ;
#37478=ORIENTED_EDGE ( 'NONE', *, *, #33849, .F. ) ;
#37479=CARTESIAN_POINT ( 'NONE',  ( 87.90883736606430432, 44.33697863951398688, 4.769790285073534086 ) ) ;
#37480=CARTESIAN_POINT ( 'NONE',  ( 70.33155363901632029, 67.77084087856721339, -10.11489276010222582 ) ) ;
#37481=CARTESIAN_POINT ( 'NONE',  ( 80.09120749856197108, 44.41673742825524585, -10.86461196121644157 ) ) ;
#37483=CARTESIAN_POINT ( 'NONE',  ( 72.98735915780690675, 70.85324004147126686, 8.065790162528031715 ) ) ;
#37484=VECTOR ( 'NONE', #90579, 1000.000000000000114 ) ;
#37485=CARTESIAN_POINT ( 'NONE',  ( 68.15993400338558672, 67.42531444003920171, -8.116946311972593975 ) ) ;
#37491=CARTESIAN_POINT ( 'NONE',  ( 80.20727400250618189, 48.45000011746393653, 13.73562201919597214 ) ) ;
#37492=CARTESIAN_POINT ( 'NONE',  ( 73.69590563849025955, 69.38244366243233685, -9.922201517543204119 ) ) ;
#37501=FACE_BOUND ( 'NONE', #71742, .T. ) ;
#37504=CARTESIAN_POINT ( 'NONE',  ( 20.07045957425421534, 33.36126292948895866, 6.180339887498949913 ) ) ;
#37514=CARTESIAN_POINT ( 'NONE',  ( 72.86116454657229724, 70.29466190917024448, -8.120416833897904141 ) ) ;
#37519=CARTESIAN_POINT ( 'NONE',  ( 30.23324123896446736, 19.58380873178788306, 6.180339887498953466 ) ) ;
#37520=CARTESIAN_POINT ( 'NONE',  ( 85.32371827457656366, 48.49939495466653483, 12.43282873216696593 ) ) ;
#37522=CARTESIAN_POINT ( 'NONE',  ( 71.71105958810139214, 72.07721142573539908, -3.586786881503329472 ) ) ;
#37531=CARTESIAN_POINT ( 'NONE',  ( 72.77745277708220328, 70.81288354178651900, -7.938184674006802943 ) ) ;
#37534=CARTESIAN_POINT ( 'NONE',  ( 40.90268743793880901, 35.56628583063844218, 9.188101187500006262 ) ) ;
#37538=B_SPLINE_CURVE_WITH_KNOTS ( 'NONE', 3,
 ( #69321, #16617, #94161, #85580, #55106, #31803, #70313, #9021, #94660, #62704 ),
 .UNSPECIFIED., .F., .F.,
 ( 4, 2, 2, 2, 4 ),
 ( 0.000000000000000000, 0.0002622400424273363395, 0.0005244800848546726790, 0.0007867201272820090185, 0.001048960169709345358 ),
 .UNSPECIFIED. ) ;
#37541=CARTESIAN_POINT ( 'NONE',  ( 12.16147613323643029, 27.99752408145590721, 5.678558825948277544 ) ) ;
#37543=CARTESIAN_POINT ( 'NONE',  ( 71.96630278948212833, 59.14415382642645369, 15.37175206046237008 ) ) ;
#37548=CARTESIAN_POINT ( 'NONE',  ( 88.23709331947554801, 44.35306696108359148, 2.575362715384265311 ) ) ;
#37549=VERTEX_POINT ( 'NONE', #3680 ) ;
#37550=CARTESIAN_POINT ( 'NONE',  ( 15.68640692011977222, 32.55466486950700045, -1.111400068045478839E-16 ) ) ;
#37552=CARTESIAN_POINT ( 'NONE',  ( 72.50785297705053267, 57.43012539693897622, 16.30925143403899824 ) ) ;
#37561=CARTESIAN_POINT ( 'NONE',  ( 80.36956643484273854, 57.45342863445996784, -16.58888403658913901 ) ) ;
#37563=ORIENTED_EDGE ( 'NONE', *, *, #29918, .F. ) ;
#37569=CARTESIAN_POINT ( 'NONE',  ( 74.41414138846958792, 62.82147636634939403, 14.66719177346846159 ) ) ;
#37577=CARTESIAN_POINT ( 'NONE',  ( 78.41477381122238910, 47.32040575024743134, -14.22103711499937617 ) ) ;
#37582=CARTESIAN_POINT ( 'NONE',  ( 73.53833585859590016, 69.81206169144661544, 9.302004287366802515 ) ) ;
#37583=LINE ( 'NONE', #7189, #26993 ) ;
#37595=CARTESIAN_POINT ( 'NONE',  ( 67.13624854745103221, 66.75749375781143158, 8.200433981937235828 ) ) ;
#37597=CARTESIAN_POINT ( 'NONE',  ( 78.48434347618606921, 47.42827226539994712, 14.25623586707808066 ) ) ;
#37601=CARTESIAN_POINT ( 'NONE',  ( 72.18576721375995930, 69.97445003978347700, 7.973227091533599875 ) ) ;
#37603=CARTESIAN_POINT ( 'NONE',  ( 87.11349487006070547, 46.19076519147612458, 8.411924245371466213 ) ) ;
#37605=CARTESIAN_POINT ( 'NONE',  ( 83.66208585045004043, 52.31085355490836264, -15.11568120807085336 ) ) ;
#37611=CARTESIAN_POINT ( 'NONE',  ( 79.14312167556931854, 57.64441083166269664, 0.000000000000000000 ) ) ;
#37615=VECTOR ( 'NONE', #26427, 1000.000000000000000 ) ;
#37628=DIRECTION ( 'NONE',  ( 0.5000000000000014433, -0.8660254037844378194, 0.000000000000000000 ) ) ;
#37637=CARTESIAN_POINT ( 'NONE',  ( 8.420521286406055239, 20.56454794089038884, 10.00000000000000355 ) ) ;
#37639=CARTESIAN_POINT ( 'NONE',  ( 71.71174882295490249, 58.93038559433049528, -15.88944412498251602 ) ) ;
#37644=CARTESIAN_POINT ( 'NONE',  ( 72.56871628006966546, 57.25199919244864333, 16.34355953453273003 ) ) ;
#37645=CARTESIAN_POINT ( 'NONE',  ( 71.34022676192449808, 69.59814005368316714, 8.523861822075398109 ) ) ;
#37646=CARTESIAN_POINT ( 'NONE',  ( 66.24005707684722211, 68.70828816332591771, -4.328508583860865677 ) ) ;
#37653=CARTESIAN_POINT ( 'NONE',  ( 27.11724708220625857, 33.84336893147757763, -7.433330006724137462 ) ) ;
#37659=CARTESIAN_POINT ( 'NONE',  ( 68.89365374505190687, 64.32635024170694749, 12.51947484636856345 ) ) ;
#37661=CARTESIAN_POINT ( 'NONE',  ( 88.19053702688614749, 44.32527345396092500, -2.493626234014364673 ) ) ;
#37664=AXIS2_PLACEMENT_3D ( 'NONE', #42750, #72714, #3303 ) ;
#37669=DIRECTION ( 'NONE',  ( -0.4635919272833941562, 0.8029647720336182681, 0.3746065934159032440 ) ) ;
#37674=DIRECTION ( 'NONE',  ( -0.8116583814955237175, -0.01378320505841506768, -0.5839697723396174434 ) ) ;
#37678=CARTESIAN_POINT ( 'NONE',  ( 17.82296297622643166, 15.45404122711132544, -8.090169943749478065 ) ) ;
#37679=CARTESIAN_POINT ( 'NONE',  ( 73.04277380876573034, 70.56196896876862468, 7.835544939490341143 ) ) ;
#37680=VERTEX_POINT ( 'NONE', #54 ) ;
#37682=CARTESIAN_POINT ( 'NONE',  ( 86.52979389935374854, 47.15173288509246419, -10.60481917042621802 ) ) ;
#37683=CARTESIAN_POINT ( 'NONE',  ( 79.27712787825650764, 45.82676469203064329, -12.41914995154098911 ) ) ;
#37686=CARTESIAN_POINT ( 'NONE',  ( 79.18418104304700478, 60.10533407485777957, -16.47260471942690074 ) ) ;
#37690=CARTESIAN_POINT ( 'NONE',  ( 69.47282375568661905, 62.69533200737101453, 13.81976147870238592 ) ) ;
#37695=CARTESIAN_POINT ( 'NONE',  ( 81.38072385067304992, 42.55310844818403382, -7.672405682984796194 ) ) ;
#37696=B_SPLINE_SURFACE_WITH_KNOTS ( 'NONE', 3, 1, ( 
 ( #94565, #31221 ),
 ( #33228, #25123 ),
 ( #24131, #56525 ),
 ( #87513, #62107 ),
 ( #24623, #93055 ),
 ( #64132, #86999 ),
 ( #85998, #93564 ),
 ( #45054, #23609 ),
 ( #70729, #56004 ),
 ( #78853, #16028 ),
 ( #17527, #8435 ),
 ( #48434, #39303 ),
 ( #70220, #827 ),
 ( #79382, #32225 ),
 ( #31706, #86493 ),
 ( #62611, #55018 ),
 ( #9435, #17020 ),
 ( #40310, #71249 ),
 ( #16525, #39797 ),
 ( #47422, #63128 ),
 ( #78347, #63628 ),
 ( #1843, #9945 ),
 ( #40807, #4218 ),
 ( #51303, #49335 ),
 ( #80786, #73151 ),
 ( #20435, #27542 ),
 ( #35116, #74145 ),
 ( #26045, #89387 ),
 ( #87903, #95980 ),
 ( #26542, #11360 ),
 ( #18446, #80275 ) ),
 .UNSPECIFIED., .F., .F., .F.,
 ( 4, 3, 3, 3, 3, 3, 3, 3, 3, 3, 4 ),
 ( 2, 2 ),
 ( 0.000000000000000000, 0.1122669598086934867, 0.2243161639709926047, 0.3396355846219420438, 0.4553962076585420515, 0.5677860799922670454, 0.6749047109689817470, 0.7773884377078588148, 0.8775581155834574210, 0.9782364162378296424, 1.000000000000000000 ),
 ( 0.000000000000000000, 1.000000000000000000 ),
 .UNSPECIFIED. ) ;
#37704=CARTESIAN_POINT ( 'NONE',  ( 68.73406594905847555, 69.12949821581069898, 5.652800877584020611 ) ) ;
#37711=CARTESIAN_POINT ( 'NONE',  ( 82.87668018738534670, 53.58938331343419748, -15.34904665510062571 ) ) ;
#37713=CARTESIAN_POINT ( 'NONE',  ( 18.60133699236122595, 19.24335787977762990, -9.188101187500008038 ) ) ;
#37720=CARTESIAN_POINT ( 'NONE',  ( 79.85280895619634123, 44.70080194145975128, 11.24692901854433735 ) ) ;
#37728=CARTESIAN_POINT ( 'NONE',  ( 74.81832046901196520, 67.48663194201290594, -12.71244991431774984 ) ) ;
#37735=CARTESIAN_POINT ( 'NONE',  ( 84.47504870052041781, 44.63565290773180294, -8.224897521149806323 ) ) ;
#37736=CARTESIAN_POINT ( 'NONE',  ( 72.99830029227618411, 70.81959382475521636, 8.127746218293800951 ) ) ;
#37738=CARTESIAN_POINT ( 'NONE',  ( 27.37565231528585841, 31.50829794293882102, -10.00000000000000355 ) ) ;
#37744=CARTESIAN_POINT ( 'NONE',  ( 79.14312167556931854, 57.64441083166269664, 0.000000000000000000 ) ) ;
#37746=( BOUNDED_CURVE ( )  B_SPLINE_CURVE ( 2, ( #99981, #30564, #32040, #47250, #54847, #79704, #86314, #71076, #24456, #17351, #94395, #80202, #64460 ),
 .UNSPECIFIED., .F., .T. ) 
 B_SPLINE_CURVE_WITH_KNOTS ( ( 3, 2, 2, 2, 2, 2, 3 ),
 ( 0.03750000000000000555, 0.04000000000000000083, 0.04499999999999999833, 0.05000000000000000278, 0.05500000000000000028, 0.05999999999999999778, 0.06250000000000000000 ),
 .UNSPECIFIED. ) 
 CURVE ( )  GEOMETRIC_REPRESENTATION_ITEM ( )  RATIONAL_B_SPLINE_CURVE ( ( 0.9755282581475768211, 0.9755282581475768211, 1.000000000000000000, 0.9510565162951535312, 1.000000000000000000, 0.9510565162951535312, 1.000000000000000000, 0.9510565162951535312, 1.000000000000000000, 0.9510565162951535312, 1.000000000000000000, 0.9755282581475768211, 0.9755282581475768211 ) ) 
 REPRESENTATION_ITEM ( '' )  );
#37748=CARTESIAN_POINT ( 'NONE',  ( 85.38646193529683615, 42.60607428054889567, 1.234017145255211112 ) ) ;
#37750=CARTESIAN_POINT ( 'NONE',  ( 84.88791182130400159, 48.20836502411282254, 11.92161542626550208 ) ) ;
#37765=CARTESIAN_POINT ( 'NONE',  ( 83.24292249771293939, 50.82510919314466236, 14.58399313936658537 ) ) ;
#37768=CARTESIAN_POINT ( 'NONE',  ( 70.09710780656028817, 70.29879786405263076, 4.725240580867070328 ) ) ;
#37770=FACE_OUTER_BOUND ( 'NONE', #15618, .T. ) ;
#37771=ORIENTED_EDGE ( 'NONE', *, *, #29502, .T. ) ;
#37778=DIRECTION ( 'NONE',  ( -0.8660254037844377084, -0.5000000000000014433, -0.000000000000000000 ) ) ;
#37784=CARTESIAN_POINT ( 'NONE',  ( 37.50955192761952617, 39.84336893147759184, -7.433330006724137462 ) ) ;
#37788=CARTESIAN_POINT ( 'NONE',  ( 26.50621139815081762, 30.70171378149920471, -9.188101187500004485 ) ) ;
#37789=CARTESIAN_POINT ( 'NONE',  ( 80.74781574657599492, 57.21644485803225422, 16.56566952311892749 ) ) ;
#37793=CARTESIAN_POINT ( 'NONE',  ( 70.89420290055875284, 60.93121495745884175, 14.54576430277729315 ) ) ;
#37798=ORIENTED_EDGE ( 'NONE', *, *, #65619, .T. ) ;
#37799=CARTESIAN_POINT ( 'NONE',  ( 73.03023235113748513, 69.68176590430279305, 9.698330045464274463 ) ) ;
#37800=CARTESIAN_POINT ( 'NONE',  ( 35.22902474502244274, 28.84335787977765619, 9.188101187500006262 ) ) ;
#37805=CARTESIAN_POINT ( 'NONE',  ( 86.40784109447328376, 47.52432272822921533, -11.05097720836334396 ) ) ;
#37811=CARTESIAN_POINT ( 'NONE',  ( 34.24030602833327208, 37.95586893147758900, 7.433330006724141015 ) ) ;
#37819=ORIENTED_EDGE ( 'NONE', *, *, #60128, .T. ) ;
#37821=CARTESIAN_POINT ( 'NONE',  ( 87.11842579636694950, 45.87328929624024454, -8.641498891285833039 ) ) ;
#37828=CARTESIAN_POINT ( 'NONE',  ( 82.08231906242987463, 40.78080646243900276, 1.383867760887848020 ) ) ;
#37831=CARTESIAN_POINT ( 'NONE',  ( 77.30991866800115986, 63.26798366544798569, -15.19874235486285663 ) ) ;
#37837=CARTESIAN_POINT ( 'NONE',  ( 36.57375671714491006, 36.51421378149921537, -9.188101187500004485 ) ) ;
#37840=CARTESIAN_POINT ( 'NONE',  ( 74.07678436671264421, 68.35284689741969544, -11.67875583378132198 ) ) ;
#37857=VERTEX_POINT ( 'NONE', #30938 ) ;
#37859=CARTESIAN_POINT ( 'NONE',  ( 73.55941717774605593, 69.21675373535786946, 9.988905871803112291 ) ) ;
#37863=CARTESIAN_POINT ( 'NONE',  ( 72.13517842779845068, 72.31474564102330760, 3.615969315562336472 ) ) ;
#37864=CARTESIAN_POINT ( 'NONE',  ( 31.23047667836735641, 41.52903772873361277, -1.583844403245329602 ) ) ;
#37868=CARTESIAN_POINT ( 'NONE',  ( 82.75828967192548191, 53.74568045750391576, -15.77735475420663569 ) ) ;
#37876=CARTESIAN_POINT ( 'NONE',  ( 73.32220977704777454, 69.17604616796300832, -9.911163241522066514 ) ) ;
#37877=CARTESIAN_POINT ( 'NONE',  ( 76.46903462498934800, 51.53433314985417013, 15.63818393615307478 ) ) ;
#37882=CARTESIAN_POINT ( 'NONE',  ( 72.21694820471849141, 72.08926726930118889, 3.059610661676269050 ) ) ;
#37885=EDGE_CURVE ( 'NONE', #80464, #65643, #4017, .T. ) ;
#37889=CARTESIAN_POINT ( 'NONE',  ( 81.35748880148537410, 42.22347387491733173, -7.155507324468848296 ) ) ;
#37890=CARTESIAN_POINT ( 'NONE',  ( 78.83097366254324356, 50.94081823793872132, -15.13050861895527177 ) ) ;
#37893=CARTESIAN_POINT ( 'NONE',  ( 23.58217936225004863, 25.56628583063841376, 9.188101187500006262 ) ) ;
#37896=CARTESIAN_POINT ( 'NONE',  ( 8.675723883004062387, 25.98502408145591147, -5.678558825948271327 ) ) ;
#37898=CARTESIAN_POINT ( 'NONE',  ( 76.88601853014658616, 63.69663891124154276, 15.33692311465240543 ) ) ;
#37909=CARTESIAN_POINT ( 'NONE',  ( 77.19879077027466963, 49.27944484189550423, 15.37723906343501490 ) ) ;
#37910=ORIENTED_EDGE ( 'NONE', *, *, #32301, .T. ) ;
#37918=CARTESIAN_POINT ( 'NONE',  ( 85.22469180575973269, 42.26411194152829154, 2.911061958177603604 ) ) ;
#37920=CARTESIAN_POINT ( 'NONE',  ( 18.54180792094154029, 32.74646525600390135, 2.839279412974139660 ) ) ;
#37921=CARTESIAN_POINT ( 'NONE',  ( 67.55733782939270782, 69.42818843681499175, -2.263445650850663515 ) ) ;
#37926=FACE_OUTER_BOUND ( 'NONE', #72010, .T. ) ;
#37932=CARTESIAN_POINT ( 'NONE',  ( 67.83594148062915963, 65.58978118587256745, -10.89425741029403305 ) ) ;
#37952=CARTESIAN_POINT ( 'NONE',  ( 67.15620270673211678, 67.72793565538280802, 6.583466307750684976 ) ) ;
#37953=EDGE_CURVE ( 'NONE', #12155, #83087, #33965, .T. ) ;
#37956=CARTESIAN_POINT ( 'NONE',  ( 68.10741622413405594, 65.45592947349832968, 10.45487064772517982 ) ) ;
#37959=CARTESIAN_POINT ( 'NONE',  ( 87.45543461181301836, 45.01664465679171201, 6.930016242323786990 ) ) ;
#37965=CARTESIAN_POINT ( 'NONE',  ( 76.18264033726677553, 51.55645319538977134, -15.67776776688645235 ) ) ;
#37967=FACE_OUTER_BOUND ( 'NONE', #61146, .T. ) ;
#37974=CARTESIAN_POINT ( 'NONE',  ( 87.95576658732893804, 44.05533438356886222, -1.735394378949605576 ) ) ;
#37977=CARTESIAN_POINT ( 'NONE',  ( 67.94548261240784370, 67.41770141102237801, -7.935486469137003951 ) ) ;
#37982=CARTESIAN_POINT ( 'NONE',  ( 80.24293753902323090, 48.56639400389035899, 13.78793733260431331 ) ) ;
#37983=CARTESIAN_POINT ( 'NONE',  ( 83.82185059330514321, 51.95230014857058620, 14.93193377595572002 ) ) ;
#37986=DIRECTION ( 'NONE',  ( -0.3473291852295006810, 0.6015917957689992379, 0.7193398003386451967 ) ) ;
#37994=CARTESIAN_POINT ( 'NONE',  ( 24.75116620650193866, 19.45404122711133965, -8.090169943749478065 ) ) ;
#38001=ORIENTED_EDGE ( 'NONE', *, *, #31161, .T. ) ;
#38003=CARTESIAN_POINT ( 'NONE',  ( 66.89604841441746430, 67.64130223492367122, -6.456890807137734889 ) ) ;
#38004=CARTESIAN_POINT ( 'NONE',  ( 73.02740203026323229, 70.73066625390264051, -7.556326162255497358 ) ) ;
#38007=CARTESIAN_POINT ( 'NONE',  ( 29.08982151148960682, 17.76426979415090912, 3.090169943749476733 ) ) ;
#38008=CARTESIAN_POINT ( 'NONE',  ( 83.48029009741895834, 41.89032089958049454, -3.321841928985223902 ) ) ;
#38021=CARTESIAN_POINT ( 'NONE',  ( 72.45751905151223582, 70.67373443742413031, -7.865264308201658672 ) ) ;
#38023=CARTESIAN_POINT ( 'NONE',  ( 44.29582294825809896, 31.28920272979930672, -7.433330006724141015 ) ) ;
#38025=AXIS2_PLACEMENT_3D ( 'NONE', #15475, #54985, #1303 ) ;
#38031=CARTESIAN_POINT ( 'NONE',  ( 15.62557774837418023, 29.99752408145591076, 5.678558825948277544 ) ) ;
#38033=CARTESIAN_POINT ( 'NONE',  ( 71.62614020371384527, 59.05562564738432485, 15.84271347433855937 ) ) ;
#38035=VERTEX_POINT ( 'NONE', #44009 ) ;
#38038=CARTESIAN_POINT ( 'NONE',  ( 75.30812353949326621, 53.54509013300328490, -16.04758382930608462 ) ) ;
#38042=CYLINDRICAL_SURFACE ( 'NONE', #68409, 16.60714546451156792 ) ;
#38043=CARTESIAN_POINT ( 'NONE',  ( 70.87177484439632735, 71.18736215039216120, -3.328809516792729628 ) ) ;
#38044=CARTESIAN_POINT ( 'NONE',  ( 76.54127139839069116, 63.71106849112843662, 14.88784118061668060 ) ) ;
#38045=CARTESIAN_POINT ( 'NONE',  ( 86.37830602736983110, 44.06976214698578076, 6.283005621740559654 ) ) ;
#38046=VERTEX_POINT ( 'NONE', #61672 ) ;
#38047=VERTEX_POINT ( 'NONE', #7998 ) ;
#38050=CARTESIAN_POINT ( 'NONE',  ( 87.75883572471174432, 43.84347704570461701, 0.1997593521038640851 ) ) ;
#38051=ORIENTED_EDGE ( 'NONE', *, *, #59259, .T. ) ;
#38053=CARTESIAN_POINT ( 'NONE',  ( 72.29580736936866003, 70.47844812545214666, 8.033860781394157158 ) ) ;
#38054=CARTESIAN_POINT ( 'NONE',  ( 80.17048798456011127, 57.79824262504149601, 16.60278798193533589 ) ) ;
#38058=EDGE_CURVE ( 'NONE', #89714, #24132, #3180, .T. ) ;
#38065=CARTESIAN_POINT ( 'NONE',  ( 78.22211991000880005, 47.46001686969969313, -14.34986434894588037 ) ) ;
#38071=CARTESIAN_POINT ( 'NONE',  ( 83.73227335166906471, 52.23299626358674175, 14.68463506771709071 ) ) ;
#38072=ORIENTED_EDGE ( 'NONE', *, *, #38842, .F. ) ;
#38074=CARTESIAN_POINT ( 'NONE',  ( 86.91531864373632743, 46.48574869114507635, 8.998937368789745150 ) ) ;
#38085=CARTESIAN_POINT ( 'NONE',  ( 67.13662373189187349, 66.66751012937585585, 8.328433812688242455 ) ) ;
#38090=CARTESIAN_POINT ( 'NONE',  ( 71.10715990604394676, 67.46059230156090791, 10.27172394241540587 ) ) ;
#38092=CARTESIAN_POINT ( 'NONE',  ( 79.59581904190152102, 45.85957369269166861, 12.92145696107577280 ) ) ;
#38095=CARTESIAN_POINT ( 'NONE',  ( 80.36388009702766055, 54.35699232560062910, -16.24410003110130418 ) ) ;
#38100=CARTESIAN_POINT ( 'NONE',  ( 72.27036641034979425, 71.53639658761527187, 5.041488442294285832 ) ) ;
#38104=CARTESIAN_POINT ( 'NONE',  ( 66.71384051412610461, 67.45816284232765270, -6.613419748436212053 ) ) ;
#38108=CARTESIAN_POINT ( 'NONE',  ( 82.31861562935819165, 40.66747216598101033, 3.229644762565942795 ) ) ;
#38123=CARTESIAN_POINT ( 'NONE',  ( 82.45677405825341566, 47.10285889642413792, -12.64402151228549620 ) ) ;
#38124=VECTOR ( 'NONE', #42477, 1000.000000000000000 ) ;
#38126=CARTESIAN_POINT ( 'NONE',  ( 3.886609837484615859, 24.01751292744054211, 6.180339887498949913 ) ) ;
#38128=CARTESIAN_POINT ( 'NONE',  ( 71.85869513609317494, 58.67586711399007982, -15.48493562761568576 ) ) ;
#38129=CARTESIAN_POINT ( 'NONE',  ( 73.04738217724886340, 69.71546789186045601, 9.669594540409617522 ) ) ;
#38133=CARTESIAN_POINT ( 'NONE',  ( 72.68285417969771345, 57.18103607157792823, 15.88118435539451490 ) ) ;
#38136=ORIENTED_EDGE ( 'NONE', *, *, #8614, .F. ) ;
#38143=CARTESIAN_POINT ( 'NONE',  ( 34.67812306484450602, 22.94754757982092030, 5.678558825948272215 ) ) ;
#38146=CARTESIAN_POINT ( 'NONE',  ( 74.95826842568676796, 53.11571732367104204, -16.02841466325640951 ) ) ;
#38147=CARTESIAN_POINT ( 'NONE',  ( 88.47356364199694667, 43.97712956045979382, 1.870819122003384516 ) ) ;
#38149=CARTESIAN_POINT ( 'NONE',  ( 68.82743466988767977, 64.08478545733547094, 12.03889531702951565 ) ) ;
#38150=ORIENTED_EDGE ( 'NONE', *, *, #64625, .T. ) ;
#38151=CARTESIAN_POINT ( 'NONE',  ( 80.90513341749731069, 49.79037932115560494, 14.73721116675313603 ) ) ;
#38155=CARTESIAN_POINT ( 'NONE',  ( 5.010160986809694350, 24.93396525600388003, 2.839279412974139660 ) ) ;
#38158=DIRECTION ( 'NONE',  ( 0.4330127018922138582, 0.2500000000000087153, 0.8660254037844388186 ) ) ;
#38162=CARTESIAN_POINT ( 'NONE',  ( 74.81832046901195099, 67.48663194201290594, -12.71244991431774984 ) ) ;
#38173=CARTESIAN_POINT ( 'NONE',  ( 81.71554479561422113, 45.45142740597917452, -10.99315133951941093 ) ) ;
#38176=CARTESIAN_POINT ( 'NONE',  ( 79.31967116076748425, 59.78699023733838658, -16.51284638439523533 ) ) ;
#38178=CARTESIAN_POINT ( 'NONE',  ( 8.736352098677466316, 26.81751292744054638, -6.180339887498951690 ) ) ;
#38179=CARTESIAN_POINT ( 'NONE',  ( 66.29454943693275482, 69.24199052626691753, -2.144636311159408226 ) ) ;
#38180=CARTESIAN_POINT ( 'NONE',  ( 69.48618880206072390, 62.61793869292603176, 13.29615132219218765 ) ) ;
#38184=CARTESIAN_POINT ( 'NONE',  ( 73.38460905275829305, 69.71371501254900238, -9.902851190597802500 ) ) ;
#38186=CARTESIAN_POINT ( 'NONE',  ( 81.45028675782795347, 42.16027941493478437, -7.981823387058465613 ) ) ;
#38188=EDGE_CURVE ( 'NONE', #33639, #8542, #74407, .T. ) ;
#38191=CARTESIAN_POINT ( 'NONE',  ( 80.61656135465395323, 47.24360202468593428, 12.89152188940151333 ) ) ;
#38192=ORIENTED_EDGE ( 'NONE', *, *, #74763, .T. ) ;
#38193=CARTESIAN_POINT ( 'NONE',  ( 69.15891061406161100, 69.66865021447996753, 4.956695084876229451 ) ) ;
#38199=CARTESIAN_POINT ( 'NONE',  ( 68.90154995574886243, 68.41372695714582619, -7.258461826296537467 ) ) ;
#38201=CARTESIAN_POINT ( 'NONE',  ( 16.48196734934595753, 24.91421378149918198, 9.188101187500008038 ) ) ;
#38204=CARTESIAN_POINT ( 'NONE',  ( 80.05322980421331636, 57.68292478952278657, 16.60179730502024142 ) ) ;
#38210=CARTESIAN_POINT ( 'NONE',  ( 77.47822618113920612, 49.74927637487309084, -15.48360864196420295 ) ) ;
#38214=DIRECTION ( 'NONE',  ( 0.3473291852294957405, -0.6015917957689906892, 0.7193398003386545225 ) ) ;
#38216=ORIENTED_EDGE ( 'NONE', *, *, #2178, .F. ) ;
#38218=CARTESIAN_POINT ( 'NONE',  ( 75.36609510305467552, 62.13380695430679168, -15.15412763540104102 ) ) ;
#38222=CARTESIAN_POINT ( 'NONE',  ( 82.85511220885132389, 53.72155160612705060, -15.38925759434244434 ) ) ;
#38225=CARTESIAN_POINT ( 'NONE',  ( 72.01470311467906527, 72.29437185155289569, 0.6840695740065164676 ) ) ;
#38228=CARTESIAN_POINT ( 'NONE',  ( 24.30227344809185652, 37.52903772873359856, -1.583844403245329602 ) ) ;
#38234=DIRECTION ( 'NONE',  ( 0.5000000000000013323, -0.8660254037844378194, 0.000000000000000000 ) ) ;
#38235=CARTESIAN_POINT ( 'NONE',  ( 79.14312167556931854, 57.64441083166269664, 0.000000000000000000 ) ) ;
#38239=CARTESIAN_POINT ( 'NONE',  ( 71.46708483896914288, 71.41611121499917658, 5.261356510684446874 ) ) ;
#38248=CARTESIAN_POINT ( 'NONE',  ( 76.94717320005119632, 54.64271564352422672, -16.08472187958355448 ) ) ;
#38250=CARTESIAN_POINT ( 'NONE',  ( 68.74472142891936244, 63.88220321458977224, -12.16134622803817500 ) ) ;
#38252=CARTESIAN_POINT ( 'NONE',  ( 82.13428468617439648, 46.48939983997102132, 12.30969175005605898 ) ) ;
#38254=CARTESIAN_POINT ( 'NONE',  ( 71.89619214677514947, 64.26066769777372656, 13.73780722179543901 ) ) ;
#38258=CARTESIAN_POINT ( 'NONE',  ( 69.70445039019863032, 69.81249935811580087, 5.371585936356678914 ) ) ;
#38261=ORIENTED_EDGE ( 'NONE', *, *, #83999, .T. ) ;
#38262=CARTESIAN_POINT ( 'NONE',  ( 75.28801175639888754, 63.39411007085420380, 15.10357975279682741 ) ) ;
#38269=CARTESIAN_POINT ( 'NONE',  ( 7.926391159377050855, 27.68290643055185285, 3.479690158560446702E-15 ) ) ;
#38271=CARTESIAN_POINT ( 'NONE',  ( 66.10780414051450293, 68.63670250712272036, 1.777645618418523865 ) ) ;
#38278=CARTESIAN_POINT ( 'NONE',  ( 33.90715327291019321, 42.68290643055190259, 3.479690158560446702E-15 ) ) ;
#38279=CARTESIAN_POINT ( 'NONE',  ( 43.54162044069033755, 26.10801979619932567, 3.090169943749476733 ) ) ;
#38282=CARTESIAN_POINT ( 'NONE',  ( 27.91230638117223606, 28.06628583063842797, -9.188101187500006262 ) ) ;
#38290=CARTESIAN_POINT ( 'NONE',  ( 84.76146393123151768, 50.45989236026047564, -13.93701821937661833 ) ) ;
#38298=CARTESIAN_POINT ( 'NONE',  ( 28.52453836335597614, 34.65586893147758474, -7.433330006724137462 ) ) ;
#38300=B_SPLINE_CURVE_WITH_KNOTS ( 'NONE', 3,
 ( #50365, #20484, #3785, #4785, #36152, #88953, #34667, #20992, #28556, #81319, #59437, #34180, #18999, #88439, #66074, #43750 ),
 .UNSPECIFIED., .F., .F.,
 ( 4, 1, 2, 2, 2, 1, 2, 2, 4 ),
 ( 0.000000000000000000, 0.1249999999999949207, 0.1874999999999934219, 0.2499999999999919509, 0.4999999999999922284, 0.6249999999999923395, 0.6874999999999938938, 0.7499999999999954481, 1.000000000000000000 ),
 .UNSPECIFIED. ) ;
#38303=ORIENTED_EDGE ( 'NONE', *, *, #33431, .T. ) ;
#38304=PLANE ( 'NONE',  #55465 ) ;
#38306=CARTESIAN_POINT ( 'NONE',  ( 84.68103419341217375, 50.25510846593720515, 13.84703097836258934 ) ) ;
#38312=CARTESIAN_POINT ( 'NONE',  ( 79.95417701789796183, 44.68756451846406463, 11.18129038331146141 ) ) ;
#38313=CARTESIAN_POINT ( 'NONE',  ( 81.42054145595460568, 55.42004525696071937, -16.32184955832448026 ) ) ;
#38314=CARTESIAN_POINT ( 'NONE',  ( 76.89034932008942747, 61.82808869569446841, -15.91935783100940860 ) ) ;
#38320=CARTESIAN_POINT ( 'NONE',  ( 87.19297534993042120, 45.95771221245824734, -8.700079422534972906 ) ) ;
#38326=CARTESIAN_POINT ( 'NONE',  ( 72.02158190405090465, 61.69589088016835632, -14.52859831159107884 ) ) ;
#38327=CARTESIAN_POINT ( 'NONE',  ( 82.80357023854472232, 40.61453041052752155, 0.9744293009809118500 ) ) ;
#38329=CARTESIAN_POINT ( 'NONE',  ( 77.03509876804180578, 63.43842436480252900, -15.45738776637924516 ) ) ;
#38333=CARTESIAN_POINT ( 'NONE',  ( 35.31444455405989657, 43.49540643055190969, 3.479690158560446702E-15 ) ) ;
#38338=ORIENTED_EDGE ( 'NONE', *, *, #38058, .F. ) ;
#38339=CARTESIAN_POINT ( 'NONE',  ( 74.02866129013209218, 68.91877476116354728, -11.13505360475025263 ) ) ;
#38347=CARTESIAN_POINT ( 'NONE',  ( 78.87748066101475786, 48.05297491638317808, 14.45999959637729049 ) ) ;
#38350=CARTESIAN_POINT ( 'NONE',  ( 80.87517248313827167, 58.64441083166272506, 0.000000000000000000 ) ) ;
#38361=CARTESIAN_POINT ( 'NONE',  ( 73.32924055991662726, 68.54209549527047329, 10.53624946344089786 ) ) ;
#38366=CARTESIAN_POINT ( 'NONE',  ( 82.10990542498430500, 41.84899041517284957, 5.504228460268151046 ) ) ;
#38381=CARTESIAN_POINT ( 'NONE',  ( 76.03486699543272209, 51.37517956710286171, 15.65877648513449394 ) ) ;
#38393=DIRECTION ( 'NONE',  ( -0.7713975076906469663, 0.000000000000000000, -0.6363535849892403284 ) ) ;
#38394=CARTESIAN_POINT ( 'NONE',  ( 87.97191574057694652, 43.96735841855976901, 0.5176211603016172003 ) ) ;
#38397=CARTESIAN_POINT ( 'NONE',  ( 66.87519508149094349, 69.72765056100607239, -0.6245140038366959745 ) ) ;
#38399=CARTESIAN_POINT ( 'NONE',  ( 15.95033727479334651, 30.18502408145591787, 5.678558825948276656 ) ) ;
#38400=FACE_OUTER_BOUND ( 'NONE', #42300, .T. ) ;
#38402=CARTESIAN_POINT ( 'NONE',  ( 18.07869151248302941, 12.29860640527291338, -2.839279412974138328 ) ) ;
#38404=CARTESIAN_POINT ( 'NONE',  ( 76.85308935164593436, 63.86692010595712787, 14.89649355574711542 ) ) ;
#38409=CARTESIAN_POINT ( 'NONE',  ( 80.85015884162737620, 54.78783238080045948, -15.87653912250667076 ) ) ;
#38414=CARTESIAN_POINT ( 'NONE',  ( 76.96233170383452205, 49.64203404956955978, 15.03896742044604373 ) ) ;
#38415=CARTESIAN_POINT ( 'NONE',  ( 82.59507288524608271, 53.86809943430368008, 15.83774089001704155 ) ) ;
#38422=CARTESIAN_POINT ( 'NONE',  ( 79.15520340520409093, 45.87709371214184273, -12.50344660193819557 ) ) ;
#38425=VECTOR ( 'NONE', #37986, 1000.000000000000000 ) ;
#38426=ORIENTED_EDGE ( 'NONE', *, *, #56421, .F. ) ;
#38428=CARTESIAN_POINT ( 'NONE',  ( 23.18645373101242413, 19.10170272979927120, -7.433330006724141015 ) ) ;
#38429=CARTESIAN_POINT ( 'NONE',  ( 74.93856232934675177, 54.57110059908732325, 16.13587931614057425 ) ) ;
#38430=CARTESIAN_POINT ( 'NONE',  ( 7.026152882275393807, 27.55466486950697913, -1.111400068045478839E-16 ) ) ;
#38437=AXIS2_PLACEMENT_3D ( 'NONE', #53815, #54825, #98963 ) ;
#38439=CARTESIAN_POINT ( 'NONE',  ( 67.74061933540588143, 65.90611994544174479, -10.51275149194319347 ) ) ;
#38440=CARTESIAN_POINT ( 'NONE',  ( 68.93202468094986557, 70.80071090747883034, -1.952293371299729907 ) ) ;
#38457=CARTESIAN_POINT ( 'NONE',  ( 66.72329116482525535, 67.50330200424541260, 6.535431412545530172 ) ) ;
#38480=CARTESIAN_POINT ( 'NONE',  ( 37.84453522905105416, 33.80066082961425167, 10.00000000000000533 ) ) ;
#38481=CARTESIAN_POINT ( 'NONE',  ( 37.92328063009087202, 22.86426979415092475, -3.090169943749474069 ) ) ;
#38483=CARTESIAN_POINT ( 'NONE',  ( 72.69644901625827060, 70.79839986596044810, 7.145041847480314345 ) ) ;
#38484=CARTESIAN_POINT ( 'NONE',  ( 70.19981261826917773, 67.37186692534301358, -9.767772922657160350 ) ) ;
#38490=CARTESIAN_POINT ( 'NONE',  ( 80.05248732009229684, 47.95723979042521279, 13.50885685003757786 ) ) ;
#38500=CARTESIAN_POINT ( 'NONE',  ( 73.73151203714552082, 55.28494777167826157, 16.11827203802588571 ) ) ;
#38501=CARTESIAN_POINT ( 'NONE',  ( 26.48321701407081363, 20.45404122711134320, -8.090169943749478065 ) ) ;
#38512=CARTESIAN_POINT ( 'NONE',  ( 66.71010751141994888, 68.10836325903318311, -6.508687729400615574 ) ) ;
#38513=CARTESIAN_POINT ( 'NONE',  ( 72.84354978475251130, 71.10232518220605868, -7.524857974791618886 ) ) ;
#38515=CARTESIAN_POINT ( 'NONE',  ( 81.82619482746289918, 41.23108798929906982, 5.814899641828136012 ) ) ;
#38519=CARTESIAN_POINT ( 'NONE',  ( 27.47308016966368882, 31.56454794089043148, 10.00000000000000355 ) ) ;
#38520=CARTESIAN_POINT ( 'NONE',  ( 84.36224227157138955, 42.17653682963820216, -2.312994364957334348 ) ) ;
#38522=FACE_OUTER_BOUND ( 'NONE', #23009, .T. ) ;
#38523=B_SPLINE_SURFACE_WITH_KNOTS ( 'NONE', 3, 1, ( 
 ( #57108, #80472 ),
 ( #72855, #37301 ),
 ( #75837, #66709 ),
 ( #83450, #53004 ),
 ( #35815, #28211 ),
 ( #99128, #98641 ),
 ( #43903, #14017 ),
 ( #97645, #58597 ),
 ( #83955, #59086 ),
 ( #36805, #21621 ),
 ( #67717, #98134 ),
 ( #75333, #68201 ),
 ( #74349, #90060 ),
 ( #29711, #52501 ),
 ( #90570, #60587 ),
 ( #97162, #20629 ),
 ( #29224, #91543 ),
 ( #45401, #44897 ),
 ( #6424, #82957 ),
 ( #22111, #60092 ),
 ( #5916, #51006 ),
 ( #51512, #14519 ),
 ( #76331, #37793 ),
 ( #6904, #27727 ),
 ( #13531, #59593 ),
 ( #89572, #20132 ),
 ( #21138, #28719 ),
 ( #81957, #12532 ),
 ( #43404, #4937 ),
 ( #82478, #13042 ),
 ( #91056, #74843 ) ),
 .UNSPECIFIED., .F., .F., .F.,
 ( 4, 3, 3, 3, 3, 3, 3, 3, 3, 3, 4 ),
 ( 2, 2 ),
 ( 0.000000000000000000, 0.1122669598086702414, 0.2243161639709582988, 0.3396355846219021313, 0.4553962076585123531, 0.5677860799922337387, 0.6749047109689639834, 0.7773884377078371655, 0.8775581155834336622, 0.9782364162377958916, 1.000000000000000000 ),
 ( 0.000000000000000000, 1.000000000000000000 ),
 .UNSPECIFIED. ) ;
#38530=AXIS2_PLACEMENT_3D ( 'NONE', #29354, #52135, #46016 ) ;
#38533=CARTESIAN_POINT ( 'NONE',  ( 69.18180081457823860, 70.09578702365529068, -5.264143515239704918 ) ) ;
#38542=CARTESIAN_POINT ( 'NONE',  ( 22.22900788544320605, 15.76004757982089544, 5.678558825948272215 ) ) ;
#38544=CARTESIAN_POINT ( 'NONE',  ( 71.46833469722506038, 59.16469923302185663, 15.28718056364334821 ) ) ;
#38547=CARTESIAN_POINT ( 'NONE',  ( 81.65498813923811383, 45.89998691845250534, -12.05192607633446578 ) ) ;
#38548=CARTESIAN_POINT ( 'NONE',  ( 73.44882731304140577, 59.76980209779112130, -15.46587551932410065 ) ) ;
#38549=CARTESIAN_POINT ( 'NONE',  ( 81.68014092384574099, 42.03450286479537112, 7.559063547066712907 ) ) ;
#38552=CARTESIAN_POINT ( 'NONE',  ( 72.61665845909378447, 71.49531248604364464, -5.610398693002283110 ) ) ;
#38553=CARTESIAN_POINT ( 'NONE',  ( 73.14850971396091950, 57.24856527839357767, 16.39375171836413614 ) ) ;
#38562=CARTESIAN_POINT ( 'NONE',  ( 70.40337949093891723, 65.94787112513976979, 11.92354459682091417 ) ) ;
#38576=CARTESIAN_POINT ( 'NONE',  ( 81.55541168055334822, 59.46620198043990513, -0.3345653031794336152 ) ) ;
#38577=CARTESIAN_POINT ( 'NONE',  ( 78.19896130658693778, 47.52697404029742501, -14.39010834518865423 ) ) ;
#38582=CARTESIAN_POINT ( 'NONE',  ( 78.28343461854488794, 47.82939899132422568, -14.51444300807813548 ) ) ;
#38585=ORIENTED_EDGE ( 'NONE', *, *, #23850, .T. ) ;
#38596=CARTESIAN_POINT ( 'NONE',  ( 70.83774435152801630, 69.32499766432513866, 7.689863540467408498 ) ) ;
#38598=CARTESIAN_POINT ( 'NONE',  ( 71.41016749218992743, 59.45273978182970609, 15.19346469599747174 ) ) ;
#38599=CARTESIAN_POINT ( 'NONE',  ( 80.01849117754963459, 40.12822637883668619, 1.972556413651486167E-15 ) ) ;
#38600=CARTESIAN_POINT ( 'NONE',  ( 71.59027552632591096, 65.27526798289987653, -12.38681006073837665 ) ) ;
#38601=CARTESIAN_POINT ( 'NONE',  ( 77.94133778169836546, 48.01103128161624056, 14.15575917907049863 ) ) ;
#38606=CARTESIAN_POINT ( 'NONE',  ( 79.09530520295683687, 46.04380001988058524, 13.24189403536401954 ) ) ;
#38607=EDGE_CURVE ( 'NONE', #42933, #65992, #55932, .T. ) ;
#38613=CARTESIAN_POINT ( 'NONE',  ( 72.59688737879588416, 71.44559626476468850, 5.687857618654109437 ) ) ;
#38616=CARTESIAN_POINT ( 'NONE',  ( 67.00896575216198414, 67.70770252604407347, -6.454429227916835821 ) ) ;
#38621=FACE_OUTER_BOUND ( 'NONE', #34813, .T. ) ;
#38623=CARTESIAN_POINT ( 'NONE',  ( 71.79693945464293847, 65.84970020821658920, 12.07886075470384135 ) ) ;
#38624=CARTESIAN_POINT ( 'NONE',  ( 88.03940145429997699, 44.60316185140228384, -4.090138835865407607 ) ) ;
#38631=ADVANCED_FACE ( 'NONE', ( #62035 ), #17330, .T. ) ;
#38635=VERTEX_POINT ( 'NONE', #35153 ) ;
#38636=ADVANCED_FACE ( 'NONE', ( #65063 ), #57955, .F. ) ;
#38637=CIRCLE ( 'NONE', #16016, 9.000000000000007105 ) ;
#38645=CARTESIAN_POINT ( 'NONE',  ( 15.32787473065566530, 20.80066082961420904, 10.00000000000000533 ) ) ;
#38648=CARTESIAN_POINT ( 'NONE',  ( 73.02433024948126672, 69.66517378990663190, 9.714162469163342806 ) ) ;
#38653=CARTESIAN_POINT ( 'NONE',  ( 72.71802232570068725, 57.16443033622703496, 15.88657016229421615 ) ) ;
#38655=CARTESIAN_POINT ( 'NONE',  ( 66.51857804634171600, 68.84334513988093818, -4.410274944405629505 ) ) ;
#38662=CARTESIAN_POINT ( 'NONE',  ( 31.70236382085744609, 33.70171378149921537, -9.188101187500004485 ) ) ;
#38667=CARTESIAN_POINT ( 'NONE',  ( 65.81547766408900202, 68.95580224303030548, 2.207512132855569131 ) ) ;
#38668=EDGE_LOOP ( 'NONE', ( #58665, #3347, #38585, #86756 ) ) ;
#38669=CARTESIAN_POINT ( 'NONE',  ( 81.81187772080372156, 54.45965212650729370, 16.10770018195577435 ) ) ;
#38672=CARTESIAN_POINT ( 'NONE',  ( 7.926391159377050855, 27.68290643055185996, 3.479690158560446702E-15 ) ) ;
#38673=ORIENTED_EDGE ( 'NONE', *, *, #66813, .T. ) ;
#38683=CARTESIAN_POINT ( 'NONE',  ( 72.99387774792295147, 70.80171071775477287, 7.420862911638799631 ) ) ;
#38686=CARTESIAN_POINT ( 'NONE',  ( 17.57657260583443559, 33.08080186712592763, -3.090169943749475845 ) ) ;
#38687=CARTESIAN_POINT ( 'NONE',  ( 82.94646378975579637, 45.29401946974905968, -10.14977777037833562 ) ) ;
#38691=CARTESIAN_POINT ( 'NONE',  ( 79.52258874318322057, 59.35007886418325285, -16.21401609639227104 ) ) ;
#38694=CARTESIAN_POINT ( 'NONE',  ( 70.01663930090745680, 62.76214446738973152, 13.38958553957018083 ) ) ;
#38702=CARTESIAN_POINT ( 'NONE',  ( 80.20053959639768948, 46.07477633858642463, 12.22461583764979132 ) ) ;
#38703=VERTEX_POINT ( 'NONE', #12375 ) ;
#38704=CARTESIAN_POINT ( 'NONE',  ( 70.56998135810292183, 71.19273197352897853, 2.578484167683574579 ) ) ;
#38707=CARTESIAN_POINT ( 'NONE',  ( 82.17853646903301978, 46.01985525210849914, 11.26429781250972084 ) ) ;
#38711=AXIS2_PLACEMENT_3D ( 'NONE', #64122, #10939, #79869 ) ;
#38712=CARTESIAN_POINT ( 'NONE',  ( 70.34489617550165974, 68.43624669578447595, -8.554681912399528798 ) ) ;
#38714=CARTESIAN_POINT ( 'NONE',  ( 12.93608109523609073, 25.65586893147755276, -7.433330006724137462 ) ) ;
#38716=CARTESIAN_POINT ( 'NONE',  ( 80.22399782384964340, 57.81478883376428968, 16.60249858296847947 ) ) ;
#38719=ORIENTED_EDGE ( 'NONE', *, *, #29628, .F. ) ;
#38724=CARTESIAN_POINT ( 'NONE',  ( 67.67928228426634973, 65.72340518148261879, -10.66721164749792550 ) ) ;
#38731=CARTESIAN_POINT ( 'NONE',  ( 74.79265276366315618, 66.79451150088598865, -13.18326711696947839 ) ) ;
#38742=ORIENTED_EDGE ( 'NONE', *, *, #51565, .F. ) ;
#38746=CARTESIAN_POINT ( 'NONE',  ( 82.76604230628169034, 46.51291437311898846, -11.43955186660948620 ) ) ;
#38751=EDGE_CURVE ( 'NONE', #22997, #7931, #77419, .T. ) ;
#38760=CARTESIAN_POINT ( 'NONE',  ( 80.65563100889036718, 57.39222741419450813, -16.23563745603325259 ) ) ;
#38768=CARTESIAN_POINT ( 'NONE',  ( 70.25824951304763033, 70.48770578870288261, 4.457343381985276132 ) ) ;
#38770=DIRECTION ( 'NONE',  ( 0.3613624741150662234, 0.7937185950816985081, 0.4893137583626408493 ) ) ;
#38775=CARTESIAN_POINT ( 'NONE',  ( 20.82171660429349203, 14.94754757982089366, 5.678558825948272215 ) ) ;
#38783=PLANE ( 'NONE',  #83073 ) ;
#38788=CARTESIAN_POINT ( 'NONE',  ( 25.62156559687931434, 36.83396525600391413, -2.839279412974133887 ) ) ;
#38789=CARTESIAN_POINT ( 'NONE',  ( 74.97344113721968029, 63.30522816103469097, -15.06658365657160381 ) ) ;
#38790=CARTESIAN_POINT ( 'NONE',  ( 82.01068334961553319, 51.50464542205782692, 15.17394240593265664 ) ) ;
#38794=CARTESIAN_POINT ( 'NONE',  ( 83.58892928146231327, 42.23796536282910097, 5.791887481487747458 ) ) ;
#38800=CARTESIAN_POINT ( 'NONE',  ( 36.24780089259745353, 32.87878583063844218, -9.188101187500006262 ) ) ;
#38803=EDGE_CURVE ( 'NONE', #85413, #45858, #42766, .T. ) ;
#38806=CARTESIAN_POINT ( 'NONE',  ( 86.36251143053004853, 47.01529372492075254, -10.02184405881504325 ) ) ;
#38808=CARTESIAN_POINT ( 'NONE',  ( 84.45465033531688448, 50.16481452220934756, 13.87013043972112847 ) ) ;
#38810=CARTESIAN_POINT ( 'NONE',  ( 81.36927088231499283, 44.63534392387484218, -11.07837440946456553 ) ) ;
#38812=CARTESIAN_POINT ( 'NONE',  ( 38.99862784774133928, 37.91421378149922816, 9.188101187500008038 ) ) ;
#38813=CARTESIAN_POINT ( 'NONE',  ( 80.28413171908289314, 44.31094758583755322, 11.35608167334395446 ) ) ;
#38815=ORIENTED_EDGE ( 'NONE', *, *, #88805, .F. ) ;
#38818=CARTESIAN_POINT ( 'NONE',  ( 81.20643963274024202, 55.68550677472633481, 16.38154045842715334 ) ) ;
#38820=CARTESIAN_POINT ( 'NONE',  ( 86.83317331226271563, 45.77437086576020420, -8.734311406240857778 ) ) ;
#38826=CARTESIAN_POINT ( 'NONE',  ( 78.88438918712202508, 46.31898556578845216, 12.90870092474543540 ) ) ;
#38833=CARTESIAN_POINT ( 'NONE',  ( 42.23901261427005949, 30.10170272979930672, -7.433330006724141015 ) ) ;
#38838=CARTESIAN_POINT ( 'NONE',  ( 76.84140186645967674, 62.34076209027359994, -15.36631987037957181 ) ) ;
#38841=CARTESIAN_POINT ( 'NONE',  ( 72.15377119973463493, 62.27101953176124738, 14.31680684859204078 ) ) ;
#38842=EDGE_CURVE ( 'NONE', #2203, #9334, #15320, .T. ) ;
#38844=CARTESIAN_POINT ( 'NONE',  ( 77.71695824120645568, 49.45779813244274692, 15.33409790704233977 ) ) ;
#38848=CARTESIAN_POINT ( 'NONE',  ( 75.69598090375797028, 54.45081556845784121, -16.58729045400416879 ) ) ;
#38854=AXIS2_PLACEMENT_3D ( 'NONE', #15011, #54001, #55499 ) ;
#38864=CARTESIAN_POINT ( 'NONE',  ( 72.28688483481026594, 65.33959170025640617, 12.64045241524083885 ) ) ;
#38865=CARTESIAN_POINT ( 'NONE',  ( 73.68985795168487130, 65.52845945377288217, 13.58442946136029228 ) ) ;
#38869=CARTESIAN_POINT ( 'NONE',  ( 72.48280754011685190, 70.60311863597817705, 7.264376673680498442 ) ) ;
#38875=CARTESIAN_POINT ( 'NONE',  ( 82.44970526080962259, 53.47733151612504088, -15.75145310647261709 ) ) ;
#38877=CARTESIAN_POINT ( 'NONE',  ( 67.85970132199700799, 69.63639107943987483, 4.385596732954796018 ) ) ;
#38878=CARTESIAN_POINT ( 'NONE',  ( 72.10617024684209753, 72.18421392457030095, 4.031754617348218162 ) ) ;
#38882=CARTESIAN_POINT ( 'NONE',  ( 78.53484019558472085, 58.14436697958397104, 16.22033106392862578 ) ) ;
#38883=CARTESIAN_POINT ( 'NONE',  ( 84.69192290788414823, 50.49093492985745257, -13.55378674288394336 ) ) ;
#38885=CARTESIAN_POINT ( 'NONE',  ( 73.69504701792554613, 69.38216658601243125, -9.921919506181135162 ) ) ;
#38886=CARTESIAN_POINT ( 'NONE',  ( 76.09822188795720876, 51.18568606329870363, 16.10049749365522942 ) ) ;
#38896=CARTESIAN_POINT ( 'NONE',  ( 88.35650425256305596, 44.18871754174234212, 0.2633948951645489478 ) ) ;
#38897=CARTESIAN_POINT ( 'NONE',  ( 7.727700963378506316, 20.16454794089039382, -10.00000000000000355 ) ) ;
#38901=CARTESIAN_POINT ( 'NONE',  ( 23.73493010604062192, 29.10171378149919974, 9.188101187500008038 ) ) ;
#38904=CARTESIAN_POINT ( 'NONE',  ( 15.97197434310064601, 12.14754757982088940, -5.678558825948276656 ) ) ;
#38907=CARTESIAN_POINT ( 'NONE',  ( 82.80988375738442642, 53.83802849848978411, -15.42793928106117818 ) ) ;
#38909=CARTESIAN_POINT ( 'NONE',  ( 73.99071832934600934, 66.66873186589971567, 12.45603791228730550 ) ) ;
#38911=CARTESIAN_POINT ( 'NONE',  ( 87.64404534381598921, 45.17643606527867917, -6.176835110407645324 ) ) ;
#38918=CARTESIAN_POINT ( 'NONE',  ( 82.52272021305054750, 54.20245997282780337, 15.57906378977955164 ) ) ;
#38922=CARTESIAN_POINT ( 'NONE',  ( 71.50240432004942193, 72.40933122983058468, 5.654570818603106787E-06 ) ) ;
#38930=CARTESIAN_POINT ( 'NONE',  ( 31.98500480842837490, 19.26216523072496400, -2.296566073217252530E-15 ) ) ;
#38931=CARTESIAN_POINT ( 'NONE',  ( 79.98829826360795892, 44.59498145176360140, 11.76229304004083964 ) ) ;
#38933=CARTESIAN_POINT ( 'NONE',  ( 75.06695094285402092, 67.05599132900849213, -12.66018568268391853 ) ) ;
#38934=EDGE_LOOP ( 'NONE', ( #33112, #66126, #72772, #35647 ) ) ;
#38935=DIRECTION ( 'NONE',  ( -0.8660254037844379305, -0.5000000000000014433, -0.000000000000000000 ) ) ;
#38941=CARTESIAN_POINT ( 'NONE',  ( 67.92368367061898482, 65.30421490620477698, -10.50538595028323918 ) ) ;
#38944=CARTESIAN_POINT ( 'NONE',  ( 71.64405606982037966, 72.29848632667865616, -2.396508723004914909 ) ) ;
#38946=B_SPLINE_CURVE_WITH_KNOTS ( 'NONE', 3,
 ( #33821, #40876, #3905, #96642, #26209, #12011, #25716, #41893, #71821, #11023, #35292, #87583, #64709, #27208, #95660, #57086 ),
 .UNSPECIFIED., .F., .F.,
 ( 4, 1, 2, 2, 2, 1, 2, 2, 4 ),
 ( 0.000000000000000000, 0.1250000000000001388, 0.1874999999999999167, 0.2499999999999997224, 0.4999999999999936717, 0.6249999999999927836, 0.6874999999999924505, 0.7499999999999920064, 1.000000000000000000 ),
 .UNSPECIFIED. ) ;
#38958=CARTESIAN_POINT ( 'NONE',  ( 66.75636626838043242, 67.88323880877007355, 6.998558940700871034 ) ) ;
#38960=CARTESIAN_POINT ( 'NONE',  ( 81.23909821190164848, 55.73431417435049440, 16.38583623711208404 ) ) ;
#38961=CARTESIAN_POINT ( 'NONE',  ( 78.19967833365834053, 48.92268198308481431, -14.50970423465381209 ) ) ;
#38965=ORIENTED_EDGE ( 'NONE', *, *, #30619, .F. ) ;
#38971=CARTESIAN_POINT ( 'NONE',  ( 76.41687528450239597, 51.62467577766678772, -15.66419350453952752 ) ) ;
#38973=CARTESIAN_POINT ( 'NONE',  ( 75.99750771566300500, 65.44421971917600445, -13.95497799904429570 ) ) ;
#38978=CARTESIAN_POINT ( 'NONE',  ( 84.01082902402941954, 43.69534178878007680, -7.113612602852647626 ) ) ;
#38983=CARTESIAN_POINT ( 'NONE',  ( 72.49859375374551007, 70.63268695749106030, 7.230702372335866990 ) ) ;
#38984=CARTESIAN_POINT ( 'NONE',  ( 67.66477494612622934, 65.93994996590180335, 10.43000742999573482 ) ) ;
#38997=CARTESIAN_POINT ( 'NONE',  ( 74.09532166844117285, 55.24532013836130773, 16.12365093312453368 ) ) ;
#38999=CARTESIAN_POINT ( 'NONE',  ( 22.94593010929795085, 36.18080186712593616, 3.090169943749475401 ) ) ;
#39006=VERTEX_POINT ( 'NONE', #5624 ) ;
#39008=CARTESIAN_POINT ( 'NONE',  ( 72.85870443091526738, 70.94102631263370995, -7.807649534274232472 ) ) ;
#39009=CARTESIAN_POINT ( 'NONE',  ( 81.58528556317443758, 41.69952858397179796, 5.867569315483937231 ) ) ;
#39011=EDGE_CURVE ( 'NONE', #75363, #33639, #70593, .T. ) ;
#39013=CARTESIAN_POINT ( 'NONE',  ( 31.08397696812772182, 23.11029122506295863, -8.090169943749478065 ) ) ;
#39015=CARTESIAN_POINT ( 'NONE',  ( 81.32995746972275697, 56.15987802315089539, 16.09091581593350639 ) ) ;
#39016=CARTESIAN_POINT ( 'NONE',  ( 87.18641337702047167, 46.17289800388120113, -8.348801549285765233 ) ) ;
#39019=CARTESIAN_POINT ( 'NONE',  ( 71.26875018709939980, 66.61859495416860000, -11.15484612302055289 ) ) ;
#39022=CARTESIAN_POINT ( 'NONE',  ( 72.69592421641890212, 70.74456683587561656, -7.971905174712502706 ) ) ;
#39028=DIRECTION ( 'NONE',  ( 0.8660254037844399289, 0.4999999999999977240, -0.000000000000000000 ) ) ;
#39031=CARTESIAN_POINT ( 'NONE',  ( 23.96105869301208813, 16.76004757982090254, 5.678558825948272215 ) ) ;
#39032=CARTESIAN_POINT ( 'NONE',  ( 8.232026531027987204, 23.49103043416547365, -8.090169943749479842 ) ) ;
#39033=CARTESIAN_POINT ( 'NONE',  ( 71.91139111156488184, 59.09947579900738646, 15.87520130762167625 ) ) ;
#39036=CARTESIAN_POINT ( 'NONE',  ( 9.941082954516852865, 14.24335787977761214, -9.188101187500008038 ) ) ;
#39037=CARTESIAN_POINT ( 'NONE',  ( 74.59194231731085267, 59.40658604406281995, -15.72090067485143550 ) ) ;
#39038=CARTESIAN_POINT ( 'NONE',  ( 81.89930626884697062, 42.21375885363389813, 7.647715624881986862 ) ) ;
#39039=CARTESIAN_POINT ( 'NONE',  ( 44.42076818640806835, 30.81029122506298634, 8.090169943749479842 ) ) ;
#39041=CARTESIAN_POINT ( 'NONE',  ( 72.33760062768145360, 71.68797599686796218, -5.790821312261726916 ) ) ;
#39043=CARTESIAN_POINT ( 'NONE',  ( 83.06993023455761715, 40.79143924675896926, 1.309702138887457679 ) ) ;
#39047=CARTESIAN_POINT ( 'NONE',  ( 87.35151617023949200, 43.63067449739911297, -0.4462371624748913690 ) ) ;
#39050=CARTESIAN_POINT ( 'NONE',  ( 69.61585729181811644, 63.78595448314586491, 13.21249610887674208 ) ) ;
#39051=CARTESIAN_POINT ( 'NONE',  ( 72.88508378922313113, 56.80021903471959632, -15.95571064693559293 ) ) ;
#39052=CARTESIAN_POINT ( 'NONE',  ( 77.30463285345523161, 63.36080703450485174, 15.53535672671000079 ) ) ;
#39059=CARTESIAN_POINT ( 'NONE',  ( 26.01788259378743717, 35.99752408145593563, 5.678558825948277544 ) ) ;
#39062=CARTESIAN_POINT ( 'NONE',  ( 71.63103492117565452, 72.07843208848032646, 3.395715836721224790 ) ) ;
#39067=CARTESIAN_POINT ( 'NONE',  ( 83.56942396399851702, 52.37055672471088741, 14.78365564216985639 ) ) ;
#39070=EDGE_LOOP ( 'NONE', ( #7160, #23406, #78255, #39729 ) ) ;
#39071=CARTESIAN_POINT ( 'NONE',  ( 87.78081971166569986, 44.10618430004836910, 2.676874261813567468 ) ) ;
#39081=CARTESIAN_POINT ( 'NONE',  ( 69.01174091589227544, 65.49457112254064839, 10.95257573316000688 ) ) ;
#39083=CARTESIAN_POINT ( 'NONE',  ( 67.41087925495308752, 66.60807491237166289, 8.627370698444245534 ) ) ;
#39084=CARTESIAN_POINT ( 'NONE',  ( 70.51113942130736234, 65.45616864928850021, -11.75070865024357403 ) ) ;
#39085=CARTESIAN_POINT ( 'NONE',  ( 78.30366600412818912, 47.44550441188034995, 14.31860126704143532 ) ) ;
#39089=CARTESIAN_POINT ( 'NONE',  ( 70.14510041679191943, 64.94605215490624062, 11.99719282233523288 ) ) ;
#39094=CARTESIAN_POINT ( 'NONE',  ( 83.53129465503697304, 51.49339246050250551, -14.42226391936362973 ) ) ;
#39097=CARTESIAN_POINT ( 'NONE',  ( 80.25077290097513583, 58.18867766503439043, -16.60702595570231566 ) ) ;
#39098=CARTESIAN_POINT ( 'NONE',  ( 72.01291228344958029, 71.60916324447191528, 5.531298035833725812 ) ) ;
#39099=CARTESIAN_POINT ( 'NONE',  ( 74.62401959271109320, 66.89443057110611335, 13.05059976691391377 ) ) ;
#39108=CARTESIAN_POINT ( 'NONE',  ( 70.74303910967452680, 62.45564769402658101, 13.80964952784702504 ) ) ;
#39110=B_SPLINE_SURFACE_WITH_KNOTS ( 'NONE', 3, 1, ( 
 ( #30631, #61516 ),
 ( #91462, #75252 ),
 ( #92463, #15404 ),
 ( #67625, #6333 ),
 ( #46297, #30124 ),
 ( #224, #22527 ),
 ( #29632, #76253 ),
 ( #77224, #60505 ),
 ( #7830, #61007 ),
 ( #22023, #31108 ),
 ( #53417, #37711 ),
 ( #92948, #54393 ),
 ( #44812, #6825 ),
 ( #52923, #83369 ),
 ( #85369, #83874 ),
 ( #44320, #98559 ),
 ( #29144, #60015 ),
 ( #90979, #63020 ),
 ( #24518, #94963 ),
 ( #16417, #86885 ),
 ( #85893, #8327 ),
 ( #16913, #32110 ),
 ( #17941, #40708 ),
 ( #2746, #71144 ),
 ( #55891, #25528 ),
 ( #54914, #47312 ),
 ( #47802, #8819 ),
 ( #48840, #39687 ),
 ( #62494, #56416 ),
 ( #31603, #32622 ),
 ( #79275, #17418 ) ),
 .UNSPECIFIED., .F., .F., .F.,
 ( 4, 3, 3, 3, 3, 3, 3, 3, 3, 3, 4 ),
 ( 2, 2 ),
 ( 0.000000000000000000, 0.1333490885032429241, 0.3007194338854423110, 0.4699862290245206409, 0.5844252810809303922, 0.6686540514502636867, 0.7354980260655383795, 0.8028463152565493699, 0.8633854507757111607, 0.9437142632667171460, 1.000000000000000000 ),
 ( 0.000000000000000000, 1.000000000000000000 ),
 .UNSPECIFIED. ) ;
#39114=CARTESIAN_POINT ( 'NONE',  ( 81.90827648927033522, 41.78436240737912755, -5.623587741670904805 ) ) ;
#39121=CARTESIAN_POINT ( 'NONE',  ( 88.03377929273251823, 44.78256942470972035, 4.638045985396566095 ) ) ;
#39124=CARTESIAN_POINT ( 'NONE',  ( 7.905500100003217234, 28.65659080271449000, -1.878358725466461243E-16 ) ) ;
#39127=CARTESIAN_POINT ( 'NONE',  ( 72.06779285608921271, 72.04837681130726423, 2.871792874092435000 ) ) ;
#39132=CARTESIAN_POINT ( 'NONE',  ( 73.60933432321982650, 55.64367109616565443, 16.10230547196763595 ) ) ;
#39134=CARTESIAN_POINT ( 'NONE',  ( 17.89217828605986327, 10.73415679381820986, 1.333680081654574804E-15 ) ) ;
#39139=CARTESIAN_POINT ( 'NONE',  ( 31.65185205300530313, 23.98920272979928114, 7.433330006724137462 ) ) ;
#39145=CARTESIAN_POINT ( 'NONE',  ( 88.35595341439740480, 43.98873182231152867, 2.401576318819967693 ) ) ;
#39146=CARTESIAN_POINT ( 'NONE',  ( 66.08603031403475825, 68.56143032305313056, 2.184140419465945726 ) ) ;
#39150=CARTESIAN_POINT ( 'NONE',  ( 4.836955906052805787, 24.83396525600387861, -2.839279412974133887 ) ) ;
#39154=CARTESIAN_POINT ( 'NONE',  ( 71.78057061738425659, 72.16630549687447171, 0.5834590807434386628 ) ) ;
#39165=CARTESIAN_POINT ( 'NONE',  ( 72.72687233632774451, 70.81140904708308881, 7.152679309755922255 ) ) ;
#39171=CARTESIAN_POINT ( 'NONE',  ( 79.13855990483197900, 59.10183223203091529, -16.21630931228972372 ) ) ;
#39173=CARTESIAN_POINT ( 'NONE',  ( 70.02188392290977959, 62.77544136721036239, 13.38372670034021894 ) ) ;
#39174=VECTOR ( 'NONE', #10672, 1000.000000000000114 ) ;
#39181=ORIENTED_EDGE ( 'NONE', *, *, #27802, .F. ) ;
#39183=CARTESIAN_POINT ( 'NONE',  ( 74.12068342383874153, 64.67028550015082544, 13.75713335287279193 ) ) ;
#39189=CARTESIAN_POINT ( 'NONE',  ( 83.09975762653809284, 48.63870101769774124, 12.90973747663798576 ) ) ;
#39198=CARTESIAN_POINT ( 'NONE',  ( 9.881553883097156543, 27.74646525600388713, 2.839279412974139660 ) ) ;
#39200=CARTESIAN_POINT ( 'NONE',  ( 80.19730562280793151, 57.80653512312768783, 16.60264294324888468 ) ) ;
#39210=CARTESIAN_POINT ( 'NONE',  ( 81.11448992224303822, 46.11779734161436295, -11.84940212323523667 ) ) ;
#39225=CARTESIAN_POINT ( 'NONE',  ( 75.57301432718394096, 65.50289043567833858, 13.81433800577013926 ) ) ;
#39228=PRODUCT_DEFINITION_CONTEXT ( 'detailed design', #33745, 'design' ) ;
#39230=CARTESIAN_POINT ( 'NONE',  ( 6.396987757676594555, 15.64441083166260427, 0.000000000000000000 ) ) ;
#39232=CARTESIAN_POINT ( 'NONE',  ( 86.04723689193814096, 45.96568028731314115, -8.941333467903920251 ) ) ;
#39234=CARTESIAN_POINT ( 'NONE',  ( 74.27850899688687036, 68.48602583890969697, -11.15250335310150298 ) ) ;
#39238=LINE ( 'NONE', #24063, #65836 ) ;
#39243=CARTESIAN_POINT ( 'NONE',  ( 80.64966744098836671, 57.49487408124664967, -16.23886060901187989 ) ) ;
#39260=CARTESIAN_POINT ( 'NONE',  ( 17.90548643172614263, 12.19860640527291373, 2.839279412974134775 ) ) ;
#39262=EDGE_CURVE ( 'NONE', #6127, #71267, #71883, .T. ) ;
#39263=CARTESIAN_POINT ( 'NONE',  ( 72.29638194752672575, 59.45177225770978424, -15.84340229133642985 ) ) ;
#39272=CARTESIAN_POINT ( 'NONE',  ( 86.47393795017364937, 47.46484117499104372, 10.41372632371118101 ) ) ;
#39280=CARTESIAN_POINT ( 'NONE',  ( 75.81625539762656274, 65.12695345013474935, -14.47344923651660054 ) ) ;
#39282=CARTESIAN_POINT ( 'NONE',  ( 74.14312167556930433, 66.30466486950707861, 1.224646799147354045E-15 ) ) ;
#39283=CARTESIAN_POINT ( 'NONE',  ( 88.49445028879968334, 43.86712364161932243, -9.307608808691473302E-08 ) ) ;
#39285=CARTESIAN_POINT ( 'NONE',  ( 73.63798764345266079, 69.67310094948797428, 10.11710443556177275 ) ) ;
#39286=CARTESIAN_POINT ( 'NONE',  ( 43.36002773778349706, 27.96004757982094446, -5.678558825948276656 ) ) ;
#39292=CARTESIAN_POINT ( 'NONE',  ( 79.59476633789469702, 59.27799801817308634, 16.56459525109986330 ) ) ;
#39297=CARTESIAN_POINT ( 'NONE',  ( 81.59199138121388728, 55.54565483415311888, -16.32615847003737386 ) ) ;
#39303=CARTESIAN_POINT ( 'NONE',  ( 77.12749119013076893, 49.43705909587082914, -14.93372123758744152 ) ) ;
#39306=CARTESIAN_POINT ( 'NONE',  ( 78.86981778719953695, 51.57386105711080404, 15.33895568566510015 ) ) ;
#39310=CARTESIAN_POINT ( 'NONE',  ( 36.30495719079549843, 21.36477965099642873, 1.583844403245364907 ) ) ;
#39313=CARTESIAN_POINT ( 'NONE',  ( 82.27383947616280579, 40.86467265836121499, 1.031166341950346954 ) ) ;
#39315=CARTESIAN_POINT ( 'NONE',  ( 76.92814081923833669, 62.93039039429913828, -15.23958875853725203 ) ) ;
#39321=CARTESIAN_POINT ( 'NONE',  ( 38.69312636016019269, 30.84335787977765619, 9.188101187500006262 ) ) ;
#39324=EDGE_CURVE ( 'NONE', #55385, #15274, #70622, .T. ) ;
#39332=CARTESIAN_POINT ( 'NONE',  ( 66.30954113569532637, 68.28728378170326607, 3.992301261007330737 ) ) ;
#39336=ORIENTED_EDGE ( 'NONE', *, *, #36119, .F. ) ;
#39338=CARTESIAN_POINT ( 'NONE',  ( 66.03861470602267048, 68.70284247729489380, -0.4429836963394074290 ) ) ;
#39340=DIRECTION ( 'NONE',  ( -0.8660254037844379305, -0.5000000000000014433, -0.000000000000000000 ) ) ;
#39350=B_SPLINE_SURFACE_WITH_KNOTS ( 'NONE', 3, 1, ( 
 ( #84486, #75372 ),
 ( #61129, #15029 ),
 ( #90607, #29750 ),
 ( #45920, #69237 ),
 ( #21174, #76839 ),
 ( #91577, #29260 ),
 ( #7436, #60622 ),
 ( #100166, #5953 ),
 ( #52054, #43938 ),
 ( #6940, #37831 ),
 ( #13569, #60129 ),
 ( #14559, #91091 ),
 ( #82992, #36847 ),
 ( #44934, #68239 ),
 ( #67755, #98680 ),
 ( #38329, #21656 ),
 ( #5460, #75880 ),
 ( #30752, #52538 ),
 ( #83489, #14055 ),
 ( #45434, #92105 ),
 ( #90096, #82516 ),
 ( #51553, #6458 ),
 ( #22149, #53040 ),
 ( #20665, #99661 ),
 ( #13077, #74877 ),
 ( #36344, #67246 ),
 ( #98176, #23620 ),
 ( #86504, #94083 ),
 ( #85492, #16536 ),
 ( #61629, #39315 ),
 ( #32736, #1352 ) ),
 .UNSPECIFIED., .F., .F., .F.,
 ( 4, 3, 3, 3, 3, 3, 3, 3, 3, 3, 4 ),
 ( 2, 2 ),
 ( 0.000000000000000000, 0.1333490885032290463, 0.3007194338854137228, 0.4699862290245038765, 0.5844252810809251741, 0.6686540514502686827, 0.7354980260655517021, 0.8028463152565618044, 0.8633854507757415808, 0.9437142632667480102, 1.000000000000000000 ),
 ( 0.000000000000000000, 1.000000000000000000 ),
 .UNSPECIFIED. ) ;
#39351=CARTESIAN_POINT ( 'NONE',  ( 72.68994967886170855, 66.60535542942379550, 11.89643324170776850 ) ) ;
#39358=CARTESIAN_POINT ( 'NONE',  ( 74.29686697005888618, 68.54486718330414874, 11.12163720784228893 ) ) ;
#39359=CARTESIAN_POINT ( 'NONE',  ( 70.87618550449425925, 71.40954602149369634, -2.428563748625821805 ) ) ;
#39362=CARTESIAN_POINT ( 'NONE',  ( 67.65687428590848640, 66.76031625959198834, 8.613883631066450164 ) ) ;
#39368=CARTESIAN_POINT ( 'NONE',  ( 84.60735463175657856, 50.53152741511170376, -13.60229262012000184 ) ) ;
#39370=CARTESIAN_POINT ( 'NONE',  ( 73.05863210132505969, 69.60576123971952711, -9.808587366596247747 ) ) ;
#39371=CARTESIAN_POINT ( 'NONE',  ( 76.31637673998004345, 51.11355729699548078, 16.05611523598242840 ) ) ;
#39372=CARTESIAN_POINT ( 'NONE',  ( 72.28884795246587203, 71.97623822831552332, -3.689212715915426877 ) ) ;
#39377=DIRECTION ( 'NONE',  ( 0.3473291852294957405, -0.6015917957689906892, 0.7193398003386545225 ) ) ;
#39381=CARTESIAN_POINT ( 'NONE',  ( 88.37416949021037738, 43.79857776338975839, 0.1607882160166528573 ) ) ;
#39385=CARTESIAN_POINT ( 'NONE',  ( 72.17322115918098291, 71.85944340353097459, -3.889528917610050041 ) ) ;
#39386=CARTESIAN_POINT ( 'NONE',  ( 69.77735531064696772, 70.84206482737464228, -4.035796813025271490 ) ) ;
#39388=CARTESIAN_POINT ( 'NONE',  ( 25.46698091360950045, 30.10171378149919974, 9.188101187500008038 ) ) ;
#39390=CARTESIAN_POINT ( 'NONE',  ( 83.29758183770785251, 47.02354989389091600, -11.60801483937473044 ) ) ;
#39391=CARTESIAN_POINT ( 'NONE',  ( 11.30507296547734697, 15.03085787977761179, 9.188101187500006262 ) ) ;
#39393=CARTESIAN_POINT ( 'NONE',  ( 76.96934732445689065, 63.82118396924765591, 14.93646943666589344 ) ) ;
#39401=CARTESIAN_POINT ( 'NONE',  ( 78.24789397509293565, 55.76986583530001695, -16.13979192025500353 ) ) ;
#39406=CARTESIAN_POINT ( 'NONE',  ( 77.21588584563488666, 49.49447693446913377, 14.93476029654182646 ) ) ;
#39411=CARTESIAN_POINT ( 'NONE',  ( 67.61525443866294438, 68.60254357949423820, -5.272938102954969786 ) ) ;
#39414=ORIENTED_EDGE ( 'NONE', *, *, #68098, .T. ) ;
#39419=CARTESIAN_POINT ( 'NONE',  ( 27.58754685475307156, 27.87878583063842797, -9.188101187500006262 ) ) ;
#39421=CARTESIAN_POINT ( 'NONE',  ( 75.04128323750522611, 66.36387088788158906, -13.13100288533564886 ) ) ;
#39428=CARTESIAN_POINT ( 'NONE',  ( 67.79325343485642463, 65.52334347001540493, 10.20133969316753131 ) ) ;
#39429=CARTESIAN_POINT ( 'NONE',  ( 67.78518765966735771, 65.95975373770653505, -10.48313618456564988 ) ) ;
#39445=CARTESIAN_POINT ( 'NONE',  ( 80.00158170572299809, 44.44258412922052770, -10.93648124919405795 ) ) ;
#39448=CARTESIAN_POINT ( 'NONE',  ( 81.32396741884589630, 55.80035763937271298, 16.38826086546822580 ) ) ;
#39456=CARTESIAN_POINT ( 'NONE',  ( 19.65800174957785629, 23.30066082961421969, -10.00000000000000533 ) ) ;
#39457=CARTESIAN_POINT ( 'NONE',  ( 76.03323602888910671, 65.53324422044475739, -14.33394004605309036 ) ) ;
#39461=CARTESIAN_POINT ( 'NONE',  ( 87.74187345177139719, 44.20045605528624577, 4.652363546664123106 ) ) ;
#39462=ORIENTED_EDGE ( 'NONE', *, *, #49000, .T. ) ;
#39464=CARTESIAN_POINT ( 'NONE',  ( 43.27754793094329244, 25.39040679176986970, -6.890680421881970419E-14 ) ) ;
#39467=B_SPLINE_CURVE_WITH_KNOTS ( 'NONE', 3,
 ( #79699, #63947, #9260, #62947, #70545, #78165, #72068, #54841, #71571, #8260, #2167, #32555, #86813, #48766, #24451, #33048 ),
 .UNSPECIFIED., .F., .F.,
 ( 4, 1, 2, 2, 2, 1, 2, 2, 4 ),
 ( 0.000000000000000000, 0.1249999999999967804, 0.1874999999999955591, 0.2499999999999943379, 0.4999999999999986677, 0.6250000000000023315, 0.6875000000000021094, 0.7500000000000019984, 1.000000000000000000 ),
 .UNSPECIFIED. ) ;
#39470=EDGE_LOOP ( 'NONE', ( #37450, #9040, #37771, #58396 ) ) ;
#39473=DIRECTION ( 'NONE',  ( 0.7905172007421643610, 0.000000000000000000, 0.6124398381316914497 ) ) ;
#39475=CARTESIAN_POINT ( 'NONE',  ( 83.82827945288542537, 51.88092520783234818, 14.50189114860043027 ) ) ;
#39484=CYLINDRICAL_SURFACE ( 'NONE', #68973, 16.60714546451156792 ) ;
#39485=CARTESIAN_POINT ( 'NONE',  ( 69.69198297313906210, 62.71137935599142565, -13.30837126644457236 ) ) ;
#39486=CARTESIAN_POINT ( 'NONE',  ( 32.90709467669684329, 21.12755873383627758, -6.180339887498949025 ) ) ;
#39494=ORIENTED_EDGE ( 'NONE', *, *, #88410, .F. ) ;
#39495=B_SPLINE_CURVE_WITH_KNOTS ( 'NONE', 3,
 ( #80058, #10626, #1360, #33775, #95100, #47439, #9459, #40329, #78873, #10969, #71268, #63647, #25140, #64661, #64148, #25664 ),
 .UNSPECIFIED., .F., .F.,
 ( 4, 1, 2, 2, 2, 1, 2, 2, 4 ),
 ( 0.000000000000000000, 0.1249999999999990841, 0.1875000000000001665, 0.2500000000000012768, 0.5000000000000003331, 0.6249999999999998890, 0.6874999999999983347, 0.7499999999999966693, 1.000000000000000000 ),
 .UNSPECIFIED. ) ;
#39500=CARTESIAN_POINT ( 'NONE',  ( 22.93916872074224855, 35.01751292744057054, 6.180339887498949913 ) ) ;
#39501=CARTESIAN_POINT ( 'NONE',  ( 34.02846334099481140, 24.81029122506296503, 8.090169943749479842 ) ) ;
#39502=CARTESIAN_POINT ( 'NONE',  ( 76.77731254116882553, 64.09355814141257213, -15.16545583891343263 ) ) ;
#39511=CARTESIAN_POINT ( 'NONE',  ( 72.62602488434787062, 66.38659855042941160, -12.03580873979266208 ) ) ;
#39513=EDGE_CURVE ( 'NONE', #13677, #58122, #51208, .T. ) ;
#39522=CARTESIAN_POINT ( 'NONE',  ( 73.62250635243425734, 69.55784274833358438, 10.23584637956793308 ) ) ;
#39524=CARTESIAN_POINT ( 'NONE',  ( 26.41418602390824333, 17.11110640527292759, -2.839279412974138328 ) ) ;
#39528=ORIENTED_EDGE ( 'NONE', *, *, #36119, .T. ) ;
#39530=CARTESIAN_POINT ( 'NONE',  ( 10.98031343905818069, 14.84335787977761179, 9.188101187500006262 ) ) ;
#39531=CARTESIAN_POINT ( 'NONE',  ( 88.22000632671873177, 44.27423112938744509, 4.003506518527978564 ) ) ;
#39532=CARTESIAN_POINT ( 'NONE',  ( 75.79749919803089142, 58.99206122708265809, -15.93881189237040097 ) ) ;
#39533=CARTESIAN_POINT ( 'NONE',  ( 71.75124654091098364, 72.49002453570855664, -1.344699539992842752 ) ) ;
#39534=VERTEX_POINT ( 'NONE', #38598 ) ;
#39536=CARTESIAN_POINT ( 'NONE',  ( 72.29604205201167133, 71.64671137691723857, -5.830803549263603891 ) ) ;
#39542=CARTESIAN_POINT ( 'NONE',  ( 66.57026871561890857, 68.76443072695623471, 4.738950751700697239 ) ) ;
#39543=CARTESIAN_POINT ( 'NONE',  ( 84.44461922012131083, 42.65730447493894673, -4.171913819451575911 ) ) ;
#39546=CARTESIAN_POINT ( 'NONE',  ( 71.82992063434448937, 72.13096581328876766, -3.644439638307356955 ) ) ;
#39547=CARTESIAN_POINT ( 'NONE',  ( 79.83401254395657531, 57.87045807247319118, 16.26439772172798115 ) ) ;
#39550=B_SPLINE_CURVE_WITH_KNOTS ( 'NONE', 3,
 ( #26652, #49947, #11477, #10455 ),
 .UNSPECIFIED., .F., .F.,
 ( 4, 4 ),
 ( 0.000000000000000000, 0.007447265025110824666 ),
 .UNSPECIFIED. ) ;
#39552=ORIENTED_EDGE ( 'NONE', *, *, #97538, .F. ) ;
#39553=CARTESIAN_POINT ( 'NONE',  ( 67.00187114335926708, 67.08813303282481399, 8.529924657355548945 ) ) ;
#39556=CARTESIAN_POINT ( 'NONE',  ( 22.00590953607929023, 34.74646525600390845, 2.839279412974139660 ) ) ;
#39558=CARTESIAN_POINT ( 'NONE',  ( 78.36279588851795097, 47.41043415324341481, -13.73196331463247155 ) ) ;
#39567=CARTESIAN_POINT ( 'NONE',  ( 84.25080109756747504, 42.92892633554705384, -5.211464095953071585 ) ) ;
#39570=VERTEX_POINT ( 'NONE', #84257 ) ;
#39577=CARTESIAN_POINT ( 'NONE',  ( 69.25351710553235307, 66.05396458075408361, 10.55744696599895427 ) ) ;
#39581=CARTESIAN_POINT ( 'NONE',  ( 75.62235313057280450, 64.20969772940269138, -14.41545499348065285 ) ) ;
#39582=CARTESIAN_POINT ( 'NONE',  ( 78.48653837275075773, 47.85077451888660960, 13.91762572861853187 ) ) ;
#39587=DIRECTION ( 'NONE',  ( 0.3940053768033583426, -0.6824373310787393843, 0.6156614753256619554 ) ) ;
#39592=CARTESIAN_POINT ( 'NONE',  ( 83.58592293191674116, 51.62412561587523641, -14.84978998814507989 ) ) ;
#39594=ORIENTED_EDGE ( 'NONE', *, *, #59547, .F. ) ;
#39598=CARTESIAN_POINT ( 'NONE',  ( 74.61783790005046058, 67.04252370310037179, 12.50665000838213814 ) ) ;
#39605=CARTESIAN_POINT ( 'NONE',  ( 85.41379983563213329, 48.29620419992356517, -11.76667240678645321 ) ) ;
#39609=CARTESIAN_POINT ( 'NONE',  ( 72.04273812837081437, 59.28583566120335746, 15.34548535902080246 ) ) ;
#39611=CARTESIAN_POINT ( 'NONE',  ( 82.00121032730237403, 41.82734585847611442, -5.599361062352755880 ) ) ;
#39620=CARTESIAN_POINT ( 'NONE',  ( 87.68052222859077460, 44.70628762572462733, 5.023047487083897700 ) ) ;
#39622=CARTESIAN_POINT ( 'NONE',  ( 13.61667370911268193, 23.56454794089040661, 10.00000000000000355 ) ) ;
#39625=B_SPLINE_CURVE_WITH_KNOTS ( 'NONE', 3,
 ( #4585, #98299, #13200, #74000, #43054, #81622, #35479, #28888, #27394, #44058, #42564, #52166, #59765, #12195, #58762, #26896, #65875, #57774, #81138, #96831, #89732, #51692, #88748, #6078 ),
 .UNSPECIFIED., .F., .F.,
 ( 4, 2, 2, 2, 2, 2, 2, 2, 2, 2, 2, 4 ),
 ( 0.000000000000000000, 0.1250000000000211220, 0.2500000000000422440, 0.3750000000000633937, 0.4375000000000662248, 0.5000000000000690559, 0.5625000000000719425, 0.6250000000000748290, 0.6875000000000777156, 0.7500000000000806022, 0.8750000000000404121, 1.000000000000000000 ),
 .UNSPECIFIED. ) ;
#39632=CARTESIAN_POINT ( 'NONE',  ( 18.10888558598233544, 12.58380873178785997, 6.180339887498953466 ) ) ;
#39638=CARTESIAN_POINT ( 'NONE',  ( 26.97895004263468266, 38.68290643055188127, 3.479690158560446702E-15 ) ) ;
#39645=CARTESIAN_POINT ( 'NONE',  ( 66.31377247145708509, 69.19807880125443944, 2.483205996023140294 ) ) ;
#39650=CARTESIAN_POINT ( 'NONE',  ( 10.91775413003093931, 21.70171378149917985, -9.188101187500004485 ) ) ;
#39658=CARTESIAN_POINT ( 'NONE',  ( 67.41069134358542669, 70.04696837240071261, -4.305487806446024446E-08 ) ) ;
#39663=ORIENTED_EDGE ( 'NONE', *, *, #76116, .F. ) ;
#39668=CARTESIAN_POINT ( 'NONE',  ( 79.23201746742373075, 59.47846325219751407, -16.53522573291432352 ) ) ;
#39670=CARTESIAN_POINT ( 'NONE',  ( 80.82248141129124974, 43.03714829935063335, 9.686067628345497837 ) ) ;
#39678=CARTESIAN_POINT ( 'NONE',  ( 73.67041371685652962, 62.60474759977234527, 14.58206332630679292 ) ) ;
#39679=VECTOR ( 'NONE', #48554, 1000.000000000000114 ) ;
#39682=ORIENTED_EDGE ( 'NONE', *, *, #17833, .F. ) ;
#39683=CARTESIAN_POINT ( 'NONE',  ( 88.05624235485146301, 44.55787864911079765, -5.145732200269208967 ) ) ;
#39684=LINE ( 'NONE', #16909, #70799 ) ;
#39687=CARTESIAN_POINT ( 'NONE',  ( 82.53534059687447666, 53.28184184896795017, -15.31749960034531099 ) ) ;
#39690=CARTESIAN_POINT ( 'NONE',  ( 17.99393647837114329, 33.49540643055186706, 3.479690158560446702E-15 ) ) ;
#39695=ORIENTED_EDGE ( 'NONE', *, *, #49987, .F. ) ;
#39700=CARTESIAN_POINT ( 'NONE',  ( 85.03726002374489212, 45.61754386869292688, -9.156370252284901312 ) ) ;
#39712=CARTESIAN_POINT ( 'NONE',  ( 82.33219852380105408, 40.34800253957620697, -1.053958929052360549 ) ) ;
#39713=CARTESIAN_POINT ( 'NONE',  ( 14.35886136108867994, 13.45404122711132011, -8.090169943749478065 ) ) ;
#39716=CARTESIAN_POINT ( 'NONE',  ( 75.62574292670869625, 65.55640874641136406, 13.80250227997792756 ) ) ;
#39723=CARTESIAN_POINT ( 'NONE',  ( 83.25269581296497279, 46.42390702885197129, -11.11998686039522433 ) ) ;
#39724=CARTESIAN_POINT ( 'NONE',  ( 23.53456118939196529, 35.36126292948896577, 6.180339887498949913 ) ) ;
#39726=CARTESIAN_POINT ( 'NONE',  ( 74.25334530965831448, 67.88333409418525832, -11.69134486559788044 ) ) ;
#39729=ORIENTED_EDGE ( 'NONE', *, *, #56731, .T. ) ;
#39740=EDGE_CURVE ( 'NONE', #90942, #23100, #64507, .T. ) ;
#39744=CARTESIAN_POINT ( 'NONE',  ( 68.75179611904260923, 68.50344063802555183, 6.907652022257806834 ) ) ;
#39746=CARTESIAN_POINT ( 'NONE',  ( 65.74726825304114186, 69.08659106095529978, 2.128305819671951817E-12 ) ) ;
#39747=ORIENTED_EDGE ( 'NONE', *, *, #82806, .F. ) ;
#39749=CARTESIAN_POINT ( 'NONE',  ( 73.67824366217406862, 55.52431661998091528, 16.58293631993679540 ) ) ;
#39752=CARTESIAN_POINT ( 'NONE',  ( 13.72994409607376731, 16.43085787977761569, -9.188101187500008038 ) ) ;
#39755=PLANE ( 'NONE',  #82429 ) ;
#39762=DIRECTION ( 'NONE',  ( 0.2359789242578316237, 0.9717581732643758574, 0.000000000000000000 ) ) ;
#39764=VERTEX_POINT ( 'NONE', #9735 ) ;
#39771=CARTESIAN_POINT ( 'NONE',  ( 83.68684867813932726, 42.36207227428623412, 5.946836090295558819 ) ) ;
#39777=CARTESIAN_POINT ( 'NONE',  ( 37.65389587561885776, 30.24335787977765833, -9.188101187500008038 ) ) ;
#39778=CARTESIAN_POINT ( 'NONE',  ( 73.08568754922542610, 70.50375409671433147, -7.993246346743384301 ) ) ;
#39783=ORIENTED_EDGE ( 'NONE', *, *, #74094, .T. ) ;
#39784=CARTESIAN_POINT ( 'NONE',  ( 79.57595289148407858, 59.38824344631919416, 16.55667218292645870 ) ) ;
#39785=CARTESIAN_POINT ( 'NONE',  ( 83.53204454370725784, 52.39401912150449903, -15.17729711222452238 ) ) ;
#39789=CARTESIAN_POINT ( 'NONE',  ( 43.45144817956826699, 30.80170272979930601, 7.433330006724137462 ) ) ;
#39793=ORIENTED_EDGE ( 'NONE', *, *, #87572, .T. ) ;
#39797=CARTESIAN_POINT ( 'NONE',  ( 77.22954108468842094, 49.67394351277923192, -14.99406558715285165 ) ) ;
#39799=CARTESIAN_POINT ( 'NONE',  ( 87.09644473823584576, 45.85687564672072369, -8.636203292310963064 ) ) ;
#39806=CARTESIAN_POINT ( 'NONE',  ( 82.53920793150861357, 41.02048457221435740, 1.071569650286623210 ) ) ;
#39807=B_SPLINE_CURVE_WITH_KNOTS ( 'NONE', 3,
 ( #57011, #4316, #43807, #34228, #28114, #87990, #80371, #10942, #96071, #42307, #80882, #34716, #96572, #41812, #99032, #7303, #38184, #68604, #76238, #91961, #36205, #30613, #36702, #45788, #77208, #83352, #75233, #59495, #90473, #13918, #60489 ),
 .UNSPECIFIED., .F., .F.,
 ( 4, 3, 3, 3, 3, 3, 3, 3, 3, 3, 4 ),
 ( 0.000000000000000000, 0.1333490885032358464, 0.3007194338854307092, 0.4699862290245053198, 0.5844252810809311693, 0.6686540514502750110, 0.7354980260655511470, 0.8028463152565725736, 0.8633854507757335872, 0.9437142632667383513, 1.000000000000000000 ),
 .UNSPECIFIED. ) ;
#39814=CARTESIAN_POINT ( 'NONE',  ( 42.56377214068922399, 30.28920272979930672, -7.433330006724141015 ) ) ;
#39816=ADVANCED_FACE ( 'NONE', ( #21678 ), #19340, .T. ) ;
#39817=CARTESIAN_POINT ( 'NONE',  ( 85.74775437209392237, 48.65322352004045570, -12.36257617231559180 ) ) ;
#39820=ADVANCED_FACE ( 'NONE', ( #14074 ), #88268, .T. ) ;
#39823=CARTESIAN_POINT ( 'NONE',  ( 73.20519886181777736, 66.25595127750490576, 12.42694502862597083 ) ) ;
#39824=CARTESIAN_POINT ( 'NONE',  ( 80.71670901379776808, 43.21196966927421101, 9.964580085028348577 ) ) ;
#39825=CARTESIAN_POINT ( 'NONE',  ( 77.83148668010572635, 49.86468963568243851, 15.45682205838144796 ) ) ;
#39831=CARTESIAN_POINT ( 'NONE',  ( 66.06214068257197880, 68.71579393632852373, -0.4716098740908712950 ) ) ;
#39832=EDGE_LOOP ( 'NONE', ( #71390, #1344, #53423, #39695 ) ) ;
#39849=ADVANCED_FACE ( 'NONE', ( #84020 ), #14579, .T. ) ;
#39850=CARTESIAN_POINT ( 'NONE',  ( 85.38599379065072981, 47.65918632720038062, 11.17564927697190136 ) ) ;
#39851=CARTESIAN_POINT ( 'NONE',  ( 74.39841895140679640, 68.21392270468032848, 11.95628786500076579 ) ) ;
#39852=CARTESIAN_POINT ( 'NONE',  ( 74.39150450060409980, 68.40979575363469678, 11.28709398736407721 ) ) ;
#39853=CARTESIAN_POINT ( 'NONE',  ( 71.56705445201096438, 71.62942160774694855, -3.393990791292070597 ) ) ;
#39856=DIRECTION ( 'NONE',  ( -0.7467472232290888190, 0.000000000000000000, 0.6651079495838592148 ) ) ;
#39861=CARTESIAN_POINT ( 'NONE',  ( 84.83678198214029464, 50.32733779148675524, -13.41632123680453148 ) ) ;
#39864=CARTESIAN_POINT ( 'NONE',  ( 66.96593609093110899, 67.02900701502181846, 8.585446814251463721 ) ) ;
#39865=CARTESIAN_POINT ( 'NONE',  ( 75.83659763066778225, 51.68804710209467856, 15.74957237791803699 ) ) ;
#39867=ADVANCED_FACE ( 'NONE', ( #15544 ), #32260, .T. ) ;
#39873=CARTESIAN_POINT ( 'NONE',  ( 80.15404930735284950, 58.24487849859600885, -16.60713908503101521 ) ) ;
#39878=CARTESIAN_POINT ( 'NONE',  ( 88.20050489759562140, 44.09937366127426372, 0.5204581161859789251 ) ) ;
#39879=ADVANCED_FACE ( 'NONE', ( #54536 ), #76861, .T. ) ;
#39880=CARTESIAN_POINT ( 'NONE',  ( 84.19158505125736269, 49.36735266572484448, -13.01182045415430011 ) ) ;
#39881=CARTESIAN_POINT ( 'NONE',  ( 81.65367170574366185, 42.93584830628305582, -8.967313168971410065 ) ) ;
#39882=CARTESIAN_POINT ( 'NONE',  ( 71.64387245797139769, 71.15203705842421300, -6.128722539184691342 ) ) ;
#39885=CARTESIAN_POINT ( 'NONE',  ( 29.48197064213787044, 19.94754757982090609, 5.678558825948272215 ) ) ;
#39888=CARTESIAN_POINT ( 'NONE',  ( 14.44138481658839090, 10.19860640527290663, 2.839279412974134775 ) ) ;
#39890=CARTESIAN_POINT ( 'NONE',  ( 76.67779265155198232, 63.58935824677200088, 15.33226443842420927 ) ) ;
#39894=CARTESIAN_POINT ( 'NONE',  ( 73.71491122270572305, 65.62341685233879218, 13.03582331581120002 ) ) ;
#39896=ADVANCED_FACE ( 'NONE', ( #9476 ), #2898, .T. ) ;
#39903=CARTESIAN_POINT ( 'NONE',  ( 76.92873890057781239, 49.89429371730488327, 15.13083596839045519 ) ) ;
#39908=CARTESIAN_POINT ( 'NONE',  ( 72.31018532003172083, 68.81932238651856437, -9.557321504549943114 ) ) ;
#39912=CARTESIAN_POINT ( 'NONE',  ( 77.21491844529388970, 44.98415679381832888, 0.000000000000000000 ) ) ;
#39916=CARTESIAN_POINT ( 'NONE',  ( 27.86299091144838869, 21.80170272979927404, 7.433330006724137462 ) ) ;
#39917=CARTESIAN_POINT ( 'NONE',  ( 79.80790316897787307, 44.74020498821185043, 11.30572903481763092 ) ) ;
#39919=CARTESIAN_POINT ( 'NONE',  ( 75.23790730487549183, 66.45095094376505074, -13.14850644163485605 ) ) ;
#39920=CARTESIAN_POINT ( 'NONE',  ( 79.92738415168659571, 49.14675435996891650, -14.16998936058186409 ) ) ;
#39921=VERTEX_POINT ( 'NONE', #80417 ) ;
#39926=CARTESIAN_POINT ( 'NONE',  ( 68.20804129788332659, 65.51386583450461387, 10.45502995425724357 ) ) ;
#39927=CARTESIAN_POINT ( 'NONE',  ( 67.69593324464777595, 65.81863650441331970, -10.57774228775840974 ) ) ;
#39928=CARTESIAN_POINT ( 'NONE',  ( 81.73360701239045056, 55.69478791075532342, -15.98344718738445991 ) ) ;
#39941=AXIS2_PLACEMENT_3D ( 'NONE', #70150, #63066, #53946 ) ;
#39946=CARTESIAN_POINT ( 'NONE',  ( 79.93105292411557627, 44.72761662377413927, -11.22918178349264551 ) ) ;
#39950=CARTESIAN_POINT ( 'NONE',  ( 81.25645528111445515, 55.75359181263093689, 16.38715272843555226 ) ) ;
#39951=CARTESIAN_POINT ( 'NONE',  ( 78.69678629884484167, 48.79589717492678602, -14.33111529692661890 ) ) ;
#39964=CARTESIAN_POINT ( 'NONE',  ( 87.58565344165421607, 44.63638434534234278, 4.979176973005301932 ) ) ;
#39965=ORIENTED_EDGE ( 'NONE', *, *, #70963, .F. ) ;
#39971=CARTESIAN_POINT ( 'NONE',  ( 71.70607908956505128, 59.57266618253179757, -15.70866010994346595 ) ) ;
#39980=CARTESIAN_POINT ( 'NONE',  ( 79.14312167556931854, 57.64441083166269664, 0.000000000000000000 ) ) ;
#39982=CARTESIAN_POINT ( 'NONE',  ( 84.06109941699628507, 51.61974178474097386, 14.72645736870185651 ) ) ;
#39987=CARTESIAN_POINT ( 'NONE',  ( 73.65144064479261488, 55.37666558215569523, 16.11406811069710443 ) ) ;
#39989=CARTESIAN_POINT ( 'NONE',  ( 33.73794667537109149, 19.28848085856232686, 1.475505719884397138E-15 ) ) ;
#39990=B_SPLINE_CURVE_WITH_KNOTS ( 'NONE', 3,
 ( #20634, #30589, #43909, #78195, #61475, #92423, #22973, #84823, #36311, #51519 ),
 .UNSPECIFIED., .F., .F.,
 ( 4, 2, 2, 2, 4 ),
 ( 0.000000000000000000, 0.2500000000000000000, 0.5000000000000000000, 0.7500000000000000000, 1.000000000000000000 ),
 .UNSPECIFIED. ) ;
#40001=EDGE_CURVE ( 'NONE', #51335, #86428, #72804, .T. ) ;
#40003=CARTESIAN_POINT ( 'NONE',  ( 81.87492437171775350, 41.18014386121605241, 5.628296993625497180 ) ) ;
#40006=DIRECTION ( 'NONE',  ( -0.8660254037844379305, -0.5000000000000014433, -0.000000000000000000 ) ) ;
#40007=CARTESIAN_POINT ( 'NONE',  ( 34.04375301561599798, 21.78380873178788946, -6.180339887498949025 ) ) ;
#40011=CARTESIAN_POINT ( 'NONE',  ( 81.68759648889933089, 55.58869686435339474, 15.96161034574013904 ) ) ;
#40015=CARTESIAN_POINT ( 'NONE',  ( 86.98925081226386169, 46.40596221211884398, -8.809588356812493970 ) ) ;
#40018=PLANE ( 'NONE',  #97603 ) ;
#40032=CARTESIAN_POINT ( 'NONE',  ( 22.39139443204644664, 24.87878583063842086, -9.188101187500006262 ) ) ;
#40037=CARTESIAN_POINT ( 'NONE',  ( 36.54023192077972482, 39.83478043621391151, -8.090169943749479842 ) ) ;
#40038=CARTESIAN_POINT ( 'NONE',  ( 12.18311320154372801, 9.960047579820882291, -5.678558825948275768 ) ) ;
#40039=CARTESIAN_POINT ( 'NONE',  ( 72.76330120127171597, 59.97484020424936091, -15.29220549501611259 ) ) ;
#40040=CARTESIAN_POINT ( 'NONE',  ( 71.94509386275791485, 72.64380087153907084, -0.7818115889975479904 ) ) ;
#40043=CARTESIAN_POINT ( 'NONE',  ( 71.68256357803392120, 71.39422369264570989, -4.342351502620559245 ) ) ;
#40050=CARTESIAN_POINT ( 'NONE',  ( 81.70142411701870344, 42.24897359289763443, -6.860144861392842408 ) ) ;
#40051=ORIENTED_EDGE ( 'NONE', *, *, #60560, .T. ) ;
#40054=CARTESIAN_POINT ( 'NONE',  ( 72.80354425691618303, 56.98564078552313106, -16.40249550304353221 ) ) ;
#40064=CARTESIAN_POINT ( 'NONE',  ( 31.32709252658613508, 23.80170272979928114, 7.433330006724137462 ) ) ;
#40066=CARTESIAN_POINT ( 'NONE',  ( 68.42576582225177617, 70.23325100905495333, -3.401356179981240402 ) ) ;
#40068=CARTESIAN_POINT ( 'NONE',  ( 74.04232911944542650, 68.62205345152153768, 10.92009053252770734 ) ) ;
#40086=CARTESIAN_POINT ( 'NONE',  ( 76.00671579873834105, 65.53670222276893753, 13.92362488849856739 ) ) ;
#40093=CARTESIAN_POINT ( 'NONE',  ( 84.17777703092687602, 41.88998738275029154, -0.4096941387594014161 ) ) ;
#40098=CARTESIAN_POINT ( 'NONE',  ( 83.65902391768069890, 51.64235791857056768, -14.83937710116058639 ) ) ;
#40100=EDGE_LOOP ( 'NONE', ( #70538, #60427, #59860, #45831 ) ) ;
#40103=( BOUNDED_CURVE ( )  B_SPLINE_CURVE ( 2, ( #25633, #8920, #78842, #819, #31695, #9425, #40300, #71242, #63618, #79374, #62603, #9937, #2338 ),
 .UNSPECIFIED., .F., .T. ) 
 B_SPLINE_CURVE_WITH_KNOTS ( ( 3, 2, 2, 2, 2, 2, 3 ),
 ( 0.4625000000000000222, 0.4650000000000000244, 0.4699999999999999734, 0.4749999999999999778, 0.4799999999999999822, 0.4849999999999999867, 0.4874999999999999889 ),
 .UNSPECIFIED. ) 
 CURVE ( )  GEOMETRIC_REPRESENTATION_ITEM ( )  RATIONAL_B_SPLINE_CURVE ( ( 0.9755282581475768211, 0.9755282581475768211, 1.000000000000000000, 0.9510565162951535312, 1.000000000000000000, 0.9510565162951535312, 1.000000000000000000, 0.9510565162951535312, 1.000000000000000000, 0.9510565162951535312, 1.000000000000000000, 0.9755282581475768211, 0.9755282581475768211 ) ) 
 REPRESENTATION_ITEM ( '' )  );
#40110=LINE ( 'NONE', #16327, #82100 ) ;
#40114=CARTESIAN_POINT ( 'NONE',  ( 75.19165711449073797, 61.00119534238836394, -15.88670729749929578 ) ) ;
#40115=CARTESIAN_POINT ( 'NONE',  ( 87.93887446415499198, 44.76116579897428238, -4.704258403839747693 ) ) ;
#40128=CARTESIAN_POINT ( 'NONE',  ( 87.94090206498698592, 44.79893454962108734, 4.853345500095875842 ) ) ;
#40130=CARTESIAN_POINT ( 'NONE',  ( 10.48369258086752787, 24.79103043416547791, 8.090169943749478065 ) ) ;
#40139=CARTESIAN_POINT ( 'NONE',  ( 13.32519098795206780, 19.64441083166259361, -10.00000000000000533 ) ) ;
#40147=CARTESIAN_POINT ( 'NONE',  ( 37.97865540203802937, 30.43085787977766188, -9.188101187500008038 ) ) ;
#40154=CARTESIAN_POINT ( 'NONE',  ( 66.08354252224813763, 69.04860372161006410, 2.576220482760897212 ) ) ;
#40160=CARTESIAN_POINT ( 'NONE',  ( 6.852252633650415703, 22.14336893147753571, 7.433330006724141015 ) ) ;
#40162=VECTOR ( 'NONE', #59887, 1000.000000000000114 ) ;
#40165=DIRECTION ( 'NONE',  ( 0.4972609476841349796, -0.8612812260087746585, 0.1045284632676570652 ) ) ;
#40166=CARTESIAN_POINT ( 'NONE',  ( 66.10228174246465471, 68.64626758112467542, 4.271897712866680408 ) ) ;
#40167=CARTESIAN_POINT ( 'NONE',  ( 87.90004739103230236, 45.00901072816738235, 6.408389154966701362 ) ) ;
#40171=EDGE_LOOP ( 'NONE', ( #49087, #92573, #77996, #26655 ) ) ;
#40173=CARTESIAN_POINT ( 'NONE',  ( 85.87397059692905543, 47.49916506119975423, 10.81363086110046190 ) ) ;
#40175=CARTESIAN_POINT ( 'NONE',  ( 25.97889144642132919, 17.12755873383626692, -6.180339887498949025 ) ) ;
#40177=ORIENTED_EDGE ( 'NONE', *, *, #39513, .F. ) ;
#40180=CARTESIAN_POINT ( 'NONE',  ( 19.03539854152464628, 16.15404122711133184, 8.090169943749479842 ) ) ;
#40187=ORIENTED_EDGE ( 'NONE', *, *, #9251, .F. ) ;
#40190=EDGE_LOOP ( 'NONE', ( #96307, #14445, #70919, #42498, #89955 ) ) ;
#40191=CARTESIAN_POINT ( 'NONE',  ( 74.19807589368119238, 65.03689309259050333, 13.58590908905372352 ) ) ;
#40196=CARTESIAN_POINT ( 'NONE',  ( 82.47798474638348409, 46.77785881030774107, 11.77598945167534161 ) ) ;
#40197=CARTESIAN_POINT ( 'NONE',  ( 70.93889008731977697, 68.42943192159272314, 9.010113148257101301 ) ) ;
#40202=CARTESIAN_POINT ( 'NONE',  ( 26.13094010387951371, 20.80170272979927049, 7.433330006724137462 ) ) ;
#40205=DIRECTION ( 'NONE',  ( 0.2702110370271901818, 0.9515975153008194853, 0.1464519181915934776 ) ) ;
#40207=DIRECTION ( 'NONE',  ( -0.8660254037844379305, -0.5000000000000014433, -0.000000000000000000 ) ) ;
#40214=CARTESIAN_POINT ( 'NONE',  ( 71.96330895120250659, 59.12713099295166330, 15.87581820695405455 ) ) ;
#40218=CARTESIAN_POINT ( 'NONE',  ( 74.92223598134692963, 66.83043205548882781, -13.20899543911387930 ) ) ;
#40221=LINE ( 'NONE', #32132, #83964 ) ;
#40231=CARTESIAN_POINT ( 'NONE',  ( 75.59035046094346910, 65.27760725598233194, 14.33377162271303540 ) ) ;
#40235=ORIENTED_EDGE ( 'NONE', *, *, #70081, .F. ) ;
#40238=CARTESIAN_POINT ( 'NONE',  ( 68.74458750670157769, 70.20414421525195792, 1.682888519748420908 ) ) ;
#40239=FACE_OUTER_BOUND ( 'NONE', #99253, .T. ) ;
#40243=CARTESIAN_POINT ( 'NONE',  ( 74.43781217983632814, 68.33376311026280803, -11.38208125649862801 ) ) ;
#40253=CARTESIAN_POINT ( 'NONE',  ( 66.75734579356596043, 67.35081300050364916, -6.869089300961301880 ) ) ;
#40254=CARTESIAN_POINT ( 'NONE',  ( 68.81249350320682368, 63.82265338634812935, -12.23679878556980150 ) ) ;
#40258=CARTESIAN_POINT ( 'NONE',  ( 72.89924121220336417, 67.41618724535075557, 11.90048241206199897 ) ) ;
#40262=ORIENTED_EDGE ( 'NONE', *, *, #26433, .F. ) ;
#40266=CARTESIAN_POINT ( 'NONE',  ( 14.05589992062122917, 20.06628583063840310, -9.188101187500006262 ) ) ;
#40277=CARTESIAN_POINT ( 'NONE',  ( 68.47753283764532739, 66.06621294245498177, -10.79241679792292530 ) ) ;
#40278=CARTESIAN_POINT ( 'NONE',  ( 26.00142736512681907, 15.41603393254325560, -1.583844403245362020 ) ) ;
#40280=ORIENTED_EDGE ( 'NONE', *, *, #2311, .F. ) ;
#40289=CARTESIAN_POINT ( 'NONE',  ( 40.50696180670117741, 29.10170272979929962, -7.433330006724141015 ) ) ;
#40290=CARTESIAN_POINT ( 'NONE',  ( 84.21805166483638061, 41.46905487699226711, 1.456718203712574322 ) ) ;
#40295=CARTESIAN_POINT ( 'NONE',  ( 83.07746382761068560, 43.99571311473679458, -9.259344712981764758 ) ) ;
#40296=ORIENTED_EDGE ( 'NONE', *, *, #90378, .T. ) ;
#40297=CARTESIAN_POINT ( 'NONE',  ( 79.55938800887707885, 59.45545654668635649, 16.55147640184673463 ) ) ;
#40300=CARTESIAN_POINT ( 'NONE',  ( 22.85147042958088193, 25.14441083166261137, 10.00000000000000533 ) ) ;
#40303=CARTESIAN_POINT ( 'NONE',  ( 72.18990340680744566, 72.03918383723207342, -3.149060597287207219 ) ) ;
#40304=CARTESIAN_POINT ( 'NONE',  ( 80.21951685124797393, 44.77929739833423639, 11.12462274611551116 ) ) ;
#40310=CARTESIAN_POINT ( 'NONE',  ( 77.22023733200087747, 49.61776833328874403, -15.48932739092899347 ) ) ;
#40311=ORIENTED_EDGE ( 'NONE', *, *, #67907, .F. ) ;
#40314=CARTESIAN_POINT ( 'NONE',  ( 78.80037227254219090, 51.26846376261736538, 15.25722946762347298 ) ) ;
#40316=CARTESIAN_POINT ( 'NONE',  ( 76.90746743093833970, 62.93938289886319382, -15.23233999435670150 ) ) ;
#40326=CARTESIAN_POINT ( 'NONE',  ( 43.68478726420265446, 28.14754757982094802, -5.678558825948276656 ) ) ;
#40329=CARTESIAN_POINT ( 'NONE',  ( 84.56191477375736554, 43.45664822029007723, -7.163795276308541737 ) ) ;
#40330=ORIENTED_EDGE ( 'NONE', *, *, #75706, .T. ) ;
#40339=CARTESIAN_POINT ( 'NONE',  ( 34.62385580964452458, 25.15404122711136026, 8.090169943749479842 ) ) ;
#40344=ORIENTED_EDGE ( 'NONE', *, *, #9117, .T. ) ;
#40359=CARTESIAN_POINT ( 'NONE',  ( 87.87749860556357362, 43.91202660816024661, 0.3985875973167696262 ) ) ;
#40364=CARTESIAN_POINT ( 'NONE',  ( 68.24846459439849866, 69.97058443567007657, 1.257665481745562586 ) ) ;
#40367=CARTESIAN_POINT ( 'NONE',  ( 67.16288355292338963, 68.85776602768420673, 5.438331637600131607 ) ) ;
#40368=CARTESIAN_POINT ( 'NONE',  ( 88.13402233310422673, 44.37312773088997631, -4.489783613381812089 ) ) ;
#40375=CARTESIAN_POINT ( 'NONE',  ( 73.80638704669732419, 68.31061168272384521, -11.57820046455322149 ) ) ;
#40379=CARTESIAN_POINT ( 'NONE',  ( 73.39426628506285510, 56.64220877263274190, -16.01712807892389634 ) ) ;
#40384=CARTESIAN_POINT ( 'NONE',  ( 77.00376392975798012, 63.39239755058648029, -15.46687034352795109 ) ) ;
#40387=CARTESIAN_POINT ( 'NONE',  ( 88.44311045277898131, 43.83777140359737956, 0.09123111681703632847 ) ) ;
#40389=CARTESIAN_POINT ( 'NONE',  ( 80.93613592869992601, 42.95327845849681836, -9.503115154567232992 ) ) ;
#40390=CARTESIAN_POINT ( 'NONE',  ( 70.57897896622060330, 71.00804091966597298, -4.942816957066797023 ) ) ;
#40394=CARTESIAN_POINT ( 'NONE',  ( 28.23826220571969969, 31.70171378149920471, -9.188101187500004485 ) ) ;
#40395=CARTESIAN_POINT ( 'NONE',  ( 81.27194768136315872, 46.27379842166399726, 12.52033010236089261 ) ) ;
#40396=CARTESIAN_POINT ( 'NONE',  ( 79.69317059041301832, 47.75519670552719731, -13.50432480851453931 ) ) ;
#40398=CARTESIAN_POINT ( 'NONE',  ( 23.64951029700315743, 14.44966523072494624, -2.296566073217252530E-15 ) ) ;
#40400=DIRECTION ( 'NONE',  ( -0.8660254037844379305, -0.5000000000000014433, -0.000000000000000000 ) ) ;
#40407=EDGE_LOOP ( 'NONE', ( #53412, #32614, #9174, #10224, #75729 ) ) ;
#40419=CARTESIAN_POINT ( 'NONE',  ( 73.01258037670726253, 68.72995673837564823, -10.14057597975430447 ) ) ;
#40423=CARTESIAN_POINT ( 'NONE',  ( 79.48876273271771709, 46.38894273206648222, -12.71961528548988873 ) ) ;
#40427=CARTESIAN_POINT ( 'NONE',  ( 22.55378097864968012, 33.99752408145592852, 5.678558825948276656 ) ) ;
#40428=CARTESIAN_POINT ( 'NONE',  ( 84.60239308390620749, 50.60453406874029270, -14.06751209996561158 ) ) ;
#40429=CARTESIAN_POINT ( 'NONE',  ( 83.78198294410601932, 48.18673714097705840, -12.33272353593454085 ) ) ;
#40434=B_SPLINE_CURVE_WITH_KNOTS ( 'NONE', 3,
 ( #29781, #4488, #90639, #20201, #66293, #67784, #44467, #29294, #75909, #60653, #58667, #27794, #89639, #23656, #7988, #69770, #84029, #23162, #16073, #99692, #92134, #22687, #22182, #38864, #378, #15063, #46975, #76400, #100199, #53075, #69271, #39351, #45466, #61166, #31267, #53566, #68768, #46456, #62153, #14588, #70265, #6976, #38361, #45953, #37859, #76870 ),
 .UNSPECIFIED., .F., .F.,
 ( 4, 1, 1, 1, 2, 2, 1, 1, 1, 2, 2, 1, 1, 2, 2, 1, 1, 2, 2, 1, 1, 2, 2, 1, 2, 2, 1, 2, 2, 4 ),
 ( 0.000000000000000000, 0.06250000000000216493, 0.09375000000000272005, 0.1093750000000035388, 0.1171875000000033029, 0.1250000000000030809, 0.1874999999999965861, 0.2187499999999915623, 0.2343749999999891476, 0.2421874999999873990, 0.2499999999999856504, 0.3124999999999859557, 0.3437499999999861777, 0.3593749999999880096, 0.3749999999999898415, 0.4374999999999897304, 0.4687499999999908407, 0.4843749999999908962, 0.4999999999999909517, 0.5624999999999934497, 0.5937499999999930056, 0.6093749999999941158, 0.6249999999999952260, 0.6874999999999963363, 0.7187499999999952260, 0.7499999999999941158, 0.8124999999999952260, 0.8437499999999956701, 0.8749999999999961142, 1.000000000000000000 ),
 .UNSPECIFIED. ) ;
#40436=ORIENTED_EDGE ( 'NONE', *, *, #83221, .F. ) ;
#40438=CARTESIAN_POINT ( 'NONE',  ( 67.71951918407867765, 65.69802484793109443, 10.71695699751798969 ) ) ;
#40440=CARTESIAN_POINT ( 'NONE',  ( 81.76940595752934371, 55.36688792037507056, -15.93096493606815933 ) ) ;
#40446=CARTESIAN_POINT ( 'NONE',  ( 71.97605894070565569, 62.66438405307972204, -14.59188024022812691 ) ) ;
#40447=CARTESIAN_POINT ( 'NONE',  ( 79.49274628814450239, 59.57836040576013659, 16.53926144102299034 ) ) ;
#40451=CARTESIAN_POINT ( 'NONE',  ( 78.12682272674805972, 61.49995998885079729, -16.15539878443392396 ) ) ;
#40456=CARTESIAN_POINT ( 'NONE',  ( 80.05471186046345622, 44.29272515403749821, -11.46072743220592294 ) ) ;
#40459=CARTESIAN_POINT ( 'NONE',  ( 82.28273451354495194, 47.89750625978791021, -12.72550930769195254 ) ) ;
#40462=ORIENTED_EDGE ( 'NONE', *, *, #47713, .T. ) ;
#40465=ORIENTED_EDGE ( 'NONE', *, *, #98665, .F. ) ;
#40466=B_SPLINE_SURFACE_WITH_KNOTS ( 'NONE', 3, 1, ( 
 ( #84652, #70409 ),
 ( #78531, #9115 ),
 ( #92745, #78026 ),
 ( #93759, #15700 ),
 ( #24317, #55192 ),
 ( #30912, #31404 ),
 ( #86176, #62291 ),
 ( #22815, #39987 ),
 ( #70928, #32414 ),
 ( #93247, #2017 ),
 ( #55683, #38500 ),
 ( #1533, #23300 ),
 ( #17203, #54691 ),
 ( #15195, #48105 ),
 ( #79048, #92267 ),
 ( #9637, #54189 ),
 ( #53695, #46598 ),
 ( #46093, #77005 ),
 ( #7611, #61799 ),
 ( #69415, #77531 ),
 ( #8124, #38997 ),
 ( #57195, #71927 ),
 ( #19728, #25306 ),
 ( #27318, #65793 ),
 ( #96752, #26321 ),
 ( #19244, #88174 ),
 ( #87189, #18721 ),
 ( #50109, #42007 ),
 ( #56194, #17722 ),
 ( #72940, #48625 ),
 ( #41499, #34409 ) ),
 .UNSPECIFIED., .F., .F., .F.,
 ( 4, 3, 3, 3, 3, 3, 3, 3, 3, 3, 4 ),
 ( 2, 2 ),
 ( 0.000000000000000000, 0.1122669598086659254, 0.2243161639709550792, 0.3396355846218998553, 0.4553962076584952556, 0.5677860799922195278, 0.6749047109689478852, 0.7773884377078161823, 0.8775581155834035751, 0.9782364162377661376, 1.000000000000000000 ),
 ( 0.000000000000000000, 1.000000000000000000 ),
 .UNSPECIFIED. ) ;
#40467=CARTESIAN_POINT ( 'NONE',  ( 80.44215978124604760, 58.39441083166272506, 0.000000000000000000 ) ) ;
#40471=CARTESIAN_POINT ( 'NONE',  ( 75.91641493099308491, 64.71284702731330185, -14.30921724464636924 ) ) ;
#40472=CARTESIAN_POINT ( 'NONE',  ( 68.20353262459525467, 69.11303344777483915, -4.901384820270958897 ) ) ;
#40474=CARTESIAN_POINT ( 'NONE',  ( 88.26872550477153823, 44.38513711945522289, 4.282355379009170626 ) ) ;
#40476=CARTESIAN_POINT ( 'NONE',  ( 85.86066238541921791, 43.85667369948165373, -5.309618687222620537 ) ) ;
#40478=CARTESIAN_POINT ( 'NONE',  ( 80.75588300432519873, 45.91452481213949710, 11.84376094130757018 ) ) ;
#40488=CARTESIAN_POINT ( 'NONE',  ( 84.69116302952653541, 43.17850746977291010, 5.277877534678879989 ) ) ;
#40490=CARTESIAN_POINT ( 'NONE',  ( 83.46272733064347449, 51.93221652752757933, 15.00972995268700139 ) ) ;
#40498=CARTESIAN_POINT ( 'NONE',  ( 31.67936943677743855, 23.45404122711135386, -8.090169943749478065 ) ) ;
#40499=CARTESIAN_POINT ( 'NONE',  ( 77.95436975687957215, 48.11784896437987413, 14.20357318872345331 ) ) ;
#40506=CARTESIAN_POINT ( 'NONE',  ( 82.51799120075359895, 48.96200246141732038, 13.33826670467029984 ) ) ;
#40509=CARTESIAN_POINT ( 'NONE',  ( 33.41142024434631708, 24.45404122711135386, -8.090169943749478065 ) ) ;
#40510=CARTESIAN_POINT ( 'NONE',  ( 82.10237303103902207, 41.84040927510496033, 5.493823265887765928 ) ) ;
#40513=CARTESIAN_POINT ( 'NONE',  ( 31.01079167849261964, 40.83705186507756224, 3.090169943749475401 ) ) ;
#40521=CARTESIAN_POINT ( 'NONE',  ( 83.53052282221433700, 51.97849157102297823, 15.01265415031365258 ) ) ;
#40525=CARTESIAN_POINT ( 'NONE',  ( 72.75575765633803371, 66.35992158122787998, -12.11670373630936304 ) ) ;
#40532=EDGE_CURVE ( 'NONE', #69750, #63734, #40221, .T. ) ;
#40533=CARTESIAN_POINT ( 'NONE',  ( 67.30637966541804929, 66.39985843937958521, -8.834011029012955873 ) ) ;
#40539=CARTESIAN_POINT ( 'NONE',  ( 30.03287232231581072, 25.84335787977764554, 9.188101187500006262 ) ) ;
#40543=ORIENTED_EDGE ( 'NONE', *, *, #36810, .F. ) ;
#40544=CARTESIAN_POINT ( 'NONE',  ( 10.54248283575963008, 11.80170272979924206, 7.433330006724137462 ) ) ;
#40545=CARTESIAN_POINT ( 'NONE',  ( 78.23242879811255079, 58.04918888810001931, -16.20759052872706718 ) ) ;
#40546=CARTESIAN_POINT ( 'NONE',  ( 71.86256228778262312, 72.60615528678948749, -0.5650332253008888417 ) ) ;
#40550=CARTESIAN_POINT ( 'NONE',  ( 85.26988926578472672, 49.08626644514237114, 12.44667837020937995 ) ) ;
#40554=ORIENTED_EDGE ( 'NONE', *, *, #70081, .T. ) ;
#40558=CARTESIAN_POINT ( 'NONE',  ( 44.68504016816520164, 27.92755873383629961, 6.180339887498953466 ) ) ;
#40560=CARTESIAN_POINT ( 'NONE',  ( 72.71055119297287206, 57.13306343736743287, -15.89095181684541380 ) ) ;
#40561=CARTESIAN_POINT ( 'NONE',  ( 4.767924915890233706, 21.49103043416546654, -8.090169943749479842 ) ) ;
#40568=CARTESIAN_POINT ( 'NONE',  ( 34.69977369993912220, 22.96004757982091959, -5.678558825948276656 ) ) ;
#40569=CARTESIAN_POINT ( 'NONE',  ( 82.57480368249606784, 41.04376301281222794, 1.111617510708536205 ) ) ;
#40570=CARTESIAN_POINT ( 'NONE',  ( 78.55309808138584060, 47.92462935717776418, -14.48522603925180796 ) ) ;
#40572=CARTESIAN_POINT ( 'NONE',  ( 73.78595477147815984, 68.43622263357737268, 11.45456581244437011 ) ) ;
#40578=CARTESIAN_POINT ( 'NONE',  ( 75.66128580626863709, 58.22407134023451647, -16.00779004018875895 ) ) ;
#40583=CARTESIAN_POINT ( 'NONE',  ( 71.63782333154907178, 69.86052725181824030, -7.572626888899040232 ) ) ;
#40590=CARTESIAN_POINT ( 'NONE',  ( 83.61201429516752626, 42.51031818454811884, -6.362242280625504343 ) ) ;
#40591=CARTESIAN_POINT ( 'NONE',  ( 67.54027896650161722, 66.67046411983839960, 8.643862525530476404 ) ) ;
#40592=CARTESIAN_POINT ( 'NONE',  ( 71.32056415648651182, 65.32475367386736309, -12.23164579019822185 ) ) ;
#40603=CARTESIAN_POINT ( 'NONE',  ( 83.67142796774817270, 51.47602654951222689, -14.37994367775212012 ) ) ;
#40617=CARTESIAN_POINT ( 'NONE',  ( 85.52974044692305711, 48.30270382619246305, -11.71869337694238133 ) ) ;
#40619=CARTESIAN_POINT ( 'NONE',  ( 80.44297273216874089, 44.73620253192707708, -11.65665792466250039 ) ) ;
#40623=B_SPLINE_CURVE_WITH_KNOTS ( 'NONE', 3,
 ( #89740, #58769, #76849, #22664, #12203, #20303, #69247, #45932, #98307, #97813, #28381, #58284, #59260, #51701, #13208, #23135, #84496, #7446, #74518, #100175, #27889, #30761, #67381, #19810, #82649, #28897, #59775, #61641, #92591, #89261, #54030, #84986, #15531, #43066, #4593, #46431, #51177, #77360, #35488, #7965, #5097, #38838, #69744, #50677, #35978, #9462 ),
 .UNSPECIFIED., .F., .F.,
 ( 4, 1, 1, 1, 2, 2, 1, 1, 1, 2, 2, 1, 1, 2, 2, 1, 1, 2, 2, 1, 1, 2, 2, 1, 2, 2, 1, 2, 2, 4 ),
 ( 0.000000000000000000, 0.06249999999997488120, 0.09374999999996232181, 0.1093749999999545780, 0.1171874999999524686, 0.1249999999999503730, 0.1874999999999391320, 0.2187499999999332756, 0.2343749999999326095, 0.2421874999999322764, 0.2499999999999319433, 0.3124999999999383826, 0.3437499999999411027, 0.3593749999999437672, 0.3749999999999464317, 0.4374999999999532041, 0.4687499999999584221, 0.4843749999999609201, 0.4999999999999634737, 0.5624999999999631406, 0.5937499999999624745, 0.6093749999999615863, 0.6249999999999606981, 0.6874999999999623634, 0.7187499999999655831, 0.7499999999999688027, 0.8124999999999790168, 0.8437499999999847899, 0.8749999999999904521, 1.000000000000000000 ),
 .UNSPECIFIED. ) ;
#40627=CARTESIAN_POINT ( 'NONE',  ( 79.56977700121861119, 52.24079475247017257, -15.41399356243466379 ) ) ;
#40634=CARTESIAN_POINT ( 'NONE',  ( 11.95823279523498073, 29.83705186507753027, 3.090169943749475401 ) ) ;
#40637=CARTESIAN_POINT ( 'NONE',  ( 71.86822536019646179, 59.56647301316700549, -15.73804542241091475 ) ) ;
#40638=CARTESIAN_POINT ( 'NONE',  ( 66.46590124120757537, 67.88977592199039179, -6.664539190546268976 ) ) ;
#40644=PLANE ( 'NONE',  #32058 ) ;
#40650=CARTESIAN_POINT ( 'NONE',  ( 39.71070620960689723, 31.43085787977766898, -9.188101187500008038 ) ) ;
#40654=CARTESIAN_POINT ( 'NONE',  ( 35.02453322635827959, 23.14754757982091959, -5.678558825948276656 ) ) ;
#40657=CARTESIAN_POINT ( 'NONE',  ( 77.72205534048291042, 61.52847525230063042, 16.09962475150207339 ) ) ;
#40658=CARTESIAN_POINT ( 'NONE',  ( 65.83236371457655878, 68.94654938641845376, 2.326923034581525940 ) ) ;
#40659=ORIENTED_EDGE ( 'NONE', *, *, #67907, .T. ) ;
#40662=CARTESIAN_POINT ( 'NONE',  ( 15.30080465516770616, 11.76004757982088300, 5.678558825948272215 ) ) ;
#40664=CARTESIAN_POINT ( 'NONE',  ( 10.03310832875943603, 27.83396525600388571, -2.839279412974133887 ) ) ;
#40666=CARTESIAN_POINT ( 'NONE',  ( 84.83352707183692587, 50.23671165375215253, -13.78554283518410095 ) ) ;
#40668=ADVANCED_FACE ( 'NONE', ( #83771 ), #52814, .T. ) ;
#40672=CARTESIAN_POINT ( 'NONE',  ( 66.27522152577653003, 68.24883630604136897, 4.052617218417564615 ) ) ;
#40673=ADVANCED_FACE ( 'NONE', ( #14332 ), #83620, .T. ) ;
#40676=ORIENTED_EDGE ( 'NONE', *, *, #45585, .F. ) ;
#40679=CARTESIAN_POINT ( 'NONE',  ( 86.00254776313695970, 47.63876908572450475, 10.87982004645334122 ) ) ;
#40683=ORIENTED_EDGE ( 'NONE', *, *, #12801, .T. ) ;
#40684=CARTESIAN_POINT ( 'NONE',  ( 78.37845639280004661, 61.47534692751145968, -15.83465071172797067 ) ) ;
#40685=CARTESIAN_POINT ( 'NONE',  ( 79.18361146787275118, 59.08720699360743112, -16.21979195788916783 ) ) ;
#40686=CARTESIAN_POINT ( 'NONE',  ( 10.82157445631582249, 29.18080186712591839, 3.090169943749475401 ) ) ;
#40687=ORIENTED_EDGE ( 'NONE', *, *, #79519, .F. ) ;
#40695=VERTEX_POINT ( 'NONE', #72555 ) ;
#40697=CARTESIAN_POINT ( 'NONE',  ( 79.91647412519343163, 45.34541341733537934, 11.77874049927093658 ) ) ;
#40703=CARTESIAN_POINT ( 'NONE',  ( 81.53569239047196504, 44.59779901518734846, 10.21677624337819346 ) ) ;
#40706=CARTESIAN_POINT ( 'NONE',  ( 72.08205655898075292, 70.58418997119434835, 6.795652346931509769 ) ) ;
#40708=CARTESIAN_POINT ( 'NONE',  ( 82.68398936210410000, 53.28103025482077015, -15.29235669276918763 ) ) ;
#40712=CARTESIAN_POINT ( 'NONE',  ( 23.32475077058400004, 14.26216523072494446, -2.296566073217252530E-15 ) ) ;
#40716=ORIENTED_EDGE ( 'NONE', *, *, #3717, .F. ) ;
#40724=CARTESIAN_POINT ( 'NONE',  ( 67.16327201103491973, 67.73731889023999031, 6.573435314091262249 ) ) ;
#40729=CARTESIAN_POINT ( 'NONE',  ( 82.35941855622118624, 40.93148445005448366, -1.241598412671953922 ) ) ;
#40737=ORIENTED_EDGE ( 'NONE', *, *, #52182, .F. ) ;
#40739=CARTESIAN_POINT ( 'NONE',  ( 67.05324003527370280, 68.69434906313091460, 4.069319704320632169 ) ) ;
#40740=CARTESIAN_POINT ( 'NONE',  ( 83.25380727528489899, 42.56249626881286474, 5.709386246556279687 ) ) ;
#40743=CARTESIAN_POINT ( 'NONE',  ( 74.11971290936233459, 68.38772044953262252, -11.66991619212280895 ) ) ;
#40748=CARTESIAN_POINT ( 'NONE',  ( 82.78588454431675814, 44.52977094881507725, 9.342758750263890022 ) ) ;
#40763=CARTESIAN_POINT ( 'NONE',  ( 21.85012855468117721, 24.56628583063841376, 9.188101187500006262 ) ) ;
#40773=CARTESIAN_POINT ( 'NONE',  ( 86.28285115951177886, 47.67076295942541009, 10.74768692570409279 ) ) ;
#40776=CARTESIAN_POINT ( 'NONE',  ( 16.98118013718471886, 32.73705186507753950, -3.090169943749475845 ) ) ;
#40782=CARTESIAN_POINT ( 'NONE',  ( 83.87116762653428736, 51.60433200805344711, -14.38557393531113071 ) ) ;
#40783=ADVANCED_FACE ( 'NONE', ( #49719 ), #65421, .T. ) ;
#40785=CARTESIAN_POINT ( 'NONE',  ( 74.89921650030801459, 53.29654407186357901, -16.52566481002074639 ) ) ;
#40787=ORIENTED_EDGE ( 'NONE', *, *, #51901, .F. ) ;
#40790=CARTESIAN_POINT ( 'NONE',  ( 38.30580752471379213, 37.51421378149922958, -9.188101187500004485 ) ) ;
#40793=CARTESIAN_POINT ( 'NONE',  ( 77.72825959162678089, 61.57464001967338163, 16.09025617263268515 ) ) ;
#40798=CARTESIAN_POINT ( 'NONE',  ( 79.06677544641175359, 59.81915678714237572, 16.49560342610751462 ) ) ;
#40801=CARTESIAN_POINT ( 'NONE',  ( 83.03630717809630823, 50.34759745827115296, -13.97564751877582090 ) ) ;
#40803=VERTEX_POINT ( 'NONE', #76258 ) ;
#40804=VERTEX_POINT ( 'NONE', #722 ) ;
#40807=CARTESIAN_POINT ( 'NONE',  ( 77.36673626426795636, 49.72045831782982361, -15.49538004450117334 ) ) ;
#40810=CARTESIAN_POINT ( 'NONE',  ( 79.17960166781870157, 53.06255416066780839, 15.69067566303936445 ) ) ;
#40811=ORIENTED_EDGE ( 'NONE', *, *, #34268, .T. ) ;
#40817=CARTESIAN_POINT ( 'NONE',  ( 70.80322137413752159, 60.50400129575321273, -14.70302039727343413 ) ) ;
#40821=B_SPLINE_CURVE_WITH_KNOTS ( 'NONE', 3,
 ( #2877, #96093, #87014, #73258, #3853, #56020, #34736, #65638, #81392, #35240, #66143, #17543, #97091, #5346, #35742, #58528, #74768, #22025, #36227, #28630, #43330, #99053, #20556, #21066, #50933, #66638, #43828, #51943, #82882, #67132, #98054, #82401, #60018, #97567, #12967, #59515, #74276, #20060, #29635, #60508, #51435, #14439, #4860, #90493, #81882, #68125 ),
 .UNSPECIFIED., .F., .F.,
 ( 4, 1, 1, 1, 2, 2, 1, 1, 1, 2, 2, 1, 1, 2, 2, 1, 1, 2, 2, 1, 1, 2, 2, 1, 2, 2, 1, 2, 2, 4 ),
 ( 0.000000000000000000, 0.06249999999999522604, 0.09374999999999183986, 0.1093749999999901468, 0.1171874999999888423, 0.1249999999999875377, 0.1874999999999799050, 0.2187499999999756584, 0.2343749999999725497, 0.2421874999999724387, 0.2499999999999722999, 0.3124999999999747979, 0.3437499999999756306, 0.3593749999999750200, 0.3749999999999744649, 0.4374999999999698019, 0.4687499999999688582, 0.4843749999999679701, 0.4999999999999671374, 0.5624999999999653610, 0.5937499999999638067, 0.6093749999999638067, 0.6249999999999636957, 0.6874999999999688027, 0.7187499999999713562, 0.7499999999999740208, 0.8124999999999810152, 0.8437499999999844569, 0.8749999999999880096, 1.000000000000000000 ),
 .UNSPECIFIED. ) ;
#40823=B_SPLINE_CURVE_WITH_KNOTS ( 'NONE', 3,
 ( #68076, #75204, #36669, #84814, #67577, #15353, #98999, #38151, #29583, #30579, #7778, #60460, #91415, #90937, #38669, #69572 ),
 .UNSPECIFIED., .F., .F.,
 ( 4, 1, 2, 2, 2, 1, 2, 2, 4 ),
 ( 0.000000000000000000, 0.1249999999999976685, 0.1874999999999974742, 0.2499999999999972800, 0.4999999999999968914, 0.6249999999999961142, 0.6874999999999962252, 0.7499999999999964473, 1.000000000000000000 ),
 .UNSPECIFIED. ) ;
#40824=CARTESIAN_POINT ( 'NONE',  ( 45.79150443358504674, 28.29860640527296667, -2.839279412974138328 ) ) ;
#40826=CARTESIAN_POINT ( 'NONE',  ( 85.71994772693146558, 48.50907089644480408, -12.26219287530961743 ) ) ;
#40828=DIRECTION ( 'NONE',  ( 0.8660254037844379305, 0.5000000000000014433, 0.000000000000000000 ) ) ;
#40844=EDGE_CURVE ( 'NONE', #329, #17646, #63195, .T. ) ;
#40852=CARTESIAN_POINT ( 'NONE',  ( 77.47753981885827557, 60.62937987968794573, -15.85731085967187504 ) ) ;
#40857=CARTESIAN_POINT ( 'NONE',  ( 85.36105550139274101, 47.58428912729043958, 11.11794341640556105 ) ) ;
#40858=CARTESIAN_POINT ( 'NONE',  ( 73.81469611240122219, 68.48838210847161179, 11.42215486908102839 ) ) ;
#40860=CARTESIAN_POINT ( 'NONE',  ( 68.94813988800106586, 70.44622341501073493, 0.2739619411755226386 ) ) ;
#40868=CARTESIAN_POINT ( 'NONE',  ( 78.49761452932601458, 57.83882379195031831, 16.22345952510868727 ) ) ;
#40873=B_SPLINE_CURVE_WITH_KNOTS ( 'NONE', 3,
 ( #69433, #30933, #28955, #61816, #45131, #92768, #85178, #15723, #46626, #77554, #8142, #67435, #16235, #62313, #94770, #78552 ),
 .UNSPECIFIED., .F., .F.,
 ( 4, 1, 2, 2, 2, 1, 2, 2, 4 ),
 ( 0.000000000000000000, 0.1250000000000014155, 0.1875000000000014433, 0.2500000000000014988, 0.5000000000000001110, 0.6249999999999990008, 0.6874999999999993339, 0.7499999999999996669, 1.000000000000000000 ),
 .UNSPECIFIED. ) ;
#40875=CARTESIAN_POINT ( 'NONE',  ( 82.29791713453792568, 53.38160488945237603, -15.38503680549501418 ) ) ;
#40876=CARTESIAN_POINT ( 'NONE',  ( 74.57652347799796644, 55.50245127849832727, -16.60469772587055814 ) ) ;
#40877=CARTESIAN_POINT ( 'NONE',  ( 71.85396936473564722, 72.11868129461186072, -1.696172015788008247 ) ) ;
#40879=CARTESIAN_POINT ( 'NONE',  ( 77.05240863693448716, 63.46827552167501096, -15.45063268884610785 ) ) ;
#40882=CARTESIAN_POINT ( 'NONE',  ( 81.16557949073278166, 51.79492549539191515, -15.46120199680615670 ) ) ;
#40887=CARTESIAN_POINT ( 'NONE',  ( 30.51038259252555207, 29.56628583063842441, 9.188101187500006262 ) ) ;
#40889=CARTESIAN_POINT ( 'NONE',  ( 78.76087375241728239, 47.95963633988191077, -13.89607590865744413 ) ) ;
#40891=CARTESIAN_POINT ( 'NONE',  ( 14.21828646722447154, 29.18502408145591431, 5.678558825948277544 ) ) ;
#40903=CARTESIAN_POINT ( 'NONE',  ( 19.15050853525752927, 34.55466486950700045, 7.012934429366973338E-14 ) ) ;
#40908=CARTESIAN_POINT ( 'NONE',  ( 70.01283242295176024, 62.80173547756309915, -13.36538303052352283 ) ) ;
#40909=CARTESIAN_POINT ( 'NONE',  ( 66.92974135600969987, 68.45175875912458707, -4.590911461443917929 ) ) ;
#40919=CARTESIAN_POINT ( 'NONE',  ( 28.99364183777449000, 25.24335787977764767, -9.188101187500008038 ) ) ;
#40920=CARTESIAN_POINT ( 'NONE',  ( 74.70969265356583833, 66.80295132244255285, -13.14574923971307641 ) ) ;
#40921=CARTESIAN_POINT ( 'NONE',  ( 80.15338731764678926, 49.08938989525468344, -14.08338104835611482 ) ) ;
#40932=CARTESIAN_POINT ( 'NONE',  ( 39.74423100597210379, 28.11029122506297639, -8.090169943749478065 ) ) ;
#40941=CARTESIAN_POINT ( 'NONE',  ( 78.17513785305828833, 61.62242163703883335, -16.13566992787025356 ) ) ;
#40942=EDGE_LOOP ( 'NONE', ( #70466, #48848, #59866, #60514 ) ) ;
#40944=VERTEX_POINT ( 'NONE', #92467 ) ;
#40945=CARTESIAN_POINT ( 'NONE',  ( 80.13920462361059549, 44.63425843043530961, -11.72084457139943581 ) ) ;
#40948=CARTESIAN_POINT ( 'NONE',  ( 28.13532114344887347, 38.01751292744058475, 6.180339887498949913 ) ) ;
#40949=CARTESIAN_POINT ( 'NONE',  ( 79.60209170223603792, 48.56606275781557969, -13.98513249790191892 ) ) ;
#40957=PLANE ( 'NONE',  #19095 ) ;
#40961=CARTESIAN_POINT ( 'NONE',  ( 88.25652195435415592, 44.39905568574920380, 4.349260828767085307 ) ) ;
#40967=DIRECTION ( 'NONE',  ( -0.2938926261462390666, 0.5090369604551334692, 0.8090169943749425663 ) ) ;
#40969=ORIENTED_EDGE ( 'NONE', *, *, #90035, .F. ) ;
#40970=LINE ( 'NONE', #34400, #72099 ) ;
#40973=CARTESIAN_POINT ( 'NONE',  ( 84.87540209878125097, 43.40687427765107742, 5.588507731394742883 ) ) ;
#40975=CARTESIAN_POINT ( 'NONE',  ( 77.85177817260189670, 62.02389414260930067, 15.65016476958103198 ) ) ;
#40977=EDGE_CURVE ( 'NONE', #63364, #4682, #30540, .T. ) ;
#40981=CARTESIAN_POINT ( 'NONE',  ( 74.97115493809580755, 63.69788091252335960, -14.47858387620434506 ) ) ;
#40983=CARTESIAN_POINT ( 'NONE',  ( 69.73423326249884724, 62.23649111975013426, -13.60044372541333857 ) ) ;
#40984=CARTESIAN_POINT ( 'NONE',  ( 24.50477583610994259, 37.08080186712593473, -3.090169943749475845 ) ) ;
#40986=ADVANCED_FACE ( 'NONE', ( #32957 ), #10177, .T. ) ;
#40990=CARTESIAN_POINT ( 'NONE',  ( 71.94636440693795976, 59.33070143154711928, -15.31651758414362696 ) ) ;
#41001=CARTESIAN_POINT ( 'NONE',  ( 81.89611374139302313, 41.17756255496580309, 5.592514320812338013 ) ) ;
#41005=CARTESIAN_POINT ( 'NONE',  ( 39.65533143765975410, 23.86426979415092475, -3.090169943749474069 ) ) ;
#41009=CARTESIAN_POINT ( 'NONE',  ( 81.03611213647164391, 56.10389352724613587, 16.10741472980589961 ) ) ;
#41010=CARTESIAN_POINT ( 'NONE',  ( 15.23341505093859816, 9.764269794150882475, 3.090169943749476733 ) ) ;
#41016=EDGE_CURVE ( 'NONE', #86729, #61384, #17256, .T. ) ;
#41018=CARTESIAN_POINT ( 'NONE',  ( 69.68416697561647766, 66.78355214756700775, -10.04849009066424870 ) ) ;
#41025=DIRECTION ( 'NONE',  ( -0.5000000000000015543, 0.8660254037844377084, 0.000000000000000000 ) ) ;
#41027=VERTEX_POINT ( 'NONE', #73476 ) ;
#41028=CARTESIAN_POINT ( 'NONE',  ( 66.36268096397610350, 69.44190093015801324, 9.875986171954755521E-07 ) ) ;
#41030=LINE ( 'NONE', #71967, #54161 ) ;
#41032=CARTESIAN_POINT ( 'NONE',  ( 20.27385872851041526, 33.74646525600390135, 2.839279412974139660 ) ) ;
#41036=EDGE_LOOP ( 'NONE', ( #87759, #22227, #48403, #83767 ) ) ;
#41037=CARTESIAN_POINT ( 'NONE',  ( 15.30080465516770616, 11.76004757982088300, 5.678558825948272215 ) ) ;
#41045=CYLINDRICAL_SURFACE ( 'NONE', #85746, 10.00000000000001066 ) ;
#41046=CARTESIAN_POINT ( 'NONE',  ( 73.83222695958433235, 64.41044440392025194, -14.27322267731098648 ) ) ;
#41054=CARTESIAN_POINT ( 'NONE',  ( 73.00396795751623813, 57.62093675937267534, -16.32480838639074960 ) ) ;
#41055=CARTESIAN_POINT ( 'NONE',  ( 77.03033377257250436, 63.66679109869721742, 15.37730549896620147 ) ) ;
#41060=ORIENTED_EDGE ( 'NONE', *, *, #905, .T. ) ;
#41063=CARTESIAN_POINT ( 'NONE',  ( 25.47001115121704373, 36.74646525600391556, 2.839279412974139660 ) ) ;
#41065=CARTESIAN_POINT ( 'NONE',  ( 78.21696194461939911, 47.89139066307899384, -14.01588872958974363 ) ) ;
#41067=CARTESIAN_POINT ( 'NONE',  ( 74.41176536287696308, 68.30213538679808494, 11.88880159922068636 ) ) ;
#41072=VECTOR ( 'NONE', #831, 1000.000000000000114 ) ;
#41073=LINE ( 'NONE', #96838, #48009 ) ;
#41074=CARTESIAN_POINT ( 'NONE',  ( 83.51844524235421829, 42.82187930146461952, -5.925958474313000046 ) ) ;
#41079=CARTESIAN_POINT ( 'NONE',  ( 68.00902249195229388, 69.32663607418423624, -3.845441495452403657 ) ) ;
#41082=CARTESIAN_POINT ( 'NONE',  ( 82.56232498766836159, 52.00393866007731702, -15.24789231007047619 ) ) ;
#41083=VECTOR ( 'NONE', #31581, 1000.000000000000114 ) ;
#41085=CARTESIAN_POINT ( 'NONE',  ( 68.55513178119723250, 64.39780669069259034, 11.67030924314737206 ) ) ;
#41088=CARTESIAN_POINT ( 'NONE',  ( 76.13230372035420146, 65.40393639426625327, 14.02425539466697479 ) ) ;
#41090=CARTESIAN_POINT ( 'NONE',  ( 19.15050853525752927, 34.55466486950700045, 7.012934429366973338E-14 ) ) ;
#41092=VERTEX_POINT ( 'NONE', #66851 ) ;
#41093=CARTESIAN_POINT ( 'NONE',  ( 85.28185142231448879, 44.17485613502010011, -6.750586009585262559 ) ) ;
#41098=CARTESIAN_POINT ( 'NONE',  ( 83.85460425676879481, 51.57915136420024282, -14.37880942938260098 ) ) ;
#41099=DIRECTION ( 'NONE',  ( 0.2925570654631259870, 0.000000000000000000, -0.9562480658530003730 ) ) ;
#41101=CARTESIAN_POINT ( 'NONE',  ( 80.29069729260778843, 58.15026982914754683, -16.60659103188077879 ) ) ;
#41103=CARTESIAN_POINT ( 'NONE',  ( 72.42095758685501039, 70.73706075180957953, 7.727740079816332042 ) ) ;
#41115=CARTESIAN_POINT ( 'NONE',  ( 70.80369121223017714, 70.91613982041616282, -4.241969676397446598 ) ) ;
#41123=CARTESIAN_POINT ( 'NONE',  ( 20.52402715336229377, 23.80066082961421969, 10.00000000000000533 ) ) ;
#41128=CARTESIAN_POINT ( 'NONE',  ( 25.79892497710874366, 15.86426979415090166, -3.090169943749474069 ) ) ;
#41130=CARTESIAN_POINT ( 'NONE',  ( 75.99750771566300500, 65.44421971917601866, -13.95497799904430458 ) ) ;
#41132=CARTESIAN_POINT ( 'NONE',  ( 73.88993811345744689, 55.02826134877724940, -16.60322266602316077 ) ) ;
#41134=CARTESIAN_POINT ( 'NONE',  ( 2.749951498565457175, 23.36126292948892313, 6.180339887498949913 ) ) ;
#41139=CARTESIAN_POINT ( 'NONE',  ( 71.76351473723394747, 71.84897031608997509, 2.971691788643012977 ) ) ;
#41146=CARTESIAN_POINT ( 'NONE',  ( 31.53879454291322659, 39.18502408145594984, 5.678558825948277544 ) ) ;
#41150=CARTESIAN_POINT ( 'NONE',  ( 28.62558104116610380, 25.03085787977764198, 9.188101187500006262 ) ) ;
#41158=CARTESIAN_POINT ( 'NONE',  ( 12.71236424662705566, 15.84335787977761534, 9.188101187500006262 ) ) ;
#41160=CARTESIAN_POINT ( 'NONE',  ( 15.51250667149479590, 27.14336893147754992, 7.433330006724141015 ) ) ;
#41169=CARTESIAN_POINT ( 'NONE',  ( 66.05904967884808343, 68.59175798592418971, 4.366901512547229025 ) ) ;
#41170=CARTESIAN_POINT ( 'NONE',  ( 87.24455917599382815, 45.43202867884257046, 7.120756001641662003 ) ) ;
#41176=CARTESIAN_POINT ( 'NONE',  ( 86.10128179547638183, 47.01522930412662760, 10.71950609365847917 ) ) ;
#41178=CARTESIAN_POINT ( 'NONE',  ( 77.79862349870425930, 57.75687281312781352, 16.17549868577739147 ) ) ;
#41183=CARTESIAN_POINT ( 'NONE',  ( 80.72039647166839416, 43.16609979737107494, 9.908769291271109836 ) ) ;
#41191=CARTESIAN_POINT ( 'NONE',  ( 33.00691499580853616, 42.55466486950702887, 7.012934429366973338E-14 ) ) ;
#41194=DIRECTION ( 'NONE',  ( -0.2347357813929480952, 0.4065742997269687908, 0.8829475928589233247 ) ) ;
#41201=CARTESIAN_POINT ( 'NONE',  ( 71.22758957664390778, 69.00678633681690144, 8.474304139278888925 ) ) ;
#41204=FACE_OUTER_BOUND ( 'NONE', #9980, .T. ) ;
#41207=CARTESIAN_POINT ( 'NONE',  ( 17.35762855594305520, 30.99752408145591431, 5.678558825948277544 ) ) ;
#41220=CARTESIAN_POINT ( 'NONE',  ( 71.40048854769935360, 59.28136089601005665, 15.74267823446789905 ) ) ;
#41221=ORIENTED_EDGE ( 'NONE', *, *, #27516, .F. ) ;
#41222=FACE_OUTER_BOUND ( 'NONE', #6913, .T. ) ;
#41224=FACE_OUTER_BOUND ( 'NONE', #98649, .T. ) ;
#41229=EDGE_CURVE ( 'NONE', #82089, #55525, #64272, .T. ) ;
#41230=CARTESIAN_POINT ( 'NONE',  ( 82.62228925795274392, 40.54765601476822923, -1.426017262080774728 ) ) ;
#41231=LINE ( 'NONE', #48355, #43717 ) ;
#41240=CARTESIAN_POINT ( 'NONE',  ( 68.88891825534665259, 70.31481240275726918, 1.479671699557132847 ) ) ;
#41242=CARTESIAN_POINT ( 'NONE',  ( 84.41257289432805067, 44.20851797303996733, 7.649024224649666692 ) ) ;
#41246=CARTESIAN_POINT ( 'NONE',  ( 74.32663207346742240, 67.92009797516583092, -11.69620558213257233 ) ) ;
#41250=CARTESIAN_POINT ( 'NONE',  ( 79.32566820500107951, 59.73991648520959075, -16.51753030644415077 ) ) ;
#41252=B_SPLINE_CURVE_WITH_KNOTS ( 'NONE', 3,
 ( #35262, #41865, #27683, #90003, #3396, #34271, #81906, #12485, #43351, #74299, #96117, #66660, #28162, #68645, #29170, #53438, #16817, #76749, #5369, #51964, #44842, #21088, #74791, #28654, #82905, #67656, #37735, #21566, #22553, #98076, #67155, #44348, #62918, #29656, #32008, #13477, #61033, #36748, #14935, #37249, #76275, #99565, #83899, #5863, #36252, #6849 ),
 .UNSPECIFIED., .F., .F.,
 ( 4, 1, 1, 1, 2, 2, 1, 1, 1, 2, 2, 1, 1, 2, 2, 1, 1, 2, 2, 1, 1, 2, 2, 1, 2, 2, 1, 2, 2, 4 ),
 ( 0.000000000000000000, 0.06249999999999693301, 0.09374999999999547584, 0.1093749999999947542, 0.1171874999999927003, 0.1249999999999906325, 0.1874999999999749922, 0.2187499999999669986, 0.2343749999999645284, 0.2421874999999631406, 0.2499999999999617528, 0.3124999999999574785, 0.3437499999999567013, 0.3593749999999563682, 0.3749999999999560907, 0.4374999999999543143, 0.4687499999999536482, 0.4843749999999518718, 0.4999999999999500955, 0.5624999999999510392, 0.5937499999999500400, 0.6093749999999494849, 0.6249999999999489297, 0.6874999999999561462, 0.7187499999999611422, 0.7499999999999661382, 0.8124999999999761302, 0.8437499999999811262, 0.8749999999999861222, 1.000000000000000000 ),
 .UNSPECIFIED. ) ;
#41254=CARTESIAN_POINT ( 'NONE',  ( 72.76446422349044951, 71.15534465558162935, -7.354170587574372142 ) ) ;
#41267=CARTESIAN_POINT ( 'NONE',  ( 13.49720994389718598, 29.83396525600389637, -2.839279412974133887 ) ) ;
#41268=CARTESIAN_POINT ( 'NONE',  ( 74.96142304803882439, 67.14338225477067112, 13.01358479607535479 ) ) ;
#41279=CARTESIAN_POINT ( 'NONE',  ( 81.50893757138975104, 55.16156497580061568, -15.92217606427533205 ) ) ;
#41281=CARTESIAN_POINT ( 'NONE',  ( 71.03936537156745601, 65.74473520561056716, -12.39895433411619763 ) ) ;
#41285=CARTESIAN_POINT ( 'NONE',  ( 80.40498937112451472, 56.16844747207684208, 16.11541614916188792 ) ) ;
#41288=CARTESIAN_POINT ( 'NONE',  ( 72.25718139279801733, 71.61371966692031776, -5.855127513239330561 ) ) ;
#41293=B_SPLINE_SURFACE_WITH_KNOTS ( 'NONE', 3, 1, ( 
 ( #15185, #39475 ),
 ( #85147, #53687 ),
 ( #78523, #8116 ),
 ( #39982, #70917 ),
 ( #84644, #1011 ),
 ( #69406, #30904 ),
 ( #86663, #31889 ),
 ( #62795, #93751 ),
 ( #46085, #15693 ),
 ( #24310, #77525 ),
 ( #37983, #23796 ),
 ( #31396, #32404 ),
 ( #23292, #63301 ),
 ( #62283, #76996 ),
 ( #94243, #61792 ),
 ( #24795, #93237 ),
 ( #92738, #76520 ),
 ( #54681, #55186 ),
 ( #55676, #68894 ),
 ( #30405, #61297 ),
 ( #3526, #71420 ),
 ( #56186, #57188 ),
 ( #40490, #25299 ),
 ( #32896, #34889 ),
 ( #41489, #87180 ),
 ( #4003, #9629 ),
 ( #11621, #50103 ),
 ( #81058, #10613 ),
 ( #65303, #72434 ),
 ( #2010, #3038 ),
 ( #88167, #18715 ) ),
 .UNSPECIFIED., .F., .F., .F.,
 ( 4, 3, 3, 3, 3, 3, 3, 3, 3, 3, 4 ),
 ( 2, 2 ),
 ( 0.000000000000000000, 0.1333490885032338480, 0.3007194338854361493, 0.4699862290245140906, 0.5844252810809331677, 0.6686540514502653521, 0.7354980260655413771, 0.8028463152565569194, 0.8633854507757173780, 0.9437142632667304687, 1.000000000000000000 ),
 ( 0.000000000000000000, 1.000000000000000000 ),
 .UNSPECIFIED. ) ;
#41294=CARTESIAN_POINT ( 'NONE',  ( 2.749951498565457175, 23.36126292948892313, 6.180339887498949913 ) ) ;
#41297=CARTESIAN_POINT ( 'NONE',  ( 77.90166149968712261, 61.78270738046986565, 16.06607043079731412 ) ) ;
#41300=CARTESIAN_POINT ( 'NONE',  ( 78.85260902839583252, 60.08087593534391857, 16.11113849416598853 ) ) ;
#41302=CARTESIAN_POINT ( 'NONE',  ( 88.26279489949382651, 43.89118386701247942, -2.126167786569203244 ) ) ;
#41303=LINE ( 'NONE', #80367, #68834 ) ;
#41304=CARTESIAN_POINT ( 'NONE',  ( 81.48361531348861320, 50.88580826621501529, -14.60796985947813731 ) ) ;
#41305=CARTESIAN_POINT ( 'NONE',  ( 80.32637618523892797, 44.90515637106070557, 11.18374640163626843 ) ) ;
#41306=CARTESIAN_POINT ( 'NONE',  ( 84.65937204597994992, 49.81022611792842270, -13.17500266760843353 ) ) ;
#41310=B_SPLINE_CURVE_WITH_KNOTS ( 'NONE', 3,
 ( #10462, #34744, #27165, #11967, #4869, #97101, #41338, #42827, #73761, #27668, #65152, #81891, #3383, #58536, #34255, #12468, #96099, #35749, #57540, #66646, #97576, #28147, #95614, #33780 ),
 .UNSPECIFIED., .F., .F.,
 ( 4, 2, 2, 2, 2, 2, 2, 2, 2, 2, 2, 4 ),
 ( 0.000000000000000000, 0.1249999999999845401, 0.2499999999999690803, 0.3749999999999535927, 0.4374999999999542588, 0.4999999999999549249, 0.5624999999999555911, 0.6249999999999563682, 0.6874999999999570344, 0.7499999999999577005, 0.8749999999999787947, 1.000000000000000000 ),
 .UNSPECIFIED. ) ;
#41315=CARTESIAN_POINT ( 'NONE',  ( 74.60301285042477559, 56.94764521179947536, 16.05680618570769624 ) ) ;
#41317=VERTEX_POINT ( 'NONE', #67835 ) ;
#41318=CARTESIAN_POINT ( 'NONE',  ( 82.21903993916642150, 41.17462734708961847, 3.239289935595443648 ) ) ;
#41324=DIRECTION ( 'NONE',  ( -0.8660254037844379305, -0.5000000000000014433, -0.000000000000000000 ) ) ;
#41331=CARTESIAN_POINT ( 'NONE',  ( 40.03666203415436797, 35.06628583063844928, -9.188101187500006262 ) ) ;
#41334=CARTESIAN_POINT ( 'NONE',  ( 31.15319227796116053, 18.39040679176984128, -6.890680421881970419E-14 ) ) ;
#41338=CARTESIAN_POINT ( 'NONE',  ( 76.24760352746896785, 65.19682467712520690, -14.16189420828948542 ) ) ;
#41361=CARTESIAN_POINT ( 'NONE',  ( 72.57128799697304089, 62.22197114735462975, -14.43632866411172344 ) ) ;
#41365=VECTOR ( 'NONE', #47019, 1000.000000000000114 ) ;
#41368=CARTESIAN_POINT ( 'NONE',  ( 80.80800637050489854, 42.99464212843047051, -9.644767597250195834 ) ) ;
#41369=CARTESIAN_POINT ( 'NONE',  ( 67.04009420809389042, 68.98588012621723919, 2.960418080124604945 ) ) ;
#41371=EDGE_CURVE ( 'NONE', #16493, #41560, #56894, .T. ) ;
#41374=CARTESIAN_POINT ( 'NONE',  ( 88.09111776262265892, 44.56188567158400815, -5.102872454969324068 ) ) ;
#41378=CARTESIAN_POINT ( 'NONE',  ( 74.45626529801648985, 55.41543688963572833, -16.12783148945726452 ) ) ;
#41385=CARTESIAN_POINT ( 'NONE',  ( 76.83221134703946120, 55.52632626272433924, -16.15978416529669914 ) ) ;
#41390=CARTESIAN_POINT ( 'NONE',  ( 77.02134436793002692, 63.41470467299149760, -15.46275534251473438 ) ) ;
#41393=CARTESIAN_POINT ( 'NONE',  ( 75.31289280905393468, 53.62176160565092431, -16.53289957284814093 ) ) ;
#41394=CARTESIAN_POINT ( 'NONE',  ( 81.51649937534789103, 59.53360007009536048, -0.2191855733945438922 ) ) ;
#41398=CARTESIAN_POINT ( 'NONE',  ( 32.83301474718356161, 37.14336893147758900, 7.433330006724141015 ) ) ;
#41399=CARTESIAN_POINT ( 'NONE',  ( 82.60066728560789784, 50.87129046802179033, 14.76979220338051491 ) ) ;
#41402=CARTESIAN_POINT ( 'NONE',  ( 20.18540868186541459, 12.44966523072493914, -2.296566073217252530E-15 ) ) ;
#41411=CARTESIAN_POINT ( 'NONE',  ( 72.56680254073344827, 71.38637538794351656, 5.777867564336608197 ) ) ;
#41414=CARTESIAN_POINT ( 'NONE',  ( 19.30862341340331412, 34.08080186712593473, -3.090169943749475845 ) ) ;
#41422=CARTESIAN_POINT ( 'NONE',  ( 77.10594840515625492, 62.91113679231831668, -15.28126102291101063 ) ) ;
#41423=EDGE_LOOP ( 'NONE', ( #72151, #33748, #93859, #91188 ) ) ;
#41426=CARTESIAN_POINT ( 'NONE',  ( 81.93977088949127108, 44.53106330606377838, 10.63662565672798443 ) ) ;
#41428=ORIENTED_EDGE ( 'NONE', *, *, #95099, .T. ) ;
#41429=CARTESIAN_POINT ( 'NONE',  ( 46.74164954608104949, 27.39040679176987325, -6.890680421881970419E-14 ) ) ;
#41430=CARTESIAN_POINT ( 'NONE',  ( 35.44910642356613550, 21.26216523072496400, -2.296566073217252530E-15 ) ) ;
#41432=CARTESIAN_POINT ( 'NONE',  ( 80.17887552957238029, 44.29837527985885970, 11.40047595680318970 ) ) ;
#41435=CARTESIAN_POINT ( 'NONE',  ( 82.65473243480592203, 40.50376448046697675, -0.5611958088008396350 ) ) ;
#41442=CARTESIAN_POINT ( 'NONE',  ( 85.59269861019149062, 48.32250421001948126, -11.70547994120720325 ) ) ;
#41448=CARTESIAN_POINT ( 'NONE',  ( 79.45469543192598394, 59.63697030301000979, 16.53293242656296869 ) ) ;
#41455=CARTESIAN_POINT ( 'NONE',  ( 80.30560875578385094, 44.94112661401950248, -11.22675700711674374 ) ) ;
#41458=CARTESIAN_POINT ( 'NONE',  ( 68.25940382258694683, 65.54188025616944913, 10.45666766922404101 ) ) ;
#41467=CARTESIAN_POINT ( 'NONE',  ( 75.93815686453476133, 64.70849926024720844, -14.31753493372995933 ) ) ;
#41469=CARTESIAN_POINT ( 'NONE',  ( 87.48880955142448101, 44.86412769470708639, -6.596395727433105094 ) ) ;
#41471=CARTESIAN_POINT ( 'NONE',  ( 87.76435223195018409, 44.22492802364795494, 4.686297260842065882 ) ) ;
#41487=CARTESIAN_POINT ( 'NONE',  ( 84.80509911768557174, 43.31890675800398327, 5.469368207548569671 ) ) ;
#41489=CARTESIAN_POINT ( 'NONE',  ( 83.43050110256683638, 51.89332412091456348, 15.00139857044202074 ) ) ;
#41497=CARTESIAN_POINT ( 'NONE',  ( 75.42132300406277068, 63.53713694569018600, -14.66775701755491745 ) ) ;
#41499=CARTESIAN_POINT ( 'NONE',  ( 74.32283972738726163, 55.33658384528776963, 16.60204640396233344 ) ) ;
#41500=CARTESIAN_POINT ( 'NONE',  ( 69.66767063274500060, 62.28281038103965273, -13.55241073290247478 ) ) ;
#41501=CARTESIAN_POINT ( 'NONE',  ( 28.73071361209859731, 38.36126292948897287, 6.180339887498949913 ) ) ;
#41509=CARTESIAN_POINT ( 'NONE',  ( 81.12568207579826662, 44.96798002130291394, 10.84245638387497657 ) ) ;
#41511=CARTESIAN_POINT ( 'NONE',  ( 87.37270799788964837, 45.80620788475513905, 8.330021955613661433 ) ) ;
#41513=CARTESIAN_POINT ( 'NONE',  ( 71.86256228778262312, 72.60615528678948749, -0.5650332253008816252 ) ) ;
#41517=CARTESIAN_POINT ( 'NONE',  ( 40.07075743699687109, 22.94473085651394939, 1.475505719884397138E-15 ) ) ;
#41525=CARTESIAN_POINT ( 'NONE',  ( 83.73865579866679809, 51.98612588642360777, 14.96617132975018372 ) ) ;
#41535=CARTESIAN_POINT ( 'NONE',  ( 67.42404893004047040, 67.25264271294523155, -8.643519966047881198 ) ) ;
#41541=CARTESIAN_POINT ( 'NONE',  ( 31.61033844661487180, 20.11110640527293825, -2.839279412974138328 ) ) ;
#41547=CARTESIAN_POINT ( 'NONE',  ( 16.25825050073692069, 15.10170272979925876, -7.433330006724141015 ) ) ;
#41551=CARTESIAN_POINT ( 'NONE',  ( 72.03955433498997252, 71.50824183410490775, -5.808600603169774779 ) ) ;
#41552=CARTESIAN_POINT ( 'NONE',  ( 82.42797444979642307, 40.90780339933488818, -0.3678846455753223554 ) ) ;
#41560=VERTEX_POINT ( 'NONE', #49519 ) ;
#41562=CARTESIAN_POINT ( 'NONE',  ( 72.02714983513547509, 72.27104924840581646, -3.542005090554713576 ) ) ;
#41563=CARTESIAN_POINT ( 'NONE',  ( 70.92012640611527274, 71.65591018854625815, -3.452294570978728050 ) ) ;
#41564=CARTESIAN_POINT ( 'NONE',  ( 77.96869982513443631, 61.39881034122267778, -16.15742658069109439 ) ) ;
#41575=CARTESIAN_POINT ( 'NONE',  ( 30.66616357392367220, 39.74646525600392977, 2.839279412974139660 ) ) ;
#41577=CARTESIAN_POINT ( 'NONE',  ( 78.46624349761390249, 48.01460221765250225, -14.00587743556854115 ) ) ;
#41579=CARTESIAN_POINT ( 'NONE',  ( 73.85129109314340212, 68.53037146055885387, 10.90305250113367741 ) ) ;
#41583=VERTEX_POINT ( 'NONE', #52504 ) ;
#41584=( BOUNDED_CURVE ( )  B_SPLINE_CURVE ( 2, ( #85878, #25510, #79755, #17924, #16404, #31588, #1729, #93950, #78723, #55383, #48822, #93447, #9312 ),
 .UNSPECIFIED., .F., .T. ) 
 B_SPLINE_CURVE_WITH_KNOTS ( ( 3, 2, 2, 2, 2, 2, 3 ),
 ( 0.8125000000000000000, 0.8149999999999999467, 0.8199999999999999512, 0.8249999999999999556, 0.8299999999999999600, 0.8349999999999999645, 0.8375000000000000222 ),
 .UNSPECIFIED. ) 
 CURVE ( )  GEOMETRIC_REPRESENTATION_ITEM ( )  RATIONAL_B_SPLINE_CURVE ( ( 0.9755282581475768211, 0.9755282581475768211, 1.000000000000000000, 0.9510565162951535312, 1.000000000000000000, 0.9510565162951535312, 1.000000000000000000, 0.9510565162951535312, 1.000000000000000000, 0.9510565162951535312, 1.000000000000000000, 0.9755282581475761550, 0.9755282581475767101 ) ) 
 REPRESENTATION_ITEM ( '' )  );
#41589=CARTESIAN_POINT ( 'NONE',  ( 69.76281041485397338, 69.71141683662550292, -5.692271621175008178 ) ) ;
#41591=CARTESIAN_POINT ( 'NONE',  ( 81.47742755412382110, 52.42827155326802568, -15.60484105884143169 ) ) ;
#41600=CARTESIAN_POINT ( 'NONE',  ( 86.35622788611077283, 44.22730618112566248, -5.622056245697837795 ) ) ;
#41601=CARTESIAN_POINT ( 'NONE',  ( 83.60889825226890082, 41.79735538044917575, 2.466802602430361091 ) ) ;
#41605=CARTESIAN_POINT ( 'NONE',  ( 73.99318389990696687, 57.32182924785170286, 15.98609978358631700 ) ) ;
#41608=CARTESIAN_POINT ( 'NONE',  ( 80.44596413951620661, 57.92004253751065335, -16.60216415864725903 ) ) ;
#41609=CARTESIAN_POINT ( 'NONE',  ( 71.81466828470752262, 72.18675276203495628, 0.5721087574936188913 ) ) ;
#41615=CARTESIAN_POINT ( 'NONE',  ( 68.00690384560408575, 68.82080238078589218, 5.313225612992173552 ) ) ;
#41618=VECTOR ( 'NONE', #48530, 1000.000000000000114 ) ;
#41620=B_SPLINE_SURFACE_WITH_KNOTS ( 'NONE', 3, 1, ( 
 ( #33202, #1313 ),
 ( #3331, #32196 ),
 ( #18021, #1814 ),
 ( #72226, #55974 ),
 ( #86466, #78823 ),
 ( #25613, #65102 ),
 ( #94539, #48407 ),
 ( #79848, #2832 ),
 ( #95567, #26610 ),
 ( #56989, #10919 ),
 ( #57485, #97523 ),
 ( #12415, #44282 ),
 ( #58965, #42776 ),
 ( #49902, #67085 ),
 ( #88979, #59468 ),
 ( #67586, #90450 ),
 ( #35192, #4292 ),
 ( #66100, #21019 ),
 ( #82842, #80860 ),
 ( #42286, #96543 ),
 ( #58482, #20013 ),
 ( #59973, #6790 ),
 ( #53862, #39154 ),
 ( #22487, #7279 ),
 ( #31071, #77705 ),
 ( #15873, #92425 ),
 ( #8289, #45280 ),
 ( #70069, #83329 ),
 ( #30087, #13892 ),
 ( #75708, #6294 ),
 ( #68086, #99008 ) ),
 .UNSPECIFIED., .F., .F., .F.,
 ( 4, 3, 3, 3, 3, 3, 3, 3, 3, 3, 4 ),
 ( 2, 2 ),
 ( 0.000000000000000000, 0.1333490885032311002, 0.3007194338854346505, 0.4699862290245186980, 0.5844252810809363874, 0.6686540514502655741, 0.7354980260655468172, 0.8028463152565521455, 0.8633854507757170449, 0.9437142632667351316, 1.000000000000000000 ),
 ( 0.000000000000000000, 1.000000000000000000 ),
 .UNSPECIFIED. ) ;
#41621=CARTESIAN_POINT ( 'NONE',  ( 19.36651902841724038, 19.38052372038640669, 10.00000000000000533 ) ) ;
#41629=CARTESIAN_POINT ( 'NONE',  ( 82.33779659592744338, 51.32762991731738822, -14.58766645682115026 ) ) ;
#41635=CARTESIAN_POINT ( 'NONE',  ( 18.62433137644124059, 29.49103043416549141, -8.090169943749479842 ) ) ;
#41638=CARTESIAN_POINT ( 'NONE',  ( 65.99211009093512814, 69.22537564306347235, 0.2727399908702655695 ) ) ;
#41639=CARTESIAN_POINT ( 'NONE',  ( 72.09683433654826956, 72.38845567423071259, -3.220643376046866901 ) ) ;
#41641=CARTESIAN_POINT ( 'NONE',  ( 73.92553126217202930, 55.61088272459142701, -16.58549581058217015 ) ) ;
#41654=CARTESIAN_POINT ( 'NONE',  ( 32.92443518896833154, 39.98502408145596121, -5.678558825948271327 ) ) ;
#41657=CARTESIAN_POINT ( 'NONE',  ( 37.13125039574066477, 23.29860640527294535, -2.839279412974138328 ) ) ;
#41662=CARTESIAN_POINT ( 'NONE',  ( 11.83670304002995266, 9.760047579820874120, 5.678558825948272215 ) ) ;
#41664=CARTESIAN_POINT ( 'NONE',  ( 20.04711164229383513, 17.28920272979926764, -7.433330006724141015 ) ) ;
#41668=CARTESIAN_POINT ( 'NONE',  ( 21.58410742392950610, 28.16454794089041869, -10.00000000000000355 ) ) ;
#41669=CARTESIAN_POINT ( 'NONE',  ( 88.17689713045484723, 44.18699809719895910, -1.761924701106883040 ) ) ;
#41670=EDGE_CURVE ( 'NONE', #97296, #85165, #69103, .T. ) ;
#41674=CARTESIAN_POINT ( 'NONE',  ( 66.04680300344115551, 68.56179634104172749, 4.439170754574295330 ) ) ;
#41677=ORIENTED_EDGE ( 'NONE', *, *, #69608, .F. ) ;
#41679=CARTESIAN_POINT ( 'NONE',  ( 86.10659305072458380, 47.03284479452093336, 10.73441527774546245 ) ) ;
#41686=CARTESIAN_POINT ( 'NONE',  ( 78.24512733555256716, 61.71755924530574333, -15.76113161412312813 ) ) ;
#41687=CARTESIAN_POINT ( 'NONE',  ( 88.54102397196729157, 43.89880672352619229, -0.3772737106920456829 ) ) ;
#41690=CARTESIAN_POINT ( 'NONE',  ( 80.74112568426333780, 43.09697088413143007, 9.813618375449099318 ) ) ;
#41695=CARTESIAN_POINT ( 'NONE',  ( 74.28011090699931174, 62.22829491240943867, 14.85767347728069154 ) ) ;
#41702=ORIENTED_EDGE ( 'NONE', *, *, #80172, .F. ) ;
#41707=ORIENTED_EDGE ( 'NONE', *, *, #45585, .T. ) ;
#41715=CARTESIAN_POINT ( 'NONE',  ( 23.18645373101242413, 19.10170272979927120, -7.433330006724141015 ) ) ;
#41726=CARTESIAN_POINT ( 'NONE',  ( 79.10094814821772502, 46.07821729000689714, 13.26225723241342003 ) ) ;
#41738=EDGE_CURVE ( 'NONE', #45167, #54308, #63006, .T. ) ;
#41749=CARTESIAN_POINT ( 'NONE',  ( 83.29197815752417000, 42.60964419094407418, 5.769052513407811666 ) ) ;
#41753=CARTESIAN_POINT ( 'NONE',  ( 74.20550489482296541, 67.87148625235720090, -11.67750707853813807 ) ) ;
#41758=CARTESIAN_POINT ( 'NONE',  ( 84.11025865604790397, 47.61814693595540149, 11.74156198426350706 ) ) ;
#41763=CARTESIAN_POINT ( 'NONE',  ( 68.91072503222051182, 64.29678190498039214, -11.91033057008465157 ) ) ;
#41765=CARTESIAN_POINT ( 'NONE',  ( 79.13689845121717781, 45.88162669096313806, -12.51413720753079772 ) ) ;
#41772=VECTOR ( 'NONE', #63212, 1000.000000000000114 ) ;
#41776=CARTESIAN_POINT ( 'NONE',  ( 26.73894555032740783, 17.29860640527292759, -2.839279412974138328 ) ) ;
#41777=CARTESIAN_POINT ( 'NONE',  ( 74.99774251554812565, 67.18734242688375957, 12.55770300872047507 ) ) ;
#41782=CARTESIAN_POINT ( 'NONE',  ( 12.54686387532899516, 29.01751292744055277, 6.180339887498949913 ) ) ;
#41788=CARTESIAN_POINT ( 'NONE',  ( 81.56133095906432118, 55.49845989692713744, -16.32137983002412085 ) ) ;
#41790=CARTESIAN_POINT ( 'NONE',  ( 76.77731254116882553, 64.09355814141257213, -15.16545583891343263 ) ) ;
#41793=CARTESIAN_POINT ( 'NONE',  ( 79.50884248659365028, 51.35306852090381824, 15.14975241329744193 ) ) ;
#41794=CARTESIAN_POINT ( 'NONE',  ( 83.77581334972808236, 52.13813006813991535, -14.62973826141883826 ) ) ;
#41795=CARTESIAN_POINT ( 'NONE',  ( 71.40824431555127205, 71.90448883543326986, -1.148190763236565326 ) ) ;
#41800=CARTESIAN_POINT ( 'NONE',  ( 3.893371226040319044, 25.18080186712590773, 3.090169943749475401 ) ) ;
#41806=ORIENTED_EDGE ( 'NONE', *, *, #45815, .F. ) ;
#41808=CARTESIAN_POINT ( 'NONE',  ( 79.09523395582193928, 59.82262253747457237, 16.49691284064748587 ) ) ;
#41810=AXIS2_PLACEMENT_3D ( 'NONE', #4635, #25956, #3170 ) ;
#41811=CARTESIAN_POINT ( 'NONE',  ( 83.55471316296232942, 50.16249053343400277, -13.72935981377203163 ) ) ;
#41812=CARTESIAN_POINT ( 'NONE',  ( 73.43716180859617282, 69.78348016549323063, -9.856747356917667346 ) ) ;
#41821=DIRECTION ( 'NONE',  ( -0.3715724127386920705, 0.6435822975543701308, -0.6691306063588670083 ) ) ;
#41827=CARTESIAN_POINT ( 'NONE',  ( 82.06339014627782547, 41.09835319584696123, 3.298898961656697715 ) ) ;
#41838=CARTESIAN_POINT ( 'NONE',  ( 70.97253302420340049, 61.11785764705713575, -14.48731777010960009 ) ) ;
#41842=CARTESIAN_POINT ( 'NONE',  ( 85.65277752055500571, 48.41186657597218357, -12.21575983946769739 ) ) ;
#41857=CARTESIAN_POINT ( 'NONE',  ( 75.91930487633969449, 61.92743185228299296, -15.32863521163103648 ) ) ;
#41861=B_SPLINE_CURVE_WITH_KNOTS ( 'NONE', 3,
 ( #44590, #61296, #59799, #60778, #30903, #6110, #67408, #53207, #69405, #38490, #52693, #37491, #76995, #37982, #7602, #29416, #83147, #51730, #21808, #18, #67915, #83655, #84160, #92259, #14706, #90265, #20838, #14213, #68399, #82673, #68893, #13238, #60285, #13715, #44092, #45105, #75036, #98835, #15184, #99820, #36505, #28927, #37005, #98333, #75525, #90770 ),
 .UNSPECIFIED., .F., .F.,
 ( 4, 1, 1, 1, 2, 2, 1, 1, 1, 2, 2, 1, 1, 2, 2, 1, 1, 2, 2, 1, 1, 2, 2, 1, 2, 2, 1, 2, 2, 4 ),
 ( 0.000000000000000000, 0.06249999999997910005, 0.09374999999997009337, 0.1093749999999655831, 0.1171874999999646949, 0.1249999999999638067, 0.1874999999999651112, 0.2187499999999650835, 0.2343749999999650835, 0.2421874999999658884, 0.2499999999999666933, 0.3124999999999751865, 0.3437499999999794609, 0.3593749999999806266, 0.3749999999999817368, 0.4374999999999826250, 0.4687499999999830136, 0.4843749999999821809, 0.4999999999999813483, 0.5624999999999810152, 0.5937499999999817923, 0.6093749999999825695, 0.6249999999999832356, 0.6874999999999895639, 0.7187499999999926725, 0.7499999999999957812, 0.8124999999999994449, 0.8437500000000004441, 0.8750000000000013323, 1.000000000000000000 ),
 .UNSPECIFIED. ) ;
#41865=CARTESIAN_POINT ( 'NONE',  ( 80.51726034258919640, 44.91748552740171618, -11.09860402559229442 ) ) ;
#41867=DIRECTION ( 'NONE',  ( 0.5000000000000013323, -0.8660254037844378194, 0.000000000000000000 ) ) ;
#41868=CARTESIAN_POINT ( 'NONE',  ( 87.98804127167099409, 43.77408088403165465, 2.388364124389103171 ) ) ;
#41875=CARTESIAN_POINT ( 'NONE',  ( 80.33434995892775987, 58.04101998076092883, 16.26088286722919207 ) ) ;
#41876=EDGE_CURVE ( 'NONE', #23100, #49399, #36681, .T. ) ;
#41879=CARTESIAN_POINT ( 'NONE',  ( 81.18390761377841613, 43.43123804279526468, -9.905827838957788956 ) ) ;
#41886=CARTESIAN_POINT ( 'NONE',  ( 66.18968672761215544, 68.49487770601442094, -4.881532527435788360 ) ) ;
#41887=CARTESIAN_POINT ( 'NONE',  ( 75.46732613426667058, 55.10851769043934922, -16.13625620877613542 ) ) ;
#41889=CYLINDRICAL_SURFACE ( 'NONE', #24116, 16.60714546451156792 ) ;
#41891=DIRECTION ( 'NONE',  ( 0.7235470741700498198, 0.1663964660674505380, -0.6699192843471699632 ) ) ;
#41893=CARTESIAN_POINT ( 'NONE',  ( 78.28713622914533232, 54.32488346555809500, -16.43848886914129892 ) ) ;
#41894=CARTESIAN_POINT ( 'NONE',  ( 76.80517106979452535, 63.30872754350402687, -15.45635652541256455 ) ) ;
#41899=CARTESIAN_POINT ( 'NONE',  ( 87.88902802526534686, 43.91876200309240375, 0.4180276961672018121 ) ) ;
#41902=CARTESIAN_POINT ( 'NONE',  ( 87.06600699492729234, 43.48165395943767209, -3.537923743661954390 ) ) ;
#41904=B_SPLINE_CURVE_WITH_KNOTS ( 'NONE', 3,
 ( #82165, #81657, #43605, #60281, #12740, #98329, #66416, #27433, #74542, #5121, #35008, #36001, #44089, #28923, #58790, #83143, #65908, #6106, #96865, #43089, #66905, #74032, #58307, #89284, #4620, #97343, #67405, #51201, #52195, #19832, #35513, #89761, #91239, #59284, #21804, #20330, #90766, #97834, #75522, #90263, #36502, #59795, #75032, #21317, #13712, #67912 ),
 .UNSPECIFIED., .F., .F.,
 ( 4, 1, 2, 2, 1, 2, 2, 1, 1, 2, 2, 1, 1, 2, 2, 1, 1, 2, 2, 1, 1, 1, 2, 2, 1, 1, 1, 2, 2, 4 ),
 ( 0.000000000000000000, 0.06250000000000548173, 0.09375000000000714706, 0.1250000000000088263, 0.1875000000000137945, 0.2187500000000155154, 0.2500000000000172085, 0.3125000000000211497, 0.3437500000000230926, 0.3593750000000227596, 0.3750000000000223710, 0.4375000000000270339, 0.4687500000000286993, 0.4843750000000284772, 0.5000000000000283107, 0.5625000000000256462, 0.5937500000000244249, 0.6093750000000237588, 0.6250000000000232037, 0.6875000000000237588, 0.7187500000000250910, 0.7343750000000247580, 0.7421875000000246470, 0.7500000000000245359, 0.8125000000000205391, 0.8437500000000190958, 0.8593750000000174305, 0.8671875000000165423, 0.8750000000000156541, 1.000000000000000000 ),
 .UNSPECIFIED. ) ;
#41905=B_SPLINE_CURVE_WITH_KNOTS ( 'NONE', 3,
 ( #48989, #64180, #11002, #33805, #9994, #71801, #65178, #87560, #2398, #96126, #73785, #88541, #33277, #10485, #72304, #95128, #80939, #11507, #42850, #34768, #65668, #96624, #25694, #4375, #27189, #56573, #58078, #35274, #66181, #27692, #2912, #89534, #64688, #95639, #70021, #44358, #31516, #13488, #84774, #28172, #15310, #53810, #23417, #90526, #59548, #93368 ),
 .UNSPECIFIED., .F., .F.,
 ( 4, 1, 2, 2, 1, 2, 2, 1, 1, 2, 2, 1, 1, 2, 2, 1, 1, 2, 2, 1, 1, 1, 2, 2, 1, 1, 1, 2, 2, 4 ),
 ( 0.000000000000000000, 0.06249999999999684974, 0.09374999999999356071, 0.1249999999999902578, 0.1874999999999888423, 0.2187499999999863165, 0.2499999999999837907, 0.3124999999999741318, 0.3437499999999710787, 0.3593749999999679146, 0.3749999999999648059, 0.4374999999999586997, 0.4687499999999537592, 0.4843749999999516498, 0.4999999999999495404, 0.5624999999999404920, 0.5937499999999356071, 0.6093749999999330536, 0.6249999999999305000, 0.6874999999999212852, 0.7187499999999167333, 0.7343749999999157341, 0.7421874999999152900, 0.7499999999999149569, 0.8124999999999369393, 0.8437499999999495959, 0.8593749999999559241, 0.8671874999999589217, 0.8749999999999620304, 1.000000000000000000 ),
 .UNSPECIFIED. ) ;
#41906=B_SPLINE_CURVE_WITH_KNOTS ( 'NONE', 3,
 ( #48408, #24598, #61595, #31194, #71223, #23093, #53983, #78825, #93542, #46386, #62085, #93029, #85456, #63600, #70700, #1314, #1816, #32700, #41793, #88470, #27117, #97050, #72742, #18519, #42778, #48915, #81840, #2323, #19535, #50892, #88981, #10415, #3814, #72227, #34695, #73221, #79850, #33723, #87486, #50397, #11921, #41285, #65596, #65105, #73711, #96546 ),
 .UNSPECIFIED., .F., .F.,
 ( 4, 1, 1, 1, 2, 2, 1, 1, 1, 2, 2, 1, 1, 2, 2, 1, 1, 2, 2, 1, 1, 2, 2, 1, 2, 2, 1, 2, 2, 4 ),
 ( 0.000000000000000000, 0.06250000000001047773, 0.09375000000001570966, 0.1093750000000168893, 0.1171875000000168615, 0.1250000000000168199, 0.1875000000000120459, 0.2187500000000090761, 0.2343750000000066891, 0.2421875000000068279, 0.2500000000000069389, 0.3125000000000091593, 0.3437500000000087708, 0.3593750000000084932, 0.3750000000000082157, 0.4375000000000059397, 0.4687500000000043299, 0.4843750000000029976, 0.5000000000000016653, 0.5624999999999990008, 0.5937499999999972244, 0.6093749999999966693, 0.6249999999999962252, 0.6874999999999936717, 0.7187499999999926725, 0.7499999999999916733, 0.8124999999999918954, 0.8437499999999930056, 0.8749999999999941158, 1.000000000000000000 ),
 .UNSPECIFIED. ) ;
#41909=CARTESIAN_POINT ( 'NONE',  ( 28.07469292777547309, 37.18502408145592852, 5.678558825948276656 ) ) ;
#41913=CARTESIAN_POINT ( 'NONE',  ( 12.48623565965559479, 28.18502408145590721, 5.678558825948277544 ) ) ;
#41921=CARTESIAN_POINT ( 'NONE',  ( 72.40694465691628068, 71.58314657692716310, 5.120125831695425234 ) ) ;
#41925=CARTESIAN_POINT ( 'NONE',  ( 26.48321701407081363, 20.45404122711134320, -8.090169943749478065 ) ) ;
#41930=CARTESIAN_POINT ( 'NONE',  ( 66.66342508697567837, 67.67433879810248243, 6.129251300726011209 ) ) ;
#41933=CARTESIAN_POINT ( 'NONE',  ( 77.28032690913880742, 63.06041134881660781, -15.26474268318221483 ) ) ;
#41939=CARTESIAN_POINT ( 'NONE',  ( 83.45060835225783080, 48.62234384012960930, 13.28461130177331739 ) ) ;
#41942=CARTESIAN_POINT ( 'NONE',  ( 33.57875857642567752, 25.10170272979928896, -7.433330006724141015 ) ) ;
#41943=CARTESIAN_POINT ( 'NONE',  ( 81.02328614318113864, 48.86991784794459193, -13.72398778456469515 ) ) ;
#41953=CARTESIAN_POINT ( 'NONE',  ( 85.66185486794186943, 48.65504738537000406, 12.40237352552430750 ) ) ;
#41959=CARTESIAN_POINT ( 'NONE',  ( 73.02433024948126672, 69.66517378990663190, 9.714162469163342806 ) ) ;
#41967=CARTESIAN_POINT ( 'NONE',  ( 87.16910242261623409, 46.28252156386203353, -8.511466890639647787 ) ) ;
#41968=CARTESIAN_POINT ( 'NONE',  ( 71.81073432603291451, 59.04159436426002827, 15.37513943015642326 ) ) ;
#41969=CARTESIAN_POINT ( 'NONE',  ( 68.32264545644088116, 65.60716676607681563, 10.42805899469778730 ) ) ;
#41978=CARTESIAN_POINT ( 'NONE',  ( 76.13295803453654287, 64.73339994552033261, -14.36036996180405190 ) ) ;
#41986=VERTEX_POINT ( 'NONE', #54359 ) ;
#41989=CARTESIAN_POINT ( 'NONE',  ( 82.80564809338142140, 40.64392876451551473, -1.326136484204850197 ) ) ;
#41997=CARTESIAN_POINT ( 'NONE',  ( 82.94122475514203074, 41.44431412578434504, 2.647178600289170625 ) ) ;
#41999=CARTESIAN_POINT ( 'NONE',  ( 78.13210272222134734, 61.89790046927922162, 15.71296101541392431 ) ) ;
#42004=CIRCLE ( 'NONE', #97094, 16.60714546451156792 ) ;
#42007=CARTESIAN_POINT ( 'NONE',  ( 74.24776760725281122, 55.43361526745665202, 16.12181039901651403 ) ) ;
#42008=LINE ( 'NONE', #27809, #77316 ) ;
#42009=CARTESIAN_POINT ( 'NONE',  ( 31.60618414714233637, 41.18080186712595747, 3.090169943749475401 ) ) ;
#42014=CARTESIAN_POINT ( 'NONE',  ( 87.04297504979803080, 43.76764958495436275, -2.970215472454977412 ) ) ;
#42018=CARTESIAN_POINT ( 'NONE',  ( 86.56732525555858615, 46.29823956478880120, 9.017236280094351741 ) ) ;
#42021=CARTESIAN_POINT ( 'NONE',  ( 82.22687830799615938, 41.30244536609086481, 5.429731213283951696 ) ) ;
#42025=CARTESIAN_POINT ( 'NONE',  ( 41.21417716447173518, 24.76426979415093044, 3.090169943749476733 ) ) ;
#42029=CARTESIAN_POINT ( 'NONE',  ( 8.420521286406058792, 20.56454794089039240, 10.00000000000000355 ) ) ;
#42046=CARTESIAN_POINT ( 'NONE',  ( 31.84670776885679899, 24.10170272979928541, -7.433330006724141015 ) ) ;
#42047=CARTESIAN_POINT ( 'NONE',  ( 72.99862419887072917, 70.74432240184056297, -7.503600154403820000 ) ) ;
#42048=CARTESIAN_POINT ( 'NONE',  ( 86.34910853269747122, 47.57366130196511023, -10.59375139789182008 ) ) ;
#42051=CARTESIAN_POINT ( 'NONE',  ( 17.19524200933981817, 21.87878583063841020, -9.188101187500006262 ) ) ;
#42052=DIRECTION ( 'NONE',  ( 0.4330127018922168558, -0.7499999999999987788, 0.5000000000000039968 ) ) ;
#42053=VERTEX_POINT ( 'NONE', #44776 ) ;
#42054=CARTESIAN_POINT ( 'NONE',  ( 72.41184042289110323, 71.17856470982957262, -6.087003264457405471 ) ) ;
#42055=ADVANCED_FACE ( 'NONE', ( #68089 ), #53865, .T. ) ;
#42068=CARTESIAN_POINT ( 'NONE',  ( 65.90172229746312382, 68.93994708409050531, -2.596590423560799277 ) ) ;
#42071=CARTESIAN_POINT ( 'NONE',  ( 72.87657325132509811, 57.63168087469550471, -16.31100355619141595 ) ) ;
#42072=CARTESIAN_POINT ( 'NONE',  ( 78.01756760496483878, 61.41364688087467272, -16.16017056289257425 ) ) ;
#42078=ORIENTED_EDGE ( 'NONE', *, *, #23312, .T. ) ;
#42079=CARTESIAN_POINT ( 'NONE',  ( 33.72069078606260462, 37.65586893147758474, -7.433330006724137462 ) ) ;
#42088=CARTESIAN_POINT ( 'NONE',  ( 75.61360636200772944, 58.23975808111319452, -16.00195830399037789 ) ) ;
#42089=CARTESIAN_POINT ( 'NONE',  ( 86.32174514625263839, 43.39275037566977034, -2.929684509001238446 ) ) ;
#42090=CARTESIAN_POINT ( 'NONE',  ( 66.23050080230359526, 68.70569274131929660, -4.319124887654028022 ) ) ;
#42104=CARTESIAN_POINT ( 'NONE',  ( 87.14406544511430752, 44.30059231523330965, -4.700414329343145958 ) ) ;
#42105=CARTESIAN_POINT ( 'NONE',  ( 84.75647422269858566, 42.83139927231500366, 4.116084768947018802 ) ) ;
#42108=CARTESIAN_POINT ( 'NONE',  ( 75.00576775672064400, 62.30322666060470738, 15.01846280378952692 ) ) ;
#42111=CARTESIAN_POINT ( 'NONE',  ( 80.07812099633126479, 57.44764983040322903, -16.59488970948942921 ) ) ;
#42112=CARTESIAN_POINT ( 'NONE',  ( 71.69140363859698084, 72.11128586088413783, 0.6349804937391964055 ) ) ;
#42119=CARTESIAN_POINT ( 'NONE',  ( 68.26860836083196205, 69.12837558592964626, 4.919393711847383166 ) ) ;
#42122=B_SPLINE_CURVE_WITH_KNOTS ( 'NONE', 3,
 ( #83218, #45174, #21877, #69473, #92324, #77070, #45659, #22378, #53276, #20914, #91317, #37079, #52763, #30476, #87, #14777 ),
 .UNSPECIFIED., .F., .F.,
 ( 4, 1, 2, 2, 2, 1, 2, 2, 4 ),
 ( 0.000000000000000000, 0.1249999999999992784, 0.1874999999999985567, 0.2499999999999978351, 0.4999999999999981126, 0.6249999999999982236, 0.6874999999999981126, 0.7499999999999980016, 1.000000000000000000 ),
 .UNSPECIFIED. ) ;
#42123=CARTESIAN_POINT ( 'NONE',  ( 16.98334746987260147, 25.50829794293879615, -10.00000000000000355 ) ) ;
#42130=CARTESIAN_POINT ( 'NONE',  ( 77.49896415157103036, 52.88957495811840204, -15.80880303492994443 ) ) ;
#42132=EDGE_CURVE ( 'NONE', #22055, #7928, #87859, .T. ) ;
#42138=CARTESIAN_POINT ( 'NONE',  ( 88.14558033319170249, 43.66656252067526367, 0.1579512601322914100 ) ) ;
#42140=CARTESIAN_POINT ( 'NONE',  ( 72.26473847452083987, 72.05163828152960548, -3.296940183535202351 ) ) ;
#42142=CARTESIAN_POINT ( 'NONE',  ( 73.83097814971496575, 55.11266741107668565, -16.12521890440442718 ) ) ;
#42153=CARTESIAN_POINT ( 'NONE',  ( 37.36761971798259196, 27.28920272979929607, -7.433330006724141015 ) ) ;
#42157=CARTESIAN_POINT ( 'NONE',  ( 30.81771801958594281, 39.83396525600392835, -2.839279412974133887 ) ) ;
#42160=CARTESIAN_POINT ( 'NONE',  ( 81.19656099875513178, 43.43094936621162105, -9.896970666190503252 ) ) ;
#42164=CARTESIAN_POINT ( 'NONE',  ( 11.67313376208573139, 15.24335787977761747, -9.188101187500008038 ) ) ;
#42166=CARTESIAN_POINT ( 'NONE',  ( 13.49720994389718598, 29.83396525600389637, -2.839279412974133887 ) ) ;
#42177=CARTESIAN_POINT ( 'NONE',  ( 87.54989630752690744, 45.07147448993671901, 6.930566558073848249 ) ) ;
#42179=( BOUNDED_CURVE ( )  B_SPLINE_CURVE ( 2, ( #99414, #45674, #46168, #30987, #67997, #62370, #76599, #99909, #61873, #93327, #30494, #92337, #29498 ),
 .UNSPECIFIED., .F., .T. ) 
 B_SPLINE_CURVE_WITH_KNOTS ( ( 3, 2, 2, 2, 2, 2, 3 ),
 ( 0.8125000000000000000, 0.8149999999999999467, 0.8199999999999999512, 0.8249999999999999556, 0.8299999999999999600, 0.8349999999999999645, 0.8375000000000000222 ),
 .UNSPECIFIED. ) 
 CURVE ( )  GEOMETRIC_REPRESENTATION_ITEM ( )  RATIONAL_B_SPLINE_CURVE ( ( 0.9755282581475768211, 0.9755282581475768211, 1.000000000000000000, 0.9510565162951535312, 1.000000000000000000, 0.9510565162951535312, 1.000000000000000000, 0.9510565162951535312, 1.000000000000000000, 0.9510565162951535312, 1.000000000000000000, 0.9755282581475761550, 0.9755282581475767101 ) ) 
 REPRESENTATION_ITEM ( '' )  );
#42182=CARTESIAN_POINT ( 'NONE',  ( 86.12260107077111115, 47.06852444819536885, 10.76136662946663947 ) ) ;
#42184=CARTESIAN_POINT ( 'NONE',  ( 80.15404930735284950, 58.24487849859603017, -16.60713908503101877 ) ) ;
#42187=CARTESIAN_POINT ( 'NONE',  ( 28.73071361209859731, 38.36126292948897287, 6.180339887498949913 ) ) ;
#42188=EDGE_CURVE ( 'NONE', #26733, #59353, #93929, .T. ) ;
#42189=CARTESIAN_POINT ( 'NONE',  ( 79.79546047556335964, 49.97060089421696460, -14.59098784290960538 ) ) ;
#42206=CARTESIAN_POINT ( 'NONE',  ( 71.65767651694793017, 69.82614052466774979, 7.647303713463401209 ) ) ;
#42208=CARTESIAN_POINT ( 'NONE',  ( 87.35192423430838460, 43.74464389095077621, 1.893651613221468688 ) ) ;
#42212=CARTESIAN_POINT ( 'NONE',  ( 22.71735025659390317, 28.51421378149919406, -9.188101187500004485 ) ) ;
#42220=CARTESIAN_POINT ( 'NONE',  ( 69.32645819574260315, 62.94046279709883152, 13.62531992251986246 ) ) ;
#42227=CARTESIAN_POINT ( 'NONE',  ( 9.861089372814316079, 17.64441083166259006, -10.00000000000000533 ) ) ;
#42232=DIRECTION ( 'NONE',  ( -0.9133924323370935516, 0.1624253398589796948, -0.3732723851573047091 ) ) ;
#42233=DIRECTION ( 'NONE',  ( 0.2938926261462335709, -0.5090369604551240323, 0.8090169943749504489 ) ) ;
#42241=ADVANCED_FACE ( 'NONE', ( #48294 ), #96712, .T. ) ;
#42242=CARTESIAN_POINT ( 'NONE',  ( 78.36279588851795097, 47.41043415324340771, -13.73196331463247688 ) ) ;
#42243=CARTESIAN_POINT ( 'NONE',  ( 75.98104421109889017, 51.53574906954564483, 16.18761828508177203 ) ) ;
#42252=CARTESIAN_POINT ( 'NONE',  ( 78.99848661620951873, 60.24637179098722584, -16.44349368446545867 ) ) ;
#42264=ORIENTED_EDGE ( 'NONE', *, *, #31981, .F. ) ;
#42269=CARTESIAN_POINT ( 'NONE',  ( 23.51121325743158508, 19.28920272979927120, -7.433330006724141015 ) ) ;
#42270=CARTESIAN_POINT ( 'NONE',  ( 74.84209865657220462, 67.13651163270155564, 12.97079428878455509 ) ) ;
#42274=CARTESIAN_POINT ( 'NONE',  ( 22.44855073024449155, 13.36477965099640208, 1.583844403245364907 ) ) ;
#42280=CARTESIAN_POINT ( 'NONE',  ( 81.62968001876643598, 55.78593752935011452, -16.36028778889455282 ) ) ;
#42284=EDGE_CURVE ( 'NONE', #62590, #26159, #36563, .T. ) ;
#42286=CARTESIAN_POINT ( 'NONE',  ( 71.69055946895421982, 72.48590965862314306, 0.9596580914388839201 ) ) ;
#42287=CARTESIAN_POINT ( 'NONE',  ( 71.64316818921393804, 72.05741665177616539, -3.509880912999890690 ) ) ;
#42290=CARTESIAN_POINT ( 'NONE',  ( 71.14876058709654671, 71.77059820202033791, -0.7402833220517009982 ) ) ;
#42292=ADVANCED_FACE ( 'NONE', ( #51790 ), #75095, .T. ) ;
#42294=CARTESIAN_POINT ( 'NONE',  ( 13.85453579343919905, 10.12755873383624206, -6.180339887498949025 ) ) ;
#42298=CARTESIAN_POINT ( 'NONE',  ( 38.08139550823666042, 22.39040679176985904, -6.890680421881970419E-14 ) ) ;
#42300=EDGE_LOOP ( 'NONE', ( #52274, #44239, #44456, #44586 ) ) ;
#42301=CARTESIAN_POINT ( 'NONE',  ( 79.06565384122613693, 60.08000270057965508, 16.12336209646970886 ) ) ;
#42307=CARTESIAN_POINT ( 'NONE',  ( 73.47631802762754205, 69.90797475050369769, -9.735925655486411756 ) ) ;
#42308=CARTESIAN_POINT ( 'NONE',  ( 84.60292230380740364, 49.80262622141071915, -13.18993139652274671 ) ) ;
#42310=EDGE_CURVE ( 'NONE', #67514, #83087, #9950, .T. ) ;
#42322=CARTESIAN_POINT ( 'NONE',  ( 81.96055694566001648, 41.06594365097284793, 3.414074282795390936 ) ) ;
#42323=CARTESIAN_POINT ( 'NONE',  ( 80.61273461444635302, 43.38457209157425609, -9.435640752088607641 ) ) ;
#42332=CARTESIAN_POINT ( 'NONE',  ( 9.553764119070452310, 20.91421378149917132, 9.188101187500008038 ) ) ;
#42339=CARTESIAN_POINT ( 'NONE',  ( 70.44287837739904035, 60.93660230331288830, 14.43604447541618008 ) ) ;
#42343=CARTESIAN_POINT ( 'NONE',  ( 88.23959751488011705, 43.87687695675944610, -2.120018653157903721 ) ) ;
#42346=CARTESIAN_POINT ( 'NONE',  ( 65.79394124285487067, 69.11298328710827832, 0.1263844587676525022 ) ) ;
#42348=DIRECTION ( 'NONE',  ( -0.5242119900219359696, 0.000000000000000000, 0.8515878049368965641 ) ) ;
#42354=CARTESIAN_POINT ( 'NONE',  ( 87.92119597943950282, 44.20992230385985522, 2.809437090033895856 ) ) ;
#42359=CARTESIAN_POINT ( 'NONE',  ( 75.68423863107267380, 61.28764373785409703, -15.43813584130047367 ) ) ;
#42360=EDGE_CURVE ( 'NONE', #71854, #7443, #52879, .T. ) ;
#42363=CARTESIAN_POINT ( 'NONE',  ( 80.90469142059797036, 42.95404229843371979, -9.526595558722311452 ) ) ;
#42368=CARTESIAN_POINT ( 'NONE',  ( 87.98904372666932261, 44.25610683789894750, -4.385737539232402504 ) ) ;
#42377=EDGE_CURVE ( 'NONE', #47356, #97296, #79491, .T. ) ;
#42380=CARTESIAN_POINT ( 'NONE',  ( 74.28057495708935676, 56.36868286471138845, -16.09213986559992549 ) ) ;
#42390=DIRECTION ( 'NONE',  ( -0.5000000000000013323, 0.8660254037844378194, 0.000000000000000000 ) ) ;
#42393=CARTESIAN_POINT ( 'NONE',  ( 35.55378427144160014, 29.03085787977765264, 9.188101187500006262 ) ) ;
#42397=CARTESIAN_POINT ( 'NONE',  ( 20.11807774711229868, 23.56628583063840665, 9.188101187500006262 ) ) ;
#42402=CARTESIAN_POINT ( 'NONE',  ( 86.72009611066519597, 47.05274629621921889, 10.38319007345879541 ) ) ;
#42408=CARTESIAN_POINT ( 'NONE',  ( 75.17844314609712342, 53.08451609724016151, 16.49030186085838778 ) ) ;
#42414=ORIENTED_EDGE ( 'NONE', *, *, #5153, .T. ) ;
#42416=EDGE_LOOP ( 'NONE', ( #86111, #62464, #54267, #37296 ) ) ;
#42423=EDGE_CURVE ( 'NONE', #28265, #67548, #33518, .T. ) ;
#42424=CARTESIAN_POINT ( 'NONE',  ( 38.36533659613348846, 24.01110640527295104, 2.839279412974134775 ) ) ;
#42425=CARTESIAN_POINT ( 'NONE',  ( 70.98683038387876820, 61.11472152276905234, -14.49225651734632692 ) ) ;
#42428=ORIENTED_EDGE ( 'NONE', *, *, #87623, .F. ) ;
#42429=ORIENTED_EDGE ( 'NONE', *, *, #95893, .F. ) ;
#42433=CARTESIAN_POINT ( 'NONE',  ( 85.94797495143531307, 48.32083425265168586, 12.00338787116683470 ) ) ;
#42448=CARTESIAN_POINT ( 'NONE',  ( 87.23257741107988750, 46.04474800944700519, -8.789869334516776433 ) ) ;
#42452=CARTESIAN_POINT ( 'NONE',  ( 7.026152882275393807, 27.55466486950697913, -1.111400068045478839E-16 ) ) ;
#42456=VERTEX_POINT ( 'NONE', #43921 ) ;
#42465=CARTESIAN_POINT ( 'NONE',  ( 69.59544983168204624, 63.11080376311066686, -13.61608123681405758 ) ) ;
#42470=CARTESIAN_POINT ( 'NONE',  ( 81.48768738999534378, 47.92560860843236981, 13.01067380738259160 ) ) ;
#42471=CARTESIAN_POINT ( 'NONE',  ( 81.95337945677349012, 41.00406898985013271, -3.180093734862122545 ) ) ;
#42477=DIRECTION ( 'NONE',  ( 0.000000000000000000, 0.000000000000000000, -1.000000000000000000 ) ) ;
#42479=CARTESIAN_POINT ( 'NONE',  ( 80.86831763631852255, 54.93583156370407039, 15.92778375911414024 ) ) ;
#42480=CARTESIAN_POINT ( 'NONE',  ( 66.46320885748656337, 68.94986384069261476, 0.01364106734875079018 ) ) ;
#42481=CARTESIAN_POINT ( 'NONE',  ( 23.90043047733868420, 15.92755873383626408, 6.180339887498953466 ) ) ;
#42482=CARTESIAN_POINT ( 'NONE',  ( 78.34913526621272695, 61.55915279984171917, 16.16953766326405528 ) ) ;
#42484=CARTESIAN_POINT ( 'NONE',  ( 89.81297465553679160, 45.16368336106900472, 0.1873032967079516220 ) ) ;
#42486=CARTESIAN_POINT ( 'NONE',  ( 70.50619853993235608, 64.86658464427489434, -12.22208435811523763 ) ) ;
#42490=CARTESIAN_POINT ( 'NONE',  ( 30.13164393277487818, 36.13478043621390157, 8.090169943749478065 ) ) ;
#42493=CARTESIAN_POINT ( 'NONE',  ( 71.77677790152782222, 58.69870002817014409, -15.46647683744001966 ) ) ;
#42494=CARTESIAN_POINT ( 'NONE',  ( 83.43238562051314489, 43.24558130407336876, -6.915862364849616029 ) ) ;
#42498=ORIENTED_EDGE ( 'NONE', *, *, #44925, .T. ) ;
#42499=CARTESIAN_POINT ( 'NONE',  ( 87.13013406632065028, 46.22635825882438354, 8.450982903413489566 ) ) ;
#42502=CARTESIAN_POINT ( 'NONE',  ( 81.75700027247154367, 41.62903602420404070, 5.464259697822261508 ) ) ;
#42505=CARTESIAN_POINT ( 'NONE',  ( 87.13039101863441260, 46.06611145402069241, 8.900391155234917306 ) ) ;
#42507=CARTESIAN_POINT ( 'NONE',  ( 36.78445495848383473, 29.43677371833804202, -10.00000000000000355 ) ) ;
#42511=CARTESIAN_POINT ( 'NONE',  ( 73.03896240731778278, 67.55704344529559080, -11.28667427251763655 ) ) ;
#42512=CARTESIAN_POINT ( 'NONE',  ( 82.78345634833958400, 53.69061190982763776, 15.38144188222361386 ) ) ;
#42514=CARTESIAN_POINT ( 'NONE',  ( 83.48272809759448876, 51.94771123612189001, 15.01134753452855009 ) ) ;
#42519=ADVANCED_FACE ( 'NONE', ( #6439 ), #60603, .T. ) ;
#42526=CARTESIAN_POINT ( 'NONE',  ( 67.00635898293039361, 66.93325455025599524, -8.753795382997793695 ) ) ;
#42532=CARTESIAN_POINT ( 'NONE',  ( 29.70508255828911004, 19.01110640527293327, 2.839279412974134775 ) ) ;
#42537=CARTESIAN_POINT ( 'NONE',  ( 18.12859834787737157, 11.26216523072493736, -2.296566073217252530E-15 ) ) ;
#42538=CARTESIAN_POINT ( 'NONE',  ( 76.03006974497249360, 60.13132759335589128, 15.77593001480065737 ) ) ;
#42542=ORIENTED_EDGE ( 'NONE', *, *, #76116, .T. ) ;
#42551=CARTESIAN_POINT ( 'NONE',  ( 66.26306969915694367, 68.66842913227013412, -2.141827346873069970 ) ) ;
#42553=CARTESIAN_POINT ( 'NONE',  ( 72.91150845015395987, 57.63568554243673248, -16.31368332975456781 ) ) ;
#42554=CARTESIAN_POINT ( 'NONE',  ( 78.35677645844283745, 61.14921145379764056, -15.90198519767692353 ) ) ;
#42558=CARTESIAN_POINT ( 'NONE',  ( 69.03518170984699509, 64.49507618471645287, 12.45339560606362284 ) ) ;
#42562=CARTESIAN_POINT ( 'NONE',  ( 31.98863997849372254, 36.65586893147758474, -7.433330006724137462 ) ) ;
#42564=CARTESIAN_POINT ( 'NONE',  ( 75.32821269442784740, 66.69330675534777697, -13.02113851420497603 ) ) ;
#42573=CARTESIAN_POINT ( 'NONE',  ( 81.10561266023913163, 56.14635974680164310, -16.08662763877836355 ) ) ;
#42575=VERTEX_POINT ( 'NONE', #73601 ) ;
#42577=CARTESIAN_POINT ( 'NONE',  ( 70.82877176157455779, 69.82901014346172985, -6.773049970042206880 ) ) ;
#42590=CARTESIAN_POINT ( 'NONE',  ( 85.72596786555051551, 44.18998096972852352, -6.301796949671089720 ) ) ;
#42595=CARTESIAN_POINT ( 'NONE',  ( 74.46953503235177152, 59.54388530620969533, 15.67556957382890559 ) ) ;
#42598=CARTESIAN_POINT ( 'NONE',  ( 80.29543856085656728, 57.12815561284512711, -16.23372326876640770 ) ) ;
#42610=CARTESIAN_POINT ( 'NONE',  ( 14.52789699003380974, 30.16126292948894871, -6.180339887498951690 ) ) ;
#42619=CARTESIAN_POINT ( 'NONE',  ( 25.62571989635185332, 15.76426979415090202, 3.090169943749476733 ) ) ;
#42620=ORIENTED_EDGE ( 'NONE', *, *, #30455, .F. ) ;
#42627=CARTESIAN_POINT ( 'NONE',  ( 16.89228056887236917, 28.49103043416548786, -8.090169943749479842 ) ) ;
#42632=CARTESIAN_POINT ( 'NONE',  ( 74.14739530845520221, 55.62984604024180868, -16.59005736389721619 ) ) ;
#42635=CARTESIAN_POINT ( 'NONE',  ( 75.06169617786551385, 67.15492690307928569, 12.60468746697864439 ) ) ;
#42637=DIRECTION ( 'NONE',  ( 0.8660254037844341557, 0.5000000000000082157, -0.000000000000000000 ) ) ;
#42639=CARTESIAN_POINT ( 'NONE',  ( 66.60661563016273590, 67.77273566365288104, -7.043189648870077590 ) ) ;
#42644=CARTESIAN_POINT ( 'NONE',  ( 30.44305165777243971, 40.68290643055189548, 3.479690158560446702E-15 ) ) ;
#42648=CARTESIAN_POINT ( 'NONE',  ( 34.71711421221060334, 41.81751292744059612, -6.180339887498951690 ) ) ;
#42650=CARTESIAN_POINT ( 'NONE',  ( 14.11662529016922640, 10.01110640527290663, 2.839279412974134775 ) ) ;
#42651=CARTESIAN_POINT ( 'NONE',  ( 71.69055946895423403, 72.48590965862312885, 0.9596580914388637140 ) ) ;
#42652=CARTESIAN_POINT ( 'NONE',  ( 22.55376741186237410, 15.94754757982089544, 5.678558825948272215 ) ) ;
#42654=AXIS2_PLACEMENT_3D ( 'NONE', #62839, #39028, #30945 ) ;
#42662=DIRECTION ( 'NONE',  ( -0.8660254037844379305, -0.5000000000000014433, -0.000000000000000000 ) ) ;
#42668=DIRECTION ( 'NONE',  ( 0.3297783986044549587, 0.8484238185761712181, -0.4140328874455618258 ) ) ;
#42687=EDGE_LOOP ( 'NONE', ( #20177, #5436, #18820, #52293, #8910 ) ) ;
#42694=CARTESIAN_POINT ( 'NONE',  ( 82.74741872462533365, 53.81327073439516795, 15.79824936317409545 ) ) ;
#42695=CARTESIAN_POINT ( 'NONE',  ( 10.64836937555893570, 29.08080186712591697, -3.090169943749475845 ) ) ;
#42701=CARTESIAN_POINT ( 'NONE',  ( 25.52954022263672940, 23.24335787977764411, -9.188101187500008038 ) ) ;
#42709=CARTESIAN_POINT ( 'NONE',  ( 16.82306525903893046, 33.21091486745860522, -1.111400068045478839E-16 ) ) ;
#42710=CARTESIAN_POINT ( 'NONE',  ( 17.22757050757671493, 15.11029122506293554, -8.090169943749478065 ) ) ;
#42720=CARTESIAN_POINT ( 'NONE',  ( 82.80564809348420852, 40.64392876433748825, -1.326136484287901096 ) ) ;
#42722=CARTESIAN_POINT ( 'NONE',  ( 84.72015715327184182, 50.52193132731910197, 13.57015802400779947 ) ) ;
#42730=CARTESIAN_POINT ( 'NONE',  ( 87.27117856089937220, 44.98890866680353895, -6.231534082530021834 ) ) ;
#42737=B_SPLINE_CURVE_WITH_KNOTS ( 'NONE', 3,
 ( #85427, #31165, #53469, #22084, #54450, #69672, #47370, #8876, #70673, #77801, #62054, #76306, #61066, #61567, #39744, #6878, #7372, #77281, #15458, #84915, #278, #46356, #7891, #38258, #93005, #1288, #16475, #23558, #37768, #38768, #92035, #68671, #53958, #76779, #52980, #83929, #100103, #30178, #15975, #22582, #30687, #85947, #99596, #46876, #93518, #14968 ),
 .UNSPECIFIED., .F., .F.,
 ( 4, 1, 1, 1, 2, 2, 1, 1, 1, 2, 2, 1, 1, 2, 2, 1, 1, 2, 2, 1, 1, 2, 2, 1, 2, 2, 1, 2, 2, 4 ),
 ( 0.000000000000000000, 0.06249999999996815048, 0.09374999999995237143, 0.1093749999999444888, 0.1171874999999418798, 0.1249999999999392708, 0.1874999999999252265, 0.2187499999999161504, 0.2343749999999128752, 0.2421874999999134304, 0.2499999999999140132, 0.3124999999999193423, 0.3437499999999231726, 0.3593749999999252265, 0.3749999999999272249, 0.4374999999999390488, 0.4687499999999459321, 0.4843749999999473754, 0.4999999999999489297, 0.5624999999999630296, 0.5937499999999682476, 0.6093749999999708011, 0.6249999999999733546, 0.6874999999999765743, 0.7187499999999773515, 0.7499999999999780176, 0.8124999999999832356, 0.8437499999999856781, 0.8749999999999882316, 1.000000000000000000 ),
 .UNSPECIFIED. ) ;
#42741=CARTESIAN_POINT ( 'NONE',  ( 83.55693731525771284, 46.16036024266245619, 10.67923881757085525 ) ) ;
#42746=CARTESIAN_POINT ( 'NONE',  ( 72.69493809724966127, 71.16443809380129437, -7.267007365939471164 ) ) ;
#42750=CARTESIAN_POINT ( 'NONE',  ( 72.38858704899024588, 72.34360798638101642, 0.000000000000000000 ) ) ;
#42752=CARTESIAN_POINT ( 'NONE',  ( 68.80363134320050733, 67.62982772949345645, 8.378572803659114498 ) ) ;
#42760=CARTESIAN_POINT ( 'NONE',  ( 24.83368966200164607, 16.19860640527292261, 2.839279412974134775 ) ) ;
#42761=CARTESIAN_POINT ( 'NONE',  ( 74.74196695595742312, 67.08715363026114176, 12.96493619559571897 ) ) ;
#42766=B_SPLINE_CURVE_WITH_KNOTS ( 'NONE', 3,
 ( #60927, #20981, #91891, #52342, #84291, #14838, #90904, #13851, #67544, #75662 ),
 .UNSPECIFIED., .F., .F.,
 ( 4, 2, 2, 2, 4 ),
 ( 0.000000000000000000, 0.0002622400424273148181, 0.0005244800848546296362, 0.0007867201272819444001, 0.001048960169709259272 ),
 .UNSPECIFIED. ) ;
#42770=CARTESIAN_POINT ( 'NONE',  ( 82.41630873631589793, 41.31828431233920895, -3.367117793111288560 ) ) ;
#42772=CARTESIAN_POINT ( 'NONE',  ( 81.39796143918844962, 55.18843397982647758, -15.93664522424668917 ) ) ;
#42776=CARTESIAN_POINT ( 'NONE',  ( 72.01395728112395034, 72.29389942223538412, 0.6844073223025460839 ) ) ;
#42778=CARTESIAN_POINT ( 'NONE',  ( 79.78296747758277263, 52.56098969188083458, 15.47212231616918388 ) ) ;
#42780=CARTESIAN_POINT ( 'NONE',  ( 71.09572938139255882, 71.74208345363453532, -0.6570354662424334746 ) ) ;
#42783=CARTESIAN_POINT ( 'NONE',  ( 12.10719531124914283, 12.15404122711131585, 8.090169943749479842 ) ) ;
#42790=CARTESIAN_POINT ( 'NONE',  ( 79.24589768621441976, 59.96875100242885992, 16.14305910152894796 ) ) ;
#42796=CARTESIAN_POINT ( 'NONE',  ( 82.58801462665896054, 50.50509293822858581, -14.17187532088357926 ) ) ;
#42806=CARTESIAN_POINT ( 'NONE',  ( 75.06692456002483027, 59.04669605262043319, 15.83186505758761164 ) ) ;
#42810=CARTESIAN_POINT ( 'NONE',  ( 82.19055047383055523, 40.63346341616176716, 3.399030102818711541 ) ) ;
#42814=EDGE_CURVE ( 'NONE', #43232, #9334, #34765, .T. ) ;
#42820=CARTESIAN_POINT ( 'NONE',  ( 70.72338235425743846, 61.42563111389683428, -14.82496901324692296 ) ) ;
#42821=CARTESIAN_POINT ( 'NONE',  ( 7.976297994771393896, 26.64646525600388571, -2.839279412974133887 ) ) ;
#42827=CARTESIAN_POINT ( 'NONE',  ( 76.26781202851402952, 65.13109020310881192, -14.20137929745961003 ) ) ;
#42829=CARTESIAN_POINT ( 'NONE',  ( 78.10439711566577614, 51.17412554839856398, -15.81061020820859575 ) ) ;
#42831=CARTESIAN_POINT ( 'NONE',  ( 85.34255252599106711, 42.75911001269964373, 2.438663257353666403 ) ) ;
#42832=CARTESIAN_POINT ( 'NONE',  ( 88.01997546958394025, 44.08896826132783531, -1.712360037130413737 ) ) ;
#42835=EDGE_LOOP ( 'NONE', ( #21045, #18313, #21486, #4612 ) ) ;
#42842=CARTESIAN_POINT ( 'NONE',  ( 88.44572534255364360, 43.94768732639445830, 1.766277459783984538 ) ) ;
#42847=CARTESIAN_POINT ( 'NONE',  ( 79.19548930461120051, 59.90515312544787463, -16.13566294680263624 ) ) ;
#42848=CARTESIAN_POINT ( 'NONE',  ( 80.56202954020663753, 57.53823600680942718, 16.23110421993949259 ) ) ;
#42850=CARTESIAN_POINT ( 'NONE',  ( 72.32858194273194385, 65.82052004871619033, -12.34639520340021868 ) ) ;
#42853=CARTESIAN_POINT ( 'NONE',  ( 80.92473437028310457, 43.34290539593628466, -9.976869929326982245 ) ) ;
#42858=PLANE ( 'NONE',  #33741 ) ;
#42866=CARTESIAN_POINT ( 'NONE',  ( 84.47262166381923976, 50.18302823219130460, 13.87459367389479326 ) ) ;
#42876=CARTESIAN_POINT ( 'NONE',  ( 72.21491844529387549, 53.64441083166271085, 0.000000000000000000 ) ) ;
#42877=CARTESIAN_POINT ( 'NONE',  ( 75.79515598915105556, 65.48576791014883725, 14.28791538466101230 ) ) ;
#42879=CARTESIAN_POINT ( 'NONE',  ( 32.24243340009443415, 30.56628583063843152, 9.188101187500006262 ) ) ;
#42883=CARTESIAN_POINT ( 'NONE',  ( 27.74991983456899902, 18.94754757982090254, 5.678558825948272215 ) ) ;
#42890=CARTESIAN_POINT ( 'NONE',  ( 75.63268008801898645, 65.14737934564519151, -14.41129995628931404 ) ) ;
#42893=CARTESIAN_POINT ( 'NONE',  ( 74.83655476915186000, 53.51806293172402462, 16.54630480363988809 ) ) ;
#42895=CARTESIAN_POINT ( 'NONE',  ( 85.85265132163429769, 47.44586991713102009, 10.77177032529229450 ) ) ;
#42898=CARTESIAN_POINT ( 'NONE',  ( 82.93531674994763137, 41.19304737833027019, 0.2619559300746566732 ) ) ;
#42903=CARTESIAN_POINT ( 'NONE',  ( 13.50136424336972141, 8.764269794150880699, 3.090169943749476733 ) ) ;
#42905=CARTESIAN_POINT ( 'NONE',  ( 88.07467786089314643, 44.31731248180877714, -4.422775558719202138 ) ) ;
#42909=CARTESIAN_POINT ( 'NONE',  ( 31.91767387367526609, 30.37878583063843152, 9.188101187500006262 ) ) ;
#42910=CARTESIAN_POINT ( 'NONE',  ( 75.70354921996640485, 59.76282743397471364, -15.78267976543943085 ) ) ;
#42917=CARTESIAN_POINT ( 'NONE',  ( 73.16956295238907160, 57.33411781477383329, 16.38320611710937058 ) ) ;
#42921=CARTESIAN_POINT ( 'NONE',  ( 85.39714985353326426, 48.29561332581459965, -11.77387981254187999 ) ) ;
#42931=CARTESIAN_POINT ( 'NONE',  ( 73.74866502313744832, 55.21092590717630344, -16.59690200530987170 ) ) ;
#42933=VERTEX_POINT ( 'NONE', #80118 ) ;
#42936=CARTESIAN_POINT ( 'NONE',  ( 87.07436038242185816, 45.84038486297258430, -8.630882807222770126 ) ) ;
#42944=AXIS2_PLACEMENT_3D ( 'NONE', #85477, #100149, #21640 ) ;
#42947=EDGE_LOOP ( 'NONE', ( #12760, #89490, #21164, #89411 ) ) ;
#42951=CARTESIAN_POINT ( 'NONE',  ( 26.29472225869274382, 23.38052372038641735, 10.00000000000000533 ) ) ;
#42952=CARTESIAN_POINT ( 'NONE',  ( 82.68642609916942376, 45.53004534498515454, 10.54796185080066984 ) ) ;
#42960=CARTESIAN_POINT ( 'NONE',  ( 82.21456097586059286, 40.60959159724548329, -3.238575740498558897 ) ) ;
#42964=CARTESIAN_POINT ( 'NONE',  ( 82.57296292288040718, 40.92493348698932465, -3.680003806365853336 ) ) ;
#42976=CARTESIAN_POINT ( 'NONE',  ( 72.06748121909076588, 71.10123967445895232, -5.802816214387736871 ) ) ;
#42977=CARTESIAN_POINT ( 'NONE',  ( 73.41259731428677071, 70.10201033320841191, -9.453773877498623079 ) ) ;
#42981=CARTESIAN_POINT ( 'NONE',  ( 41.98277471387834225, 25.20801979619931998, -3.090169943749474069 ) ) ;
#42986=CARTESIAN_POINT ( 'NONE',  ( 85.26069992303990830, 43.42143465718991280, -5.099252233888901920 ) ) ;
#42990=ORIENTED_EDGE ( 'NONE', *, *, #9051, .T. ) ;
#42991=CARTESIAN_POINT ( 'NONE',  ( 87.15721324309708962, 46.06501070407752252, 8.877681887861816890 ) ) ;
#42992=CARTESIAN_POINT ( 'NONE',  ( 18.79197634579341525, 22.80066082961421614, 10.00000000000000533 ) ) ;
#42993=CARTESIAN_POINT ( 'NONE',  ( 37.37984742713354791, 29.78052372038643369, -10.00000000000000355 ) ) ;
#42995=CARTESIAN_POINT ( 'NONE',  ( 87.25346308258933448, 46.04525953206349698, 8.773708642049088624 ) ) ;
#42998=CARTESIAN_POINT ( 'NONE',  ( 43.01983786573178037, 33.03677371833806120, 10.00000000000000533 ) ) ;
#43001=AXIS2_PLACEMENT_3D ( 'NONE', #20693, #72921, #3512 ) ;
#43006=VECTOR ( 'NONE', #58444, 1000.000000000000114 ) ;
#43009=CYLINDRICAL_SURFACE ( 'NONE', #53861, 16.60714546451156792 ) ;
#43011=ORIENTED_EDGE ( 'NONE', *, *, #33898, .T. ) ;
#43016=CARTESIAN_POINT ( 'NONE',  ( 67.26473598584114200, 66.56549206475087033, -8.572050621364043721 ) ) ;
#43021=CARTESIAN_POINT ( 'NONE',  ( 30.18562306610639112, 29.37878583063842441, 9.188101187500006262 ) ) ;
#43023=CARTESIAN_POINT ( 'NONE',  ( 86.52710474712628752, 47.22253658430707901, -10.13945441009946968 ) ) ;
#43026=CARTESIAN_POINT ( 'NONE',  ( 9.708348802340269756, 27.64646525600388571, -2.839279412974133887 ) ) ;
#43027=CARTESIAN_POINT ( 'NONE',  ( 31.15319227796116053, 18.39040679176984128, -6.890680421881970419E-14 ) ) ;
#43033=CARTESIAN_POINT ( 'NONE',  ( 76.67567146729665239, 63.34086528488000312, -15.41964329106466103 ) ) ;
#43040=CARTESIAN_POINT ( 'NONE',  ( 66.11215637706905568, 68.56181850691201873, -2.272870840636120882 ) ) ;
#43043=CARTESIAN_POINT ( 'NONE',  ( 78.30529379001707468, 61.64230706715306241, -15.78713534414099051 ) ) ;
#43044=CARTESIAN_POINT ( 'NONE',  ( 72.13964350835141204, 72.31942673879332517, -1.245071394591160674 ) ) ;
#43052=CARTESIAN_POINT ( 'NONE',  ( 34.51575008502857855, 31.87878583063843863, -9.188101187500006262 ) ) ;
#43054=CARTESIAN_POINT ( 'NONE',  ( 75.23976045582850247, 66.94057334133056258, -12.81464017275781941 ) ) ;
#43059=( BOUNDED_CURVE ( )  B_SPLINE_CURVE ( 2, ( #35832, #34823, #90589, #4433, #11560, #81478, #12051, #21635, #89113, #5440, #42903, #36323, #96680 ),
 .UNSPECIFIED., .F., .T. ) 
 B_SPLINE_CURVE_WITH_KNOTS ( ( 3, 2, 2, 2, 2, 2, 3 ),
 ( 0.01250000000000000069, 0.01499999999999999944, 0.02000000000000000042, 0.02500000000000000139, 0.02999999999999999889, 0.03500000000000000333, 0.03750000000000000555 ),
 .UNSPECIFIED. ) 
 CURVE ( )  GEOMETRIC_REPRESENTATION_ITEM ( )  RATIONAL_B_SPLINE_CURVE ( ( 0.9755282581475768211, 0.9755282581475768211, 1.000000000000000000, 0.9510565162951535312, 1.000000000000000000, 0.9510565162951535312, 1.000000000000000000, 0.9510565162951535312, 1.000000000000000000, 0.9510565162951535312, 1.000000000000000000, 0.9755282581475767101, 0.9755282581475768211 ) ) 
 REPRESENTATION_ITEM ( '' )  );
#43060=CARTESIAN_POINT ( 'NONE',  ( 81.66071111044179531, 55.73219010195405332, 16.34934455148813370 ) ) ;
#43066=CARTESIAN_POINT ( 'NONE',  ( 75.00750624606230588, 62.98958700368800834, -14.74961995160845163 ) ) ;
#43067=CARTESIAN_POINT ( 'NONE',  ( 66.06012914866342101, 68.52786067758134436, -4.567821539730282154 ) ) ;
#43073=CARTESIAN_POINT ( 'NONE',  ( 80.57137527226012708, 55.64701761767596366, 16.43878515310709787 ) ) ;
#43083=CARTESIAN_POINT ( 'NONE',  ( 81.98739982517574276, 58.71797656568649870, -0.08682408883346368067 ) ) ;
#43086=CARTESIAN_POINT ( 'NONE',  ( 74.84842711207834043, 61.45602019284894624, 15.25606177542201536 ) ) ;
#43089=CARTESIAN_POINT ( 'NONE',  ( 76.99493330467112173, 57.26266963217694439, 16.17658719691544889 ) ) ;
#43095=CARTESIAN_POINT ( 'NONE',  ( 73.51948839908328637, 69.73627507762921596, -9.361350578256052657 ) ) ;
#43098=CARTESIAN_POINT ( 'NONE',  ( 70.10062891805684160, 70.95873945766187774, 2.129561960066722826 ) ) ;
#43101=CARTESIAN_POINT ( 'NONE',  ( 20.25339421822757302, 23.64441083166260782, -10.00000000000000533 ) ) ;
#43116=CARTESIAN_POINT ( 'NONE',  ( 17.41189581114303309, 28.79103043416549212, 8.090169943749478065 ) ) ;
#43117=CARTESIAN_POINT ( 'NONE',  ( 85.60773205244574058, 48.97959825543787105, 12.21184514131274312 ) ) ;
#43122=CARTESIAN_POINT ( 'NONE',  ( 73.78934571132764120, 55.49050343092449111, -16.58731856350070899 ) ) ;
#43125=CARTESIAN_POINT ( 'NONE',  ( 74.95743781794847393, 67.19740583228991682, 12.53491114478569912 ) ) ;
#43135=ADVANCED_FACE ( 'NONE', ( #35954 ), #91690, .T. ) ;
#43136=CARTESIAN_POINT ( 'NONE',  ( 78.98991491668435572, 60.09931805977702624, 16.11723901038370244 ) ) ;
#43137=CARTESIAN_POINT ( 'NONE',  ( 36.57256041901661803, 33.06628583063844928, -9.188101187500006262 ) ) ;
#43138=CARTESIAN_POINT ( 'NONE',  ( 27.35777070392073185, 16.76426979415090557, 3.090169943749476733 ) ) ;
#43144=CARTESIAN_POINT ( 'NONE',  ( 17.90851666933368236, 18.84335787977762777, 9.188101187500006262 ) ) ;
#43145=CARTESIAN_POINT ( 'NONE',  ( 71.57943482431291216, 72.41997303871664826, 0.9858917062509064966 ) ) ;
#43146=CARTESIAN_POINT ( 'NONE',  ( 82.33565291927013163, 54.25759526660485932, 15.62409434222757376 ) ) ;
#43148=DIRECTION ( 'NONE',  ( 0.4827766168686586368, 0.5834231310750571664, 0.6531035050674810494 ) ) ;
#43150=VECTOR ( 'NONE', #18938, 1000.000000000000000 ) ;
#43158=CARTESIAN_POINT ( 'NONE',  ( 66.61276649528306848, 68.27696284464261112, 4.555325784153476221 ) ) ;
#43167=CARTESIAN_POINT ( 'NONE',  ( 80.28516836418320679, 58.07801345963574846, 16.26295356561165661 ) ) ;
#43170=CARTESIAN_POINT ( 'NONE',  ( 78.19646929978586058, 61.02229919570467587, -15.90908970393073396 ) ) ;
#43171=CARTESIAN_POINT ( 'NONE',  ( 88.45958475239287111, 43.85926912372239883, -0.5941283661710258235 ) ) ;
#43173=CARTESIAN_POINT ( 'NONE',  ( 80.77763420391843852, 43.45617620844090112, 9.404609412801525181 ) ) ;
#43178=CARTESIAN_POINT ( 'NONE',  ( 73.41744195450526433, 58.55286001146748731, 15.72156431111986663 ) ) ;
#43189=VERTEX_POINT ( 'NONE', #20278 ) ;
#43190=CARTESIAN_POINT ( 'NONE',  ( 73.05912352472130067, 69.60491006942920933, 9.219028434792550186 ) ) ;
#43193=CARTESIAN_POINT ( 'NONE',  ( 11.06379537489605802, 28.16126292948894161, -6.180339887498951690 ) ) ;
#43198=CARTESIAN_POINT ( 'NONE',  ( 66.52392041426838887, 68.84470833973988135, -4.415679280545953489 ) ) ;
#43221=ADVANCED_FACE ( 'NONE', ( #459 ), #95886, .T. ) ;
#43232=VERTEX_POINT ( 'NONE', #2474 ) ;
#43233=CARTESIAN_POINT ( 'NONE',  ( 74.17419530692131957, 68.61376803465689989, 11.49684454571890591 ) ) ;
#43238=CARTESIAN_POINT ( 'NONE',  ( 3.606438777009930430, 25.58029201028039523, 1.583844403245363353 ) ) ;
#43244=VERTEX_POINT ( 'NONE', #10064 ) ;
#43253=CARTESIAN_POINT ( 'NONE',  ( 73.67129923898167476, 69.53774399045309451, 9.705214532217949497 ) ) ;
#43256=CARTESIAN_POINT ( 'NONE',  ( 72.48613895716145805, 57.45971281110428919, 15.82031199903085472 ) ) ;
#43257=CARTESIAN_POINT ( 'NONE',  ( 68.85652538089030372, 67.72390236607947145, 8.290076536751538328 ) ) ;
#43262=CARTESIAN_POINT ( 'NONE',  ( 84.85648000362951393, 46.82103691607230900, 11.23615365138597788 ) ) ;
#43264=CARTESIAN_POINT ( 'NONE',  ( 18.86656744736070124, 32.93396525600390845, 2.839279412974139660 ) ) ;
#43275=DIRECTION ( 'NONE',  ( -0.4330127018922203530, 0.7500000000000046629, 0.4999999999999919509 ) ) ;
#43277=CARTESIAN_POINT ( 'NONE',  ( 81.68773053310077614, 55.22504345363421407, -15.91572386494825508 ) ) ;
#43283=CARTESIAN_POINT ( 'NONE',  ( 84.92204705518831531, 44.20989360438028370, 7.136245731002743398 ) ) ;
#43286=CARTESIAN_POINT ( 'NONE',  ( 69.89065256384225222, 70.96540875737194654, 1.221569532770550914 ) ) ;
#43290=CARTESIAN_POINT ( 'NONE',  ( 1.988115337714555064, 24.08080186712590276, -3.090169943749475845 ) ) ;
#43294=CARTESIAN_POINT ( 'NONE',  ( 86.43879872498249028, 47.50144577818752367, -11.01113278173269627 ) ) ;
#43301=CARTESIAN_POINT ( 'NONE',  ( 75.35759910184178523, 53.42226962351871578, 16.03358801198504224 ) ) ;
#43306=CARTESIAN_POINT ( 'NONE',  ( 81.43089153347496278, 41.93548625179531797, -7.634709731026679158 ) ) ;
#43320=CARTESIAN_POINT ( 'NONE',  ( 81.90780539245514547, 41.08307300545056506, 3.607455742197654303 ) ) ;
#43321=CARTESIAN_POINT ( 'NONE',  ( 80.71947726780676646, 43.20949036903483176, -9.150662618319326924 ) ) ;
#43325=LINE ( 'NONE', #57028, #8074 ) ;
#43326=CARTESIAN_POINT ( 'NONE',  ( 27.10026011071931151, 20.81029122506295437, 8.090169943749479842 ) ) ;
#43330=CARTESIAN_POINT ( 'NONE',  ( 76.21559454301076642, 57.26398044443746471, 16.12431043198527902 ) ) ;
#43331=CARTESIAN_POINT ( 'NONE',  ( 4.512196379633642174, 24.64646525600387861, -2.839279412974133887 ) ) ;
#43339=CARTESIAN_POINT ( 'NONE',  ( 83.30032458682389063, 49.65944847437223331, -13.96189754096489288 ) ) ;
#43340=CARTESIAN_POINT ( 'NONE',  ( 67.86860378221429357, 65.58690806574966814, -10.91583492536020472 ) ) ;
#43341=CARTESIAN_POINT ( 'NONE',  ( 84.04231234028014796, 41.83853045254244307, 0.6551603079148081710 ) ) ;
#43342=CARTESIAN_POINT ( 'NONE',  ( 88.39405946958876825, 44.08409158760228053, -2.802556091636618341 ) ) ;
#43345=CARTESIAN_POINT ( 'NONE',  ( 66.45390109022466163, 68.94435773741150797, 0.02467235416223488229 ) ) ;
#43351=CARTESIAN_POINT ( 'NONE',  ( 81.61276851515816588, 44.80639225569448314, -10.39255593558327462 ) ) ;
#43355=CARTESIAN_POINT ( 'NONE',  ( 88.26049611827410502, 43.94792280741877732, 2.484900765466349082 ) ) ;
#43360=CARTESIAN_POINT ( 'NONE',  ( 80.04426707012592601, 58.13730958922976555, 16.26787960027916569 ) ) ;
#43361=CARTESIAN_POINT ( 'NONE',  ( 85.76519349052995267, 48.62301808087004673, -11.86379414718568093 ) ) ;
#43370=CARTESIAN_POINT ( 'NONE',  ( 87.66150902149263402, 44.36974732289110790, -4.043329145106127065 ) ) ;
#43372=CARTESIAN_POINT ( 'NONE',  ( 78.76277686495221531, 54.87806250904672112, 16.03155917534425967 ) ) ;
#43375=CARTESIAN_POINT ( 'NONE',  ( 75.99421521153445269, 51.38408235280206071, 15.66610209674420062 ) ) ;
#43379=CARTESIAN_POINT ( 'NONE',  ( 85.04850917506151120, 49.90949791588273143, 13.51477744872044262 ) ) ;
#43384=DIRECTION ( 'NONE',  ( -0.8660254037844379305, -0.5000000000000014433, -0.000000000000000000 ) ) ;
#43387=CARTESIAN_POINT ( 'NONE',  ( 5.211622267866312441, 23.98502408145590081, -5.678558825948271327 ) ) ;
#43391=CARTESIAN_POINT ( 'NONE',  ( 86.44709368921655823, 43.17377345843237180, -0.6848223079830935145 ) ) ;
#43395=CARTESIAN_POINT ( 'NONE',  ( 33.43441462842632461, 34.70171378149922248, -9.188101187500004485 ) ) ;
#43399=CARTESIAN_POINT ( 'NONE',  ( 25.85429974905589745, 23.43085787977764056, -9.188101187500008038 ) ) ;
#43404=CARTESIAN_POINT ( 'NONE',  ( 70.95991511397710383, 61.13971250865433404, 15.00408310107609644 ) ) ;
#43408=CARTESIAN_POINT ( 'NONE',  ( 87.35668359673078953, 44.84080960044052233, -6.701380392922977158 ) ) ;
#43411=CARTESIAN_POINT ( 'NONE',  ( 75.34529629774760906, 53.42024133556077459, 16.03399186784752217 ) ) ;
#43418=CARTESIAN_POINT ( 'NONE',  ( 86.39765121943966619, 44.20258484113508501, 5.509774257601782743 ) ) ;
#43420=CARTESIAN_POINT ( 'NONE',  ( 77.16771381044527800, 63.58369421181528480, -15.05433088148817511 ) ) ;
#43429=VECTOR ( 'NONE', #27378, 1000.000000000000227 ) ;
#43430=CARTESIAN_POINT ( 'NONE',  ( 30.66616357392367220, 39.74646525600392977, 2.839279412974139660 ) ) ;
#43431=CARTESIAN_POINT ( 'NONE',  ( 74.81245076906620284, 60.05495312879037328, -15.59845400761551559 ) ) ;
#43434=CARTESIAN_POINT ( 'NONE',  ( 87.14368005316970311, 45.34715801825632298, 7.070389941925012245 ) ) ;
#43437=PLANE ( 'NONE',  #83290 ) ;
#43439=CARTESIAN_POINT ( 'NONE',  ( 68.34553620988224054, 65.65657992573082424, 10.39144713415675270 ) ) ;
#43441=CARTESIAN_POINT ( 'NONE',  ( 85.54016331024442366, 48.30264805437344933, -11.71386965376238365 ) ) ;
#43444=CARTESIAN_POINT ( 'NONE',  ( 82.08531156464800915, 40.77555587586176955, 1.302602283300562824 ) ) ;
#43448=CARTESIAN_POINT ( 'NONE',  ( 88.32078559155080200, 44.16791947909882765, 0.3596700509409204716 ) ) ;
#43455=EDGE_LOOP ( 'NONE', ( #39663, #11211, #57891, #78899, #60593 ) ) ;
#43456=CARTESIAN_POINT ( 'NONE',  ( 86.95562746175168911, 45.78762616370607930, -8.653322509500107174 ) ) ;
#43466=CARTESIAN_POINT ( 'NONE',  ( 27.69565257936902469, 21.15404122711134605, 8.090169943749479842 ) ) ;
#43467=CARTESIAN_POINT ( 'NONE',  ( 81.82192856674927839, 43.76204572152891359, 9.071121036995474896 ) ) ;
#43473=CARTESIAN_POINT ( 'NONE',  ( 81.92774799985024003, 49.39617170011497649, 13.74847781650752765 ) ) ;
#43481=CARTESIAN_POINT ( 'NONE',  ( 67.38373687966300452, 69.45179799017431321, -1.105247961781016919 ) ) ;
#43484=CARTESIAN_POINT ( 'NONE',  ( 14.28567607145357421, 31.18080186712592550, 3.090169943749475401 ) ) ;
#43485=CARTESIAN_POINT ( 'NONE',  ( 77.64328263671511365, 61.91708053827061065, 15.64711088792926041 ) ) ;
#43490=EDGE_CURVE ( 'NONE', #30622, #44213, #70226, .T. ) ;
#43495=ADVANCED_FACE ( 'NONE', ( #77340, #62616 ), #69729, .T. ) ;
#43496=CARTESIAN_POINT ( 'NONE',  ( 39.83529790697233608, 25.12755873383629179, -6.180339887498949025 ) ) ;
#43497=CARTESIAN_POINT ( 'NONE',  ( 79.77742007133535651, 56.10585682640231653, -16.52583479100570685 ) ) ;
#43499=CARTESIAN_POINT ( 'NONE',  ( 87.27919387765231818, 43.83186819549126056, -2.650470388296021440 ) ) ;
#43507=CARTESIAN_POINT ( 'NONE',  ( 87.10076192357585967, 46.06401709681040302, 8.920816893773267253 ) ) ;
#43510=CARTESIAN_POINT ( 'NONE',  ( 71.65515660876562265, 72.43366598492664821, -1.354044368658560815 ) ) ;
#43515=CARTESIAN_POINT ( 'NONE',  ( 5.010160986809694350, 24.93396525600388003, 2.839279412974139660 ) ) ;
#43530=ORIENTED_EDGE ( 'NONE', *, *, #34630, .F. ) ;
#43538=CARTESIAN_POINT ( 'NONE',  ( 26.79248755578709762, 33.65586893147757763, -7.433330006724137462 ) ) ;
#43540=CARTESIAN_POINT ( 'NONE',  ( 86.20715737948781054, 46.96926287157581470, -10.06788908585955511 ) ) ;
#43542=ORIENTED_EDGE ( 'NONE', *, *, #48827, .T. ) ;
#43543=CARTESIAN_POINT ( 'NONE',  ( 11.06573324809563807, 29.49540643055186351, 3.479690158560446702E-15 ) ) ;
#43545=CARTESIAN_POINT ( 'NONE',  ( 67.81490795777737901, 69.52803666604617661, -2.566435835120146169 ) ) ;
#43559=CARTESIAN_POINT ( 'NONE',  ( 66.09459138788395194, 68.54660210817900179, -2.305970830781039815 ) ) ;
#43567=DIRECTION ( 'NONE',  ( 0.5000000000000013323, -0.8660254037844378194, 0.000000000000000000 ) ) ;
#43584=PLANE ( 'NONE',  #88516 ) ;
#43591=CARTESIAN_POINT ( 'NONE',  ( 80.21278584107015774, 53.44521250575849791, 16.08036484325488757 ) ) ;
#43596=VERTEX_POINT ( 'NONE', #97993 ) ;
#43598=CARTESIAN_POINT ( 'NONE',  ( 74.67000616351420206, 66.81477949400924388, -13.12245706047550797 ) ) ;
#43602=CARTESIAN_POINT ( 'NONE',  ( 73.71376407998293701, 56.08882236293795387, 16.08428922147598428 ) ) ;
#43605=CARTESIAN_POINT ( 'NONE',  ( 77.54335625564391421, 61.27816323999952175, 15.77127415614125461 ) ) ;
#43607=CARTESIAN_POINT ( 'NONE',  ( 72.53840899933517505, 71.27365409391698847, -6.036301325323600864 ) ) ;
#43609=CARTESIAN_POINT ( 'NONE',  ( 73.66740156979760457, 69.66397881967726846, -9.561189449020471187 ) ) ;
#43615=CARTESIAN_POINT ( 'NONE',  ( 21.61359102238895957, 12.28848085856230732, 1.475505719884397138E-15 ) ) ;
#43620=CARTESIAN_POINT ( 'NONE',  ( 72.28313422013535217, 71.96753738583048232, -3.711430182928289856 ) ) ;
#43626=CARTESIAN_POINT ( 'NONE',  ( 66.82592210189895354, 67.33918606646240335, -6.964996463769947965 ) ) ;
#43631=CARTESIAN_POINT ( 'NONE',  ( 27.61987535298997187, 21.11029122506295508, -8.090169943749478065 ) ) ;
#43632=CARTESIAN_POINT ( 'NONE',  ( 85.43645318413936707, 48.61927365843763482, 12.47466632846418122 ) ) ;
#43637=CARTESIAN_POINT ( 'NONE',  ( 75.25170673533752108, 66.73598490943447814, 12.94887977284632896 ) ) ;
#43648=CARTESIAN_POINT ( 'NONE',  ( 34.56506555475243658, 38.14336893147758900, 7.433330006724141015 ) ) ;
#43651=CARTESIAN_POINT ( 'NONE',  ( 25.38349897777161601, 16.78380873178787169, -6.180339887498949025 ) ) ;
#43655=CARTESIAN_POINT ( 'NONE',  ( 11.06573324809563807, 29.49540643055186351, 3.479690158560446702E-15 ) ) ;
#43656=CARTESIAN_POINT ( 'NONE',  ( 71.61987371496263677, 72.44464069648768145, 0.9664813023029263928 ) ) ;
#43671=ORIENTED_EDGE ( 'NONE', *, *, #69535, .T. ) ;
#43679=CARTESIAN_POINT ( 'NONE',  ( 80.38386138148599969, 57.79680026592914999, 16.59996232260768778 ) ) ;
#43683=ADVANCED_FACE ( 'NONE', ( #52864 ), #45265, .T. ) ;
#43696=ORIENTED_EDGE ( 'NONE', *, *, #48827, .F. ) ;
#43699=CARTESIAN_POINT ( 'NONE',  ( 82.98423510826575011, 53.52344736239029288, 15.67380116644083721 ) ) ;
#43706=CARTESIAN_POINT ( 'NONE',  ( 81.37674444193763179, 55.19836804271280783, -15.94010240901345199 ) ) ;
#43707=CARTESIAN_POINT ( 'NONE',  ( 38.01218019840322881, 27.11029122506296929, -8.090169943749478065 ) ) ;
#43713=CARTESIAN_POINT ( 'NONE',  ( 76.98069296933027772, 53.91054578136119346, -16.01903993249421632 ) ) ;
#43717=VECTOR ( 'NONE', #42233, 1000.000000000000114 ) ;
#43718=EDGE_LOOP ( 'NONE', ( #65056, #29176, #19054, #76539 ) ) ;
#43728=CARTESIAN_POINT ( 'NONE',  ( 84.56517416216006211, 50.64586678990350777, 13.69612687457570033 ) ) ;
#43735=CARTESIAN_POINT ( 'NONE',  ( 74.41897651308048012, 68.01641561303326000, -11.65844777088098461 ) ) ;
#43749=CARTESIAN_POINT ( 'NONE',  ( 13.50136424336972141, 8.764269794150880699, 3.090169943749476733 ) ) ;
#43750=CARTESIAN_POINT ( 'NONE',  ( 79.11275361910446691, 46.11146926033848104, 13.27945046499836579 ) ) ;
#43751=CARTESIAN_POINT ( 'NONE',  ( 71.64977493859507263, 59.13526382602540821, -15.32350604844225295 ) ) ;
#43752=CARTESIAN_POINT ( 'NONE',  ( 73.67278091869266632, 69.61283722901053750, 9.621970401190987232 ) ) ;
#43756=CARTESIAN_POINT ( 'NONE',  ( 70.86977990947116268, 70.80167083835577557, 4.702927032916670136 ) ) ;
#43759=B_SPLINE_CURVE_WITH_KNOTS ( 'NONE', 3,
 ( #20724, #19731, #12627, #43497, #66801, #74927, #67299, #74439, #82058, #58686, #91143, #37391, #97728, #75420, #35405, #5509 ),
 .UNSPECIFIED., .F., .F.,
 ( 4, 1, 2, 2, 2, 1, 2, 2, 4 ),
 ( 0.000000000000000000, 0.1249999999999976685, 0.1874999999999985012, 0.2499999999999993339, 0.5000000000000033307, 0.6250000000000053291, 0.6875000000000044409, 0.7500000000000035527, 1.000000000000000000 ),
 .UNSPECIFIED. ) ;
#43763=CARTESIAN_POINT ( 'NONE',  ( 80.07812099633126479, 57.44764983040322903, -16.59488970948942921 ) ) ;
#43765=CARTESIAN_POINT ( 'NONE',  ( 27.91230638117223606, 28.06628583063842797, -9.188101187500006262 ) ) ;
#43767=CARTESIAN_POINT ( 'NONE',  ( 83.82065378329919270, 51.84410121092205515, -14.88618515114630370 ) ) ;
#43770=CARTESIAN_POINT ( 'NONE',  ( 75.27726335905293809, 66.87231400452490959, 13.31561030640130738 ) ) ;
#43771=CARTESIAN_POINT ( 'NONE',  ( 68.53512761445865920, 64.30306519794643805, 11.73731604961160180 ) ) ;
#43775=CARTESIAN_POINT ( 'NONE',  ( 70.93378986505813089, 67.06125297378586936, -11.22077736235704926 ) ) ;
#43777=CARTESIAN_POINT ( 'NONE',  ( 9.573022157908470220, 14.03085787977760823, 9.188101187500006262 ) ) ;
#43779=PLANE ( 'NONE',  #81345 ) ;
#43781=B_SPLINE_CURVE_WITH_KNOTS ( 'NONE', 3,
 ( #89936, #34694, #66101, #73710, #65595, #36182, #96545, #97049, #27617, #20014, #50891, #81839, #88980, #88469, #12416, #43782, #27116, #94667, #19534, #20514, #57999, #12923, #74727, #49903, #80861, #67087, #50396, #43283, #35699, #74228, #11434, #4293, #98010, #97525, #28095, #58966, #73220, #81350, #28588, #51390, #3813, #82355, #86589, #48020, #9551, #11920 ),
 .UNSPECIFIED., .F., .F.,
 ( 4, 1, 1, 1, 2, 2, 1, 1, 1, 2, 2, 1, 1, 2, 2, 1, 1, 2, 2, 1, 1, 2, 2, 1, 2, 2, 1, 2, 2, 4 ),
 ( 0.000000000000000000, 0.06249999999999292233, 0.09374999999998942513, 0.1093749999999886896, 0.1171874999999882455, 0.1249999999999877875, 0.1874999999999923672, 0.2187499999999937550, 0.2343749999999936162, 0.2421874999999925615, 0.2499999999999915068, 0.3124999999999931721, 0.3437499999999940603, 0.3593749999999954481, 0.3749999999999968359, 0.4374999999999996114, 0.4687499999999996114, 0.4843749999999998335, 0.5000000000000000000, 0.5624999999999985567, 0.5937499999999972244, 0.6093749999999973355, 0.6249999999999974465, 0.6874999999999983347, 0.7187499999999987788, 0.7499999999999992228, 0.8125000000000003331, 0.8437500000000008882, 0.8750000000000014433, 1.000000000000000000 ),
 .UNSPECIFIED. ) ;
#43782=CARTESIAN_POINT ( 'NONE',  ( 83.81822528977980369, 42.74170432803968112, 5.348213412007799761 ) ) ;
#43788=CARTESIAN_POINT ( 'NONE',  ( 74.23555041547365363, 68.49601928387087924, -11.11897725275786719 ) ) ;
#43791=CARTESIAN_POINT ( 'NONE',  ( 19.29290913472606661, 12.10801979619928126, 3.090169943749476733 ) ) ;
#43792=CARTESIAN_POINT ( 'NONE',  ( 84.31969329757113485, 49.65246679347950476, 13.61885025447953979 ) ) ;
#43795=CARTESIAN_POINT ( 'NONE',  ( 86.37995054896607883, 46.98508828575033647, -10.52062608394495591 ) ) ;
#43807=CARTESIAN_POINT ( 'NONE',  ( 73.34867049892106650, 70.14346970443526175, -9.354907352444854496 ) ) ;
#43816=CARTESIAN_POINT ( 'NONE',  ( 81.94787918575768515, 52.94560862287604408, 15.29677040454687642 ) ) ;
#43822=CARTESIAN_POINT ( 'NONE',  ( 87.62133583293774564, 45.31115884160843876, -7.293173845241961217 ) ) ;
#43823=DIRECTION ( 'NONE',  ( 0.4972609476841349796, -0.8612812260087746585, 0.1045284632676570652 ) ) ;
#43825=CARTESIAN_POINT ( 'NONE',  ( 72.02695394113958116, 68.29673134482877117, -9.986728363011483367 ) ) ;
#43828=CARTESIAN_POINT ( 'NONE',  ( 76.46110298587262832, 58.51621405362541850, 16.04222249715220983 ) ) ;
#43829=CARTESIAN_POINT ( 'NONE',  ( 4.886862741447147940, 23.79752408145590081, -5.678558825948271327 ) ) ;
#43836=CARTESIAN_POINT ( 'NONE',  ( 78.12823040285628906, 47.68785961753161473, -13.94170588958538026 ) ) ;
#43842=CARTESIAN_POINT ( 'NONE',  ( 88.44266034405603705, 44.03949081389492903, -2.406584733330055847 ) ) ;
#43845=CARTESIAN_POINT ( 'NONE',  ( 71.04498658471177919, 63.38740358822698795, -13.40332908134212175 ) ) ;
#43848=CARTESIAN_POINT ( 'NONE',  ( 86.81641918289878390, 45.77657501471897916, -8.750901752256119437 ) ) ;
#43853=CARTESIAN_POINT ( 'NONE',  ( 88.27656095359526489, 44.31834822599916635, 2.178649859666209387 ) ) ;
#43855=ORIENTED_EDGE ( 'NONE', *, *, #55293, .F. ) ;
#43858=CARTESIAN_POINT ( 'NONE',  ( 80.56229873119019658, 57.64365382000625715, 16.23737920899276688 ) ) ;
#43859=DIRECTION ( 'NONE',  ( -0.1039558454088829048, 0.1800568059919617214, 0.9781476007338041345 ) ) ;
#43863=CARTESIAN_POINT ( 'NONE',  ( 84.52717288222906689, 47.01816712101242501, 11.03627013421178304 ) ) ;
#43869=CARTESIAN_POINT ( 'NONE',  ( 78.17977472700404462, 52.13989681908228135, 15.57239507869588913 ) ) ;
#43872=CARTESIAN_POINT ( 'NONE',  ( 69.81582973455006425, 63.14295414310246457, -13.67321376818634882 ) ) ;
#43876=CARTESIAN_POINT ( 'NONE',  ( 84.39448865303761238, 50.06170295690048988, 13.83095091856771219 ) ) ;
#43878=EDGE_CURVE ( 'NONE', #59778, #6177, #46782, .T. ) ;
#43883=CARTESIAN_POINT ( 'NONE',  ( 81.85856577761916242, 58.94112368179924033, 0.4414737964294648265 ) ) ;
#43887=CARTESIAN_POINT ( 'NONE',  ( 9.725772901699041739, 17.56628583063838889, 9.188101187500006262 ) ) ;
#43894=CARTESIAN_POINT ( 'NONE',  ( 40.31210609084968866, 28.98920272979929535, 7.433330006724137462 ) ) ;
#43896=CARTESIAN_POINT ( 'NONE',  ( 86.47331868612941719, 47.35852300529328573, 10.29769560459374667 ) ) ;
#43898=CARTESIAN_POINT ( 'NONE',  ( 26.73894555032740783, 17.29860640527292759, -2.839279412974138328 ) ) ;
#43903=CARTESIAN_POINT ( 'NONE',  ( 70.35832557788559427, 61.08735884527625615, 14.88019646618581149 ) ) ;
#43906=CARTESIAN_POINT ( 'NONE',  ( 72.57482212583268222, 71.55826866971187883, 5.407793347878283363 ) ) ;
#43907=CARTESIAN_POINT ( 'NONE',  ( 87.37223321024185907, 44.84069173413745091, -6.683519980512460101 ) ) ;
#43909=CARTESIAN_POINT ( 'NONE',  ( 69.40201478176561523, 62.74293981228880313, 13.19403646481873338 ) ) ;
#43910=ORIENTED_EDGE ( 'NONE', *, *, #55892, .T. ) ;
#43914=CARTESIAN_POINT ( 'NONE',  ( 86.17717080636731453, 43.91654295222171811, 5.091268916963881175 ) ) ;
#43921=CARTESIAN_POINT ( 'NONE',  ( 86.54822389131679472, 42.74345947012793090, -2.172736160200603931E-06 ) ) ;
#43923=CARTESIAN_POINT ( 'NONE',  ( 40.27059248445925732, 25.11110640527295601, -2.839279412974138328 ) ) ;
#43930=CARTESIAN_POINT ( 'NONE',  ( 5.530962353892124206, 15.14441083166257584, 0.000000000000000000 ) ) ;
#43936=CARTESIAN_POINT ( 'NONE',  ( 82.14221379916808985, 40.79694460358976471, 1.153306960283028149 ) ) ;
#43938=CARTESIAN_POINT ( 'NONE',  ( 77.30329167060655493, 63.33344332055067127, -15.17436694516359097 ) ) ;
#43946=ORIENTED_EDGE ( 'NONE', *, *, #45220, .F. ) ;
#43948=CARTESIAN_POINT ( 'NONE',  ( 71.55103965959418133, 59.07988815573101959, 15.32428709606925921 ) ) ;
#43960=CARTESIAN_POINT ( 'NONE',  ( 83.55986682201206861, 47.94177803495283996, 12.26456158152270071 ) ) ;
#43962=CARTESIAN_POINT ( 'NONE',  ( 69.59273039108451542, 62.48764762269725992, -13.40792685205324908 ) ) ;
#43974=CARTESIAN_POINT ( 'NONE',  ( 68.79206230443567449, 70.05501897347022577, -2.776141514423435375 ) ) ;
#43979=FACE_OUTER_BOUND ( 'NONE', #34624, .T. ) ;
#43982=DIRECTION ( 'NONE',  ( -0.5000000000000013323, 0.8660254037844379305, 0.000000000000000000 ) ) ;
#43983=CARTESIAN_POINT ( 'NONE',  ( 13.83924611881801958, 13.15404122711132118, 8.090169943749479842 ) ) ;
#43984=CARTESIAN_POINT ( 'NONE',  ( 33.16502987395432456, 42.08080186712595605, -3.090169943749475845 ) ) ;
#43987=CARTESIAN_POINT ( 'NONE',  ( 72.14066163544119092, 72.07444104301772825, 2.939506046423011831 ) ) ;
#43993=CARTESIAN_POINT ( 'NONE',  ( 77.68426462998779414, 51.26866757787253448, -15.41241789615859936 ) ) ;
#43996=CARTESIAN_POINT ( 'NONE',  ( 17.33597792084844258, 30.98502408145592213, -5.678558825948271327 ) ) ;
#43999=CARTESIAN_POINT ( 'NONE',  ( 36.44916501977947831, 42.81751292744058901, -6.180339887498951690 ) ) ;
#44001=CARTESIAN_POINT ( 'NONE',  ( 76.32091777638089525, 59.04525850092294093, -16.41165238920815383 ) ) ;
#44004=CARTESIAN_POINT ( 'NONE',  ( 71.84119047025625093, 67.74597162956264640, -10.41150127685602911 ) ) ;
#44006=CARTESIAN_POINT ( 'NONE',  ( 82.07091975778192250, 41.09839960039168005, 3.280828371301158342 ) ) ;
#44009=CARTESIAN_POINT ( 'NONE',  ( 80.51198428680065433, 43.68793065238016737, 9.861687463089015893 ) ) ;
#44010=EDGE_LOOP ( 'NONE', ( #9110, #22758, #91929, #40311 ) ) ;
#44015=DIRECTION ( 'NONE',  ( 0.2633726137851623572, 0.9634420117996734811, -0.04913609882122786654 ) ) ;
#44022=CARTESIAN_POINT ( 'NONE',  ( 31.05164846989082506, 29.87878583063843507, -9.188101187500006262 ) ) ;
#44029=CARTESIAN_POINT ( 'NONE',  ( 19.94606896448370392, 26.91421378149918908, 9.188101187500008038 ) ) ;
#44030=CARTESIAN_POINT ( 'NONE',  ( 76.42898847865113510, 62.85965002459411011, 15.15259878098221691 ) ) ;
#44032=LINE ( 'NONE', #3579, #56986 ) ;
#44037=ORIENTED_EDGE ( 'NONE', *, *, #67667, .F. ) ;
#44041=CARTESIAN_POINT ( 'NONE',  ( 70.65128213755779996, 71.32262211326366241, -4.112991392911065525 ) ) ;
#44042=CARTESIAN_POINT ( 'NONE',  ( 65.83005313167186046, 68.93055679263270008, -2.414931814313005631 ) ) ;
#44044=DIRECTION ( 'NONE',  ( -0.4996954135095461047, 0.8654978445076770832, -0.03489949670251103753 ) ) ;
#44058=CARTESIAN_POINT ( 'NONE',  ( 75.32733312582141139, 66.71342752998261005, -13.00712609038388479 ) ) ;
#44064=CARTESIAN_POINT ( 'NONE',  ( 87.65336964024139377, 45.10687245489101116, 6.884500160062612117 ) ) ;
#44066=ADVANCED_FACE ( 'NONE', ( #66439 ), #34372, .T. ) ;
#44069=CARTESIAN_POINT ( 'NONE',  ( 88.22000632671873177, 44.27423112938744509, 4.003506518527982116 ) ) ;
#44071=CARTESIAN_POINT ( 'NONE',  ( 72.58391486703608564, 69.83303746380133248, -8.484543846056432415 ) ) ;
#44072=ADVANCED_FACE ( 'NONE', ( #21337 ), #84874, .T. ) ;
#44073=CARTESIAN_POINT ( 'NONE',  ( 76.15417792458961799, 51.07502231937492354, -16.06867589080808401 ) ) ;
#44075=DIRECTION ( 'NONE',  ( -0.8660254037844378194, -0.5000000000000014433, -0.000000000000000000 ) ) ;
#44077=LINE ( 'NONE', #75016, #14443 ) ;
#44082=CARTESIAN_POINT ( 'NONE',  ( 81.21903618153429250, 44.31068850558377648, -10.11524766067121384 ) ) ;
#44083=CARTESIAN_POINT ( 'NONE',  ( 85.08339545359741862, 43.17538514247008408, 4.622258380740561279 ) ) ;
#44085=CARTESIAN_POINT ( 'NONE',  ( 73.05937878676877517, 70.59762130387636603, 7.796525793287967687 ) ) ;
#44089=CARTESIAN_POINT ( 'NONE',  ( 77.24725012743233776, 58.87555087126124675, 16.09217688641884081 ) ) ;
#44092=CARTESIAN_POINT ( 'NONE',  ( 81.23969665105722981, 52.59010616956271633, 15.26830288788405987 ) ) ;
#44094=B_SPLINE_CURVE_WITH_KNOTS ( 'NONE', 3,
 ( #66110, #89946, #20523, #4303, #59480, #67098, #74737, #5316, #97058, #97534 ),
 .UNSPECIFIED., .F., .F.,
 ( 4, 2, 2, 2, 4 ),
 ( 0.000000000000000000, 0.0002622400424273354179, 0.0005244800848546708359, 0.0007867201272820061996, 0.001048960169709341672 ),
 .UNSPECIFIED. ) ;
#44096=CARTESIAN_POINT ( 'NONE',  ( 70.61771366156216345, 71.37294255471428528, 1.331711565741383385 ) ) ;
#44104=CARTESIAN_POINT ( 'NONE',  ( 25.63248128490755562, 16.92755873383626763, 6.180339887498953466 ) ) ;
#44107=LINE ( 'NONE', #45116, #6443 ) ;
#44114=ADVANCED_FACE ( 'NONE', ( #32428 ), #49731, .T. ) ;
#44116=CARTESIAN_POINT ( 'NONE',  ( 66.72164201642236492, 67.46051856063240848, -6.617423282627738601 ) ) ;
#44120=CARTESIAN_POINT ( 'NONE',  ( 29.16343140518078414, 25.03677371833803278, 10.00000000000000533 ) ) ;
#44121=CARTESIAN_POINT ( 'NONE',  ( 71.96639307748559133, 71.49757472301890004, -5.734781593071435424 ) ) ;
#44130=CARTESIAN_POINT ( 'NONE',  ( 75.11332179147987631, 67.11795023670394755, 12.64955091210966742 ) ) ;
#44132=B_SPLINE_CURVE_WITH_KNOTS ( 'NONE', 3,
 ( #10795, #25999, #69699, #18395, #22611, #38290, #76804, #55850, #33591, #40666, #307, #80227, #84940, #61091, #69200, #53497, #30209, #56373, #87371, #63977, #100126, #86845, #9806, #72100, #56870, #92062, #84451, #61594, #49289, #92545, #17900 ),
 .UNSPECIFIED., .F., .F.,
 ( 4, 3, 3, 3, 3, 3, 3, 3, 3, 3, 4 ),
 ( 0.000000000000000000, 0.1333490885032359574, 0.3007194338854340954, 0.4699862290245186980, 0.5844252810809413834, 0.6686540514502794519, 0.7354980260655689106, 0.8028463152565833427, 0.8633854507757432462, 0.9437142632667659958, 1.000000000000000000 ),
 .UNSPECIFIED. ) ;
#44139=CARTESIAN_POINT ( 'NONE',  ( 43.68478726420265446, 28.14754757982094802, -5.678558825948276656 ) ) ;
#44146=CARTESIAN_POINT ( 'NONE',  ( 21.21803360120161486, 14.11110640527291871, -2.839279412974138328 ) ) ;
#44148=CARTESIAN_POINT ( 'NONE',  ( 82.53276180672601470, 53.86864964727561755, 15.84768121842077271 ) ) ;
#44153=CARTESIAN_POINT ( 'NONE',  ( 84.30322693489105745, 45.55207041838918514, -10.27315936618584047 ) ) ;
#44154=CARTESIAN_POINT ( 'NONE',  ( 81.37151302304147293, 42.01189121629286660, 7.817116131920905708 ) ) ;
#44158=CARTESIAN_POINT ( 'NONE',  ( 67.97811056134003138, 69.84350333162846880, 0.3721567129542452390 ) ) ;
#44160=CARTESIAN_POINT ( 'NONE',  ( 81.38228331512368641, 42.18052851754683275, 8.075145019496558163 ) ) ;
#44167=ORIENTED_EDGE ( 'NONE', *, *, #93249, .F. ) ;
#44169=CARTESIAN_POINT ( 'NONE',  ( 80.17693862949111860, 57.41387879531588112, -16.59169664258510224 ) ) ;
#44170=CARTESIAN_POINT ( 'NONE',  ( 76.92873890057782660, 49.89429371730488327, 15.13083596839045519 ) ) ;
#44172=CARTESIAN_POINT ( 'NONE',  ( 87.70375725421425273, 45.31067632575319237, -6.371254654310869014 ) ) ;
#44173=CARTESIAN_POINT ( 'NONE',  ( 80.87722779131914308, 43.49871416137424518, 9.386169728457165462 ) ) ;
#44175=VERTEX_POINT ( 'NONE', #68301 ) ;
#44184=CARTESIAN_POINT ( 'NONE',  ( 38.41907791167486153, 30.38052372038644577, 10.00000000000000533 ) ) ;
#44188=CARTESIAN_POINT ( 'NONE',  ( 75.15191903148871688, 52.97183600646508239, -16.48001256418180915 ) ) ;
#44190=CARTESIAN_POINT ( 'NONE',  ( 82.70618072881376293, 53.83593579450209177, 15.81121719814037796 ) ) ;
#44191=CARTESIAN_POINT ( 'NONE',  ( 17.82296297622643166, 15.45404122711132544, -8.090169943749478065 ) ) ;
#44198=CARTESIAN_POINT ( 'NONE',  ( 76.62092529291432186, 57.15656925429084367, -16.16476570274940983 ) ) ;
#44206=CARTESIAN_POINT ( 'NONE',  ( 80.33594858597078314, 52.74141113690976113, -15.46677329171331650 ) ) ;
#44208=EDGE_CURVE ( 'NONE', #64640, #82637, #51345, .T. ) ;
#44209=CARTESIAN_POINT ( 'NONE',  ( 79.66724985528871628, 45.93439818594649182, 12.94489230522013301 ) ) ;
#44210=EDGE_CURVE ( 'NONE', #9334, #83096, #28660, .T. ) ;
#44213=VERTEX_POINT ( 'NONE', #84552 ) ;
#44221=CARTESIAN_POINT ( 'NONE',  ( 84.25609682182033566, 50.63756641705167283, 13.79401547250049909 ) ) ;
#44228=DIRECTION ( 'NONE',  ( -0.8116583814955280474, -0.01378320505840839941, 0.5839697723396116702 ) ) ;
#44229=ADVANCED_FACE ( 'NONE', ( #24211 ), #63709, .T. ) ;
#44231=CARTESIAN_POINT ( 'NONE',  ( 76.29269770996508271, 51.10466816460979089, 16.05732426857825246 ) ) ;
#44232=CARTESIAN_POINT ( 'NONE',  ( 81.90994132515743331, 41.13720830924725647, -5.473952179386033734 ) ) ;
#44234=( BOUNDED_CURVE ( )  B_SPLINE_CURVE ( 2, ( #33133, #15413, #46308, #57422, #95986, #4224, #95500, #25542, #65528, #79785, #48851, #49834, #87910 ),
 .UNSPECIFIED., .F., .T. ) 
 B_SPLINE_CURVE_WITH_KNOTS ( ( 3, 2, 2, 2, 2, 2, 3 ),
 ( 0.9375000000000000000, 0.9399999999999999467, 0.9449999999999999512, 0.9499999999999999556, 0.9549999999999999600, 0.9599999999999999645, 0.9625000000000000222 ),
 .UNSPECIFIED. ) 
 CURVE ( )  GEOMETRIC_REPRESENTATION_ITEM ( )  RATIONAL_B_SPLINE_CURVE ( ( 0.9755282581475768211, 0.9755282581475768211, 1.000000000000000000, 0.9510565162951535312, 1.000000000000000000, 0.9510565162951535312, 1.000000000000000000, 0.9510565162951535312, 1.000000000000000000, 0.9510565162951535312, 1.000000000000000000, 0.9755282581475761550, 0.9755282581475767101 ) ) 
 REPRESENTATION_ITEM ( '' )  );
#44237=ADVANCED_FACE ( 'NONE', ( #32304 ), #29593, .T. ) ;
#44239=ORIENTED_EDGE ( 'NONE', *, *, #30144, .T. ) ;
#44241=EDGE_CURVE ( 'NONE', #63156, #31137, #9287, .T. ) ;
#44243=CARTESIAN_POINT ( 'NONE',  ( 79.00863916493514694, 47.82580172363768156, -14.30855080123139800 ) ) ;
#44247=CARTESIAN_POINT ( 'NONE',  ( 5.030029564959478172, 25.83705186507751606, 3.090169943749475401 ) ) ;
#44249=CARTESIAN_POINT ( 'NONE',  ( 71.82174548183152751, 58.68616614677867460, -15.47660959074812403 ) ) ;
#44250=CARTESIAN_POINT ( 'NONE',  ( 66.32523131455108967, 68.13125372015736048, -4.501321185133645209 ) ) ;
#44254=CARTESIAN_POINT ( 'NONE',  ( 72.48465836905157289, 57.53796734512142308, 15.80717508320729792 ) ) ;
#44255=CARTESIAN_POINT ( 'NONE',  ( 68.70128421410518627, 67.44681517729620168, 8.549379373129788462 ) ) ;
#44257=( BOUNDED_CURVE ( )  B_SPLINE_CURVE ( 2, ( #95922, #26483, #88334, #58351, #81214, #12277, #65962, #56360, #11300, #34565, #43138, #49769, #74080 ),
 .UNSPECIFIED., .F., .T. ) 
 B_SPLINE_CURVE_WITH_KNOTS ( ( 3, 2, 2, 2, 2, 2, 3 ),
 ( 0.4124999999999999778, 0.4149999999999999800, 0.4199999999999999845, 0.4249999999999999889, 0.4299999999999999933, 0.4349999999999999978, 0.4375000000000000000 ),
 .UNSPECIFIED. ) 
 CURVE ( )  GEOMETRIC_REPRESENTATION_ITEM ( )  RATIONAL_B_SPLINE_CURVE ( ( 0.9755282581475768211, 0.9755282581475768211, 1.000000000000000000, 0.9510565162951535312, 1.000000000000000000, 0.9510565162951535312, 1.000000000000000000, 0.9510565162951535312, 1.000000000000000000, 0.9510565162951535312, 1.000000000000000000, 0.9755282581475768211, 0.9755282581475768211 ) ) 
 REPRESENTATION_ITEM ( '' )  );
#44260=B_SPLINE_CURVE_WITH_KNOTS ( 'NONE', 3,
 ( #3363, #87001, #10442, #17529, #56527, #87515, #72769, #70731, #41315, #65132, #57521, #11462, #19059, #49933, #63130, #94074, #24626, #35228, #42806, #74756, #5336, #97558, #73247, #82874, #3841, #81381, #75245, #36217, #36713, #73739, #58031, #98549, #97078, #4330, #82387, #67119, #98043, #34726, #35730, #11948, #12447, #81870, #89488, #28621, #67620, #52415 ),
 .UNSPECIFIED., .F., .F.,
 ( 4, 1, 1, 1, 2, 2, 1, 1, 1, 2, 2, 1, 1, 2, 2, 1, 1, 2, 2, 1, 1, 2, 2, 1, 2, 2, 1, 2, 2, 4 ),
 ( 0.000000000000000000, 0.06249999999999474032, 0.09374999999999351907, 0.1093749999999934081, 0.1171874999999933387, 0.1249999999999932832, 0.1874999999999907296, 0.2187499999999880373, 0.2343749999999852340, 0.2421874999999834299, 0.2499999999999815703, 0.3124999999999802935, 0.3437499999999796829, 0.3593749999999787947, 0.3749999999999779066, 0.4374999999999760747, 0.4687499999999755751, 0.4843749999999764633, 0.4999999999999773515, 0.5624999999999864553, 0.5937499999999923395, 0.6093749999999942268, 0.6249999999999961142, 0.6874999999999993339, 0.7187500000000019984, 0.7500000000000025535, 0.8125000000000031086, 0.8437500000000033307, 0.8750000000000036637, 1.000000000000000000 ),
 .UNSPECIFIED. ) ;
#44265=CARTESIAN_POINT ( 'NONE',  ( 30.57771352727866443, 18.44966523072494979, -2.296566073217252530E-15 ) ) ;
#44272=CARTESIAN_POINT ( 'NONE',  ( 68.53468829871430046, 64.27236547913501852, 11.76169348210352972 ) ) ;
#44280=CARTESIAN_POINT ( 'NONE',  ( 70.21329603614420023, 69.13614683806369499, 7.337258324027051692 ) ) ;
#44282=CARTESIAN_POINT ( 'NONE',  ( 72.04176329605472517, 72.30724862116409213, 0.7207730510373432375 ) ) ;
#44289=CARTESIAN_POINT ( 'NONE',  ( 15.24017643949430401, 10.92755873383624454, 6.180339887498953466 ) ) ;
#44294=CARTESIAN_POINT ( 'NONE',  ( 86.22341231051544241, 46.94107917315361078, -10.56950783746432698 ) ) ;
#44296=VERTEX_POINT ( 'NONE', #3431 ) ;
#44304=CARTESIAN_POINT ( 'NONE',  ( 69.13511649644314616, 71.04256955909853843, 2.869324681485878275E-06 ) ) ;
#44305=CARTESIAN_POINT ( 'NONE',  ( 81.32775793644282203, 42.22126959800928603, -7.181039397308548011 ) ) ;
#44306=EDGE_LOOP ( 'NONE', ( #45301, #32221, #84353, #59372 ) ) ;
#44308=CARTESIAN_POINT ( 'NONE',  ( 88.42339661562220954, 43.82656006556687345, 0.1181016345699155146 ) ) ;
#44310=CARTESIAN_POINT ( 'NONE',  ( 71.90400658755810070, 72.53437165389429708, 1.750395423964758557 ) ) ;
#44313=CARTESIAN_POINT ( 'NONE',  ( 87.87588256303088485, 45.05834245088315981, 6.537532970176371805 ) ) ;
#44316=CARTESIAN_POINT ( 'NONE',  ( 71.41016749218992743, 59.45273978182970609, 15.69346469599747174 ) ) ;
#44320=CARTESIAN_POINT ( 'NONE',  ( 82.71327011143105779, 53.60354310397067934, -15.74390733313335922 ) ) ;
#44324=CARTESIAN_POINT ( 'NONE',  ( 11.13306418284875576, 18.37878583063839244, 9.188101187500006262 ) ) ;
#44325=ORIENTED_EDGE ( 'NONE', *, *, #20805, .T. ) ;
#44332=EDGE_CURVE ( 'NONE', #5374, #22952, #4437, .T. ) ;
#44337=CARTESIAN_POINT ( 'NONE',  ( 86.93970924122183419, 44.33811398603066323, 5.029826232848033207 ) ) ;
#44339=VERTEX_POINT ( 'NONE', #6887 ) ;
#44348=CARTESIAN_POINT ( 'NONE',  ( 85.38005290443321371, 44.62545188726001300, -7.421218069141172435 ) ) ;
#44351=CARTESIAN_POINT ( 'NONE',  ( 75.99079911453461023, 65.46731794264749738, 14.35477091480207967 ) ) ;
#44358=CARTESIAN_POINT ( 'NONE',  ( 69.56932906937804262, 66.26470779536496991, -10.53527169505675509 ) ) ;
#44360=CARTESIAN_POINT ( 'NONE',  ( 85.24872127118341325, 42.51433283568908195, 1.035734531770441169 ) ) ;
#44362=CARTESIAN_POINT ( 'NONE',  ( 84.25611980550206681, 46.28114692587162438, 10.44557183192605265 ) ) ;
#44364=EDGE_CURVE ( 'NONE', #24743, #59656, #12892, .T. ) ;
#44369=CARTESIAN_POINT ( 'NONE',  ( 79.28644739073136805, 58.22391059449252282, 16.22396175955610786 ) ) ;
#44376=CARTESIAN_POINT ( 'NONE',  ( 85.03805233423882726, 49.96613157754471501, 13.55353664355913956 ) ) ;
#44386=CARTESIAN_POINT ( 'NONE',  ( 84.27014134724090866, 42.34832866126101436, -3.331555649036015865 ) ) ;
#44388=CARTESIAN_POINT ( 'NONE',  ( 75.88363445057348144, 65.49265179502715739, 14.31053417012051376 ) ) ;
#44390=CARTESIAN_POINT ( 'NONE',  ( 36.73494696561986217, 42.18502408145594984, 5.678558825948276656 ) ) ;
#44392=FACE_BOUND ( 'NONE', #13035, .T. ) ;
#44393=ORIENTED_EDGE ( 'NONE', *, *, #32855, .T. ) ;
#44394=CARTESIAN_POINT ( 'NONE',  ( 28.18775043786755319, 21.98920272979927759, 7.433330006724137462 ) ) ;
#44400=CARTESIAN_POINT ( 'NONE',  ( 75.95690509902382814, 65.20561023377018728, -14.47468716891346219 ) ) ;
#44402=CARTESIAN_POINT ( 'NONE',  ( 73.27399602445112237, 57.75849500631026245, 16.33089542203346767 ) ) ;
#44405=CARTESIAN_POINT ( 'NONE',  ( 75.09903334936105068, 52.93404696900269357, -16.00280056458343836 ) ) ;
#44413=CARTESIAN_POINT ( 'NONE',  ( 66.10228174255657052, 68.64626758096548542, 4.271897712742703135 ) ) ;
#44416=CARTESIAN_POINT ( 'NONE',  ( 87.07963357598215737, 43.74386682785180369, 2.609826112548035759 ) ) ;
#44417=VECTOR ( 'NONE', #55390, 1000.000000000000114 ) ;
#44426=CARTESIAN_POINT ( 'NONE',  ( 38.69312636016019269, 30.84335787977765975, 9.188101187500006262 ) ) ;
#44427=CARTESIAN_POINT ( 'NONE',  ( 77.46076174113461832, 59.13541342898363240, -16.06266701479841785 ) ) ;
#44432=CARTESIAN_POINT ( 'NONE',  ( 81.54798657518921345, 42.52537976816986287, 7.469856817513908176 ) ) ;
#44437=CARTESIAN_POINT ( 'NONE',  ( 74.11595357172687670, 61.08279995983697575, -15.22303157954070940 ) ) ;
#44447=CARTESIAN_POINT ( 'NONE',  ( 73.82480279627529285, 68.30552952313148296, -11.59219441058860589 ) ) ;
#44450=CARTESIAN_POINT ( 'NONE',  ( 67.70744425388356547, 69.01537731644371831, 5.819509745403966150 ) ) ;
#44451=EDGE_CURVE ( 'NONE', #92910, #47283, #1296, .T. ) ;
#44452=B_SPLINE_CURVE_WITH_KNOTS ( 'NONE', 3,
 ( #83589, #90706, #67856, #13661, #6049, #83090, #5553, #82609, #52141, #53144, #20772, #51142, #82106, #36438, #84100, #21748, #13175, #45039, #67345, #75982, #6557, #36943, #29849, #98777, #44532, #14652, #37430, #99263, #75464, #45530, #68339, #29358, #43545, #60224, #76461, #74486, #37921, #99758, #30348, #5064, #91186, #35946, #66847, #32342, #8551, #47044 ),
 .UNSPECIFIED., .F., .F.,
 ( 4, 1, 2, 2, 1, 2, 2, 1, 1, 2, 2, 1, 1, 2, 2, 1, 1, 2, 2, 1, 1, 1, 2, 2, 1, 1, 1, 2, 2, 4 ),
 ( 0.000000000000000000, 0.06250000000000141553, 0.09375000000000073552, 0.1250000000000000555, 0.1874999999999985012, 0.2187499999999978073, 0.2499999999999971412, 0.3124999999999955036, 0.3437499999999950040, 0.3593749999999945599, 0.3749999999999940603, 0.4374999999999884537, 0.4687499999999856781, 0.4843749999999853451, 0.4999999999999849565, 0.5624999999999893419, 0.5937499999999898970, 0.6093749999999897859, 0.6249999999999896749, 0.6874999999999938938, 0.7187499999999972244, 0.7343749999999993339, 0.7421875000000008882, 0.7500000000000025535, 0.8125000000000000000, 0.8437499999999998890, 0.8593749999999997780, 0.8671875000000003331, 0.8750000000000007772, 1.000000000000000000 ),
 .UNSPECIFIED. ) ;
#44456=ORIENTED_EDGE ( 'NONE', *, *, #10755, .T. ) ;
#44467=CARTESIAN_POINT ( 'NONE',  ( 71.33560860404993775, 62.23091869455711134, 14.08802979949528655 ) ) ;
#44468=CARTESIAN_POINT ( 'NONE',  ( 82.63281508735799719, 40.94328431217294195, -3.617117793222135447 ) ) ;
#44473=CARTESIAN_POINT ( 'NONE',  ( 83.88636183630472942, 44.33847814200196069, 8.266257927242135040 ) ) ;
#44474=CYLINDRICAL_SURFACE ( 'NONE', #21951, 16.60714546451156792 ) ;
#44475=CARTESIAN_POINT ( 'NONE',  ( 70.43138298049650814, 61.25676307520114250, -14.82522626399372889 ) ) ;
#44476=EDGE_CURVE ( 'NONE', #24132, #69830, #78194, .T. ) ;
#44477=CARTESIAN_POINT ( 'NONE',  ( 70.02137158282522478, 70.42997685080844406, -4.196993381856343852 ) ) ;
#44486=CARTESIAN_POINT ( 'NONE',  ( 73.71929281187129845, 69.57097904280846024, -9.712794511546583465 ) ) ;
#44489=CARTESIAN_POINT ( 'NONE',  ( 33.58045587329145576, 41.16126292948898424, -6.180339887498951690 ) ) ;
#44492=CARTESIAN_POINT ( 'NONE',  ( 72.11830045305705994, 72.06781504142615802, 2.913192023061343949 ) ) ;
#44496=CARTESIAN_POINT ( 'NONE',  ( 81.57843032188139887, 42.64747388495735692, -7.641580732431849654 ) ) ;
#44498=CARTESIAN_POINT ( 'NONE',  ( 72.12583136055069133, 72.30106763173874640, -1.396970068680259969 ) ) ;
#44502=CARTESIAN_POINT ( 'NONE',  ( 18.45699304436188015, 28.84336893147756342, -7.433330006724137462 ) ) ;
#44503=CARTESIAN_POINT ( 'NONE',  ( 31.27486418823966119, 41.55466486950703597, 7.012934429366973338E-14 ) ) ;
#44505=CARTESIAN_POINT ( 'NONE',  ( 34.47489329363036603, 42.83705186507756935, 3.090169943749475401 ) ) ;
#44509=CARTESIAN_POINT ( 'NONE',  ( 73.35233208022572171, 64.24922777283234154, 13.69859057857681250 ) ) ;
#44510=CARTESIAN_POINT ( 'NONE',  ( 73.94193992219132383, 67.36277748690798717, -11.91547202175585340 ) ) ;
#44519=CARTESIAN_POINT ( 'NONE',  ( 88.92874521539408761, 44.69521367694441949, 1.972556413651489717E-15 ) ) ;
#44524=CARTESIAN_POINT ( 'NONE',  ( 79.12983535314947403, 46.24050403399365194, -12.75843083597309402 ) ) ;
#44530=CARTESIAN_POINT ( 'NONE',  ( 27.97303175072023151, 18.01110640527293327, 2.839279412974134775 ) ) ;
#44531=CARTESIAN_POINT ( 'NONE',  ( 68.55211899962544919, 64.27634076875820313, 12.40740400025066670 ) ) ;
#44532=CARTESIAN_POINT ( 'NONE',  ( 69.01602661498650093, 69.91613256616328442, -3.960103623913056037 ) ) ;
#44535=CARTESIAN_POINT ( 'NONE',  ( 77.33932581937109774, 58.33597099166552624, 16.55227366965920766 ) ) ;
#44543=CARTESIAN_POINT ( 'NONE',  ( 65.95699843562651665, 69.05652685496262677, -2.081137445023961252 ) ) ;
#44545=CARTESIAN_POINT ( 'NONE',  ( 81.89485588203808675, 55.22971306509116829, 16.24120679747551677 ) ) ;
#44552=CARTESIAN_POINT ( 'NONE',  ( 79.09182929055386069, 45.95956795106130244, 13.18793794369859818 ) ) ;
#44556=ORIENTED_EDGE ( 'NONE', *, *, #94262, .T. ) ;
#44557=CARTESIAN_POINT ( 'NONE',  ( 76.27486002672000609, 65.07516076971148777, 14.62441312286923534 ) ) ;
#44560=CARTESIAN_POINT ( 'NONE',  ( 84.51277906370384585, 42.32962709305126481, -4.653106241441020252 ) ) ;
#44561=CARTESIAN_POINT ( 'NONE',  ( 81.29647558948052222, 56.17074938437520615, 16.09536513502975552 ) ) ;
#44563=ADVANCED_FACE ( 'NONE', ( #11904 ), #58649, .T. ) ;
#44564=CARTESIAN_POINT ( 'NONE',  ( 71.07161859112099478, 65.75594004187888686, 11.78334260209157236 ) ) ;
#44571=CARTESIAN_POINT ( 'NONE',  ( 76.19538127100192071, 51.60791020780316529, -16.17731679098115549 ) ) ;
#44573=CARTESIAN_POINT ( 'NONE',  ( 81.05763270389509501, 43.67158023151814916, 9.470390458390101074 ) ) ;
#44579=VERTEX_POINT ( 'NONE', #79172 ) ;
#44583=VECTOR ( 'NONE', #56044, 1000.000000000000227 ) ;
#44584=CARTESIAN_POINT ( 'NONE',  ( 79.51536559218330069, 59.45954251456831230, -16.20368373865058231 ) ) ;
#44585=CARTESIAN_POINT ( 'NONE',  ( 68.00997593938822661, 67.42022595953058328, -7.990198427795091263 ) ) ;
#44586=ORIENTED_EDGE ( 'NONE', *, *, #2141, .T. ) ;
#44590=CARTESIAN_POINT ( 'NONE',  ( 79.49951204047911801, 46.37032438487753438, 12.70281872619212926 ) ) ;
#44591=CARTESIAN_POINT ( 'NONE',  ( 73.59092698701640245, 69.71842387940506569, -9.437048835751642883 ) ) ;
#44594=CARTESIAN_POINT ( 'NONE',  ( 71.38700058129320780, 71.90615381975096909, 0.1362715070751574220 ) ) ;
#44598=CARTESIAN_POINT ( 'NONE',  ( 25.25549177415141955, 22.78052372038641238, -10.00000000000000355 ) ) ;
#44608=CARTESIAN_POINT ( 'NONE',  ( 66.86791019689516702, 67.62081465971216687, -6.465500182084312542 ) ) ;
#44614=CARTESIAN_POINT ( 'NONE',  ( 29.35192616055884685, 22.11029122506295863, -8.090169943749478065 ) ) ;
#44615=CARTESIAN_POINT ( 'NONE',  ( 85.38233340156565987, 49.09383606134155542, 12.40279396366186404 ) ) ;
#44617=CARTESIAN_POINT ( 'NONE',  ( 71.94697066620052794, 72.20377774097838142, -3.624262489285473343 ) ) ;
#44625=CARTESIAN_POINT ( 'NONE',  ( 39.57658603661993624, 34.80066082961425877, 10.00000000000000533 ) ) ;
#44628=CARTESIAN_POINT ( 'NONE',  ( 72.78963790118945099, 71.14248580567580404, -7.401817665068024077 ) ) ;
#44631=CARTESIAN_POINT ( 'NONE',  ( 35.00289615805098009, 41.18502408145595695, 5.678558825948277544 ) ) ;
#44637=CARTESIAN_POINT ( 'NONE',  ( 19.72235211587467063, 17.10170272979926764, -7.433330006724141015 ) ) ;
#44640=CARTESIAN_POINT ( 'NONE',  ( 71.46833469722506038, 59.16469923302185663, 15.78718056386504642 ) ) ;
#44645=CARTESIAN_POINT ( 'NONE',  ( 84.80046560730060889, 45.49911806156455185, -9.891506693440607734 ) ) ;
#44646=CARTESIAN_POINT ( 'NONE',  ( 81.77267345883888083, 42.08915124187546297, 7.561132706673316939 ) ) ;
#44649=CARTESIAN_POINT ( 'NONE',  ( 67.15811240557331985, 69.28574695336774880, 1.445375503756383795 ) ) ;
#44654=ORIENTED_EDGE ( 'NONE', *, *, #70279, .T. ) ;
#44660=CARTESIAN_POINT ( 'NONE',  ( 80.46516936217979321, 57.89407423507869055, 16.25250200478403428 ) ) ;
#44681=CARTESIAN_POINT ( 'NONE',  ( 73.67010975928342020, 69.53433136659224090, 9.708230610803601834 ) ) ;
#44683=CARTESIAN_POINT ( 'NONE',  ( 82.45129306854981621, 53.84777233740991420, 15.85475489262521620 ) ) ;
#44691=CARTESIAN_POINT ( 'NONE',  ( 79.26668090384839616, 56.12960650164554011, -16.16769687457144755 ) ) ;
#44692=CARTESIAN_POINT ( 'NONE',  ( 30.63508420971764679, 41.18528772668520332, -1.583844403245363575 ) ) ;
#44694=CARTESIAN_POINT ( 'NONE',  ( 66.62671586282783665, 69.45108170673691461, 2.068076428306299785 ) ) ;
#44696=CARTESIAN_POINT ( 'NONE',  ( 86.51086010412997496, 43.19054546371415171, 3.687685646923426930 ) ) ;
#44700=CARTESIAN_POINT ( 'NONE',  ( 79.16171021146236342, 53.16507682567369386, -15.71592495584207150 ) ) ;
#44702=CARTESIAN_POINT ( 'NONE',  ( 79.05185236193558751, 46.14960762662803972, 12.72882390507626127 ) ) ;
#44704=CARTESIAN_POINT ( 'NONE',  ( 83.71005568810697639, 52.19702411997352698, -14.66788051681769822 ) ) ;
#44705=VERTEX_POINT ( 'NONE', #5613 ) ;
#44707=CARTESIAN_POINT ( 'NONE',  ( 83.43812176953721860, 42.81150887395778426, 7.143380295109257538 ) ) ;
#44712=CARTESIAN_POINT ( 'NONE',  ( 84.14312167556933275, 48.98415679381830756, 0.000000000000000000 ) ) ;
#44720=CARTESIAN_POINT ( 'NONE',  ( 73.05912352472130067, 69.60491006942920933, 9.219028434792550186 ) ) ;
#44721=DIRECTION ( 'NONE',  ( 0.5840252505817135065, 0.000000000000000000, 0.8117354905897405937 ) ) ;
#44725=CARTESIAN_POINT ( 'NONE',  ( 81.71293863666839741, 41.47842697493793196, -5.166121441586708052 ) ) ;
#44731=CARTESIAN_POINT ( 'NONE',  ( 79.18684305567127524, 59.44391592844133498, -16.53590917749600919 ) ) ;
#44734=EDGE_CURVE ( 'NONE', #57136, #54902, #41861, .T. ) ;
#44737=CARTESIAN_POINT ( 'NONE',  ( 69.20949672380906748, 68.87578926811286806, -7.751714074739255445 ) ) ;
#44740=CARTESIAN_POINT ( 'NONE',  ( 71.78644915716171226, 58.70311003640473757, -15.46670377541668273 ) ) ;
#44746=CARTESIAN_POINT ( 'NONE',  ( 73.93007176995158147, 55.19876193233204020, 16.12294130170896622 ) ) ;
#44748=CARTESIAN_POINT ( 'NONE',  ( 66.32312229954955285, 68.11665519946647862, -4.542135202938414551 ) ) ;
#44749=EDGE_LOOP ( 'NONE', ( #40187, #92186, #88876, #93289 ) ) ;
#44755=CARTESIAN_POINT ( 'NONE',  ( 23.58217936225004863, 25.56628583063841376, 9.188101187500006262 ) ) ;
#44760=CARTESIAN_POINT ( 'NONE',  ( 88.07864672190808619, 43.84249974723677923, 2.482382391715419523 ) ) ;
#44761=CARTESIAN_POINT ( 'NONE',  ( 75.07027850253338386, 67.11046765588916685, 13.07895222455245055 ) ) ;
#44762=CARTESIAN_POINT ( 'NONE',  ( 69.09645378865941723, 64.24355404979770867, 12.03626827164885604 ) ) ;
#44764=DIRECTION ( 'NONE',  ( -0.7162481363636782339, 0.000000000000000000, 0.6978456900745019231 ) ) ;
#44766=CARTESIAN_POINT ( 'NONE',  ( 69.17795686453304427, 67.22120498262539456, -9.978070790114912825 ) ) ;
#44770=CARTESIAN_POINT ( 'NONE',  ( 70.76518571626657206, 70.00280625673043744, 6.363910008508249838 ) ) ;
#44773=EDGE_CURVE ( 'NONE', #39921, #25006, #35080, .T. ) ;
#44776=CARTESIAN_POINT ( 'NONE',  ( 81.87359138893998534, 41.32955797152818889, 5.976920566253458134 ) ) ;
#44781=CARTESIAN_POINT ( 'NONE',  ( 11.59314018038319283, 18.64441083166259361, -10.00000000000000533 ) ) ;
#44782=DIRECTION ( 'NONE',  ( 0.2347357813929421555, -0.4065742997269585213, 0.8829475928589297640 ) ) ;
#44787=ORIENTED_EDGE ( 'NONE', *, *, #4754, .F. ) ;
#44790=B_SPLINE_CURVE_WITH_KNOTS ( 'NONE', 3,
 ( #46467, #84529, #69779, #30794, #15073, #45962, #61673, #92623, #23173, #31276, #62164, #93113, #23665, #85541, #16082, #1896 ),
 .UNSPECIFIED., .F., .F.,
 ( 4, 1, 2, 2, 2, 1, 2, 2, 4 ),
 ( 0.000000000000000000, 0.1250000000000054956, 0.1875000000000070499, 0.2500000000000086042, 0.5000000000000109912, 0.6250000000000103251, 0.6875000000000102141, 0.7500000000000101030, 1.000000000000000000 ),
 .UNSPECIFIED. ) ;
#44798=CARTESIAN_POINT ( 'NONE',  ( 81.64801244726884022, 42.30507044763769642, -8.030039233986487446 ) ) ;
#44802=ORIENTED_EDGE ( 'NONE', *, *, #49958, .F. ) ;
#44805=CARTESIAN_POINT ( 'NONE',  ( 69.48788112159641628, 70.05884240972372368, 4.410909553017925866 ) ) ;
#44806=EDGE_LOOP ( 'NONE', ( #5183, #34108, #76943, #87866 ) ) ;
#44809=VECTOR ( 'NONE', #35881, 1000.000000000000227 ) ;
#44812=CARTESIAN_POINT ( 'NONE',  ( 82.74895235971042950, 53.70034252712168410, -15.76590362002541390 ) ) ;
#44817=CARTESIAN_POINT ( 'NONE',  ( 19.72235211587467063, 17.10170272979926764, -7.433330006724141015 ) ) ;
#44823=ORIENTED_EDGE ( 'NONE', *, *, #49010, .F. ) ;
#44834=( BOUNDED_CURVE ( )  B_SPLINE_CURVE ( 2, ( #10540, #73342, #27734, #80477, #41925, #58121, #18644, #35318, #3451, #50030, #41414, #11047, #40903 ),
 .UNSPECIFIED., .F., .T. ) 
 B_SPLINE_CURVE_WITH_KNOTS ( ( 3, 2, 2, 2, 2, 2, 3 ),
 ( 0.4874999999999999889, 0.4899999999999999911, 0.4949999999999999956, 0.5000000000000000000, 0.5050000000000000044, 0.5100000000000000089, 0.5125000000000000666 ),
 .UNSPECIFIED. ) 
 CURVE ( )  GEOMETRIC_REPRESENTATION_ITEM ( )  RATIONAL_B_SPLINE_CURVE ( ( 0.9755282581475768211, 0.9755282581475768211, 1.000000000000000000, 0.9510565162951535312, 1.000000000000000000, 0.9510565162951535312, 1.000000000000000000, 0.9510565162951535312, 1.000000000000000000, 0.9510565162951535312, 1.000000000000000000, 0.9755282581475761550, 0.9755282581475767101 ) ) 
 REPRESENTATION_ITEM ( '' )  );
#44842=CARTESIAN_POINT ( 'NONE',  ( 83.48498291495343437, 44.67303044464677697, -9.033275216153651144 ) ) ;
#44853=CARTESIAN_POINT ( 'NONE',  ( 85.04377965201177858, 48.84687674572034410, 12.36303725827022149 ) ) ;
#44857=CARTESIAN_POINT ( 'NONE',  ( 87.72832916959468719, 44.38926273554258728, -3.984038184195087595 ) ) ;
#44858=CARTESIAN_POINT ( 'NONE',  ( 66.31795133325435643, 69.20145725284447735, 2.477662600225432055 ) ) ;
#44862=CARTESIAN_POINT ( 'NONE',  ( 77.25811804238409763, 54.54226996051674803, -16.06399464395360255 ) ) ;
#44869=CARTESIAN_POINT ( 'NONE',  ( 84.56695678370634539, 50.23807730109928826, 13.87492620287773804 ) ) ;
#44874=VECTOR ( 'NONE', #44782, 999.9999999999998863 ) ;
#44877=CARTESIAN_POINT ( 'NONE',  ( 12.88253908977640094, 9.298606405272902720, -2.839279412974138328 ) ) ;
#44878=CARTESIAN_POINT ( 'NONE',  ( 67.68582956716421961, 65.71206495485193955, 10.68281714332846555 ) ) ;
#44879=ADVANCED_FACE ( 'NONE', ( #51598 ), #16084, .T. ) ;
#44880=CARTESIAN_POINT ( 'NONE',  ( 9.678154728840961951, 27.36126292948894090, 6.180339887498949913 ) ) ;
#44881=CARTESIAN_POINT ( 'NONE',  ( 83.06579348197817581, 42.04301930353511807, -4.596628070075716721 ) ) ;
#44885=CARTESIAN_POINT ( 'NONE',  ( 41.60632629512001301, 26.94754757982093096, 5.678558825948272215 ) ) ;
#44887=FACE_BOUND ( 'NONE', #99690, .T. ) ;
#44889=CARTESIAN_POINT ( 'NONE',  ( 29.48197064213787044, 19.94754757982090609, 5.678558825948272215 ) ) ;
#44891=CARTESIAN_POINT ( 'NONE',  ( 16.37683477841346047, 11.58380873178785642, 6.180339887498953466 ) ) ;
#44896=EDGE_CURVE ( 'NONE', #32075, #19304, #56393, .T. ) ;
#44897=CARTESIAN_POINT ( 'NONE',  ( 70.73225150608038803, 60.85528942256977558, 14.53863242546318446 ) ) ;
#44901=STYLED_ITEM('',(#100338),#9388);
#44906=CARTESIAN_POINT ( 'NONE',  ( 66.10335034196877757, 68.51773249980182356, 4.672338372422939479 ) ) ;
#44912=CARTESIAN_POINT ( 'NONE',  ( 85.03805233423882726, 49.96613157754471501, 13.55353664355913956 ) ) ;
#44915=DIRECTION ( 'NONE',  ( 0.3473291852294957405, -0.6015917957689906892, 0.7193398003386545225 ) ) ;
#44916=CARTESIAN_POINT ( 'NONE',  ( 37.11382629638189457, 33.37878583063844218, 9.188101187500006262 ) ) ;
#44918=CARTESIAN_POINT ( 'NONE',  ( 75.97978661270015266, 62.19592087238390121, -15.66257012141549687 ) ) ;
#44924=CARTESIAN_POINT ( 'NONE',  ( 84.37825102736907468, 49.99960613749294680, 13.80049582259581520 ) ) ;
#44925=EDGE_CURVE ( 'NONE', #17810, #69750, #98767, .T. ) ;
#44931=CARTESIAN_POINT ( 'NONE',  ( 82.37522948072516726, 40.40699566382964036, 1.446055329426206848 ) ) ;
#44934=CARTESIAN_POINT ( 'NONE',  ( 77.06427544118604089, 63.50113506902185634, -15.44174958657458951 ) ) ;
#44941=CARTESIAN_POINT ( 'NONE',  ( 28.93411276635479368, 38.74646525600392266, 2.839279412974139660 ) ) ;
#44946=CARTESIAN_POINT ( 'NONE',  ( 74.21927401529055146, 68.62113723208385352, -11.51360559050239374 ) ) ;
#44976=CARTESIAN_POINT ( 'NONE',  ( 31.27486418823966119, 41.55466486950703597, 7.012934429366973338E-14 ) ) ;
#44981=DIRECTION ( 'NONE',  ( -0.4999999999999974465, 0.8660254037844402619, 0.000000000000000000 ) ) ;
#44984=CARTESIAN_POINT ( 'NONE',  ( 66.62014279665129379, 67.58845556211061023, 6.252763347840865293 ) ) ;
#44987=CARTESIAN_POINT ( 'NONE',  ( 73.51766844768523868, 69.20770085021928253, -10.00626470679032387 ) ) ;
#44988=CARTESIAN_POINT ( 'NONE',  ( 70.70420039156243774, 71.94848598797803163, 6.061257734329015641E-06 ) ) ;
#44989=LINE ( 'NONE', #21219, #68562 ) ;
#44991=CARTESIAN_POINT ( 'NONE',  ( 82.26031953026701160, 54.24911196204305242, 15.63359092428133401 ) ) ;
#44992=CARTESIAN_POINT ( 'NONE',  ( 71.81276634784433099, 72.21619144530795609, 3.256612196116196234 ) ) ;
#44995=CARTESIAN_POINT ( 'NONE',  ( 81.19911097159209135, 42.30626095209706961, -7.446220821091688258 ) ) ;
#44999=CARTESIAN_POINT ( 'NONE',  ( 71.77363275119753894, 72.50400781664164640, -1.333432854898964681 ) ) ;
#45001=CIRCLE ( 'NONE', #95190, 15.10714546451156792 ) ;
#45002=CARTESIAN_POINT ( 'NONE',  ( 16.96131155903493593, 31.83396525600390348, -2.839279412974133887 ) ) ;
#45005=CARTESIAN_POINT ( 'NONE',  ( 46.16810866859812990, 28.78380873178791077, -6.180339887498949025 ) ) ;
#45011=CARTESIAN_POINT ( 'NONE',  ( 72.09886792114333787, 59.49856892740179148, 15.29648596422838658 ) ) ;
#45021=VERTEX_POINT ( 'NONE', #88676 ) ;
#45029=AXIS2_PLACEMENT_3D ( 'NONE', #17959, #733, #2257 ) ;
#45031=CARTESIAN_POINT ( 'NONE',  ( 79.33488432162613435, 46.38139623303920445, -12.77319259312810118 ) ) ;
#45037=CARTESIAN_POINT ( 'NONE',  ( 21.52536902826200915, 24.37878583063841376, 9.188101187500006262 ) ) ;
#45038=CARTESIAN_POINT ( 'NONE',  ( 75.81630083228941430, 58.88796208816045663, 15.95549709212262535 ) ) ;
#45039=CARTESIAN_POINT ( 'NONE',  ( 70.06226729709648282, 70.14289581699462417, -5.146418532987001804 ) ) ;
#45040=CARTESIAN_POINT ( 'NONE',  ( 75.06185269395857063, 67.24559711482957880, -12.98328508234621026 ) ) ;
#45042=DIRECTION ( 'NONE',  ( -0.8660254037844361541, -0.5000000000000042188, -0.000000000000000000 ) ) ;
#45043=B_SPLINE_CURVE_WITH_KNOTS ( 'NONE', 3,
 ( #35682, #21006, #20499, #45267, #76200, #6776, #75199, #66584, #52369, #74211, #68069, #91407, #43767, #51372, #98503, #13396, #83314, #97994, #98993, #13876, #75690, #6277, #90931, #37171, #60454, #5775, #12908, #21972, #99491, #82828, #74711 ),
 .UNSPECIFIED., .F., .F.,
 ( 4, 3, 3, 3, 3, 3, 3, 3, 3, 3, 4 ),
 ( 0.000000000000000000, 0.1333490885032327655, 0.3007194338854324855, 0.4699862290245073182, 0.5844252810809297261, 0.6686540514502762322, 0.7354980260655518132, 0.8028463152565620264, 0.8633854507757146024, 0.9437142632667205877, 1.000000000000000000 ),
 .UNSPECIFIED. ) ;
#45046=CARTESIAN_POINT ( 'NONE',  ( 80.33776826693566875, 49.81241265353616399, -14.39611721561766799 ) ) ;
#45054=CARTESIAN_POINT ( 'NONE',  ( 77.18288558774111152, 49.26002351683675329, -15.37362206159445144 ) ) ;
#45055=CARTESIAN_POINT ( 'NONE',  ( 77.99518601148065500, 61.05539905302716619, -15.87786080876372985 ) ) ;
#45062=CARTESIAN_POINT ( 'NONE',  ( 73.29685492166123595, 60.06436106922850371, -15.83144761987708549 ) ) ;
#45070=FACE_OUTER_BOUND ( 'NONE', #8807, .T. ) ;
#45072=CARTESIAN_POINT ( 'NONE',  ( 88.02796755599807454, 43.59779901362369259, -1.172627947537940913E-07 ) ) ;
#45075=CARTESIAN_POINT ( 'NONE',  ( 71.63128215215617445, 67.23017368855626330, 10.79322251376788877 ) ) ;
#45076=CARTESIAN_POINT ( 'NONE',  ( 87.41847558182290356, 44.98594970355500777, 6.912341091792677084 ) ) ;
#45078=CARTESIAN_POINT ( 'NONE',  ( 20.25339421822757302, 23.64441083166260782, -10.00000000000000533 ) ) ;
#45082=CARTESIAN_POINT ( 'NONE',  ( 76.28872632189685987, 51.00282802106350744, -16.03419075290740636 ) ) ;
#45084=AXIS2_PLACEMENT_3D ( 'NONE', #8649, #25868, #41025 ) ;
#45085=CARTESIAN_POINT ( 'NONE',  ( 66.18968672761215544, 68.49487770601442094, -4.881532527435788360 ) ) ;
#45095=CARTESIAN_POINT ( 'NONE',  ( 80.47590545208809942, 44.37644993918018343, -10.62012430727854806 ) ) ;
#45096=CARTESIAN_POINT ( 'NONE',  ( 86.59400028779953118, 45.20624741140364478, 7.285646471211377317 ) ) ;
#45097=CARTESIAN_POINT ( 'NONE',  ( 88.05069107734583156, 43.77613950941169918, -2.175448891271404506 ) ) ;
#45099=CARTESIAN_POINT ( 'NONE',  ( 73.28493474805527796, 66.86745001568056068, -12.01134084813802438 ) ) ;
#45105=CARTESIAN_POINT ( 'NONE',  ( 81.29352784059901182, 52.88188998950131747, 15.35000877273065889 ) ) ;
#45106=CARTESIAN_POINT ( 'NONE',  ( 73.68745215720861097, 69.36524252693955361, -9.936694521456994167 ) ) ;
#45113=CARTESIAN_POINT ( 'NONE',  ( 19.48182849416020090, 34.18080186712593616, 3.090169943749475401 ) ) ;
#45116=CARTESIAN_POINT ( 'NONE',  ( 80.44297273216872668, 44.73620253192707708, -11.65665792466250927 ) ) ;
#45118=CARTESIAN_POINT ( 'NONE',  ( 72.00136543793328769, 71.75253384267894319, -3.919387538446478025 ) ) ;
#45122=CARTESIAN_POINT ( 'NONE',  ( 66.72975355781689188, 67.37222994295811418, -6.798010804002465157 ) ) ;
#45123=CARTESIAN_POINT ( 'NONE',  ( 72.87252120309179304, 71.00776288696198435, -7.711505026642224259 ) ) ;
#45126=CARTESIAN_POINT ( 'NONE',  ( 25.72017957606892580, 26.80066082961422680, 10.00000000000000533 ) ) ;
#45127=CARTESIAN_POINT ( 'NONE',  ( 85.16413976203500624, 49.03542080487202526, 12.45445162886715451 ) ) ;
#45129=CARTESIAN_POINT ( 'NONE',  ( 71.85042758235270810, 71.69843285251393183, -3.789477364735267084 ) ) ;
#45131=CARTESIAN_POINT ( 'NONE',  ( 82.78613357252183391, 43.65115152597518033, 9.027654786050977265 ) ) ;
#45134=EDGE_CURVE ( 'NONE', #60500, #51335, #39495, .T. ) ;
#45140=CARTESIAN_POINT ( 'NONE',  ( 66.57727237866471626, 69.35756060501768161, -2.461574745472292935 ) ) ;
#45142=CARTESIAN_POINT ( 'NONE',  ( 78.77203581278492095, 60.02538875188410827, 16.11206551482094795 ) ) ;
#45143=CARTESIAN_POINT ( 'NONE',  ( 42.32740281844729680, 26.29860640527295601, -2.839279412974138328 ) ) ;
#45151=CARTESIAN_POINT ( 'NONE',  ( 11.20403028766721398, 24.65586893147754921, -7.433330006724137462 ) ) ;
#45153=CARTESIAN_POINT ( 'NONE',  ( 71.94031269653281413, 59.11929964053626918, 15.37436981742643738 ) ) ;
#45158=CARTESIAN_POINT ( 'NONE',  ( 83.28414321500220296, 45.66981348057217360, -11.01983884672045910 ) ) ;
#45159=CARTESIAN_POINT ( 'NONE',  ( 81.64255549193633499, 42.62546693999003367, 7.546458374570336858 ) ) ;
#45160=EDGE_LOOP ( 'NONE', ( #3821, #51172, #82256, #47027 ) ) ;
#45161=DIRECTION ( 'NONE',  ( 0.5000000000000014433, -0.8660254037844378194, 0.000000000000000000 ) ) ;
#45167=VERTEX_POINT ( 'NONE', #48456 ) ;
#45173=CARTESIAN_POINT ( 'NONE',  ( 80.46882139176624094, 57.60428850591405592, -16.59250918983046574 ) ) ;
#45174=CARTESIAN_POINT ( 'NONE',  ( 72.76796725029400648, 69.66064322242992546, -9.545088302685920567 ) ) ;
#45180=CARTESIAN_POINT ( 'NONE',  ( 75.18426732535230883, 66.40243072218130749, 13.13391322278640239 ) ) ;
#45183=DIRECTION ( 'NONE',  ( 0.5000000000000014433, -0.8660254037844378194, 0.000000000000000000 ) ) ;
#45188=CARTESIAN_POINT ( 'NONE',  ( 83.54910681719562149, 52.38058030375331242, 14.79278836691776533 ) ) ;
#45200=CARTESIAN_POINT ( 'NONE',  ( 70.78197494834935810, 69.22129442327373283, 7.798897796936612004 ) ) ;
#45205=CARTESIAN_POINT ( 'NONE',  ( 78.33405375115705738, 47.76087145685212931, 13.91665194331178768 ) ) ;
#45209=CARTESIAN_POINT ( 'NONE',  ( 76.66452470125624075, 54.01436104093935597, -16.04660053521852703 ) ) ;
#45212=B_SPLINE_CURVE_WITH_KNOTS ( 'NONE', 3,
 ( #99258, #46015, #36939, #90700, #1323, #84582, #91675, #37918, #6551, #40290, #14145, #32205, #24607, #68830 ),
 .UNSPECIFIED., .F., .F.,
 ( 4, 2, 2, 2, 2, 2, 4 ),
 ( 0.000000000000000000, 0.2231112372999934090, 0.3346668559499891837, 0.4462224745999849307, 0.6693337118999764801, 0.7808893305499718940, 0.8924449491999673079 ),
 .UNSPECIFIED. ) ;
#45214=CARTESIAN_POINT ( 'NONE',  ( 83.58053473790808141, 52.37444464214736684, -15.15899823554475212 ) ) ;
#45219=CARTESIAN_POINT ( 'NONE',  ( 72.48454840684568978, 71.59325672763723958, 6.192859277029571174 ) ) ;
#45220=EDGE_CURVE ( 'NONE', #83087, #24162, #48711, .T. ) ;
#45224=VECTOR ( 'NONE', #23941, 1000.000000000000114 ) ;
#45225=CYLINDRICAL_SURFACE ( 'NONE', #51301, 10.00000000000001066 ) ;
#45226=CARTESIAN_POINT ( 'NONE',  ( 84.13204908911603752, 50.42604040346916605, 13.71367173376234838 ) ) ;
#45232=CARTESIAN_POINT ( 'NONE',  ( 75.06695094285400671, 67.05599132900850634, -12.66018568268392208 ) ) ;
#45236=CARTESIAN_POINT ( 'NONE',  ( 81.73784743073348125, 41.66220971920373017, -5.569503698209836706 ) ) ;
#45241=ORIENTED_EDGE ( 'NONE', *, *, #7646, .T. ) ;
#45248=CARTESIAN_POINT ( 'NONE',  ( 14.99119413235835729, 10.78380873178785393, -6.180339887498949025 ) ) ;
#45250=CARTESIAN_POINT ( 'NONE',  ( 71.67621869789168443, 58.80470100248025034, -15.42187440688404010 ) ) ;
#45252=ADVANCED_FACE ( 'NONE', ( #32743 ), #56023, .T. ) ;
#45257=CARTESIAN_POINT ( 'NONE',  ( 72.71764745495315196, 57.12077235107377504, 16.37631838998483857 ) ) ;
#45258=CARTESIAN_POINT ( 'NONE',  ( 66.21002856626215305, 68.68800931748855021, -4.337945611540375168 ) ) ;
#45264=CARTESIAN_POINT ( 'NONE',  ( 25.31423016981892715, 26.56628583063841731, 9.188101187500006262 ) ) ;
#45265=CYLINDRICAL_SURFACE ( 'NONE', #26500, 16.60714546451156792 ) ;
#45266=EDGE_CURVE ( 'NONE', #19562, #10543, #70940, .T. ) ;
#45267=CARTESIAN_POINT ( 'NONE',  ( 83.66208585045004043, 52.31085355490836264, -15.11568120807085336 ) ) ;
#45269=CARTESIAN_POINT ( 'NONE',  ( 88.09744597521934395, 43.85530739230785713, 2.493575494356681688 ) ) ;
#45271=CARTESIAN_POINT ( 'NONE',  ( 68.69116047246832579, 64.25973440136523607, 12.48137981580948441 ) ) ;
#45274=CARTESIAN_POINT ( 'NONE',  ( 75.75493378409400691, 65.86437009324527025, -14.07593894684413804 ) ) ;
#45276=CARTESIAN_POINT ( 'NONE',  ( 3.278110179240818045, 23.93396525600387648, 2.839279412974139660 ) ) ;
#45278=DIRECTION ( 'NONE',  ( -0.8845109580947931871, 0.1124011590738229760, -0.4527762631246169400 ) ) ;
#45280=CARTESIAN_POINT ( 'NONE',  ( 71.69150499680799271, 72.11108097137680772, 0.6386526183549271485 ) ) ;
#45284=CARTESIAN_POINT ( 'NONE',  ( 69.33671394560225565, 70.52709464844167542, 2.076833668242843434 ) ) ;
#45288=CARTESIAN_POINT ( 'NONE',  ( 13.83924611881801958, 13.15404122711132118, 8.090169943749479842 ) ) ;
#45300=CARTESIAN_POINT ( 'NONE',  ( 69.40990849430419019, 62.86359034874993057, 13.12394659649692841 ) ) ;
#45301=ORIENTED_EDGE ( 'NONE', *, *, #48612, .F. ) ;
#45305=CARTESIAN_POINT ( 'NONE',  ( 81.20826322331814140, 42.31471022520455705, -7.450868512929636367 ) ) ;
#45306=VERTEX_POINT ( 'NONE', #4866 ) ;
#45309=CARTESIAN_POINT ( 'NONE',  ( 80.64008363966095772, 47.31418076955320373, 12.92985048805446802 ) ) ;
#45311=CARTESIAN_POINT ( 'NONE',  ( 69.72532707139153274, 70.32948975208321940, 4.014237884418147218 ) ) ;
#45312=VECTOR ( 'NONE', #68168, 1000.000000000000114 ) ;
#45318=CARTESIAN_POINT ( 'NONE',  ( 67.66304282922978075, 68.28595519557160287, -6.094803320878922293 ) ) ;
#45319=ORIENTED_EDGE ( 'NONE', *, *, #18143, .T. ) ;
#45321=CARTESIAN_POINT ( 'NONE',  ( 12.86511499041763074, 19.37878583063839244, 9.188101187500006262 ) ) ;
#45324=CARTESIAN_POINT ( 'NONE',  ( 80.42870892512175374, 57.78063267130220027, 16.59889063300756007 ) ) ;
#45330=CARTESIAN_POINT ( 'NONE',  ( 79.76359975193354046, 44.98417069036879923, 11.54310746654911846 ) ) ;
#45337=CARTESIAN_POINT ( 'NONE',  ( 71.58048890525513741, 63.26397358144141236, -13.65483747980514728 ) ) ;
#45344=CARTESIAN_POINT ( 'NONE',  ( 72.10371214944608198, 72.33074704757831341, 0.8698369498405258415 ) ) ;
#45345=CARTESIAN_POINT ( 'NONE',  ( 72.47401207315012073, 70.81051498135123268, 7.656770371261347741 ) ) ;
#45347=CARTESIAN_POINT ( 'NONE',  ( 33.52502306405203569, 19.75978393459167037, -1.583844403245396437 ) ) ;
#45357=CARTESIAN_POINT ( 'NONE',  ( 81.04334714743738743, 43.68570708857655660, -9.496964033599468280 ) ) ;
#45362=CARTESIAN_POINT ( 'NONE',  ( 65.85576469104950093, 68.94656342641907543, 2.408941155072679585 ) ) ;
#45363=CARTESIAN_POINT ( 'NONE',  ( 87.33294734268930881, 44.88192199842172414, 6.808005391826766228 ) ) ;
#45364=CARTESIAN_POINT ( 'NONE',  ( 84.14312167556933275, 48.98415679381830756, 0.000000000000000000 ) ) ;
#45365=CARTESIAN_POINT ( 'NONE',  ( 81.10163913880589348, 53.21425096942738264, -15.47470560983101073 ) ) ;
#45368=CARTESIAN_POINT ( 'NONE',  ( 81.94022493854585321, 45.96546865081016620, 11.96996177621078949 ) ) ;
#45370=EDGE_CURVE ( 'NONE', #1813, #65113, #75757, .T. ) ;
#45375=ORIENTED_EDGE ( 'NONE', *, *, #14490, .F. ) ;
#45381=CARTESIAN_POINT ( 'NONE',  ( 10.59179830548347745, 18.06628583063839599, -9.188101187500006262 ) ) ;
#45385=CARTESIAN_POINT ( 'NONE',  ( 9.089523648746947515, 28.18080186712591484, 3.090169943749475401 ) ) ;
#45390=CARTESIAN_POINT ( 'NONE',  ( 43.88624854525928498, 27.19860640527296169, 2.839279412974134775 ) ) ;
#45392=FACE_OUTER_BOUND ( 'NONE', #25098, .T. ) ;
#45393=ORIENTED_EDGE ( 'NONE', *, *, #84255, .F. ) ;
#45394=CARTESIAN_POINT ( 'NONE',  ( 24.26418115112394247, 34.98502408145593279, -5.678558825948271327 ) ) ;
#45401=CARTESIAN_POINT ( 'NONE',  ( 70.69745823082493530, 60.91555314307392877, 15.03376646005350459 ) ) ;
#45402=CARTESIAN_POINT ( 'NONE',  ( 76.02744352951765450, 65.34233732453844823, -14.42760839744433632 ) ) ;
#45406=ORIENTED_EDGE ( 'NONE', *, *, #2847, .T. ) ;
#45412=CARTESIAN_POINT ( 'NONE',  ( 86.30977306730703447, 47.58285218899635538, -10.62438056216879900 ) ) ;
#45417=CARTESIAN_POINT ( 'NONE',  ( 35.53452623260358934, 35.91421378149921395, 9.188101187500008038 ) ) ;
#45419=CARTESIAN_POINT ( 'NONE',  ( 70.24301845481265616, 63.89562358154542210, -13.37649194025576094 ) ) ;
#45432=CARTESIAN_POINT ( 'NONE',  ( 82.32629218823147710, 40.36489395171674488, 1.301855596286184635 ) ) ;
#45434=CARTESIAN_POINT ( 'NONE',  ( 76.96225540874074511, 63.35506444885830035, -15.47139205492574554 ) ) ;
#45439=CARTESIAN_POINT ( 'NONE',  ( 44.10936046141049616, 26.26216523072498887, -2.296566073217252530E-15 ) ) ;
#45443=ORIENTED_EDGE ( 'NONE', *, *, #23730, .F. ) ;
#45444=CARTESIAN_POINT ( 'NONE',  ( 74.11971290936233459, 68.38772044953262252, -11.66991619212280895 ) ) ;
#45445=ADVANCED_FACE ( 'NONE', ( #61522 ), #14919, .T. ) ;
#45466=CARTESIAN_POINT ( 'NONE',  ( 72.70312890837641362, 66.64619018610765977, 11.87070177491906442 ) ) ;
#45467=CARTESIAN_POINT ( 'NONE',  ( 82.41110115525400204, 41.31668765478222838, -3.372589341468242186 ) ) ;
#45470=ADVANCED_FACE ( 'NONE', ( #78244 ), #85377, .T. ) ;
#45471=CARTESIAN_POINT ( 'NONE',  ( 71.65180518398884146, 72.09936778357817388, 3.358463432740969257 ) ) ;
#45473=CARTESIAN_POINT ( 'NONE',  ( 84.46573575848765358, 45.41160421943110492, 9.290855630086788608 ) ) ;
#45476=CARTESIAN_POINT ( 'NONE',  ( 82.73042059842214258, 53.63367031839453603, -15.74978661431507909 ) ) ;
#45484=CARTESIAN_POINT ( 'NONE',  ( 73.64702576733991179, 69.30673894177056127, -9.977882152455165965 ) ) ;
#45486=CARTESIAN_POINT ( 'NONE',  ( 2.403541337051680493, 23.16126292948892740, -6.180339887498951690 ) ) ;
#45487=CARTESIAN_POINT ( 'NONE',  ( 45.86230232835321630, 26.28848085856235173, 1.475505719884397138E-15 ) ) ;
#45490=DIRECTION ( 'NONE',  ( 0.4635919272833914917, -0.8029647720336136052, 0.3746065934159158450 ) ) ;
#45497=CARTESIAN_POINT ( 'NONE',  ( 81.76532694727032435, 50.08884948260267578, -14.15377366074380738 ) ) ;
#45500=CARTESIAN_POINT ( 'NONE',  ( 20.98410315089673261, 24.06628583063841376, -9.188101187500006262 ) ) ;
#45503=CARTESIAN_POINT ( 'NONE',  ( 13.34262526062736676, 23.10171378149917842, 9.188101187500008038 ) ) ;
#45504=CARTESIAN_POINT ( 'NONE',  ( 66.52392041426838887, 68.84470833973988135, -4.415679280545959706 ) ) ;
#45517=CARTESIAN_POINT ( 'NONE',  ( 77.66033283744638993, 49.34596622033864577, 15.30541677020318936 ) ) ;
#45524=CARTESIAN_POINT ( 'NONE',  ( 79.29599111977559289, 45.69620181558697425, -12.92830799085840177 ) ) ;
#45528=CARTESIAN_POINT ( 'NONE',  ( 19.79331822069313418, 23.37878583063840665, 9.188101187500006262 ) ) ;
#45529=CARTESIAN_POINT ( 'NONE',  ( 75.32210451894222558, 56.33950100161004571, 16.14035722671651030 ) ) ;
#45530=CARTESIAN_POINT ( 'NONE',  ( 68.38740636103155168, 69.72993023537252100, -3.234909568346066244 ) ) ;
#45539=CARTESIAN_POINT ( 'NONE',  ( 67.68417759276564993, 65.75923827970558477, -10.63272006068741682 ) ) ;
#45558=B_SPLINE_CURVE_WITH_KNOTS ( 'NONE', 3,
 ( #83114, #13684, #44557, #83616, #75492, #6077, #36970, #91210, #97152, #98631, #34794, #28704, #50012, #51499, #44388, #90044, #98119, #42877, #97633, #28198, #66213, #59074, #20617, #82468, #35804, #57595, #27718, #4925, #58586, #88576, #96651 ),
 .UNSPECIFIED., .F., .F.,
 ( 4, 3, 3, 3, 3, 3, 3, 3, 3, 3, 4 ),
 ( 0.000000000000000000, 0.1333490885032479201, 0.3007194338854572990, 0.4699862290245473417, 0.5844252810809665855, 0.6686540514502945509, 0.7354980260655585855, 0.8028463152565719074, 0.8633854507757248165, 0.9437142632667163689, 1.000000000000000000 ),
 .UNSPECIFIED. ) ;
#45560=CARTESIAN_POINT ( 'NONE',  ( 66.56339537322608635, 67.82455691954585575, 6.899508657999463779 ) ) ;
#45561=CARTESIAN_POINT ( 'NONE',  ( 6.396987757676594555, 15.64441083166260427, 0.000000000000000000 ) ) ;
#45562=CARTESIAN_POINT ( 'NONE',  ( 84.93732889701342970, 42.42729486305053399, -4.181145052139376261 ) ) ;
#45564=CARTESIAN_POINT ( 'NONE',  ( 67.87358026886720097, 65.44943466354128248, 10.32536289689572584 ) ) ;
#45567=CARTESIAN_POINT ( 'NONE',  ( 87.34055741008818075, 44.89555582937400402, 6.825810004488442218 ) ) ;
#45571=CARTESIAN_POINT ( 'NONE',  ( 76.24518087481982320, 51.59313173972786615, -15.67787985409661111 ) ) ;
#45573=DIRECTION ( 'NONE',  ( 0.7467472232290895962, 0.000000000000000000, -0.6651079495838584377 ) ) ;
#45584=CARTESIAN_POINT ( 'NONE',  ( 72.94747830045673709, 70.90780099059745112, 7.943658523256118542 ) ) ;
#45585=EDGE_CURVE ( 'NONE', #826, #52395, #81735, .T. ) ;
#45590=CARTESIAN_POINT ( 'NONE',  ( 82.44914618329345046, 40.96452554122298295, 1.009388433876072355 ) ) ;
#45595=CARTESIAN_POINT ( 'NONE',  ( 71.08151174896164548, 71.70762546245575209, 0.6123320000693289744 ) ) ;
#45599=CARTESIAN_POINT ( 'NONE',  ( 28.21526782163968861, 21.45404122711134320, -8.090169943749478065 ) ) ;
#45608=CARTESIAN_POINT ( 'NONE',  ( 66.51752898485065657, 67.96052159512244373, -6.582747979517454162 ) ) ;
#45609=CARTESIAN_POINT ( 'NONE',  ( 73.09646855998906290, 70.52920676086053220, -7.962158031461710195 ) ) ;
#45611=CARTESIAN_POINT ( 'NONE',  ( 81.83412826008793672, 41.20383488999954835, 5.740616493571673473 ) ) ;
#45615=CARTESIAN_POINT ( 'NONE',  ( 27.45223038363779722, 27.80066082961423035, 10.00000000000000533 ) ) ;
#45616=CARTESIAN_POINT ( 'NONE',  ( 82.70173759442589301, 41.68243550408067222, -4.153490145786375543 ) ) ;
#45623=CARTESIAN_POINT ( 'NONE',  ( 81.87359138893998534, 41.32955797152818889, 5.976920566253458134 ) ) ;
#45628=CARTESIAN_POINT ( 'NONE',  ( 36.89851624356406745, 36.70171378149922248, -9.188101187500004485 ) ) ;
#45635=CARTESIAN_POINT ( 'NONE',  ( 21.67811977205257890, 27.91421378149918553, 9.188101187500008038 ) ) ;
#45637=CARTESIAN_POINT ( 'NONE',  ( 71.44576612263118420, 59.19700591949954571, 15.77431131436991407 ) ) ;
#45639=VERTEX_POINT ( 'NONE', #38599 ) ;
#45642=CARTESIAN_POINT ( 'NONE',  ( 75.22004289090682505, 53.63718660003009120, -16.53846879587417718 ) ) ;
#45644=CARTESIAN_POINT ( 'NONE',  ( 81.45834803924864786, 41.98143484532695169, 7.684766122967380930 ) ) ;
#45647=CARTESIAN_POINT ( 'NONE',  ( 70.18022655624727690, 70.95232338804223104, -2.456227850087851827 ) ) ;
#45648=CARTESIAN_POINT ( 'NONE',  ( 76.86365259909378267, 63.86390198653350581, 14.89973402578624473 ) ) ;
#45650=EDGE_CURVE ( 'NONE', #41317, #17810, #58694, .T. ) ;
#45657=DIRECTION ( 'NONE',  ( -0.8660254037844378194, -0.5000000000000014433, -0.000000000000000000 ) ) ;
#45658=CARTESIAN_POINT ( 'NONE',  ( 79.86744359784395897, 58.00471593829997374, 16.26723200184080653 ) ) ;
#45659=CARTESIAN_POINT ( 'NONE',  ( 70.69733468835805468, 69.84023709405138902, -7.592114496330573559 ) ) ;
#45661=EDGE_LOOP ( 'NONE', ( #25365, #83982, #12378, #11691 ) ) ;
#45669=FACE_OUTER_BOUND ( 'NONE', #80020, .T. ) ;
#45673=CARTESIAN_POINT ( 'NONE',  ( 78.60735446187601383, 47.91558663937575346, -14.46554739992949834 ) ) ;
#45674=CARTESIAN_POINT ( 'NONE',  ( 30.72385922946222792, 41.23654200823205684, 1.583844403245363353 ) ) ;
#45677=CARTESIAN_POINT ( 'NONE',  ( 72.91150544132388234, 59.06535682740706505, -15.54152198706926313 ) ) ;
#45685=CARTESIAN_POINT ( 'NONE',  ( 70.69181040969623098, 69.05249515714282893, 7.974372502152151654 ) ) ;
#45688=CARTESIAN_POINT ( 'NONE',  ( 66.97592682939898623, 66.94584532911248687, 8.711456034417569327 ) ) ;
#45690=CARTESIAN_POINT ( 'NONE',  ( 78.18706620576766397, 47.52751489781214644, 14.39385552048683437 ) ) ;
#45691=VERTEX_POINT ( 'NONE', #37107 ) ;
#45693=CARTESIAN_POINT ( 'NONE',  ( 71.39380143430086889, 68.16157986366320642, 9.700154972268515863 ) ) ;
#45696=CARTESIAN_POINT ( 'NONE',  ( 79.12912844008201319, 45.88903201271446619, 13.12629439217962357 ) ) ;
#45703=VERTEX_POINT ( 'NONE', #51830 ) ;
#45706=CARTESIAN_POINT ( 'NONE',  ( 72.58623256761462983, 71.41713459486039994, 5.736086548208264801 ) ) ;
#45707=ADVANCED_FACE ( 'NONE', ( #21908 ), #89457, .T. ) ;
#45716=CARTESIAN_POINT ( 'NONE',  ( 82.16888635695728738, 40.69672472932156637, 3.699334420833011450 ) ) ;
#45719=CARTESIAN_POINT ( 'NONE',  ( 74.35485255615375877, 67.94178241879927782, -11.69148233987723806 ) ) ;
#45721=PLANE ( 'NONE',  #38437 ) ;
#45723=CARTESIAN_POINT ( 'NONE',  ( 81.68123830234790717, 41.59537758512663430, -5.490745364427081832 ) ) ;
#45731=CARTESIAN_POINT ( 'NONE',  ( 81.71726183135250210, 47.25007601922910538, -13.05188860062295042 ) ) ;
#45733=CARTESIAN_POINT ( 'NONE',  ( 13.76346889243896321, 13.11029122506292843, -8.090169943749478065 ) ) ;
#45735=CARTESIAN_POINT ( 'NONE',  ( 71.75673953893199553, 59.57128976058874059, -15.71773281170402825 ) ) ;
#45741=CARTESIAN_POINT ( 'NONE',  ( 72.55719605514633486, 57.27873603870379782, 15.85570519528398137 ) ) ;
#45748=CARTESIAN_POINT ( 'NONE',  ( 36.41017387241338810, 23.94754757982092030, 5.678558825948272215 ) ) ;
#45752=CARTESIAN_POINT ( 'NONE',  ( 88.30945731027941292, 43.97049527616571396, 2.452112525173334223 ) ) ;
#45762=CARTESIAN_POINT ( 'NONE',  ( 7.453652514893187586, 19.70171378149916919, -9.188101187500004485 ) ) ;
#45763=ORIENTED_EDGE ( 'NONE', *, *, #2788, .F. ) ;
#45770=CARTESIAN_POINT ( 'NONE',  ( 69.25674720781552196, 70.45917808822757422, 2.199828333335145825 ) ) ;
#45776=CARTESIAN_POINT ( 'NONE',  ( 69.48172542408106267, 66.96606747815684457, 10.45582737889983882 ) ) ;
#45777=CARTESIAN_POINT ( 'NONE',  ( 85.89091867366458644, 45.03324537760627067, -7.686407249209525894 ) ) ;
#45780=CARTESIAN_POINT ( 'NONE',  ( 79.31084698818210654, 59.85625551150463508, -16.50595436643998681 ) ) ;
#45782=CARTESIAN_POINT ( 'NONE',  ( 12.72979851930235107, 19.30066082961420548, -10.00000000000000533 ) ) ;
#45783=CARTESIAN_POINT ( 'NONE',  ( 75.13365046141905168, 53.63593841991193045, -16.54225084687872283 ) ) ;
#45784=CARTESIAN_POINT ( 'NONE',  ( 69.88684495751175518, 62.60609260009564281, 13.43558750483837372 ) ) ;
#45788=CARTESIAN_POINT ( 'NONE',  ( 73.22483582419529569, 69.61542381504622767, -9.909891866396675297 ) ) ;
#45791=B_SPLINE_SURFACE_WITH_KNOTS ( 'NONE', 3, 1, ( 
 ( #72926, #81049 ),
 ( #80540, #88157 ),
 ( #66294, #87672 ),
 ( #42960, #95749 ),
 ( #58183, #73901 ),
 ( #18206, #49099 ),
 ( #18705, #3516 ),
 ( #96233, #19222 ),
 ( #11612, #42471 ),
 ( #4489, #34878 ),
 ( #65778, #89167 ),
 ( #19713, #35382 ),
 ( #27795, #58668 ),
 ( #28277, #36880 ),
 ( #91123, #83523 ),
 ( #53567, #59154 ),
 ( #98204, #15065 ),
 ( #22688, #60159 ),
 ( #68273, #74905 ),
 ( #90124, #83025 ),
 ( #76402, #21688 ),
 ( #5984, #51587 ),
 ( #59667, #7469 ),
 ( #76871, #52567 ),
 ( #5490, #61167 ),
 ( #36372, #13594 ),
 ( #67785, #99196 ),
 ( #67278, #75400 ),
 ( #14589, #82543 ),
 ( #92135, #45467 ),
 ( #44468, #45954 ) ),
 .UNSPECIFIED., .F., .F., .F.,
 ( 4, 3, 3, 3, 3, 3, 3, 3, 3, 3, 4 ),
 ( 2, 2 ),
 ( 0.000000000000000000, 0.1122669598086790121, 0.2243161639709752020, 0.3396355846219183960, 0.4553962076585234553, 0.5677860799922451740, 0.6749047109689819690, 0.7773884377078301711, 0.8775581155834233371, 0.9782364162378153205, 1.000000000000000000 ),
 ( 0.000000000000000000, 1.000000000000000000 ),
 .UNSPECIFIED. ) ;
#45797=CARTESIAN_POINT ( 'NONE',  ( 68.99318464718037092, 69.46180787594425965, 5.229098606639764668 ) ) ;
#45802=CARTESIAN_POINT ( 'NONE',  ( 67.52224811643590385, 68.26499532685183169, -5.959467176383858700 ) ) ;
#45805=CARTESIAN_POINT ( 'NONE',  ( 12.79778405566451482, 30.49540643055186351, 3.479690158560446702E-15 ) ) ;
#45807=CARTESIAN_POINT ( 'NONE',  ( 80.38386138148599969, 57.79680026592915709, 16.59996232260768068 ) ) ;
#45813=CARTESIAN_POINT ( 'NONE',  ( 83.01663263273712801, 45.84489330812576213, -10.66041702595184582 ) ) ;
#45815=EDGE_CURVE ( 'NONE', #57901, #78755, #61029, .T. ) ;
#45819=CARTESIAN_POINT ( 'NONE',  ( 75.07659682177998661, 67.19019193167019921, -13.02721601185334066 ) ) ;
#45826=CARTESIAN_POINT ( 'NONE',  ( 72.05561987901629095, 72.31305038834268828, 0.7486621910535968816 ) ) ;
#45829=CARTESIAN_POINT ( 'NONE',  ( 76.26477717271305323, 65.12336802401900115, 14.59904178568168476 ) ) ;
#45830=DIRECTION ( 'NONE',  ( 0.4493970231495826861, -0.7783784768652872721, -0.4383711467890751834 ) ) ;
#45831=ORIENTED_EDGE ( 'NONE', *, *, #19104, .F. ) ;
#45834=CARTESIAN_POINT ( 'NONE',  ( 67.44257088943838596, 67.25355904234817217, -8.657396272410824878 ) ) ;
#45835=CARTESIAN_POINT ( 'NONE',  ( 85.04155063335291231, 42.38172213771981234, 0.7433201199607106791 ) ) ;
#45837=CARTESIAN_POINT ( 'NONE',  ( 84.17792904279457389, 46.08690578416687345, 10.28387621250127104 ) ) ;
#45843=CARTESIAN_POINT ( 'NONE',  ( 66.26992252404669159, 69.16262777561748010, 2.541374374801295133 ) ) ;
#45849=CARTESIAN_POINT ( 'NONE',  ( 68.76220232199221982, 63.85858675847342880, -12.18730015502817920 ) ) ;
#45858=VERTEX_POINT ( 'NONE', #72024 ) ;
#45862=CARTESIAN_POINT ( 'NONE',  ( 12.32384911305235420, 19.06628583063839955, -9.188101187500006262 ) ) ;
#45865=CARTESIAN_POINT ( 'NONE',  ( 66.03570291327434916, 68.57356300261318438, 1.927684033228001859 ) ) ;
#45871=CARTESIAN_POINT ( 'NONE',  ( 38.02916716989017942, 40.14336893147758900, 7.433330006724141015 ) ) ;
#45875=CARTESIAN_POINT ( 'NONE',  ( 27.19903172117837542, 31.10171378149920329, 9.188101187500008038 ) ) ;
#45888=CARTESIAN_POINT ( 'NONE',  ( 33.05914333415502426, 24.80170272979928470, 7.433330006724137462 ) ) ;
#45894=CARTESIAN_POINT ( 'NONE',  ( 86.35276101173943175, 47.57280788579409148, -10.59090733898761627 ) ) ;
#45896=CARTESIAN_POINT ( 'NONE',  ( 84.95191157424133621, 50.11551264433204267, 13.67402201518260441 ) ) ;
#45900=AXIS2_PLACEMENT_3D ( 'NONE', #79598, #92781, #16248 ) ;
#45902=CARTESIAN_POINT ( 'NONE',  ( 82.90200020812584114, 45.15967755036723474, -10.71970635951677941 ) ) ;
#45903=FACE_OUTER_BOUND ( 'NONE', #62400, .T. ) ;
#45917=CARTESIAN_POINT ( 'NONE',  ( 74.94965141288585642, 60.80520178593948799, -15.45531043546616878 ) ) ;
#45920=CARTESIAN_POINT ( 'NONE',  ( 76.90757676121016573, 64.01000647765765450, -15.22607040013521029 ) ) ;
#45926=CARTESIAN_POINT ( 'NONE',  ( 40.42517716772906056, 31.84335787977767041, 9.188101187500006262 ) ) ;
#45932=CARTESIAN_POINT ( 'NONE',  ( 70.23932605309654775, 64.16367945268753203, -12.59136813384165166 ) ) ;
#45935=CARTESIAN_POINT ( 'NONE',  ( 30.05030659499110968, 29.30066082961423746, -10.00000000000000533 ) ) ;
#45953=CARTESIAN_POINT ( 'NONE',  ( 73.45867522032249042, 68.92373273176619364, 10.23420689778941473 ) ) ;
#45954=CARTESIAN_POINT ( 'NONE',  ( 82.41630873631589793, 41.31828431233921606, -3.367117793111293889 ) ) ;
#45962=CARTESIAN_POINT ( 'NONE',  ( 73.75605216947923282, 65.80208602379973115, -13.43874901075588824 ) ) ;
#45967=CARTESIAN_POINT ( 'NONE',  ( 66.54075137518580618, 68.81555626029071959, -2.231460399992863497 ) ) ;
#45970=CARTESIAN_POINT ( 'NONE',  ( 78.56719005003022005, 47.98515344134877836, 13.96283253221395704 ) ) ;
#45971=CARTESIAN_POINT ( 'NONE',  ( 73.30483403957811106, 69.17932697374330075, -9.895411455429709235 ) ) ;
#45972=CARTESIAN_POINT ( 'NONE',  ( 75.98104421115762364, 51.53574906944388800, 16.18761828526978164 ) ) ;
#45976=CARTESIAN_POINT ( 'NONE',  ( 71.81503955391033855, 71.89711284198503449, 2.894600326227580567 ) ) ;
#45987=CARTESIAN_POINT ( 'NONE',  ( 20.27082849090286842, 27.10171378149918908, 9.188101187500008038 ) ) ;
#45990=CARTESIAN_POINT ( 'NONE',  ( 14.76917458061509514, 17.03085787977762067, 9.188101187500006262 ) ) ;
#45993=CARTESIAN_POINT ( 'NONE',  ( 79.17632907059281422, 57.86865562274022068, -16.61182437452083249 ) ) ;
#45998=CARTESIAN_POINT ( 'NONE',  ( 74.34271649381057046, 57.05639872568476534, -16.02907805139209074 ) ) ;
#46003=ORIENTED_EDGE ( 'NONE', *, *, #16470, .T. ) ;
#46004=CARTESIAN_POINT ( 'NONE',  ( 76.91861570892473310, 49.78243787368231921, 15.09545489314607281 ) ) ;
#46013=CARTESIAN_POINT ( 'NONE',  ( 79.19750788024767019, 46.06220688912179639, -13.21515928786401695 ) ) ;
#46015=CARTESIAN_POINT ( 'NONE',  ( 87.10572595599398937, 44.47484308406081510, 6.276395280311344749 ) ) ;
#46016=DIRECTION ( 'NONE',  ( 0.000000000000000000, 0.7457702847286276082, 0.6662031840330557841 ) ) ;
#46017=VERTEX_POINT ( 'NONE', #5599 ) ;
#46018=CARTESIAN_POINT ( 'NONE',  ( 16.80975711337266176, 31.74646525600390135, 2.839279412974139660 ) ) ;
#46019=CARTESIAN_POINT ( 'NONE',  ( 75.03770635709581427, 55.01706581963784259, 16.14491965273878904 ) ) ;
#46030=CARTESIAN_POINT ( 'NONE',  ( 67.80572549195380816, 65.59792567543669861, -10.86872875137217243 ) ) ;
#46047=ORIENTED_EDGE ( 'NONE', *, *, #42284, .F. ) ;
#46051=CARTESIAN_POINT ( 'NONE',  ( 66.87684795978640295, 67.53304424843219067, 6.646635947192834237 ) ) ;
#46056=CARTESIAN_POINT ( 'NONE',  ( 70.35440405002556474, 63.74960742650419121, 12.91260164709814084 ) ) ;
#46062=ORIENTED_EDGE ( 'NONE', *, *, #61273, .T. ) ;
#46072=CARTESIAN_POINT ( 'NONE',  ( 83.09294558526256935, 43.66384112246667826, -7.909259972356729840 ) ) ;
#46078=CARTESIAN_POINT ( 'NONE',  ( 79.49298289701215481, 59.22797875817073532, -16.22298816110328445 ) ) ;
#46079=CARTESIAN_POINT ( 'NONE',  ( 68.91844246388177453, 67.43096903599641223, -8.746045204043648269 ) ) ;
#46085=CARTESIAN_POINT ( 'NONE',  ( 83.90995141641640487, 51.89037297248786018, 14.88406197085304150 ) ) ;
#46093=CARTESIAN_POINT ( 'NONE',  ( 74.05984977965144367, 55.09172014556617114, 16.60385058087775434 ) ) ;
#46094=CARTESIAN_POINT ( 'NONE',  ( 22.68382546022871438, 31.83478043621389020, -8.090169943749479842 ) ) ;
#46103=CARTESIAN_POINT ( 'NONE',  ( 72.67905965592417772, 70.26320000030698054, -8.002569769838697056 ) ) ;
#46107=CARTESIAN_POINT ( 'NONE',  ( 76.96225540874074511, 63.35506444885830035, -15.47139205492574554 ) ) ;
#46108=CARTESIAN_POINT ( 'NONE',  ( 24.08258844821711264, 36.83705186507755514, 3.090169943749475401 ) ) ;
#46111=DIRECTION ( 'NONE',  ( 0.8660254037844379305, 0.5000000000000014433, 0.000000000000000000 ) ) ;
#46116=CARTESIAN_POINT ( 'NONE',  ( 44.67827877960949223, 26.76426979415094110, 3.090169943749476733 ) ) ;
#46119=CARTESIAN_POINT ( 'NONE',  ( 66.45982511243997237, 67.83556696074005288, 6.764132809977054350 ) ) ;
#46120=CARTESIAN_POINT ( 'NONE',  ( 36.98912467918979274, 21.75978393459167393, -1.583844403245396437 ) ) ;
#46121=CARTESIAN_POINT ( 'NONE',  ( 77.16105698610837749, 49.60253137911669796, -14.98352156587448114 ) ) ;
#46130=CARTESIAN_POINT ( 'NONE',  ( 26.78885238572174998, 16.26216523072495690, -2.296566073217252530E-15 ) ) ;
#46132=CARTESIAN_POINT ( 'NONE',  ( 71.40067601551650966, 59.33978977576644098, 15.72537452617927478 ) ) ;
#46135=CARTESIAN_POINT ( 'NONE',  ( 6.802937163926562114, 15.87878583063839066, -9.188101187500006262 ) ) ;
#46137=CARTESIAN_POINT ( 'NONE',  ( 81.64627816295647733, 42.63038875969535724, 7.551097713807430445 ) ) ;
#46141=CARTESIAN_POINT ( 'NONE',  ( 72.57727468335085064, 71.31820506079068878, -5.984807345722121141 ) ) ;
#46142=CARTESIAN_POINT ( 'NONE',  ( 76.78727678290111669, 63.87399086453137187, 14.88032377382801030 ) ) ;
#46148=CARTESIAN_POINT ( 'NONE',  ( 85.27848080570771572, 42.86259319836502613, -3.223099939885945453 ) ) ;
#46151=CARTESIAN_POINT ( 'NONE',  ( 21.80251038182309031, 34.36126292948896577, 6.180339887498949913 ) ) ;
#46152=CARTESIAN_POINT ( 'NONE',  ( 80.03994542435373205, 57.65115798690544580, 16.60126445886218249 ) ) ;
#46168=CARTESIAN_POINT ( 'NONE',  ( 31.01079167849261964, 40.83705186507756224, 3.090169943749475401 ) ) ;
#46172=CARTESIAN_POINT ( 'NONE',  ( 86.97134532988273747, 46.47825607565307138, 8.944163774166895564 ) ) ;
#46173=CARTESIAN_POINT ( 'NONE',  ( 82.50043972687433325, 42.71205652650662188, -6.855908010978745359 ) ) ;
#46183=CARTESIAN_POINT ( 'NONE',  ( 67.56897137201481485, 70.11578694084727204, 0.8315581512064480485 ) ) ;
#46184=CARTESIAN_POINT ( 'NONE',  ( 67.17708281894157096, 66.61742757574968721, 8.430827746126428934 ) ) ;
#46185=CARTESIAN_POINT ( 'NONE',  ( 72.64749865597310929, 65.05606228103368949, -12.97249523173932317 ) ) ;
#46186=CARTESIAN_POINT ( 'NONE',  ( 78.12916722883838361, 47.65424050001094969, 14.47278094148724747 ) ) ;
#46191=CARTESIAN_POINT ( 'NONE',  ( 82.53859975423060291, 41.16651341379471774, -2.370924961068094028 ) ) ;
#46194=CARTESIAN_POINT ( 'NONE',  ( 78.88871661031990357, 46.37012301642865708, 12.94053771451172352 ) ) ;
#46200=CARTESIAN_POINT ( 'NONE',  ( 72.27003297432077034, 71.75159315020286499, 5.546042747704616360 ) ) ;
#46211=CARTESIAN_POINT ( 'NONE',  ( 71.03260519239540827, 63.40884879191646917, 13.38662637038426162 ) ) ;
#46212=CARTESIAN_POINT ( 'NONE',  ( 88.07640460957951234, 44.67800788684087365, -4.250388008292100395 ) ) ;
#46216=DIRECTION ( 'NONE',  ( -0.3473291852295006810, 0.6015917957689992379, 0.7193398003386451967 ) ) ;
#46223=CARTESIAN_POINT ( 'NONE',  ( 80.76073326117044360, 47.44888180215133389, -13.52495504245785796 ) ) ;
#46226=CARTESIAN_POINT ( 'NONE',  ( 13.59582392308679033, 19.80066082961420548, 10.00000000000000533 ) ) ;
#46229=CARTESIAN_POINT ( 'NONE',  ( 75.20389695419315501, 52.88180760346911313, -15.99093876381489920 ) ) ;
#46233=CARTESIAN_POINT ( 'NONE',  ( 73.08053648531546287, 57.27840619054814653, 15.90006795040070564 ) ) ;
#46235=CARTESIAN_POINT ( 'NONE',  ( 66.61202643439548865, 68.34816216382951382, -4.339165927432250491 ) ) ;
#46236=VERTEX_POINT ( 'NONE', #65772 ) ;
#46241=CARTESIAN_POINT ( 'NONE',  ( 25.24689923506580769, 37.68290643055188838, 3.479690158560446702E-15 ) ) ;
#46245=EDGE_CURVE ( 'NONE', #95962, #90569, #25808, .T. ) ;
#46246=CARTESIAN_POINT ( 'NONE',  ( 68.81692840119013965, 68.11752969850674333, 8.558253326585221643 ) ) ;
#46248=CARTESIAN_POINT ( 'NONE',  ( 68.45038622130651618, 64.39200674863153040, 12.27119139371030876 ) ) ;
#46253=CARTESIAN_POINT ( 'NONE',  ( 8.064688198948626763, 22.84336893147754211, -7.433330006724137462 ) ) ;
#46268=CARTESIAN_POINT ( 'NONE',  ( 72.94255135865869022, 70.82539339859251015, 7.334897578941317775 ) ) ;
#46271=CARTESIAN_POINT ( 'NONE',  ( 17.37407021781635663, 33.52903772873357013, -1.583844403245363575 ) ) ;
#46272=CARTESIAN_POINT ( 'NONE',  ( 82.67802903814479976, 45.32635663605926624, -10.34136681600037022 ) ) ;
#46275=CARTESIAN_POINT ( 'NONE',  ( 79.32566820500106530, 59.73991648520960496, -16.51753030644416498 ) ) ;
#46277=CARTESIAN_POINT ( 'NONE',  ( 69.78819819425497428, 62.70547683012449625, 13.91779829744284314 ) ) ;
#46282=CARTESIAN_POINT ( 'NONE',  ( 81.47153209085804804, 42.18456630836416110, -8.000817679882061384 ) ) ;
#46286=CARTESIAN_POINT ( 'NONE',  ( 74.34779163019582882, 65.75635227628464463, 13.22858955973211970 ) ) ;
#46288=CARTESIAN_POINT ( 'NONE',  ( 70.29083157674634208, 70.92442123829498257, 3.057200561768157687 ) ) ;
#46292=CARTESIAN_POINT ( 'NONE',  ( 83.82827945288542537, 51.88092520783234818, 14.50189114860043205 ) ) ;
#46296=B_SPLINE_CURVE_WITH_KNOTS ( 'NONE', 3,
 ( #42425, #82979, #52040, #58620, #28741, #13554, #5937, #27255, #58138, #66733, #5446, #81983, #73358, #89595, #20160, #88609, #81486, #89118, #81001, #12557, #3946, #43431, #4439, #98664, #4958, #42910, #59617, #35839, #34829, #97666, #28234, #13065, #90082, #73851, #44427, #20650, #21159, #90595, #75356, #36831, #67740, #65730, #29246, #19176, #96685, #6924 ),
 .UNSPECIFIED., .F., .F.,
 ( 4, 1, 1, 1, 2, 2, 1, 1, 1, 2, 2, 1, 1, 2, 2, 1, 1, 2, 2, 1, 1, 2, 2, 1, 2, 2, 1, 2, 2, 4 ),
 ( 0.000000000000000000, 0.06249999999997736533, 0.09374999999996795619, 0.1093749999999633349, 0.1171874999999610173, 0.1249999999999586997, 0.1874999999999466260, 0.2187499999999406863, 0.2343749999999379663, 0.2421874999999366063, 0.2499999999999352185, 0.3124999999999348854, 0.3437499999999346634, 0.3593749999999363842, 0.3749999999999381051, 0.4374999999999475420, 0.4687499999999538147, 0.4843749999999565348, 0.4999999999999592548, 0.5624999999999614753, 0.5937499999999609201, 0.6093749999999625855, 0.6249999999999642508, 0.6874999999999723554, 0.7187499999999767963, 0.7499999999999812372, 0.8124999999999902300, 0.8437499999999923395, 0.8749999999999944489, 1.000000000000000000 ),
 .UNSPECIFIED. ) ;
#46297=CARTESIAN_POINT ( 'NONE',  ( 82.62542648728522465, 54.14492212412226024, -15.90696914271030238 ) ) ;
#46299=CARTESIAN_POINT ( 'NONE',  ( 79.88009824201490972, 55.32498818933279949, -16.43691830321638747 ) ) ;
#46300=CARTESIAN_POINT ( 'NONE',  ( 14.59716579798650571, 20.37878583063839955, 9.188101187500006262 ) ) ;
#46303=CARTESIAN_POINT ( 'NONE',  ( 80.35079170152107508, 57.80872192622026517, 16.60075256504292796 ) ) ;
#46308=CARTESIAN_POINT ( 'NONE',  ( 44.85148386036637191, 26.86426979415093541, -3.090169943749474069 ) ) ;
#46309=CARTESIAN_POINT ( 'NONE',  ( 77.23415525214731758, 49.64680416525870044, -15.49634504973622562 ) ) ;
#46310=SHAPE_REPRESENTATION ( 'Center Base Mounting Screw', ( #68784 ), #26785 ) ;
#46325=CARTESIAN_POINT ( 'NONE',  ( 72.55393231385352237, 70.87694079910581024, 7.622851120052400731 ) ) ;
#46330=AXIS2_PLACEMENT_3D ( 'NONE', #24558, #54955, #47355 ) ;
#46334=CARTESIAN_POINT ( 'NONE',  ( 85.28648675625211695, 46.08015217243080031, -9.601151076074931012 ) ) ;
#46336=B_SPLINE_CURVE_WITH_KNOTS ( 'NONE', 3,
 ( #85364, #23498, #47308, #93961, #31104, #77739, #71137, #40703, #54388, #24013, #32105, #61992, #78732, #24513, #92460, #23005, #38707, #48324, #1740, #32619, #55392, #40196, #15911, #8324, #46815, #15398, #54909, #77221, #100040, #53898, #94454, #63516, #39189, #9322, #25009, #17414, #70103, #79269, #86379, #70611, #93458, #92944, #8815, #9842, #62491, #46292 ),
 .UNSPECIFIED., .F., .F.,
 ( 4, 1, 1, 1, 2, 2, 1, 1, 1, 2, 2, 1, 1, 2, 2, 1, 1, 2, 2, 1, 1, 2, 2, 1, 2, 2, 1, 2, 2, 4 ),
 ( 0.000000000000000000, 0.06250000000000717482, 0.09375000000001090794, 0.1093750000000126149, 0.1171875000000136141, 0.1250000000000146272, 0.1875000000000213163, 0.2187500000000239531, 0.2343750000000244804, 0.2421875000000247580, 0.2500000000000249800, 0.3125000000000254796, 0.3437500000000270339, 0.3593750000000276446, 0.3750000000000282552, 0.4375000000000335842, 0.4687500000000353606, 0.4843750000000357492, 0.5000000000000360822, 0.5625000000000328626, 0.5937500000000315303, 0.6093750000000305311, 0.6250000000000295319, 0.6875000000000242029, 0.7187500000000208722, 0.7500000000000175415, 0.8125000000000122125, 0.8437500000000094369, 0.8750000000000067724, 1.000000000000000000 ),
 .UNSPECIFIED. ) ;
#46337=LINE ( 'NONE', #77260, #85160 ) ;
#46338=CARTESIAN_POINT ( 'NONE',  ( 82.38813812040005757, 42.78134201135360115, 7.123226640718979930 ) ) ;
#46342=DIRECTION ( 'NONE',  ( -0.3297783986044553473, -0.8484238185761712181, 0.4140328874455617147 ) ) ;
#46347=CARTESIAN_POINT ( 'NONE',  ( 29.70092825881656751, 40.08080186712595605, -3.090169943749475845 ) ) ;
#46351=CARTESIAN_POINT ( 'NONE',  ( 81.38957022129915231, 44.58922959300493716, 11.03339234182588413 ) ) ;
#46356=CARTESIAN_POINT ( 'NONE',  ( 69.40468783160719113, 69.42147328788952620, 5.860110772957342284 ) ) ;
#46360=CARTESIAN_POINT ( 'NONE',  ( 74.07655054661930194, 57.25575122610550949, 16.47418694559453556 ) ) ;
#46363=CARTESIAN_POINT ( 'NONE',  ( 18.23327619575285041, 19.03085787977762067, 9.188101187500006262 ) ) ;
#46365=CARTESIAN_POINT ( 'NONE',  ( 77.75856728979914578, 57.69604372946123050, -16.59626237126559900 ) ) ;
#46371=DIRECTION ( 'NONE',  ( 0.9364604334398963781, -0.2023802897980917226, -0.2865031848039421014 ) ) ;
#46373=CARTESIAN_POINT ( 'NONE',  ( 86.15627751966195547, 47.68681392592237955, 10.83869660506637089 ) ) ;
#46376=CARTESIAN_POINT ( 'NONE',  ( 30.51038259252555207, 29.56628583063842441, 9.188101187500006262 ) ) ;
#46383=EDGE_CURVE ( 'NONE', #7164, #5821, #12052, .T. ) ;
#46384=VECTOR ( 'NONE', #6209, 1000.000000000000000 ) ;
#46386=CARTESIAN_POINT ( 'NONE',  ( 79.06941788075492639, 49.65996601992884507, 14.60823914099390919 ) ) ;
#46389=LINE ( 'NONE', #39282, #76023 ) ;
#46392=EDGE_LOOP ( 'NONE', ( #38136, #52147, #58028, #52640 ) ) ;
#46395=CARTESIAN_POINT ( 'NONE',  ( 37.18115723113500337, 22.26216523072496400, -2.296566073217252530E-15 ) ) ;
#46401=CARTESIAN_POINT ( 'NONE',  ( 86.53662601515709696, 47.28685775360474253, -10.20020400134509408 ) ) ;
#46403=CARTESIAN_POINT ( 'NONE',  ( 84.51504024060453446, 50.21520769139153373, 13.87897165174792846 ) ) ;
#46407=CARTESIAN_POINT ( 'NONE',  ( 42.15722797529793553, 32.84335787977767041, 9.188101187500006262 ) ) ;
#46427=CARTESIAN_POINT ( 'NONE',  ( 42.00264329202813229, 26.11110640527295601, -2.839279412974138328 ) ) ;
#46430=CARTESIAN_POINT ( 'NONE',  ( 73.98570270871887544, 68.92876820612472955, -11.10152750440661862 ) ) ;
#46431=CARTESIAN_POINT ( 'NONE',  ( 75.56481254617771981, 62.80431594364750936, -14.94990648061137328 ) ) ;
#46434=CARTESIAN_POINT ( 'NONE',  ( 72.24607194888514528, 62.62084493799169138, 14.18516964437414352 ) ) ;
#46435=CARTESIAN_POINT ( 'NONE',  ( 66.73387148584731676, 68.35900400491371443, 4.521128723796655535 ) ) ;
#46437=ORIENTED_EDGE ( 'NONE', *, *, #34876, .T. ) ;
#46438=CARTESIAN_POINT ( 'NONE',  ( 36.61341721041482344, 22.10801979619931501, 3.090169943749476733 ) ) ;
#46456=CARTESIAN_POINT ( 'NONE',  ( 73.01434170154392689, 67.59968775764829729, 11.23568329902283125 ) ) ;
#46462=CARTESIAN_POINT ( 'NONE',  ( 83.50657803916486444, 43.71961979256885655, 7.634715688034919623 ) ) ;
#46466=CARTESIAN_POINT ( 'NONE',  ( 70.47935399718505778, 60.87681273810773064, -14.99835320260665306 ) ) ;
#46467=CARTESIAN_POINT ( 'NONE',  ( 75.63268008801900066, 65.14737934564519151, -14.41129995628930516 ) ) ;
#46475=CARTESIAN_POINT ( 'NONE',  ( 84.78922593834768406, 50.40041394048158452, -13.47278310779192623 ) ) ;
#46479=CARTESIAN_POINT ( 'NONE',  ( 75.97679052025780777, 51.38226631630038810, 16.15713118531126469 ) ) ;
#46484=CARTESIAN_POINT ( 'NONE',  ( 71.64065041137482126, 72.08859242525181799, 3.376608021325395725 ) ) ;
#46489=CARTESIAN_POINT ( 'NONE',  ( 70.62955678152276562, 60.80479719363771807, -15.06269029744276011 ) ) ;
#46490=CARTESIAN_POINT ( 'NONE',  ( 88.31734708748101070, 44.16587181541018481, 0.3721755419053404124 ) ) ;
#46494=CARTESIAN_POINT ( 'NONE',  ( 32.30976433484754295, 19.44966523072496045, -2.296566073217252530E-15 ) ) ;
#46495=DIRECTION ( 'NONE',  ( 0.5000000000000014433, -0.8660254037844378194, 0.000000000000000000 ) ) ;
#46496=CARTESIAN_POINT ( 'NONE',  ( 80.85352406992397789, 47.50882711102294564, -12.96424570248204944 ) ) ;
#46497=CARTESIAN_POINT ( 'NONE',  ( 10.20631340951632104, 27.93396525600388713, 2.839279412974139660 ) ) ;
#46499=CARTESIAN_POINT ( 'NONE',  ( 77.32817876982274186, 63.13942984521013813, 15.61058464551961933 ) ) ;
#46500=CARTESIAN_POINT ( 'NONE',  ( 82.60582504534620796, 54.05721848903051807, -15.51501040363680772 ) ) ;
#46504=EDGE_CURVE ( 'NONE', #66013, #64000, #99824, .T. ) ;
#46510=CARTESIAN_POINT ( 'NONE',  ( 77.55434755293194371, 49.25411156172739879, 15.29420696795023993 ) ) ;
#46511=CARTESIAN_POINT ( 'NONE',  ( 82.73238768416140942, 53.97435551261711595, 15.47794029334955290 ) ) ;
#46515=CARTESIAN_POINT ( 'NONE',  ( 71.60825314380221585, 68.87726608393772665, -8.959588779531696190 ) ) ;
#46516=EDGE_CURVE ( 'NONE', #39570, #71517, #86597, .T. ) ;
#46517=ORIENTED_EDGE ( 'NONE', *, *, #32855, .F. ) ;
#46520=CARTESIAN_POINT ( 'NONE',  ( 79.47501604884325843, 46.39112505788885699, -12.72631656372365327 ) ) ;
#46524=CARTESIAN_POINT ( 'NONE',  ( 22.11595037535113661, 30.95586893147756413, 7.433330006724141015 ) ) ;
#46525=CARTESIAN_POINT ( 'NONE',  ( 75.35044267779828431, 56.47610766855712683, 16.13648771087090950 ) ) ;
#46527=CARTESIAN_POINT ( 'NONE',  ( 74.86346538573357634, 67.47285165321517297, -12.74145591711592296 ) ) ;
#46528=VERTEX_POINT ( 'NONE', #64647 ) ;
#46534=CARTESIAN_POINT ( 'NONE',  ( 68.07754589302088277, 65.45337442352710866, 10.44018349253913946 ) ) ;
#46535=CARTESIAN_POINT ( 'NONE',  ( 67.93659143534979705, 65.44611157119403799, -10.36544933898279552 ) ) ;
#46553=ORIENTED_EDGE ( 'NONE', *, *, #64872, .F. ) ;
#46555=CARTESIAN_POINT ( 'NONE',  ( 66.87731416404506035, 67.95854068482356070, 6.988359128739752180 ) ) ;
#46558=LINE ( 'NONE', #68864, #33688 ) ;
#46559=CARTESIAN_POINT ( 'NONE',  ( 77.79060403590699480, 49.02752842191024030, -14.64657546086520590 ) ) ;
#46566=ORIENTED_EDGE ( 'NONE', *, *, #93120, .F. ) ;
#46567=CARTESIAN_POINT ( 'NONE',  ( 76.36355602522917252, 51.65656375226136987, -16.16753059234807566 ) ) ;
#46568=CARTESIAN_POINT ( 'NONE',  ( 76.25827818320625795, 65.17332737998212622, -14.17717953946896436 ) ) ;
#46575=CARTESIAN_POINT ( 'NONE',  ( 83.28364122651360901, 43.66763108505107027, -7.749604338574708429 ) ) ;
#46578=CARTESIAN_POINT ( 'NONE',  ( 33.51440821012886317, 31.30066082961424456, -10.00000000000000533 ) ) ;
#46580=CARTESIAN_POINT ( 'NONE',  ( 72.45510692969175182, 70.78848362686431983, 7.675293421552856543 ) ) ;
#46581=PLANE ( 'NONE',  #85885 ) ;
#46586=VECTOR ( 'NONE', #81579, 1000.000000000000114 ) ;
#46598=CARTESIAN_POINT ( 'NONE',  ( 73.95246095525199337, 55.20797954095843352, 16.12289266927081854 ) ) ;
#46601=CARTESIAN_POINT ( 'NONE',  ( 24.67798091686682938, 37.18080186712595037, 3.090169943749475401 ) ) ;
#46605=CARTESIAN_POINT ( 'NONE',  ( 67.69237348538018750, 66.82088825431439716, 8.559571887000263501 ) ) ;
#46613=CARTESIAN_POINT ( 'NONE',  ( 73.10686818167350509, 70.63172961811761752, -7.803365976151034111 ) ) ;
#46617=CARTESIAN_POINT ( 'NONE',  ( 77.08262651433446422, 63.62497865693946153, -15.40261155718560815 ) ) ;
#46619=CARTESIAN_POINT ( 'NONE',  ( 26.78025984663613457, 31.16454794089042224, -10.00000000000000355 ) ) ;
#46620=CARTESIAN_POINT ( 'NONE',  ( 82.65091073267497279, 41.67014845218071173, -4.206092679686253888 ) ) ;
#46622=CARTESIAN_POINT ( 'NONE',  ( 81.25383428119911855, 56.17809469613565909, 16.10000759051138175 ) ) ;
#46624=EDGE_CURVE ( 'NONE', #81636, #46528, #58517, .T. ) ;
#46626=CARTESIAN_POINT ( 'NONE',  ( 83.96886348723032256, 46.13120489799907631, 11.07011704621705128 ) ) ;
#46627=CARTESIAN_POINT ( 'NONE',  ( 84.07404364193551771, 51.51966214638420638, 14.67759748506154338 ) ) ;
#46631=CARTESIAN_POINT ( 'NONE',  ( 36.46445469440066489, 39.79103043416552055, 8.090169943749478065 ) ) ;
#46639=DIRECTION ( 'NONE',  ( -0.8660254037844377084, -0.5000000000000014433, -0.000000000000000000 ) ) ;
#46645=CARTESIAN_POINT ( 'NONE',  ( 23.10466909204031083, 21.84335787977762777, 9.188101187500006262 ) ) ;
#46647=CARTESIAN_POINT ( 'NONE',  ( 71.55582279638187515, 59.08747183676958770, 15.82285513313428105 ) ) ;
#46650=CARTESIAN_POINT ( 'NONE',  ( 11.99908958663318970, 18.87878583063839955, -9.188101187500006262 ) ) ;
#46651=EDGE_CURVE ( 'NONE', #68627, #30181, #33239, .T. ) ;
#46652=CARTESIAN_POINT ( 'NONE',  ( 73.06697666995047769, 59.88521403644757868, -15.37108490149400275 ) ) ;
#46653=CARTESIAN_POINT ( 'NONE',  ( 88.22316733864592209, 44.26875609612613971, 2.029272769359137474 ) ) ;
#46658=CARTESIAN_POINT ( 'NONE',  ( 77.22649460905378760, 63.31555197798695644, 15.15381191669832184 ) ) ;
#46659=CARTESIAN_POINT ( 'NONE',  ( 86.45920310846531720, 44.18811037999328306, 6.432687887546634009 ) ) ;
#46661=EDGE_LOOP ( 'NONE', ( #34206, #43696, #19328, #16624 ) ) ;
#46664=CARTESIAN_POINT ( 'NONE',  ( 82.38352151192086126, 42.31992766688023977, -6.241314886312054888 ) ) ;
#46669=CARTESIAN_POINT ( 'NONE',  ( 72.92091214766469420, 56.78235363556951398, -15.96102170641831819 ) ) ;
#46670=CARTESIAN_POINT ( 'NONE',  ( 3.540199675970839177, 23.81751292744053927, -6.180339887498951690 ) ) ;
#46680=CARTESIAN_POINT ( 'NONE',  ( 33.71705561599726053, 20.26216523072496045, -2.296566073217252530E-15 ) ) ;
#46687=CARTESIAN_POINT ( 'NONE',  ( 83.50150581922116544, 52.39864595077343523, 14.81182293697902530 ) ) ;
#46700=CARTESIAN_POINT ( 'NONE',  ( 69.89728461977614415, 67.46325532689361637, 9.448739956629149006 ) ) ;
#46701=AXIS2_PLACEMENT_3D ( 'NONE', #64062, #56454, #87446 ) ;
#46704=CARTESIAN_POINT ( 'NONE',  ( 69.62290603085084228, 65.57344325233756877, -11.19888540440396696 ) ) ;
#46705=CARTESIAN_POINT ( 'NONE',  ( 78.50823532819325123, 47.87735602650093369, 13.92489207041279897 ) ) ;
#46713=CARTESIAN_POINT ( 'NONE',  ( 83.61062943468348863, 51.62670160475642689, -14.84472182808584328 ) ) ;
#46716=FACE_OUTER_BOUND ( 'NONE', #38934, .T. ) ;
#46717=CARTESIAN_POINT ( 'NONE',  ( 72.11862359525288468, 71.68643115293319568, 5.491312638656053124 ) ) ;
#46718=CARTESIAN_POINT ( 'NONE',  ( 74.65352423280955918, 67.09549399619112364, 12.48430392623164309 ) ) ;
#46726=CARTESIAN_POINT ( 'NONE',  ( 85.68890431086639126, 48.40205047417678230, -11.72463670400526325 ) ) ;
#46728=CARTESIAN_POINT ( 'NONE',  ( 71.19401572595349137, 63.93336477220826453, 13.13347857285084785 ) ) ;
#46729=CARTESIAN_POINT ( 'NONE',  ( 87.83581743205598968, 44.43730844317693141, -3.939890015914216725 ) ) ;
#46731=CARTESIAN_POINT ( 'NONE',  ( 73.46955079657830368, 61.49715917090933459, 15.42325390693441456 ) ) ;
#46732=ADVANCED_FACE ( 'NONE', ( #96072 ), #36858, .T. ) ;
#46748=AXIS2_PLACEMENT_3D ( 'NONE', #69725, #1340, #94072 ) ;
#46749=CARTESIAN_POINT ( 'NONE',  ( 14.26779446008844410, 16.43677371833800294, -10.00000000000000355 ) ) ;
#46752=CARTESIAN_POINT ( 'NONE',  ( 73.13496796734084171, 69.72571060213493865, 9.125874619874972282 ) ) ;
#46756=CARTESIAN_POINT ( 'NONE',  ( 73.11532976057090139, 57.21814247004398624, 16.39520198499102932 ) ) ;
#46758=CARTESIAN_POINT ( 'NONE',  ( 66.64344042913042188, 68.36362187625169895, -4.347781399904284250 ) ) ;
#46759=ORIENTED_EDGE ( 'NONE', *, *, #77623, .F. ) ;
#46765=CARTESIAN_POINT ( 'NONE',  ( 28.23826220571969969, 31.70171378149920471, -9.188101187500004485 ) ) ;
#46770=CARTESIAN_POINT ( 'NONE',  ( 88.48864216585432985, 44.00423028902886813, 2.007554169862328486 ) ) ;
#46772=CARTESIAN_POINT ( 'NONE',  ( 66.30941063773362032, 69.19462254233461351, 2.488570590289448159 ) ) ;
#46773=ORIENTED_EDGE ( 'NONE', *, *, #15155, .F. ) ;
#46778=CARTESIAN_POINT ( 'NONE',  ( 16.58301002715608519, 15.28920272979925876, -7.433330006724141015 ) ) ;
#46782=B_SPLINE_CURVE_WITH_KNOTS ( 'NONE', 3,
 ( #71089, #63469, #86831, #65959, #89325, #19879, #11784, #4155, #8377, #39243, #70153, #23549, #38760, #84412, #7364, #16959, #62044, #32164, #61560, #77792, #54442, #85418, #8868, #763 ),
 .UNSPECIFIED., .F., .F.,
 ( 4, 2, 2, 2, 2, 2, 2, 2, 2, 2, 2, 4 ),
 ( 0.000000000000000000, 0.1249999999999867051, 0.2499999999999734102, 0.3749999999999601430, 0.4374999999999588662, 0.4999999999999575895, 0.5624999999999563682, 0.6249999999999551470, 0.6874999999999539257, 0.7499999999999527045, 0.8749999999999764633, 1.000000000000000000 ),
 .UNSPECIFIED. ) ;
#46793=B_SPLINE_CURVE_WITH_KNOTS ( 'NONE', 3,
 ( #13560, #74869, #81492, #5451, #36336, #67237, #75365, #12061, #5944, #36838, #98671, #77338, #55020, #38320, #23611, #14551, #7946, #37821, #39799, #69228, #62110, #86001, #70223, #16527, #47424, #78350, #31708, #61119, #8933, #38820, #30239 ),
 .UNSPECIFIED., .F., .F.,
 ( 4, 3, 3, 3, 3, 3, 3, 3, 3, 3, 4 ),
 ( 0.000000000000000000, 0.1333490885032394824, 0.3007194338854430882, 0.4699862290245251373, 0.5844252810809388299, 0.6686540514502711252, 0.7354980260655488156, 0.8028463152565757932, 0.8633854507757249275, 0.9437142632667384623, 1.000000000000000000 ),
 .UNSPECIFIED. ) ;
#46798=CARTESIAN_POINT ( 'NONE',  ( 81.09808841527535606, 45.53856527529837450, -11.38469005618299335 ) ) ;
#46801=CARTESIAN_POINT ( 'NONE',  ( 79.49673530597218019, 59.23457754060601133, -16.22261858990263761 ) ) ;
#46803=EDGE_LOOP ( 'NONE', ( #29470, #89046, #58642, #54748 ) ) ;
#46807=VERTEX_POINT ( 'NONE', #23999 ) ;
#46809=ORIENTED_EDGE ( 'NONE', *, *, #65690, .T. ) ;
#46810=CARTESIAN_POINT ( 'NONE',  ( 79.76359975193354046, 44.98417069036879923, 11.54310746654911846 ) ) ;
#46812=CARTESIAN_POINT ( 'NONE',  ( 68.28783021080273841, 68.52322149771096349, 6.374026897414869275 ) ) ;
#46815=CARTESIAN_POINT ( 'NONE',  ( 82.72537510787563519, 47.46459017876031083, 12.21375674901907615 ) ) ;
#46824=CARTESIAN_POINT ( 'NONE',  ( 11.28581492663933084, 21.91421378149917487, 9.188101187500008038 ) ) ;
#46826=CARTESIAN_POINT ( 'NONE',  ( 80.75322455565131463, 57.27148952657293535, 16.56885343786527187 ) ) ;
#46828=DIRECTION ( 'NONE',  ( -0.9619696745371179025, 0.2731562652969018457, 0.000000000000000000 ) ) ;
#46834=CARTESIAN_POINT ( 'NONE',  ( 84.05047897864028528, 45.71949378961764410, -9.925846697072392644 ) ) ;
#46839=CARTESIAN_POINT ( 'NONE',  ( 74.89653295760797391, 66.81943746227949532, -13.20645658646817822 ) ) ;
#46843=EDGE_CURVE ( 'NONE', #93369, #92094, #41584, .T. ) ;
#46844=CARTESIAN_POINT ( 'NONE',  ( 82.32950663482070297, 40.35259760736478540, -1.135274614268407589 ) ) ;
#46845=CARTESIAN_POINT ( 'NONE',  ( 8.827418999677703937, 23.83478043621386178, -8.090169943749479842 ) ) ;
#46847=CARTESIAN_POINT ( 'NONE',  ( 72.57700935610729687, 70.89248372566723333, 7.619130926959984507 ) ) ;
#46849=CARTESIAN_POINT ( 'NONE',  ( 75.65669688662353565, 65.40331689797208981, 14.28920693795837948 ) ) ;
#46850=VECTOR ( 'NONE', #55244, 1000.000000000000227 ) ;
#46860=CARTESIAN_POINT ( 'NONE',  ( 74.30189495389348053, 67.90489423305770345, -11.69701164576238384 ) ) ;
#46876=CARTESIAN_POINT ( 'NONE',  ( 71.70511086140308521, 71.96099529401990935, 1.996604445853504162 ) ) ;
#46879=EDGE_LOOP ( 'NONE', ( #70567, #3720, #66009, #27276 ) ) ;
#46880=CARTESIAN_POINT ( 'NONE',  ( 75.52901426996652390, 64.87836950227075761, 14.51720410870508537 ) ) ;
#46884=CARTESIAN_POINT ( 'NONE',  ( 17.79544559245429625, 15.98920272979925628, 7.433330006724137462 ) ) ;
#46888=CARTESIAN_POINT ( 'NONE',  ( 15.90241741327948866, 17.38052372038639604, 10.00000000000000533 ) ) ;
#46893=CARTESIAN_POINT ( 'NONE',  ( 81.96759120377315355, 40.97872302293440328, -3.040391630107510679 ) ) ;
#46894=FACE_OUTER_BOUND ( 'NONE', #82148, .T. ) ;
#46895=LINE ( 'NONE', #23083, #94430 ) ;
#46896=EDGE_LOOP ( 'NONE', ( #27362, #63267, #80253, #43542 ) ) ;
#46899=CARTESIAN_POINT ( 'NONE',  ( 80.87172617107097494, 46.94429920451448623, 13.16013926657569932 ) ) ;
#46900=EDGE_CURVE ( 'NONE', #20229, #91452, #32608, .T. ) ;
#46902=CARTESIAN_POINT ( 'NONE',  ( 75.93601443309867705, 65.18730796954976370, -14.47772449952195117 ) ) ;
#46904=CARTESIAN_POINT ( 'NONE',  ( 72.40857565946932084, 71.84120774512069829, -5.522868224832428119 ) ) ;
#46908=CARTESIAN_POINT ( 'NONE',  ( 73.39522077465731797, 69.90148087279546019, 9.687480369506271671 ) ) ;
#46910=CARTESIAN_POINT ( 'NONE',  ( 40.09738740370236343, 25.01110640527295104, 2.839279412974134775 ) ) ;
#46911=EDGE_LOOP ( 'NONE', ( #3980, #85008, #65983, #31548 ) ) ;
#46915=ORIENTED_EDGE ( 'NONE', *, *, #12143, .T. ) ;
#46916=CARTESIAN_POINT ( 'NONE',  ( 79.42847595952265749, 59.61293774653857724, 16.17779656922536802 ) ) ;
#46924=CARTESIAN_POINT ( 'NONE',  ( 87.35668359673078953, 44.84080960044052944, -6.701380392922970053 ) ) ;
#46925=CARTESIAN_POINT ( 'NONE',  ( 81.52014092374062670, 55.46057516179622837, -16.31907950184206157 ) ) ;
#46930=CARTESIAN_POINT ( 'NONE',  ( 81.23909821190164848, 55.73431417435049440, 16.38583623711208404 ) ) ;
#46933=CARTESIAN_POINT ( 'NONE',  ( 79.06962916857435175, 52.50278213231310076, 15.56900390533574097 ) ) ;
#46945=B_SPLINE_CURVE_WITH_KNOTS ( 'NONE', 3,
 ( #13936, #89977, #91465, #5835, #29147, #36724, #52925, #83877, #67628, #6827 ),
 .UNSPECIFIED., .F., .F.,
 ( 4, 2, 2, 2, 4 ),
 ( 0.000000000000000000, 0.2499999999999998890, 0.4999999999999998890, 0.7499999999999998890, 1.000000000000000000 ),
 .UNSPECIFIED. ) ;
#46949=ORIENTED_EDGE ( 'NONE', *, *, #96915, .T. ) ;
#46950=EDGE_LOOP ( 'NONE', ( #8591, #33488, #8175, #47213 ) ) ;
#46962=FACE_OUTER_BOUND ( 'NONE', #40407, .T. ) ;
#46966=LINE ( 'NONE', #16563, #19612 ) ;
#46975=CARTESIAN_POINT ( 'NONE',  ( 72.36980820381833723, 65.60254448469738975, 12.49385853657623713 ) ) ;
#46985=CARTESIAN_POINT ( 'NONE',  ( 74.17864136715245138, 68.61070255371173232, 11.00189009658737760 ) ) ;
#46987=CARTESIAN_POINT ( 'NONE',  ( 71.04509092612660481, 70.63270342239739819, -5.353015442558778147 ) ) ;
#46995=CARTESIAN_POINT ( 'NONE',  ( 78.41884288903450795, 57.22565492815783728, 16.22179344803242174 ) ) ;
#46997=CARTESIAN_POINT ( 'NONE',  ( 73.38460905275829305, 69.71371501254900238, -9.902851190597802500 ) ) ;
#46998=CARTESIAN_POINT ( 'NONE',  ( 75.84431070414076714, 51.61172808879248208, 15.73310713704503172 ) ) ;
#47007=CARTESIAN_POINT ( 'NONE',  ( 88.08442549207046568, 44.03285108406542747, 0.5600040541675376238 ) ) ;
#47013=CARTESIAN_POINT ( 'NONE',  ( 24.61059131263772670, 35.18502408145593563, 5.678558825948276656 ) ) ;
#47015=CARTESIAN_POINT ( 'NONE',  ( 83.02916638930869908, 47.07448630088824615, -11.77228440242573448 ) ) ;
#47016=CARTESIAN_POINT ( 'NONE',  ( 11.52878981408637848, 24.84336893147754921, -7.433330006724137462 ) ) ;
#47019=DIRECTION ( 'NONE',  ( -0.8660254037844378194, -0.5000000000000014433, -0.000000000000000000 ) ) ;
#47027=ORIENTED_EDGE ( 'NONE', *, *, #52092, .T. ) ;
#47028=CARTESIAN_POINT ( 'NONE',  ( 77.17767550845273661, 49.49660620011481882, 14.94353481738494516 ) ) ;
#47030=VERTEX_POINT ( 'NONE', #65014 ) ;
#47033=CARTESIAN_POINT ( 'NONE',  ( 69.40581272701848548, 68.85202937589532723, -6.985974446829570361 ) ) ;
#47036=ORIENTED_EDGE ( 'NONE', *, *, #849, .T. ) ;
#47037=CARTESIAN_POINT ( 'NONE',  ( 79.48193946498695084, 46.39014452590906501, -12.72302186241215871 ) ) ;
#47042=CARTESIAN_POINT ( 'NONE',  ( 20.27385872851041526, 33.74646525600390135, 2.839279412974139660 ) ) ;
#47043=CARTESIAN_POINT ( 'NONE',  ( 75.07462636293115565, 55.18389248688383475, 16.14775407556821207 ) ) ;
#47044=CARTESIAN_POINT ( 'NONE',  ( 66.06214068257196459, 68.71579393632853794, -0.4716098740908659659 ) ) ;
#47045=CARTESIAN_POINT ( 'NONE',  ( 75.19555136791578320, 66.41508560950431672, -13.15604408571534911 ) ) ;
#47047=CARTESIAN_POINT ( 'NONE',  ( 79.58936028502597537, 59.22294857574253513, 16.56770033466462166 ) ) ;
#47052=CARTESIAN_POINT ( 'NONE',  ( 67.66077361873938401, 65.75280524250749181, 10.62536374143375362 ) ) ;
#47053=CARTESIAN_POINT ( 'NONE',  ( 67.68680448008480255, 65.78880813601070088, -10.60348352081087064 ) ) ;
#47054=CARTESIAN_POINT ( 'NONE',  ( 81.37674444193763179, 55.19836804271280783, -15.94010240901345199 ) ) ;
#47065=CARTESIAN_POINT ( 'NONE',  ( 77.99401760355904401, 61.40429962668400776, -16.15929906019731632 ) ) ;
#47066=EDGE_LOOP ( 'NONE', ( #62797, #2878, #24305, #51570 ) ) ;
#47069=CARTESIAN_POINT ( 'NONE',  ( 80.14490519927410617, 44.22583949863496855, -11.35176587220589717 ) ) ;
#47076=ORIENTED_EDGE ( 'NONE', *, *, #94947, .T. ) ;
#47084=CARTESIAN_POINT ( 'NONE',  ( 88.18953256495667858, 44.42393962918851713, 4.547252263720216625 ) ) ;
#47090=LINE ( 'NONE', #25292, #6109 ) ;
#47095=CARTESIAN_POINT ( 'NONE',  ( 72.19109158906036328, 71.10838548458626462, -5.953967166465967686 ) ) ;
#47105=FACE_OUTER_BOUND ( 'NONE', #61855, .T. ) ;
#47106=CARTESIAN_POINT ( 'NONE',  ( 79.81461207562318805, 55.55380833237374105, 16.46868291673067830 ) ) ;
#47107=CARTESIAN_POINT ( 'NONE',  ( 24.41587626779758580, 32.83478043621389020, -8.090169943749479842 ) ) ;
#47122=CARTESIAN_POINT ( 'NONE',  ( 28.51231065420500954, 32.16454794089043645, -10.00000000000000355 ) ) ;
#47125=CARTESIAN_POINT ( 'NONE',  ( 73.76584831522595209, 68.38082682530665579, 11.49424229391075514 ) ) ;
#47133=CARTESIAN_POINT ( 'NONE',  ( 70.06557347674625191, 70.21240958854686198, -6.167066747300089524 ) ) ;
#47141=CARTESIAN_POINT ( 'NONE',  ( 25.05680157815287146, 15.26216523072494624, -2.296566073217252530E-15 ) ) ;
#47147=CARTESIAN_POINT ( 'NONE',  ( 14.11662529016922640, 10.01110640527290663, 2.839279412974134775 ) ) ;
#47149=CARTESIAN_POINT ( 'NONE',  ( 85.29362735876655677, 48.41412782346649379, 12.38048700662148072 ) ) ;
#47150=CARTESIAN_POINT ( 'NONE',  ( 88.04483770822093902, 44.27991475445110581, 2.801538001295460045 ) ) ;
#47153=CARTESIAN_POINT ( 'NONE',  ( 72.54986628483382560, 71.52703918853448783, -5.429478830856362848 ) ) ;
#47154=CARTESIAN_POINT ( 'NONE',  ( 82.65729034470932390, 41.03234709804823410, -0.08711758718608976493 ) ) ;
#47156=EDGE_CURVE ( 'NONE', #22952, #64642, #29454, .T. ) ;
#47160=CARTESIAN_POINT ( 'NONE',  ( 83.13734387462676523, 42.41847577218787535, -5.524755388486198626 ) ) ;
#47163=CARTESIAN_POINT ( 'NONE',  ( 72.10046935555597258, 72.37486351763082837, -3.289382622874389206 ) ) ;
#47164=CARTESIAN_POINT ( 'NONE',  ( 80.06670661031179748, 58.13998254173431235, 16.26766733971359358 ) ) ;
#47171=EDGE_LOOP ( 'NONE', ( #84163, #95829, #51220, #14269 ) ) ;
#47175=CARTESIAN_POINT ( 'NONE',  ( 25.06043674821822265, 32.65586893147757053, -7.433330006724137462 ) ) ;
#47187=ORIENTED_EDGE ( 'NONE', *, *, #94357, .F. ) ;
#47188=CARTESIAN_POINT ( 'NONE',  ( 86.75857413767654691, 46.45790643663872288, 9.084114997326295793 ) ) ;
#47199=CARTESIAN_POINT ( 'NONE',  ( 67.69237348538017329, 66.82088825431436874, 8.559571887000258172 ) ) ;
#47200=CARTESIAN_POINT ( 'NONE',  ( 68.34576586436469370, 65.68917945663493185, -10.35820680181607401 ) ) ;
#47201=CARTESIAN_POINT ( 'NONE',  ( 69.35253854976203058, 63.01665765323906498, 13.58811665770852350 ) ) ;
#47206=LINE ( 'NONE', #78129, #54566 ) ;
#47211=CARTESIAN_POINT ( 'NONE',  ( 83.55263137061618295, 51.48653217629340162, -14.41405146157727479 ) ) ;
#47213=ORIENTED_EDGE ( 'NONE', *, *, #55887, .T. ) ;
#47215=( BOUNDED_CURVE ( )  B_SPLINE_CURVE ( 2, ( #58472, #12404, #65089, #41782, #50384, #34683, #4282, #19018, #89445, #35181, #97038, #42274, #3318 ),
 .UNSPECIFIED., .F., .T. ) 
 B_SPLINE_CURVE_WITH_KNOTS ( ( 3, 2, 2, 2, 2, 2, 3 ),
 ( 0.2625000000000000111, 0.2650000000000000133, 0.2700000000000000178, 0.2750000000000000222, 0.2800000000000000266, 0.2849999999999999756, 0.2874999999999999778 ),
 .UNSPECIFIED. ) 
 CURVE ( )  GEOMETRIC_REPRESENTATION_ITEM ( )  RATIONAL_B_SPLINE_CURVE ( ( 0.9755282581475768211, 0.9755282581475768211, 1.000000000000000000, 0.9510565162951535312, 1.000000000000000000, 0.9510565162951535312, 1.000000000000000000, 0.9510565162951535312, 1.000000000000000000, 0.9510565162951535312, 1.000000000000000000, 0.9755282581475768211, 0.9755282581475768211 ) ) 
 REPRESENTATION_ITEM ( '' )  );
#47216=CARTESIAN_POINT ( 'NONE',  ( 71.95473880081605955, 71.54457537667215661, 5.606738443688825235 ) ) ;
#47226=CARTESIAN_POINT ( 'NONE',  ( 72.42166623772517653, 61.87394061769263942, -15.04969437984479796 ) ) ;
#47232=B_SPLINE_SURFACE_WITH_KNOTS ( 'NONE', 3, 1, ( 
 ( #51469, #50965 ),
 ( #82437, #74801 ),
 ( #28665, #69530 ),
 ( #77654, #21097 ),
 ( #636, #51974 ),
 ( #66669, #13000 ),
 ( #69023, #8240 ),
 ( #12494, #140 ),
 ( #5379, #99953 ),
 ( #62410, #43361 ),
 ( #92376, #35774 ),
 ( #36265, #31024 ),
 ( #67165, #74311 ),
 ( #22923, #61915 ),
 ( #30536, #54307 ),
 ( #61423, #92863 ),
 ( #15823, #46726 ),
 ( #78147, #1655 ),
 ( #17848, #24435 ),
 ( #95396, #32540 ),
 ( #87314, #71053 ),
 ( #32018, #79178 ),
 ( #62927, #85802 ),
 ( #2650, #40617 ),
 ( #23923, #8734 ),
 ( #55311, #2147 ),
 ( #63928, #9757 ),
 ( #78651, #39605 ),
 ( #94372, #86292 ),
 ( #9236, #63435 ),
 ( #48233, #24927 ) ),
 .UNSPECIFIED., .F., .F., .F.,
 ( 4, 3, 3, 3, 3, 3, 3, 3, 3, 3, 4 ),
 ( 2, 2 ),
 ( 0.000000000000000000, 0.1333490885032397044, 0.3007194338854659588, 0.4699862290245639951, 0.5844252810809660303, 0.6686540514503046539, 0.7354980260655714641, 0.8028463152565815664, 0.8633854507757389163, 0.9437142632667553377, 1.000000000000000000 ),
 ( 0.000000000000000000, 1.000000000000000000 ),
 .UNSPECIFIED. ) ;
#47233=CARTESIAN_POINT ( 'NONE',  ( 73.87133013375215285, 63.28806875567715196, 14.81981384368521582 ) ) ;
#47242=CARTESIAN_POINT ( 'NONE',  ( 87.89309248043456080, 44.79219472772870603, 4.915507336728490273 ) ) ;
#47244=CARTESIAN_POINT ( 'NONE',  ( 18.10888558598233899, 12.58380873178785819, 6.180339887498953466 ) ) ;
#47247=DIRECTION ( 'NONE',  ( 0.1710100716628310258, -0.2961981327260192476, 0.9396926207859104263 ) ) ;
#47250=CARTESIAN_POINT ( 'NONE',  ( 12.12248498587032586, 9.127558733836242055, -6.180339887498949025 ) ) ;
#47253=CARTESIAN_POINT ( 'NONE',  ( 11.78719504716597299, 22.50829794293879260, -10.00000000000000355 ) ) ;
#47259=CARTESIAN_POINT ( 'NONE',  ( 27.63686232447692603, 34.14336893147756768, 7.433330006724141015 ) ) ;
#47265=CARTESIAN_POINT ( 'NONE',  ( 66.20598794047340618, 69.12131181250303769, 2.565109441349023189 ) ) ;
#47266=ORIENTED_EDGE ( 'NONE', *, *, #22121, .F. ) ;
#47270=CARTESIAN_POINT ( 'NONE',  ( 14.61458989734527947, 10.29860640527290805, -2.839279412974138328 ) ) ;
#47282=CARTESIAN_POINT ( 'NONE',  ( 72.98255309615508679, 70.80854987616386609, 7.399406208479893721 ) ) ;
#47283=VERTEX_POINT ( 'NONE', #71505 ) ;
#47284=CARTESIAN_POINT ( 'NONE',  ( 17.99199860517156324, 32.16126292948895582, -6.180339887498951690 ) ) ;
#47287=EDGE_CURVE ( 'NONE', #2005, #86000, #92815, .T. ) ;
#47290=CARTESIAN_POINT ( 'NONE',  ( 17.29678581741014654, 10.39040679176981996, 1.333680081654574804E-15 ) ) ;
#47291=CARTESIAN_POINT ( 'NONE',  ( 69.39239498971687681, 62.76033227987573326, 13.75497651673264521 ) ) ;
#47292=VECTOR ( 'NONE', #36433, 1000.000000000000114 ) ;
#47303=CARTESIAN_POINT ( 'NONE',  ( 72.84729272447545156, 59.04174750966416241, 15.54885058021578814 ) ) ;
#47304=ORIENTED_EDGE ( 'NONE', *, *, #57998, .F. ) ;
#47307=CARTESIAN_POINT ( 'NONE',  ( 88.09111776262265892, 44.56188567158400815, -5.102872454969319627 ) ) ;
#47308=CARTESIAN_POINT ( 'NONE',  ( 81.27042111320733397, 44.06946909743304985, 9.799045354441355826 ) ) ;
#47312=CARTESIAN_POINT ( 'NONE',  ( 82.60068805421772709, 53.27059767035463267, -15.30334251677975388 ) ) ;
#47316=CARTESIAN_POINT ( 'NONE',  ( 23.79748941506785442, 22.24335787977763346, -9.188101187500008038 ) ) ;
#47321=CYLINDRICAL_SURFACE ( 'NONE', #4518, 16.60714546451156792 ) ;
#47326=CARTESIAN_POINT ( 'NONE',  ( 80.31171660912499988, 46.24781510277671970, -12.29402398486336701 ) ) ;
#47328=CARTESIAN_POINT ( 'NONE',  ( 71.38818891405433931, 59.36944044145746346, 15.71463273504962110 ) ) ;
#47332=CARTESIAN_POINT ( 'NONE',  ( 74.68932948184826159, 66.80812537921995897, -13.13442079021221431 ) ) ;
#47336=CARTESIAN_POINT ( 'NONE',  ( 82.33632248375091933, 40.34752097026218820, -1.014975778927596828 ) ) ;
#47341=CARTESIAN_POINT ( 'NONE',  ( 75.67456858315887303, 65.42170317558291970, 14.28506259273864565 ) ) ;
#47344=ORIENTED_EDGE ( 'NONE', *, *, #80604, .F. ) ;
#47349=CARTESIAN_POINT ( 'NONE',  ( 81.67133165517434179, 46.72149670578906466, -12.10404611631500060 ) ) ;
#47350=CARTESIAN_POINT ( 'NONE',  ( 83.90260833528412832, 43.42355591996152953, 6.759210671933336911 ) ) ;
#47353=CARTESIAN_POINT ( 'NONE',  ( 74.27638480340351634, 67.89356557358171074, -11.69403406648106447 ) ) ;
#47355=DIRECTION ( 'NONE',  ( -0.7713975076906485207, 0.000000000000000000, 0.6363535849892383300 ) ) ;
#47356=VERTEX_POINT ( 'NONE', #91207 ) ;
#47359=B_SPLINE_CURVE_WITH_KNOTS ( 'NONE', 3,
 ( #72536, #94346, #94841, #24407 ),
 .UNSPECIFIED., .F., .F.,
 ( 4, 4 ),
 ( 0.000000000000000000, 0.1734847945017928272 ),
 .UNSPECIFIED. ) ;
#47362=FACE_OUTER_BOUND ( 'NONE', #80890, .T. ) ;
#47370=CARTESIAN_POINT ( 'NONE',  ( 68.20121996687745991, 67.65983906480657595, 7.773794612277492355 ) ) ;
#47374=CARTESIAN_POINT ( 'NONE',  ( 74.44098624100845996, 58.95453109306149031, 16.23807160063391208 ) ) ;
#47377=CARTESIAN_POINT ( 'NONE',  ( 8.301057521190555732, 26.83396525600388571, -2.839279412974133887 ) ) ;
#47380=CARTESIAN_POINT ( 'NONE',  ( 77.16803028340585513, 57.91059354089997413, -16.56554699001202025 ) ) ;
#47386=PLANE ( 'NONE',  #38025 ) ;
#47387=CARTESIAN_POINT ( 'NONE',  ( 44.29582294825809896, 31.28920272979930672, -7.433330006724141015 ) ) ;
#47388=CARTESIAN_POINT ( 'NONE',  ( 41.55205903992003158, 29.15404122711137447, 8.090169943749479842 ) ) ;
#47398=CARTESIAN_POINT ( 'NONE',  ( 74.99443409587989606, 53.05053269064024590, -16.02027138122841876 ) ) ;
#47400=ORIENTED_EDGE ( 'NONE', *, *, #95548, .T. ) ;
#47402=CARTESIAN_POINT ( 'NONE',  ( 31.21403501649405854, 38.99752408145594273, 5.678558825948277544 ) ) ;
#47404=CARTESIAN_POINT ( 'NONE',  ( 78.44279992643997446, 61.32017871564067946, 16.22697472196324853 ) ) ;
#47409=CARTESIAN_POINT ( 'NONE',  ( 86.54659259230355417, 47.35344409918261732, -10.80230753912618802 ) ) ;
#47414=CARTESIAN_POINT ( 'NONE',  ( 80.14677080614116278, 45.54587722633649349, -12.47700090210163104 ) ) ;
#47421=VERTEX_POINT ( 'NONE', #28369 ) ;
#47422=CARTESIAN_POINT ( 'NONE',  ( 77.27258907709742175, 49.66860660035752062, -15.49621856359588357 ) ) ;
#47424=CARTESIAN_POINT ( 'NONE',  ( 86.95562746175168911, 45.78762616370607930, -8.653322509500107174 ) ) ;
#47431=CARTESIAN_POINT ( 'NONE',  ( 82.81294776526844714, 40.62066890938785946, 0.9850604075177307184 ) ) ;
#47437=CARTESIAN_POINT ( 'NONE',  ( 39.17063663036994114, 34.56628583063844928, 9.188101187500006262 ) ) ;
#47439=CARTESIAN_POINT ( 'NONE',  ( 83.09463924182568917, 43.40643806361209300, -8.435373655842957064 ) ) ;
#47446=CARTESIAN_POINT ( 'NONE',  ( 81.04401415297212452, 43.04793497936152846, 9.543169053269965119 ) ) ;
#47448=CARTESIAN_POINT ( 'NONE',  ( 26.12309927540532328, 38.58029201028043076, 1.583844403245397769 ) ) ;
#47450=ORIENTED_EDGE ( 'NONE', *, *, #84369, .F. ) ;
#47455=ORIENTED_EDGE ( 'NONE', *, *, #47648, .T. ) ;
#47469=CARTESIAN_POINT ( 'NONE',  ( 73.40128984104008225, 64.43477936578551635, 14.11777066946370063 ) ) ;
#47475=CARTESIAN_POINT ( 'NONE',  ( 74.41176536287696308, 68.30213538679808494, 11.88880159922067747 ) ) ;
#47476=CARTESIAN_POINT ( 'NONE',  ( 73.79690245017815187, 68.46445494392735043, 10.93464038932060411 ) ) ;
#47477=CARTESIAN_POINT ( 'NONE',  ( 69.79493031643249878, 70.93090587422946669, -0.9144303869529551987 ) ) ;
#47484=CARTESIAN_POINT ( 'NONE',  ( 78.63106618800820513, 59.04553955275220289, 16.18459533489969360 ) ) ;
#47485=CARTESIAN_POINT ( 'NONE',  ( 84.52323392980522954, 49.80928010723963695, -13.22128011046212670 ) ) ;
#47486=CARTESIAN_POINT ( 'NONE',  ( 78.19610093930316452, 61.82192816133139956, 15.73638231904944718 ) ) ;
#47500=B_SPLINE_CURVE_WITH_KNOTS ( 'NONE', 3,
 ( #58128, #73841, #27742, #58610, #89586, #20149, #81971, #67222, #22624, #7410, #98147, #44416, #15003, #98653, #60597, #52030, #28732, #36818, #91553 ),
 .UNSPECIFIED., .F., .F.,
 ( 4, 2, 2, 2, 1, 2, 2, 2, 2, 4 ),
 ( 0.4743041966560226363, 0.5400161720740214166, 0.6057281474920201969, 0.6385841352010184213, 0.6714401229100168678, 0.7371520983280135386, 0.8028640737460100985, 0.8685760491640068803, 0.9342880245820035512, 1.000000000000000000 ),
 .UNSPECIFIED. ) ;
#47501=CARTESIAN_POINT ( 'NONE',  ( 88.21238909966383801, 43.70556102481675964, 0.1923655077720384798 ) ) ;
#47503=CARTESIAN_POINT ( 'NONE',  ( 71.76465953926796715, 72.09915442159702081, -3.621776363507912766 ) ) ;
#47505=CARTESIAN_POINT ( 'NONE',  ( 33.66714878060290772, 21.29860640527294180, -2.839279412974138328 ) ) ;
#47507=CARTESIAN_POINT ( 'NONE',  ( 81.93674055385325516, 47.28776839916499597, -12.40202553389867823 ) ) ;
#47508=CARTESIAN_POINT ( 'NONE',  ( 12.04840505635704417, 25.14336893147754282, 7.433330006724141015 ) ) ;
#47510=CARTESIAN_POINT ( 'NONE',  ( 76.67587641197377479, 63.85108742147927074, 14.86537621106540819 ) ) ;
#47517=CARTESIAN_POINT ( 'NONE',  ( 74.58224166234337815, 56.98362197102031956, -16.05243990554664890 ) ) ;
#47521=CARTESIAN_POINT ( 'NONE',  ( 77.63908229418555607, 49.31861150414459871, 15.29991512875208137 ) ) ;
#47526=CARTESIAN_POINT ( 'NONE',  ( 72.07913036110144844, 68.84169458634234218, -9.362130312896965734 ) ) ;
#47529=VERTEX_POINT ( 'NONE', #5573 ) ;
#47530=CARTESIAN_POINT ( 'NONE',  ( 65.93560523737669143, 69.04367854582200437, -2.085430103607250008 ) ) ;
#47534=CARTESIAN_POINT ( 'NONE',  ( 22.00590953607929023, 34.74646525600390845, 2.839279412974139660 ) ) ;
#47536=CARTESIAN_POINT ( 'NONE',  ( 74.73078456835838779, 66.79972942087577792, -13.15602295301254721 ) ) ;
#47537=CARTESIAN_POINT ( 'NONE',  ( 79.26897965571234295, 49.31431488444046352, -14.41357357798955974 ) ) ;
#47539=DIRECTION ( 'NONE',  ( -0.8660254037844378194, -0.5000000000000014433, -0.000000000000000000 ) ) ;
#47545=CARTESIAN_POINT ( 'NONE',  ( 67.87593105113009528, 65.67175317894806597, 10.83526793861203430 ) ) ;
#47546=CARTESIAN_POINT ( 'NONE',  ( 68.03752145569828258, 65.19644328924185572, -10.68142545458115933 ) ) ;
#47547=CARTESIAN_POINT ( 'NONE',  ( 81.78126323850756307, 55.46774195332329782, -15.94567292164773420 ) ) ;
#47553=CARTESIAN_POINT ( 'NONE',  ( 79.15819921557465477, 59.82093924937031204, 16.50069780760281901 ) ) ;
#47558=CARTESIAN_POINT ( 'NONE',  ( 77.99937045744943021, 62.11896432438783933, -16.00068414206377554 ) ) ;
#47563=CARTESIAN_POINT ( 'NONE',  ( 80.02183673286208432, 44.83754558038893379, -11.27937077477422356 ) ) ;
#47567=CARTESIAN_POINT ( 'NONE',  ( 79.84557217427597209, 48.50462519541254380, -13.88470291381558219 ) ) ;
#47570=VERTEX_POINT ( 'NONE', #32368 ) ;
#47575=DIRECTION ( 'NONE',  ( 0.4330127018922168558, -0.7499999999999987788, 0.5000000000000039968 ) ) ;
#47577=CARTESIAN_POINT ( 'NONE',  ( 22.87232021560678064, 28.90829794293881605, 10.00000000000000355 ) ) ;
#47580=CARTESIAN_POINT ( 'NONE',  ( 88.03991489039286478, 44.69748799199468436, 4.347629997315069161 ) ) ;
#47588=VECTOR ( 'NONE', #16975, 1000.000000000000000 ) ;
#47590=EDGE_LOOP ( 'NONE', ( #50439, #89600, #76857, #24051 ) ) ;
#47593=CARTESIAN_POINT ( 'NONE',  ( 83.75763820169687790, 42.17253232718462641, 3.815062152321099465 ) ) ;
#47603=DIRECTION ( 'NONE',  ( 0.5000000000000014433, -0.8660254037844378194, 0.000000000000000000 ) ) ;
#47604=CARTESIAN_POINT ( 'NONE',  ( 69.93344588439701681, 62.81717858415346001, -13.32880143434356235 ) ) ;
#47605=CARTESIAN_POINT ( 'NONE',  ( 24.93549151006825326, 33.13478043621389446, 8.090169943749478065 ) ) ;
#47608=DIRECTION ( 'NONE',  ( 0.5000000000000013323, -0.8660254037844378194, 0.000000000000000000 ) ) ;
#47613=CARTESIAN_POINT ( 'NONE',  ( 82.65478504301806595, 49.50942564885856711, 13.62198326750848310 ) ) ;
#47617=CARTESIAN_POINT ( 'NONE',  ( 81.84418131458886592, 41.19320572020597382, 5.701826843178367632 ) ) ;
#47620=CARTESIAN_POINT ( 'NONE',  ( 27.37348498259797935, 38.73705186507756082, -3.090169943749475845 ) ) ;
#47623=CARTESIAN_POINT ( 'NONE',  ( 73.80638704669730998, 68.31061168272385942, -11.57820046455322505 ) ) ;
#47628=CARTESIAN_POINT ( 'NONE',  ( 74.14183300149377942, 66.03016674703368949, -12.94810846154004302 ) ) ;
#47634=CARTESIAN_POINT ( 'NONE',  ( 67.04476328957329656, 66.83327842152489495, -8.922081757671701752 ) ) ;
#47635=CARTESIAN_POINT ( 'NONE',  ( 66.22544472841278207, 69.36168339246577830, 0.1681495645362227065 ) ) ;
#47638=CARTESIAN_POINT ( 'NONE',  ( 27.42516030814984163, 18.76004757982090609, 5.678558825948272215 ) ) ;
#47645=CARTESIAN_POINT ( 'NONE',  ( 71.61159621314317292, 72.40963678617121957, -1.342178375522450562 ) ) ;
#47647=CARTESIAN_POINT ( 'NONE',  ( 72.26191451101281871, 71.91445694603925176, -5.118044210176697639 ) ) ;
#47648=EDGE_CURVE ( 'NONE', #51005, #47892, #28628, .T. ) ;
#47655=DIRECTION ( 'NONE',  ( 0.5000000000000013323, -0.8660254037844378194, 0.000000000000000000 ) ) ;
#47656=CARTESIAN_POINT ( 'NONE',  ( 83.32680864440213497, 42.44806103200585312, -5.336843269292388392 ) ) ;
#47660=CARTESIAN_POINT ( 'NONE',  ( 71.68807920414248258, 72.06984970416017688, -3.563505611461031286 ) ) ;
#47661=FACE_OUTER_BOUND ( 'NONE', #75600, .T. ) ;
#47662=CARTESIAN_POINT ( 'NONE',  ( 5.995650155809629567, 19.16454794089039382, -10.00000000000000355 ) ) ;
#47671=CARTESIAN_POINT ( 'NONE',  ( 27.31210279805776509, 33.95586893147756768, 7.433330006724141015 ) ) ;
#47674=CARTESIAN_POINT ( 'NONE',  ( 74.38015889281619764, 68.44084013566667579, 11.75477996513195933 ) ) ;
#47678=ORIENTED_EDGE ( 'NONE', *, *, #55408, .F. ) ;
#47691=CARTESIAN_POINT ( 'NONE',  ( 76.20055470335279324, 65.09253202017347917, 14.18943646504600054 ) ) ;
#47692=CARTESIAN_POINT ( 'NONE',  ( 69.34698985851524355, 65.60308984842636448, -11.02141108540449288 ) ) ;
#47700=CARTESIAN_POINT ( 'NONE',  ( 83.83309058964263727, 51.93283190383716885, -14.92096955093740362 ) ) ;
#47713=EDGE_CURVE ( 'NONE', #93369, #80464, #55623, .T. ) ;
#47714=CARTESIAN_POINT ( 'NONE',  ( 75.96427205163369933, 60.71763398054469718, -16.06735551131085060 ) ) ;
#47715=ORIENTED_EDGE ( 'NONE', *, *, #89381, .F. ) ;
#47716=CARTESIAN_POINT ( 'NONE',  ( 71.84021079141780319, 65.98448790626392224, 11.99618737985939987 ) ) ;
#47718=CARTESIAN_POINT ( 'NONE',  ( 68.49446975927493497, 70.11123478153655242, -1.325469564123312516 ) ) ;
#47728=ORIENTED_EDGE ( 'NONE', *, *, #24516, .T. ) ;
#47729=EDGE_CURVE ( 'NONE', #18043, #98408, #59782, .T. ) ;
#47733=CARTESIAN_POINT ( 'NONE',  ( 16.19390013444010279, 21.30066082961420904, -10.00000000000000533 ) ) ;
#47748=CARTESIAN_POINT ( 'NONE',  ( 27.19903172117837542, 31.10171378149920329, 9.188101187500008038 ) ) ;
#47749=DIRECTION ( 'NONE',  ( 0.5000000000000014433, -0.8660254037844378194, 0.000000000000000000 ) ) ;
#47754=CARTESIAN_POINT ( 'NONE',  ( 65.84451031894835182, 68.99484999965710585, 2.058805951153825031 ) ) ;
#47759=CARTESIAN_POINT ( 'NONE',  ( 16.72130706672766109, 10.44966523072493025, -2.296566073217252530E-15 ) ) ;
#47767=CARTESIAN_POINT ( 'NONE',  ( 87.66117359288392663, 45.35348716220470067, 6.484875789303244709 ) ) ;
#47771=B_SPLINE_CURVE_WITH_KNOTS ( 'NONE', 3,
 ( #89414, #50842, #81792, #56944, #87930, #89890, #12369, #74175, #35649, #66549, #97479, #28044, #80300, #51339, #82306, #43735, #15313, #30541, #45719, #5254, #83275, #92379, #74678, #98961 ),
 .UNSPECIFIED., .F., .F.,
 ( 4, 2, 2, 2, 2, 2, 2, 2, 2, 2, 2, 4 ),
 ( 0.000000000000000000, 0.1249999999999878153, 0.2499999999999756306, 0.3749999999999634737, 0.4374999999999670819, 0.4999999999999706901, 0.5624999999999743538, 0.6249999999999780176, 0.6874999999999816813, 0.7499999999999853451, 0.8749999999999926725, 1.000000000000000000 ),
 .UNSPECIFIED. ) ;
#47773=CARTESIAN_POINT ( 'NONE',  ( 86.45558908622700756, 47.52558151742778847, 10.49075240043499591 ) ) ;
#47781=CARTESIAN_POINT ( 'NONE',  ( 78.98660877947106940, 59.42842565914681785, -16.52762269555201868 ) ) ;
#47782=CARTESIAN_POINT ( 'NONE',  ( 83.56140931445644071, 47.55900624907771856, -12.50891871133917199 ) ) ;
#47793=CARTESIAN_POINT ( 'NONE',  ( 80.20973102464937199, 46.09908331049562236, 12.23914068923185461 ) ) ;
#47802=CARTESIAN_POINT ( 'NONE',  ( 82.44970526080962259, 53.47733151612504088, -15.75145310647262065 ) ) ;
#47806=CARTESIAN_POINT ( 'NONE',  ( 23.96105869301208813, 16.76004757982090254, 5.678558825948272215 ) ) ;
#47823=CARTESIAN_POINT ( 'NONE',  ( 82.21221196657927521, 40.84058624180994457, -1.181054413250449464 ) ) ;
#47824=CARTESIAN_POINT ( 'NONE',  ( 7.026152882275393807, 27.55466486950697913, -1.111400068045478839E-16 ) ) ;
#47827=CARTESIAN_POINT ( 'NONE',  ( 75.87952572578419108, 65.59853847594877152, 13.85574643265811723 ) ) ;
#47835=CYLINDRICAL_SURFACE ( 'NONE', #34047, 16.60714546451156792 ) ;
#47836=CARTESIAN_POINT ( 'NONE',  ( 82.19874836290229325, 41.39239848049727755, 4.139731784179837781 ) ) ;
#47844=EDGE_CURVE ( 'NONE', #56530, #59778, #46296, .T. ) ;
#47849=CARTESIAN_POINT ( 'NONE',  ( 68.59598715216472442, 64.19765338651440345, -12.48679878568064971 ) ) ;
#47865=CARTESIAN_POINT ( 'NONE',  ( 15.97197434310064601, 12.14754757982088940, -5.678558825948276656 ) ) ;
#47867=CARTESIAN_POINT ( 'NONE',  ( 70.81316579126399802, 61.41551742065354347, -14.85192641751565468 ) ) ;
#47872=CARTESIAN_POINT ( 'NONE',  ( 21.45610022030931674, 34.16126292948896293, -6.180339887498951690 ) ) ;
#47881=EDGE_CURVE ( 'NONE', #8972, #56753, #5245, .T. ) ;
#47883=CARTESIAN_POINT ( 'NONE',  ( 85.57885443703831641, 45.56984769523893419, 9.424717718146821355 ) ) ;
#47890=CARTESIAN_POINT ( 'NONE',  ( 36.96107555259132482, 29.84335787977765619, 9.188101187500006262 ) ) ;
#47892=VERTEX_POINT ( 'NONE', #30231 ) ;
#47898=ADVANCED_FACE ( 'NONE', ( #45903 ), #60112, .T. ) ;
#47901=CARTESIAN_POINT ( 'NONE',  ( 86.16957357854950317, 44.43129735356627208, -7.220647133741227464 ) ) ;
#47904=CARTESIAN_POINT ( 'NONE',  ( 85.97422890462554790, 44.88503902940634305, -8.159254893437074330 ) ) ;
#47913=CARTESIAN_POINT ( 'NONE',  ( 81.17432035541970947, 55.57579169957366361, 16.36820043613993292 ) ) ;
#47915=ORIENTED_EDGE ( 'NONE', *, *, #36778, .F. ) ;
#47918=ORIENTED_EDGE ( 'NONE', *, *, #95424, .T. ) ;
#47923=CARTESIAN_POINT ( 'NONE',  ( 82.54798078747610646, 40.46213573055935342, 0.9004448831076741211 ) ) ;
#47931=CARTESIAN_POINT ( 'NONE',  ( 85.68734770396230260, 48.85621462398719217, -12.54449143327925498 ) ) ;
#47936=CARTESIAN_POINT ( 'NONE',  ( 32.41152252715882298, 42.21091486745863364, 7.012934429366973338E-14 ) ) ;
#47938=CARTESIAN_POINT ( 'NONE',  ( 71.52353591355296203, 59.88240882867724224, 15.08427714274043829 ) ) ;
#47946=CARTESIAN_POINT ( 'NONE',  ( 66.00531965145684410, 68.68482112325794731, -0.3732326179758673756 ) ) ;
#47956=B_SPLINE_CURVE_WITH_KNOTS ( 'NONE', 3,
 ( #28282, #81533, #80545, #59158, #27799, #74910, #5494, #12105, #42964, #34883 ),
 .UNSPECIFIED., .F., .F.,
 ( 4, 2, 2, 2, 4 ),
 ( 0.000000000000000000, 0.0002622400424272329066, 0.0005244800848544658133, 0.0007867201272816987199, 0.001048960169708931627 ),
 .UNSPECIFIED. ) ;
#47964=CARTESIAN_POINT ( 'NONE',  ( 16.98334746987259791, 25.50829794293879615, -10.00000000000000355 ) ) ;
#47965=CARTESIAN_POINT ( 'NONE',  ( 74.06759120418938380, 68.62503282117260994, 10.93070749243084450 ) ) ;
#47966=CARTESIAN_POINT ( 'NONE',  ( 68.39103212955656375, 70.07216116922043625, 1.057113424849359662 ) ) ;
#47972=ADVANCED_FACE ( 'NONE', ( #61111 ), #92086, .T. ) ;
#47975=CARTESIAN_POINT ( 'NONE',  ( 77.82957106945204373, 53.72413217592595203, 15.93988384268166669 ) ) ;
#47978=CARTESIAN_POINT ( 'NONE',  ( 77.58957552442460326, 61.75793702469097468, 15.67560070342385892 ) ) ;
#47986=TOROIDAL_SURFACE ( 'NONE', #10774, 15.10714546451156970, 0.5000000000000000000 ) ;
#47995=DIRECTION ( 'NONE',  ( -0.7905172007421654712, 0.000000000000000000, 0.6124398381316900064 ) ) ;
#47998=CARTESIAN_POINT ( 'NONE',  ( 79.19548930461120051, 59.90515312544787463, -16.13566294680263624 ) ) ;
#48000=CARTESIAN_POINT ( 'NONE',  ( 25.90481151690805106, 33.14336893147756768, 7.433330006724141015 ) ) ;
#48005=CARTESIAN_POINT ( 'NONE',  ( 19.63753723929501760, 13.19860640527291551, 2.839279412974134775 ) ) ;
#48007=CARTESIAN_POINT ( 'NONE',  ( 76.62859868508415673, 63.47930858090246176, 15.36151106740648409 ) ) ;
#48009=VECTOR ( 'NONE', #96334, 999.9999999999998863 ) ;
#48019=ORIENTED_EDGE ( 'NONE', *, *, #57729, .T. ) ;
#48020=CARTESIAN_POINT ( 'NONE',  ( 86.25434633476642432, 46.76098024266752873, 9.759940948247864512 ) ) ;
#48021=CARTESIAN_POINT ( 'NONE',  ( 82.29966782571446515, 53.62663270485408162, 15.81823675489985703 ) ) ;
#48025=CARTESIAN_POINT ( 'NONE',  ( 70.46465484163427107, 68.90236690406180742, -7.952911809055608572 ) ) ;
#48029=ORIENTED_EDGE ( 'NONE', *, *, #51816, .T. ) ;
#48030=CARTESIAN_POINT ( 'NONE',  ( 79.14312167556931854, 57.64441083166269664, 0.000000000000000000 ) ) ;
#48035=CARTESIAN_POINT ( 'NONE',  ( 27.77157046966360809, 18.96004757982091249, -5.678558825948275768 ) ) ;
#48036=CARTESIAN_POINT ( 'NONE',  ( 75.14516343145004384, 66.38879684927510993, -13.15419235483435045 ) ) ;
#48037=CARTESIAN_POINT ( 'NONE',  ( 82.20012801274769743, 48.57593112100128252, -13.18042320071303664 ) ) ;
#48041=CARTESIAN_POINT ( 'NONE',  ( 81.56753329430793542, 59.44520672954722329, 0.3596699001693225983 ) ) ;
#48046=CARTESIAN_POINT ( 'NONE',  ( 67.67694934082794589, 65.73157130137430215, 10.65708354426730864 ) ) ;
#48048=CARTESIAN_POINT ( 'NONE',  ( 81.74146036984987518, 55.29309318191306488, -15.92173512836979654 ) ) ;
#48053=CARTESIAN_POINT ( 'NONE',  ( 74.90858141719442642, 61.82407377426982009, -15.58808111368598048 ) ) ;
#48054=CARTESIAN_POINT ( 'NONE',  ( 79.53039288183295241, 59.52037319582147035, 16.54552321433123652 ) ) ;
#48060=ORIENTED_EDGE ( 'NONE', *, *, #92636, .T. ) ;
#48064=CARTESIAN_POINT ( 'NONE',  ( 80.39210556992956924, 44.73937495152041777, -11.68521036719157458 ) ) ;
#48069=CARTESIAN_POINT ( 'NONE',  ( 84.80231054593309636, 47.28878989737494720, -11.15588628155341056 ) ) ;
#48077=EDGE_CURVE ( 'NONE', #89630, #96180, #62198, .T. ) ;
#48081=CARTESIAN_POINT ( 'NONE',  ( 87.56490573087398843, 44.61754441107329683, 4.959165031671988189 ) ) ;
#48084=CARTESIAN_POINT ( 'NONE',  ( 84.25039669599603087, 43.70795126229808147, -6.896957926195620203 ) ) ;
#48096=FACE_OUTER_BOUND ( 'NONE', #75086, .T. ) ;
#48098=CARTESIAN_POINT ( 'NONE',  ( 78.01910789048406514, 61.79390329888819622, 16.07883194446994679 ) ) ;
#48105=CARTESIAN_POINT ( 'NONE',  ( 73.83712343681983725, 55.22609035296176927, 16.12121283296830399 ) ) ;
#48108=CARTESIAN_POINT ( 'NONE',  ( 27.87997788293534285, 34.83478043621390441, -8.090169943749479842 ) ) ;
#48118=CARTESIAN_POINT ( 'NONE',  ( 83.13520543127567919, 52.15262426605146118, 14.79738518802719049 ) ) ;
#48121=CARTESIAN_POINT ( 'NONE',  ( 35.05457148360284236, 21.20801979619930933, -3.090169943749474069 ) ) ;
#48122=CARTESIAN_POINT ( 'NONE',  ( 72.13088006912725803, 72.32200972276189077, -1.116376892176975000 ) ) ;
#48126=CARTESIAN_POINT ( 'NONE',  ( 33.51440821012886317, 31.30066082961424456, -10.00000000000000533 ) ) ;
#48131=CARTESIAN_POINT ( 'NONE',  ( 73.29578800698439522, 66.59928693814347866, 12.71955346165220568 ) ) ;
#48137=CARTESIAN_POINT ( 'NONE',  ( 76.77731254116881132, 64.09355814141257213, -15.16545583891343263 ) ) ;
#48139=EDGE_CURVE ( 'NONE', #41560, #83225, #71648, .T. ) ;
#48147=CARTESIAN_POINT ( 'NONE',  ( 66.31687960855757069, 69.41545726844323383, 0.05603871075114778139 ) ) ;
#48148=LINE ( 'NONE', #69076, #92757 ) ;
#48151=CARTESIAN_POINT ( 'NONE',  ( 28.38260615371904905, 22.10170272979928185, -7.433330006724141015 ) ) ;
#48158=CARTESIAN_POINT ( 'NONE',  ( 6.089662503932698812, 18.91421378149916421, 9.188101187500008038 ) ) ;
#48159=CARTESIAN_POINT ( 'NONE',  ( 76.39671315866488044, 58.77431009255887062, -16.02812391186772700 ) ) ;
#48160=CARTESIAN_POINT ( 'NONE',  ( 71.59149729713742261, 72.39908022291972145, -1.330894502438451754 ) ) ;
#48164=CARTESIAN_POINT ( 'NONE',  ( 72.11718761729461846, 71.53392678631075796, -5.852761162471809442 ) ) ;
#48165=CARTESIAN_POINT ( 'NONE',  ( 85.34302531380257051, 49.09540806577671646, 12.42140015106420847 ) ) ;
#48175=CARTESIAN_POINT ( 'NONE',  ( 72.77847538495844049, 57.31112570069235090, -15.86834930776232255 ) ) ;
#48182=ORIENTED_EDGE ( 'NONE', *, *, #9124, .T. ) ;
#48185=CARTESIAN_POINT ( 'NONE',  ( 30.18562306610639112, 29.37878583063842441, 9.188101187500006262 ) ) ;
#48187=CARTESIAN_POINT ( 'NONE',  ( 78.29597207138884585, 47.82683086104820092, -14.50971761538352744 ) ) ;
#48189=CARTESIAN_POINT ( 'NONE',  ( 73.85129109314340212, 68.53037146055885387, 11.40305250113368629 ) ) ;
#48196=CARTESIAN_POINT ( 'NONE',  ( 77.08943580299947484, 49.61595851769168064, 15.51385818994994459 ) ) ;
#48200=CARTESIAN_POINT ( 'NONE',  ( 71.05045428464670465, 69.84340204859232415, -6.994201869904678404 ) ) ;
#48208=CARTESIAN_POINT ( 'NONE',  ( 83.13810225994288317, 42.45549248814388932, -6.801163518002313779 ) ) ;
#48209=CARTESIAN_POINT ( 'NONE',  ( 76.04328680567357424, 65.50720358278793753, 13.94868768647875612 ) ) ;
#48210=CARTESIAN_POINT ( 'NONE',  ( 72.69105027424014054, 65.04613689808410015, -12.99582216046819205 ) ) ;
#48216=CARTESIAN_POINT ( 'NONE',  ( 86.13879346367242817, 46.95025718893440825, -10.63009676298479356 ) ) ;
#48218=CARTESIAN_POINT ( 'NONE',  ( 83.81598819787330967, 51.53879304665028371, -14.37095643376077092 ) ) ;
#48220=VERTEX_POINT ( 'NONE', #71169 ) ;
#48233=CARTESIAN_POINT ( 'NONE',  ( 85.33699565288863198, 48.33901173460943568, -12.30238903177782817 ) ) ;
#48238=DIRECTION ( 'NONE',  ( -0.8660254037844378194, -0.5000000000000014433, -0.000000000000000000 ) ) ;
#48241=ADVANCED_FACE ( 'NONE', ( #17969 ), #88636, .T. ) ;
#48246=CARTESIAN_POINT ( 'NONE',  ( 75.36487073175837281, 53.53173320265494084, -16.04382577248123809 ) ) ;
#48248=ADVANCED_FACE ( 'NONE', ( #3275 ), #81783, .T. ) ;
#48250=CARTESIAN_POINT ( 'NONE',  ( 88.03824807523534446, 44.69492972130227315, 4.342143822040329226 ) ) ;
#48252=CARTESIAN_POINT ( 'NONE',  ( 12.20045371381521626, 28.81751292744055704, -6.180339887498951690 ) ) ;
#48253=CARTESIAN_POINT ( 'NONE',  ( 68.45344762042827824, 64.57392882346940155, 12.12708197196866600 ) ) ;
#48255=CARTESIAN_POINT ( 'NONE',  ( 72.28203645621837836, 72.07279491845184793, 3.271428334514307590 ) ) ;
#48258=CARTESIAN_POINT ( 'NONE',  ( 35.21268636174862365, 20.73415679381824006, 1.333680081654574804E-15 ) ) ;
#48261=DIRECTION ( 'NONE',  ( -0.5000000000000082157, 0.8660254037844338226, 0.000000000000000000 ) ) ;
#48265=CARTESIAN_POINT ( 'NONE',  ( 66.85524610400479162, 67.34209505064850987, -6.990925417236247164 ) ) ;
#48267=AXIS2_PLACEMENT_3D ( 'NONE', #26417, #34992, #74020 ) ;
#48269=CARTESIAN_POINT ( 'NONE',  ( 33.97448420766330202, 31.56628583063843152, 9.188101187500006262 ) ) ;
#48274=CARTESIAN_POINT ( 'NONE',  ( 31.05045217176252237, 26.43085787977764767, -9.188101187500008038 ) ) ;
#48278=CARTESIAN_POINT ( 'NONE',  ( 66.10780414051451714, 68.63670250712272036, 1.777645618418522533 ) ) ;
#48284=CARTESIAN_POINT ( 'NONE',  ( 11.13306418284875576, 18.37878583063839244, 9.188101187500006262 ) ) ;
#48286=CARTESIAN_POINT ( 'NONE',  ( 20.65814732634927609, 20.43085787977763346, -9.188101187500008038 ) ) ;
#48290=CARTESIAN_POINT ( 'NONE',  ( 88.03317622032373890, 44.09547299458050418, -1.704834311733967711 ) ) ;
#48291=ORIENTED_EDGE ( 'NONE', *, *, #73168, .F. ) ;
#48292=CARTESIAN_POINT ( 'NONE',  ( 32.88524308553003550, 19.39040679176984838, -6.890680421881970419E-14 ) ) ;
#48294=FACE_OUTER_BOUND ( 'NONE', #71440, .T. ) ;
#48295=CARTESIAN_POINT ( 'NONE',  ( 87.66085752470290515, 45.43799534522830896, 6.661108708518598043 ) ) ;
#48301=CARTESIAN_POINT ( 'NONE',  ( 86.47146563682314024, 47.48338690922361138, 10.43545430509261607 ) ) ;
#48306=CARTESIAN_POINT ( 'NONE',  ( 78.33236083551435058, 61.59332569120734036, -15.80201694036198745 ) ) ;
#48307=CARTESIAN_POINT ( 'NONE',  ( 78.94155721643029722, 59.44305089757030913, -16.52414004995257457 ) ) ;
#48310=VERTEX_POINT ( 'NONE', #29052 ) ;
#48320=CARTESIAN_POINT ( 'NONE',  ( 72.60116808109883380, 58.01589515306911693, 15.73743885619152394 ) ) ;
#48321=ORIENTED_EDGE ( 'NONE', *, *, #65995, .F. ) ;
#48323=EDGE_LOOP ( 'NONE', ( #64831, #18545, #29249, #44325 ) ) ;
#48324=CARTESIAN_POINT ( 'NONE',  ( 82.29696812179142285, 46.31306431584521732, 11.46503684240460963 ) ) ;
#48331=CARTESIAN_POINT ( 'NONE',  ( 75.98104421109889017, 51.53574906954565193, 16.18761828508177558 ) ) ;
#48332=CARTESIAN_POINT ( 'NONE',  ( 27.97303175072023151, 18.01110640527293327, 2.839279412974134775 ) ) ;
#48345=ORIENTED_EDGE ( 'NONE', *, *, #34475, .F. ) ;
#48347=CARTESIAN_POINT ( 'NONE',  ( 14.42807667092211865, 8.734156793818204534, -7.779800476318352071E-15 ) ) ;
#48348=CARTESIAN_POINT ( 'NONE',  ( 74.82458239918587140, 66.79921256097770765, -13.19236156228706847 ) ) ;
#48353=CARTESIAN_POINT ( 'NONE',  ( 82.09771067107622855, 40.75407999355962119, -0.9479713174774019313 ) ) ;
#48355=CARTESIAN_POINT ( 'NONE',  ( 81.30975366074838462, 56.24313983998633404, -16.44754541364717326 ) ) ;
#48359=CARTESIAN_POINT ( 'NONE',  ( 75.51323141522172477, 65.35427051582675517, 13.87231131232226922 ) ) ;
#48366=CARTESIAN_POINT ( 'NONE',  ( 80.25009607139122636, 47.00733110321809960, -12.86902101113169294 ) ) ;
#48367=CARTESIAN_POINT ( 'NONE',  ( 83.72222592155259235, 43.16924363288482880, 6.458418534604592587 ) ) ;
#48368=DIRECTION ( 'NONE',  ( -0.4996954135095461047, 0.8654978445076770832, -0.03489949670251103753 ) ) ;
#48370=CARTESIAN_POINT ( 'NONE',  ( 74.40386970632725649, 67.99584678604389865, -11.66886300729125914 ) ) ;
#48373=B_SPLINE_CURVE_WITH_KNOTS ( 'NONE', 3,
 ( #42243, #88425, #49855, #65552, #13367, #44231, #89892, #5744, #51342, #36634 ),
 .UNSPECIFIED., .F., .F.,
 ( 4, 2, 2, 2, 4 ),
 ( 0.000000000000000000, 0.0002622400424273647456, 0.0005244800848547294912, 0.0007867201272820942368, 0.001048960169709458982 ),
 .UNSPECIFIED. ) ;
#48376=CARTESIAN_POINT ( 'NONE',  ( 84.55105187355179908, 49.10534814802225867, 12.70480211847229235 ) ) ;
#48383=LINE ( 'NONE', #32671, #12786 ) ;
#48385=CARTESIAN_POINT ( 'NONE',  ( 72.54275072821182846, 68.03364687615834328, -11.16216900646165122 ) ) ;
#48392=CARTESIAN_POINT ( 'NONE',  ( 15.60392711327956761, 29.98502408145592213, -5.678558825948271327 ) ) ;
#48393=CARTESIAN_POINT ( 'NONE',  ( 74.80730538133219909, 67.19677535317899242, 12.47566025441376603 ) ) ;
#48394=CARTESIAN_POINT ( 'NONE',  ( 79.14312167556931854, 57.64441083166269664, 0.000000000000000000 ) ) ;
#48400=CARTESIAN_POINT ( 'NONE',  ( 45.79150443358504674, 28.29860640527296667, -2.839279412974138328 ) ) ;
#48403=ORIENTED_EDGE ( 'NONE', *, *, #90823, .T. ) ;
#48407=CARTESIAN_POINT ( 'NONE',  ( 72.12922596056051816, 72.33235173570187726, 1.011742168054688307 ) ) ;
#48408=CARTESIAN_POINT ( 'NONE',  ( 78.56719005003022005, 47.98515344134877836, 13.96283253221395704 ) ) ;
#48411=CARTESIAN_POINT ( 'NONE',  ( 74.96609828305089707, 53.12645705097258997, -16.02874109550557336 ) ) ;
#48415=CARTESIAN_POINT ( 'NONE',  ( 32.22500930073565684, 40.64646525600392835, -2.839279412974133887 ) ) ;
#48423=CARTESIAN_POINT ( 'NONE',  ( 79.36969597941133259, 59.79870839543468009, 16.16250099277175067 ) ) ;
#48427=FACE_OUTER_BOUND ( 'NONE', #42835, .T. ) ;
#48428=CARTESIAN_POINT ( 'NONE',  ( 84.76617582037141574, 50.00026310130547813, -13.66906362199170921 ) ) ;
#48434=CARTESIAN_POINT ( 'NONE',  ( 77.14493030857452993, 49.40685365668701934, -15.43250326293851415 ) ) ;
#48435=ORIENTED_EDGE ( 'NONE', *, *, #67698, .F. ) ;
#48436=CARTESIAN_POINT ( 'NONE',  ( 88.36122950843017065, 44.19684974305501157, -0.04416232360327642520 ) ) ;
#48437=VECTOR ( 'NONE', #78073, 999.9999999999998863 ) ;
#48439=ORIENTED_EDGE ( 'NONE', *, *, #49194, .T. ) ;
#48441=CARTESIAN_POINT ( 'NONE',  ( 29.20513097723256024, 32.56454794089043503, 10.00000000000000355 ) ) ;
#48443=CARTESIAN_POINT ( 'NONE',  ( 70.62434185772895034, 62.04354964908118575, -13.98456736824397062 ) ) ;
#48451=CARTESIAN_POINT ( 'NONE',  ( 70.58921092982998857, 61.38955905053295936, -14.80681037022087132 ) ) ;
#48453=CARTESIAN_POINT ( 'NONE',  ( 36.73494696561986217, 42.18502408145594984, 5.678558825948277544 ) ) ;
#48456=CARTESIAN_POINT ( 'NONE',  ( 83.61754957953866096, 52.24592005514148951, -14.70745080183156972 ) ) ;
#48462=CARTESIAN_POINT ( 'NONE',  ( 73.01840184697886116, 65.54798808777084673, 12.82851028372286706 ) ) ;
#48471=ORIENTED_EDGE ( 'NONE', *, *, #30619, .T. ) ;
#48489=CARTESIAN_POINT ( 'NONE',  ( 74.13497556468038852, 68.62018799133311120, 11.47049235834077408 ) ) ;
#48497=CARTESIAN_POINT ( 'NONE',  ( 7.330671393470725050, 16.18347333012629008, -9.594050593750004907 ) ) ;
#48499=VECTOR ( 'NONE', #2242, 1000.000000000000000 ) ;
#48502=CARTESIAN_POINT ( 'NONE',  ( 78.23645445329486847, 55.98478834354698819, 16.17353624429016534 ) ) ;
#48503=CARTESIAN_POINT ( 'NONE',  ( 77.80179017151976950, 62.02139351241540766, 15.64422485472365487 ) ) ;
#48504=CARTESIAN_POINT ( 'NONE',  ( 67.27848795683267724, 66.89052574399529760, 9.026760262957274961 ) ) ;
#48513=CARTESIAN_POINT ( 'NONE',  ( 73.43001404989733771, 69.84121715231802341, 9.192346335135486157 ) ) ;
#48519=CARTESIAN_POINT ( 'NONE',  ( 88.46984543095399545, 43.85297569260386297, 0.05479058522690674615 ) ) ;
#48524=CARTESIAN_POINT ( 'NONE',  ( 26.34264212020660167, 36.18502408145594273, 5.678558825948276656 ) ) ;
#48526=CARTESIAN_POINT ( 'NONE',  ( 80.80681612256114477, 47.51855870693373163, -12.98719063757217107 ) ) ;
#48528=CARTESIAN_POINT ( 'NONE',  ( 20.82171660429349203, 14.94754757982089366, 5.678558825948272215 ) ) ;
#48530=DIRECTION ( 'NONE',  ( -0.06958655048002569676, 0.1205274409548614395, -0.9902680687415721383 ) ) ;
#48537=CARTESIAN_POINT ( 'NONE',  ( 75.28764074951533303, 53.10663795412859400, 16.48602496812178941 ) ) ;
#48538=ORIENTED_EDGE ( 'NONE', *, *, #73168, .T. ) ;
#48539=CARTESIAN_POINT ( 'NONE',  ( 82.36618331495026268, 53.78214551141626742, 15.85029956610786783 ) ) ;
#48543=CARTESIAN_POINT ( 'NONE',  ( 67.16135865072904210, 68.50708211668059278, -4.823428580958654344 ) ) ;
#48547=CARTESIAN_POINT ( 'NONE',  ( 72.38244233070295763, 71.76593646792086645, 5.668245152086862859 ) ) ;
#48552=CARTESIAN_POINT ( 'NONE',  ( 29.87828763904599683, 19.11110640527293469, -2.839279412974138328 ) ) ;
#48553=CARTESIAN_POINT ( 'NONE',  ( 75.00762831775020345, 66.90256318391985246, -13.19391308334217783 ) ) ;
#48554=DIRECTION ( 'NONE',  ( -0.8660254037844378194, -0.5000000000000014433, -0.000000000000000000 ) ) ;
#48569=VECTOR ( 'NONE', #15505, 999.9999999999998863 ) ;
#48571=CARTESIAN_POINT ( 'NONE',  ( 73.07159975088246995, 72.16059528448882077, 0.000000000000000000 ) ) ;
#48576=CARTESIAN_POINT ( 'NONE',  ( 77.91028351001615704, 61.39461664896379034, -16.15133184208620420 ) ) ;
#48577=VERTEX_POINT ( 'NONE', #16704 ) ;
#48580=CARTESIAN_POINT ( 'NONE',  ( 80.32560484147226987, 44.93948968179056180, -11.21518412823304445 ) ) ;
#48583=CARTESIAN_POINT ( 'NONE',  ( 84.53427811226562483, 42.13127511552543325, -0.9647912365454934802 ) ) ;
#48584=CARTESIAN_POINT ( 'NONE',  ( 81.01193622735327438, 48.21211403554050179, -13.36836587503643159 ) ) ;
#48590=VERTEX_POINT ( 'NONE', #67670 ) ;
#48594=EDGE_LOOP ( 'NONE', ( #72116, #64531, #72413, #57282 ) ) ;
#48595=B_SPLINE_CURVE_WITH_KNOTS ( 'NONE', 3,
 ( #26882, #32967, #19308, #25898, #18293, #41563, #57263, #80625, #3593, #11201 ),
 .UNSPECIFIED., .F., .F.,
 ( 4, 2, 2, 2, 4 ),
 ( 0.3240010727220205000, 0.6620005363610115268, 0.7465004022707594222, 0.8310002681805074287, 1.000000000000000000 ),
 .UNSPECIFIED. ) ;
#48596=B_SPLINE_CURVE_WITH_KNOTS ( 'NONE', 3,
 ( #18330, #64417, #2632, #42104, #11728, #4106, #65410, #10725, #41600, #11241, #26919, #82158, #42590, #56805, #58299, #41093, #74025, #72029, #80159, #57798, #64922, #87790, #72544, #3149, #95866, #65901, #88275, #96857, #27424, #66407, #18825, #58783, #50695, #57304, #81650, #49708, #19347, #50209, #4613, #20321, #67904, #21798, #44082, #12733, #45095, #60275 ),
 .UNSPECIFIED., .F., .F.,
 ( 4, 1, 2, 2, 1, 2, 2, 1, 1, 2, 2, 1, 1, 2, 2, 1, 1, 2, 2, 1, 1, 1, 2, 2, 1, 1, 1, 2, 2, 4 ),
 ( 0.000000000000000000, 0.06249999999999407418, 0.09374999999999257538, 0.1249999999999910905, 0.1874999999999910905, 0.2187499999999912015, 0.2499999999999912847, 0.3124999999999945599, 0.3437499999999963363, 0.3593749999999957256, 0.3749999999999951150, 0.4374999999999903966, 0.4687499999999894529, 0.4843749999999891198, 0.4999999999999887867, 0.5624999999999840128, 0.5937499999999800160, 0.6093749999999782396, 0.6249999999999763522, 0.6874999999999722444, 0.7187499999999702460, 0.7343749999999693578, 0.7421874999999686917, 0.7499999999999680256, 0.8124999999999780176, 0.8437499999999812372, 0.8593749999999812372, 0.8671874999999825695, 0.8749999999999840128, 1.000000000000000000 ),
 .UNSPECIFIED. ) ;
#48598=CARTESIAN_POINT ( 'NONE',  ( 73.16146949562005375, 69.20639639887286876, -9.765445885128082537 ) ) ;
#48600=CARTESIAN_POINT ( 'NONE',  ( 87.95873400847938228, 44.36334681983743877, 4.762736470890962082 ) ) ;
#48612=EDGE_CURVE ( 'NONE', #24001, #86729, #27312, .T. ) ;
#48614=CARTESIAN_POINT ( 'NONE',  ( 83.45685042842153223, 41.88942480781632582, 3.373892084012322989 ) ) ;
#48616=CARTESIAN_POINT ( 'NONE',  ( 78.41424692880730163, 61.43889907920149795, 16.20108440401020999 ) ) ;
#48625=CARTESIAN_POINT ( 'NONE',  ( 74.25213553829982516, 55.44843064055443449, 16.12155446884580812 ) ) ;
#48626=CARTESIAN_POINT ( 'NONE',  ( 79.98875348938439345, 57.15387458570124579, 16.58871383043193859 ) ) ;
#48627=CARTESIAN_POINT ( 'NONE',  ( 36.02478613032081967, 22.92755873383628540, 6.180339887498953466 ) ) ;
#48644=CARTESIAN_POINT ( 'NONE',  ( 36.13333420750807079, 36.56454794089044924, 10.00000000000000355 ) ) ;
#48648=CARTESIAN_POINT ( 'NONE',  ( 81.69294868133339094, 55.63836673252024667, 15.97022168499915828 ) ) ;
#48649=CARTESIAN_POINT ( 'NONE',  ( 11.84292332949202020, 15.03677371833800080, 10.00000000000000533 ) ) ;
#48652=B_SPLINE_CURVE_WITH_KNOTS ( 'NONE', 3,
 ( #17593, #18099, #8010, #47484, #23672, #93121, #17084, #38882, #40868, #16090, #32784, #46995, #25185, #64191, #70281, #79440, #77909, #48502, #8497, #892, #78920, #70797, #1407, #32288, #63189, #93628, #24195, #94131, #47975, #71814, #2411, #33289, #71311, #63692, #94628, #34293, #4387, #27705, #80442, #88058, #34778, #27201, #65680, #26694, #97615, #57580 ),
 .UNSPECIFIED., .F., .F.,
 ( 4, 1, 2, 2, 1, 2, 2, 1, 1, 2, 2, 1, 1, 2, 2, 1, 1, 2, 2, 1, 1, 1, 2, 2, 1, 1, 1, 2, 2, 4 ),
 ( 0.000000000000000000, 0.06250000000000137390, 0.09375000000000205391, 0.1250000000000027478, 0.1875000000000019984, 0.2187500000000013878, 0.2500000000000007772, 0.3124999999999995559, 0.3437499999999978906, 0.3593749999999973910, 0.3749999999999968914, 0.4374999999999915623, 0.4687499999999882316, 0.4843749999999878431, 0.4999999999999874545, 0.5624999999999912292, 0.5937499999999941158, 0.6093749999999962252, 0.6249999999999983347, 0.6875000000000041078, 0.7187500000000061062, 0.7343750000000067724, 0.7421875000000062172, 0.7500000000000055511, 0.8125000000000018874, 0.8437500000000003331, 0.8593750000000000000, 0.8671874999999997780, 0.8749999999999994449, 1.000000000000000000 ),
 .UNSPECIFIED. ) ;
#48655=DIRECTION ( 'NONE',  ( -0.4827766168686586923, -0.5834231310750570554, -0.6531035050674809384 ) ) ;
#48662=DIRECTION ( 'NONE',  ( -0.8660254037844378194, -0.5000000000000014433, -0.000000000000000000 ) ) ;
#48664=CARTESIAN_POINT ( 'NONE',  ( 82.63281508726200286, 40.94328431233920895, -3.617117793111280122 ) ) ;
#48665=LINE ( 'NONE', #2570, #97614 ) ;
#48667=B_SPLINE_CURVE_WITH_KNOTS ( 'NONE', 3,
 ( #93539, #93025, #77307, #23086, #61088, #15999, #100123, #84936, #6900, #92058, #38789, #99623, #1310, #83950, #69695, #53492 ),
 .UNSPECIFIED., .F., .F.,
 ( 4, 1, 2, 2, 2, 1, 2, 2, 4 ),
 ( 0.000000000000000000, 0.1249999999999935607, 0.1874999999999922839, 0.2499999999999910072, 0.4999999999999943379, 0.6249999999999965583, 0.6874999999999971134, 0.7499999999999976685, 1.000000000000000000 ),
 .UNSPECIFIED. ) ;
#48669=CARTESIAN_POINT ( 'NONE',  ( 26.18145187173165311, 30.51421378149920116, -9.188101187500004485 ) ) ;
#48674=CARTESIAN_POINT ( 'NONE',  ( 11.13306418284875576, 18.37878583063839244, 9.188101187500006262 ) ) ;
#48675=LINE ( 'NONE', #18275, #20567 ) ;
#48679=CARTESIAN_POINT ( 'NONE',  ( 72.20607312672656519, 71.10925155450907198, -5.972286613955676948 ) ) ;
#48685=CARTESIAN_POINT ( 'NONE',  ( 69.36140278139266968, 71.17324983025980600, 0.8027048792421369594 ) ) ;
#48690=CARTESIAN_POINT ( 'NONE',  ( 72.63904040253795813, 57.48289066996441932, -16.31294606514927636 ) ) ;
#48691=CARTESIAN_POINT ( 'NONE',  ( 77.16076033720362659, 63.58031483167507503, 15.43380074518343825 ) ) ;
#48692=CARTESIAN_POINT ( 'NONE',  ( 72.21491844529387549, 53.64441083166271085, 0.000000000000000000 ) ) ;
#48699=CARTESIAN_POINT ( 'NONE',  ( 33.57875857642567752, 25.10170272979928896, -7.433330006724141015 ) ) ;
#48701=CARTESIAN_POINT ( 'NONE',  ( 78.24399414866135771, 47.91685926408410268, -14.02064381479976340 ) ) ;
#48704=CARTESIAN_POINT ( 'NONE',  ( 74.07459009150333884, 68.62600853808264389, 11.43350474783684767 ) ) ;
#48709=CARTESIAN_POINT ( 'NONE',  ( 87.79538347886169447, 45.10662587206184071, 6.725936807544243834 ) ) ;
#48711=( BOUNDED_CURVE ( )  B_SPLINE_CURVE ( 2, ( #845, #24642, #94585, #2370, #32245, #48959, #18062, #62628, #93584, #8949, #10458, #2879, #41334 ),
 .UNSPECIFIED., .F., .T. ) 
 B_SPLINE_CURVE_WITH_KNOTS ( ( 3, 2, 2, 2, 2, 2, 3 ),
 ( 0.5125000000000000666, 0.5150000000000000133, 0.5200000000000000178, 0.5250000000000000222, 0.5300000000000000266, 0.5350000000000000311, 0.5375000000000000888 ),
 .UNSPECIFIED. ) 
 CURVE ( )  GEOMETRIC_REPRESENTATION_ITEM ( )  RATIONAL_B_SPLINE_CURVE ( ( 0.9755282581475767101, 0.9755282581475772652, 1.000000000000000000, 0.9510565162951535312, 1.000000000000000000, 0.9510565162951535312, 1.000000000000000000, 0.9510565162951535312, 1.000000000000000000, 0.9510565162951535312, 1.000000000000000000, 0.9755282581475761550, 0.9755282581475767101 ) ) 
 REPRESENTATION_ITEM ( '' )  );
#48712=CARTESIAN_POINT ( 'NONE',  ( 74.46650544198260491, 58.60527373928128725, -15.83729253052527319 ) ) ;
#48714=CARTESIAN_POINT ( 'NONE',  ( 78.65816961274913410, 57.55682543410598839, 16.60711249658122668 ) ) ;
#48720=B_SPLINE_CURVE_WITH_KNOTS ( 'NONE', 3,
 ( #63266, #971, #16663, #47558, #9073, #70877, #71387, #1483, #32366, #94206, #16167, #62244, #40941, #71887, #24761, #32861, #40451, #55640, #2484, #25262, #17675, #86626, #47065, #33366, #23750, #48576, #25786, #77980, #17160, #56663, #87647 ),
 .UNSPECIFIED., .F., .F.,
 ( 4, 3, 3, 3, 3, 3, 3, 3, 3, 3, 4 ),
 ( 0.000000000000000000, 0.1333490885032390105, 0.3007194338854328186, 0.4699862290245252483, 0.5844252810809424936, 0.6686540514502805621, 0.7354980260655528124, 0.8028463152565618044, 0.8633854507757205976, 0.9437142632667329112, 1.000000000000000000 ),
 .UNSPECIFIED. ) ;
#48724=CARTESIAN_POINT ( 'NONE',  ( 67.40908756201770302, 66.96761179404961695, 9.024507661442916273 ) ) ;
#48730=CARTESIAN_POINT ( 'NONE',  ( 84.28294931125054745, 42.37490528802118206, 3.413621673734357209 ) ) ;
#48733=CARTESIAN_POINT ( 'NONE',  ( 83.77043784194415821, 51.50489687730897259, -14.36765084287526406 ) ) ;
#48737=CARTESIAN_POINT ( 'NONE',  ( 80.41065583177754661, 57.49148768039361812, -16.58946210043120217 ) ) ;
#48740=CARTESIAN_POINT ( 'NONE',  ( 72.99786219007800980, 70.75108751906873295, 8.232086053012798388 ) ) ;
#48747=CARTESIAN_POINT ( 'NONE',  ( 83.90596095485256001, 41.21795184261720379, -1.108148245180562033E-06 ) ) ;
#48749=CARTESIAN_POINT ( 'NONE',  ( 72.82155047740585019, 61.75947611529039705, -15.18569844785497480 ) ) ;
#48759=CARTESIAN_POINT ( 'NONE',  ( 80.20189741304909603, 52.03696804570480339, -15.25587582201593229 ) ) ;
#48762=CARTESIAN_POINT ( 'NONE',  ( 87.83617351001007023, 44.77714871921288875, 4.967881908888847953 ) ) ;
#48764=CARTESIAN_POINT ( 'NONE',  ( 15.16022976130349065, 27.49103043416548431, -8.090169943749479842 ) ) ;
#48766=CARTESIAN_POINT ( 'NONE',  ( 77.96183350652215438, 50.52624373792482970, -15.65746755701282211 ) ) ;
#48768=CARTESIAN_POINT ( 'NONE',  ( 72.02410375280403798, 72.02863993979345025, 2.848237292894958639 ) ) ;
#48775=EDGE_LOOP ( 'NONE', ( #40969, #42429, #69647, #2986 ) ) ;
#48781=CARTESIAN_POINT ( 'NONE',  ( 29.25887229277395463, 38.93396525600392266, 2.839279412974139660 ) ) ;
#48786=CARTESIAN_POINT ( 'NONE',  ( 29.97031301328857467, 32.70171378149920827, -9.188101187500004485 ) ) ;
#48793=CARTESIAN_POINT ( 'NONE',  ( 6.244247187202517146, 25.64646525600388216, -2.839279412974133887 ) ) ;
#48795=CARTESIAN_POINT ( 'NONE',  ( 14.92192532440567199, 20.56628583063839955, 9.188101187500006262 ) ) ;
#48798=CARTESIAN_POINT ( 'NONE',  ( 87.90399932408934092, 44.03024641107109005, -1.767293127319844670 ) ) ;
#48800=CARTESIAN_POINT ( 'NONE',  ( 26.78025984663613812, 31.16454794089042579, -10.00000000000000355 ) ) ;
#48803=CARTESIAN_POINT ( 'NONE',  ( 87.45543461181301836, 45.01664465679169780, 6.930016242323781661 ) ) ;
#48806=ORIENTED_EDGE ( 'NONE', *, *, #44451, .F. ) ;
#48809=CARTESIAN_POINT ( 'NONE',  ( 86.72009611066519597, 47.05274629621921889, 10.38319007345879541 ) ) ;
#48814=CARTESIAN_POINT ( 'NONE',  ( 78.38473537823422532, 61.45169569177851088, -15.84070094600075684 ) ) ;
#48815=CARTESIAN_POINT ( 'NONE',  ( 85.19897760540997922, 48.35682075688382042, -11.91179608430785208 ) ) ;
#48816=CARTESIAN_POINT ( 'NONE',  ( 77.38344707992527560, 49.10671604805792612, -15.27628165681131200 ) ) ;
#48822=CARTESIAN_POINT ( 'NONE',  ( 40.07751882555258049, 24.10801979619931501, 3.090169943749476733 ) ) ;
#48825=CARTESIAN_POINT ( 'NONE',  ( 33.16502987395432456, 42.08080186712595605, -3.090169943749475845 ) ) ;
#48826=EDGE_LOOP ( 'NONE', ( #24024, #12661, #31005, #62111 ) ) ;
#48827=EDGE_CURVE ( 'NONE', #329, #7306, #46337, .T. ) ;
#48832=CARTESIAN_POINT ( 'NONE',  ( 67.71970704014216835, 67.69221244699392059, 7.277574328431961170 ) ) ;
#48837=CARTESIAN_POINT ( 'NONE',  ( 71.17403661793173342, 68.90151599838424090, 8.574984275677001833 ) ) ;
#48840=CARTESIAN_POINT ( 'NONE',  ( 82.41797270617800564, 53.48512899883142779, -15.75897339677477937 ) ) ;
#48842=VERTEX_POINT ( 'NONE', #33675 ) ;
#48844=CARTESIAN_POINT ( 'NONE',  ( 24.68213521633936836, 16.11110640527292759, -2.839279412974138328 ) ) ;
#48848=ORIENTED_EDGE ( 'NONE', *, *, #68274, .F. ) ;
#48851=CARTESIAN_POINT ( 'NONE',  ( 36.03373902044236132, 43.73705186507757503, -3.090169943749475845 ) ) ;
#48853=B_SPLINE_CURVE_WITH_KNOTS ( 'NONE', 3,
 ( #30814, #13135, #37397, #6012, #90669, #36905, #91643, #43993, #99726, #74935, #22210, #84064, #37890, #100228, #29320, #68798, #61694, #91148, #30312, #61198, #14618, #83553, #14118, #5518, #75944, #6521, #68302, #99225, #45497, #92646, #23195, #7003, #92166, #22717, #53596, #85041, #9528, #32805, #85565, #93139, #39880, #32305, #70816, #31789, #2430, #62691 ),
 .UNSPECIFIED., .F., .F.,
 ( 4, 1, 1, 1, 2, 2, 1, 1, 1, 2, 2, 1, 1, 2, 2, 1, 1, 2, 2, 1, 1, 2, 2, 1, 2, 2, 1, 2, 2, 4 ),
 ( 0.000000000000000000, 0.06249999999998029354, 0.09374999999997235545, 0.1093749999999686084, 0.1171874999999683725, 0.1249999999999681366, 0.1874999999999587830, 0.2187499999999538425, 0.2343749999999514277, 0.2421874999999502343, 0.2499999999999490408, 0.3124999999999495404, 0.3437499999999494849, 0.3593749999999494293, 0.3749999999999493183, 0.4374999999999565903, 0.4687499999999620304, 0.4843749999999648059, 0.4999999999999675815, 0.5624999999999735767, 0.5937499999999764633, 0.6093749999999774625, 0.6249999999999785727, 0.6874999999999792388, 0.7187499999999815703, 0.7499999999999837907, 0.8124999999999882316, 0.8437499999999902300, 0.8749999999999921174, 1.000000000000000000 ),
 .UNSPECIFIED. ) ;
#48856=ORIENTED_EDGE ( 'NONE', *, *, #22761, .F. ) ;
#48858=CARTESIAN_POINT ( 'NONE',  ( 5.294102074706517058, 26.55466486950697558, -1.111400068045478839E-16 ) ) ;
#48864=CARTESIAN_POINT ( 'NONE',  ( 82.10501726141201573, 40.76148666933337239, -0.9869235838961029073 ) ) ;
#48872=CARTESIAN_POINT ( 'NONE',  ( 68.21128839155480250, 69.77371198540542707, 2.434279403033834388 ) ) ;
#48873=CARTESIAN_POINT ( 'NONE',  ( 82.63815169587347498, 41.85270833316975825, 4.777311450696864803 ) ) ;
#48877=CARTESIAN_POINT ( 'NONE',  ( 73.98570270871888965, 68.92876820612471533, -11.10152750440661684 ) ) ;
#48880=CARTESIAN_POINT ( 'NONE',  ( 84.41763424635644242, 48.60878372575622564, 12.39659109532091641 ) ) ;
#48882=EDGE_CURVE ( 'NONE', #90329, #14068, #94496, .T. ) ;
#48884=CARTESIAN_POINT ( 'NONE',  ( 68.87871463239315517, 64.28074856791785407, -11.90835882824521796 ) ) ;
#48896=CARTESIAN_POINT ( 'NONE',  ( 21.77916244986271366, 18.28920272979926764, -7.433330006724141015 ) ) ;
#48908=CARTESIAN_POINT ( 'NONE',  ( 81.64224228150362705, 55.84784712173523502, -16.01176111343366770 ) ) ;
#48910=CARTESIAN_POINT ( 'NONE',  ( 72.87137282294411023, 65.35262256510435463, -13.40290358551061445 ) ) ;
#48915=CARTESIAN_POINT ( 'NONE',  ( 79.80408092812572818, 52.66049817665187760, 15.49629232015225000 ) ) ;
#48917=CARTESIAN_POINT ( 'NONE',  ( 72.37288529989473318, 71.73372848700918780, -5.731447342215284735 ) ) ;
#48921=CARTESIAN_POINT ( 'NONE',  ( 6.591042624459347188, 19.50829794293877839, -10.00000000000000355 ) ) ;
#48924=CARTESIAN_POINT ( 'NONE',  ( 77.98425798866018965, 61.79443237021894930, 16.07418881765924823 ) ) ;
#48926=CARTESIAN_POINT ( 'NONE',  ( 85.63227550969774882, 43.97216078338577461, -6.976400197485735255 ) ) ;
#48932=CARTESIAN_POINT ( 'NONE',  ( 80.49435834713268889, 44.43729004761577528, 11.36066671759673241 ) ) ;
#48933=CARTESIAN_POINT ( 'NONE',  ( 84.74798064930895691, 49.97902072749974423, -13.66263633214625806 ) ) ;
#48944=CARTESIAN_POINT ( 'NONE',  ( 78.63153613502940686, 50.56850472993508561, 15.05419567323381536 ) ) ;
#48947=CARTESIAN_POINT ( 'NONE',  ( 78.75297625639956323, 47.66336229257158408, 14.29739783539338482 ) ) ;
#48953=CARTESIAN_POINT ( 'NONE',  ( 84.18924544147772338, 41.92290757784675748, -3.949398286619972165 ) ) ;
#48957=CARTESIAN_POINT ( 'NONE',  ( 70.79161049076395784, 61.41985499215619626, -14.84464568873325518 ) ) ;
#48959=CARTESIAN_POINT ( 'NONE',  ( 24.00897855452593888, 29.56454794089042082, 10.00000000000000355 ) ) ;
#48967=CARTESIAN_POINT ( 'NONE',  ( 77.95436975687957215, 48.11784896437988834, 14.20357318872344621 ) ) ;
#48972=CARTESIAN_POINT ( 'NONE',  ( 65.73886374032248625, 69.08165079949409915, -0.06455758818544669875 ) ) ;
#48973=ORIENTED_EDGE ( 'NONE', *, *, #6421, .F. ) ;
#48983=AXIS2_PLACEMENT_3D ( 'NONE', #31564, #45278, #23463 ) ;
#48986=CARTESIAN_POINT ( 'NONE',  ( 76.45572749640668064, 51.64231386250387601, -16.15369532800221819 ) ) ;
#48989=CARTESIAN_POINT ( 'NONE',  ( 75.87525401958798454, 64.72722897157592570, -14.29033900848947169 ) ) ;
#48991=CARTESIAN_POINT ( 'NONE',  ( 80.75774510745969792, 43.20856077877414236, -9.122087061355482973 ) ) ;
#48996=CARTESIAN_POINT ( 'NONE',  ( 88.19817206715259772, 44.49282453600611831, -4.737833512016797144 ) ) ;
#49000=EDGE_CURVE ( 'NONE', #31328, #65871, #66059, .T. ) ;
#49008=CARTESIAN_POINT ( 'NONE',  ( 77.99682093914630343, 55.11119047563809659, -16.10778797222130621 ) ) ;
#49009=CYLINDRICAL_SURFACE ( 'NONE', #33420, 16.60714546451156792 ) ;
#49010=EDGE_CURVE ( 'NONE', #69987, #14298, #72697, .T. ) ;
#49011=CARTESIAN_POINT ( 'NONE',  ( 73.64088816139484095, 69.63733386616164012, 10.15931356738738423 ) ) ;
#49022=CARTESIAN_POINT ( 'NONE',  ( 26.97895004263468266, 38.68290643055188838, 3.479690158560446702E-15 ) ) ;
#49023=CARTESIAN_POINT ( 'NONE',  ( 82.34816312114848813, 49.74663056318024701, 14.30763284621803244 ) ) ;
#49024=CARTESIAN_POINT ( 'NONE',  ( 84.83591964108416050, 46.74628741325042114, -10.57126189487417633 ) ) ;
#49035=CARTESIAN_POINT ( 'NONE',  ( 87.53367671268780725, 44.88112536278567433, -6.578546970659244764 ) ) ;
#49037=CARTESIAN_POINT ( 'NONE',  ( 74.82952949953238431, 53.40084132974138953, 16.53760015760405722 ) ) ;
#49039=CARTESIAN_POINT ( 'NONE',  ( 82.07496931413966479, 54.01582194328672415, 15.59905118150530967 ) ) ;
#49040=ORIENTED_EDGE ( 'NONE', *, *, #69955, .F. ) ;
#49043=CARTESIAN_POINT ( 'NONE',  ( 73.00396795756827828, 57.62093675928252878, -16.32480838619500219 ) ) ;
#49050=ORIENTED_EDGE ( 'NONE', *, *, #21817, .T. ) ;
#49051=CARTESIAN_POINT ( 'NONE',  ( 30.86762485498029207, 38.79752408145594700, -5.678558825948271327 ) ) ;
#49052=CARTESIAN_POINT ( 'NONE',  ( 80.14444365492592226, 44.30149127559567290, 11.42155680931026573 ) ) ;
#49053=CARTESIAN_POINT ( 'NONE',  ( 84.88199885514633536, 50.20673742124042604, -13.33258340498515437 ) ) ;
#49056=AXIS2_PLACEMENT_3D ( 'NONE', #52727, #33442, #64340 ) ;
#49057=FACE_OUTER_BOUND ( 'NONE', #30099, .T. ) ;
#49060=EDGE_LOOP ( 'NONE', ( #51663, #32754, #78592, #21335 ) ) ;
#49064=CARTESIAN_POINT ( 'NONE',  ( 81.45669997382150029, 55.98862135975878118, -16.04303691645969820 ) ) ;
#49067=CARTESIAN_POINT ( 'NONE',  ( 70.34454795188869980, 61.29844696716961749, 14.78467410895967760 ) ) ;
#49076=CARTESIAN_POINT ( 'NONE',  ( 74.62401959271109320, 66.89443057110609914, 13.05059976691390311 ) ) ;
#49080=CARTESIAN_POINT ( 'NONE',  ( 80.42297664653236211, 44.73783946406587830, -11.66823080374195420 ) ) ;
#49081=FACE_OUTER_BOUND ( 'NONE', #12674, .T. ) ;
#49083=CARTESIAN_POINT ( 'NONE',  ( 83.90325127553046514, 41.85121661673234428, -1.721470070664741225 ) ) ;
#49087=ORIENTED_EDGE ( 'NONE', *, *, #34396, .F. ) ;
#49091=CARTESIAN_POINT ( 'NONE',  ( 31.17504386912796477, 20.12755873383627758, -6.180339887498949025 ) ) ;
#49092=CARTESIAN_POINT ( 'NONE',  ( 70.71923034029678945, 69.39805573920016002, -7.454743742243774562 ) ) ;
#49093=CARTESIAN_POINT ( 'NONE',  ( 87.77567103309253582, 45.10408226285451150, -6.743331934586553444 ) ) ;
#49095=CARTESIAN_POINT ( 'NONE',  ( 87.92412256492882250, 44.79819542341160599, 4.880203861778121599 ) ) ;
#49096=VERTEX_POINT ( 'NONE', #92871 ) ;
#49099=CARTESIAN_POINT ( 'NONE',  ( 81.96852851063667345, 40.98455881841368154, -3.062051805011598571 ) ) ;
#49107=CARTESIAN_POINT ( 'NONE',  ( 84.37722046559913736, 42.81587621694462342, 4.768053884619589233 ) ) ;
#49108=CARTESIAN_POINT ( 'NONE',  ( 24.77599400646307970, 14.70852965304480087, 1.583844403245364907 ) ) ;
#49112=VERTEX_POINT ( 'NONE', #60926 ) ;
#49121=CARTESIAN_POINT ( 'NONE',  ( 40.07751882555258049, 24.10801979619931501, 3.090169943749476733 ) ) ;
#49129=CARTESIAN_POINT ( 'NONE',  ( 81.36240293647936994, 45.51711427137305321, 11.23452077343203115 ) ) ;
#49132=CARTESIAN_POINT ( 'NONE',  ( 87.06988255670405863, 46.05766899987094831, 8.936389965629217613 ) ) ;
#49133=CARTESIAN_POINT ( 'NONE',  ( 30.64569906364082641, 29.64441083166262558, -10.00000000000000533 ) ) ;
#49134=CARTESIAN_POINT ( 'NONE',  ( 81.88434891954030093, 41.68080424094055303, 5.410084833112948743 ) ) ;
#49138=CARTESIAN_POINT ( 'NONE',  ( 39.48212635690286021, 23.76426979415093044, 3.090169943749476733 ) ) ;
#49147=CARTESIAN_POINT ( 'NONE',  ( 83.78171082742430542, 51.97306301863909539, 14.95037678041454932 ) ) ;
#49148=EDGE_CURVE ( 'NONE', #14885, #72252, #85285, .T. ) ;
#49157=CARTESIAN_POINT ( 'NONE',  ( 67.23736956560070155, 67.19511859228909145, -8.571709603932553989 ) ) ;
#49162=CARTESIAN_POINT ( 'NONE',  ( 72.12749769884386808, 68.75288622073954059, 10.17241042758247183 ) ) ;
#49163=CARTESIAN_POINT ( 'NONE',  ( 31.43713336585798146, 20.01110640527293683, 2.839279412974134775 ) ) ;
#49168=CARTESIAN_POINT ( 'NONE',  ( 21.04482852044473162, 14.01110640527291906, 2.839279412974134775 ) ) ;
#49169=B_SPLINE_CURVE_WITH_KNOTS ( 'NONE', 3,
 ( #25817, #80037, #4492, #27798, #58672, #89644, #51076, #56693, #82038, #12613 ),
 .UNSPECIFIED., .F., .F.,
 ( 4, 2, 2, 2, 4 ),
 ( 0.000000000000000000, 0.0002622400424273094513, 0.0005244800848546189026, 0.0007867201272819283539, 0.001048960169709237805 ),
 .UNSPECIFIED. ) ;
#49172=CARTESIAN_POINT ( 'NONE',  ( 77.56105267981615725, 49.72783448595330213, -15.46007777815280981 ) ) ;
#49178=CARTESIAN_POINT ( 'NONE',  ( 68.61392852225033323, 65.52134601779788170, -11.40821467630667563 ) ) ;
#49185=CARTESIAN_POINT ( 'NONE',  ( 45.27367124825920541, 27.10801979619933277, 3.090169943749476733 ) ) ;
#49187=CARTESIAN_POINT ( 'NONE',  ( 73.06484434959700991, 57.43056366546561975, -15.87593782397910402 ) ) ;
#49188=CARTESIAN_POINT ( 'NONE',  ( 77.99401760355904401, 61.40429962668400776, -16.15929906019731632 ) ) ;
#49191=ADVANCED_FACE ( 'NONE', ( #53337 ), #52340, .T. ) ;
#49194=EDGE_CURVE ( 'NONE', #77668, #79774, #84290, .T. ) ;
#49199=CARTESIAN_POINT ( 'NONE',  ( 30.33837380989695731, 32.91421378149920685, 9.188101187500008038 ) ) ;
#49204=CARTESIAN_POINT ( 'NONE',  ( 74.35260113823048300, 68.48135296369000002, 11.70560402319360449 ) ) ;
#49210=CARTESIAN_POINT ( 'NONE',  ( 73.78529867857243119, 58.81232895305485187, -15.71900575702707847 ) ) ;
#49215=CARTESIAN_POINT ( 'NONE',  ( 68.62755322380348844, 69.49084673843516669, -4.507018638050549697 ) ) ;
#49227=CARTESIAN_POINT ( 'NONE',  ( 84.46936203225826034, 42.55036768791385526, 3.687038961768065448 ) ) ;
#49229=CARTESIAN_POINT ( 'NONE',  ( 79.45058217612400142, 59.65650951519399570, -16.18060345040571590 ) ) ;
#49230=CARTESIAN_POINT ( 'NONE',  ( 73.91967031219644468, 56.99378804825083478, 16.01627465200614964 ) ) ;
#49233=CARTESIAN_POINT ( 'NONE',  ( 80.45778748667572700, 57.56998633490270123, -16.59146305250142817 ) ) ;
#49240=CARTESIAN_POINT ( 'NONE',  ( 68.18175421089479471, 69.02745595044970628, 5.050215709098530681 ) ) ;
#49249=CARTESIAN_POINT ( 'NONE',  ( 77.67544480499739734, 52.83525693180617111, -15.78147281318218198 ) ) ;
#49257=CARTESIAN_POINT ( 'NONE',  ( 17.74301629803562719, 32.01751292744057054, 6.180339887498949913 ) ) ;
#49258=CARTESIAN_POINT ( 'NONE',  ( 85.69655150396907572, 48.70939609366209311, 11.94995701397517784 ) ) ;
#49259=CARTESIAN_POINT ( 'NONE',  ( 66.14445876615877751, 69.31385697677988844, 0.2434306055318663509 ) ) ;
#49262=CARTESIAN_POINT ( 'NONE',  ( 73.75732063271028949, 55.42083462481677003, -16.58942913474808734 ) ) ;
#49269=CARTESIAN_POINT ( 'NONE',  ( 88.45958475239287111, 43.85926912372239173, -0.5941283661710181629 ) ) ;
#49274=CARTESIAN_POINT ( 'NONE',  ( 35.70653501523218409, 32.56628583063843507, 9.188101187500006262 ) ) ;
#49276=CYLINDRICAL_SURFACE ( 'NONE', #84067, 10.00000000000001066 ) ;
#49277=CARTESIAN_POINT ( 'NONE',  ( 27.52682148520507965, 37.93396525600392266, 2.839279412974139660 ) ) ;
#49281=CARTESIAN_POINT ( 'NONE',  ( 80.76024885531072073, 43.13123959331257851, -9.841151695238801622 ) ) ;
#49284=CARTESIAN_POINT ( 'NONE',  ( 4.685401460390529849, 24.74646525600388003, 2.839279412974139660 ) ) ;
#49286=CARTESIAN_POINT ( 'NONE',  ( 10.40777469057294091, 26.98502408145591502, -5.678558825948271327 ) ) ;
#49289=CARTESIAN_POINT ( 'NONE',  ( 84.46699969863880142, 49.90279977532637901, -13.71381277893580197 ) ) ;
#49291=VERTEX_POINT ( 'NONE', #32025 ) ;
#49294=CARTESIAN_POINT ( 'NONE',  ( 66.07429888242232607, 68.52750538357182108, 4.592745147667558037 ) ) ;
#49299=ORIENTED_EDGE ( 'NONE', *, *, #6057, .F. ) ;
#49302=CARTESIAN_POINT ( 'NONE',  ( 86.10592739760618031, 47.67974530001434630, 10.86095660826619813 ) ) ;
#49304=CARTESIAN_POINT ( 'NONE',  ( 78.22302278738825976, 60.67164067339659539, 15.94566782436302610 ) ) ;
#49307=CARTESIAN_POINT ( 'NONE',  ( 79.35772302032123093, 59.09242961143867490, -16.22768995670567094 ) ) ;
#49309=CARTESIAN_POINT ( 'NONE',  ( 80.75624902194448396, 43.07755972626095087, 9.780254146993412334 ) ) ;
#49310=EDGE_LOOP ( 'NONE', ( #89155, #16405, #39783, #14285 ) ) ;
#49313=CARTESIAN_POINT ( 'NONE',  ( 73.43553217956821300, 58.62768804998614769, 15.70915590920282945 ) ) ;
#49318=EDGE_LOOP ( 'NONE', ( #34333, #5432, #46062, #82971 ) ) ;
#49324=DIRECTION ( 'NONE',  ( -0.1378186779084930869, 0.2387089523694814197, -0.9612616959383223358 ) ) ;
#49328=CARTESIAN_POINT ( 'NONE',  ( 69.55475657562975300, 65.34938856974197563, 11.35858988098566513 ) ) ;
#49330=LINE ( 'NONE', #53779, #4676 ) ;
#49333=CARTESIAN_POINT ( 'NONE',  ( 18.13223351794271565, 28.65586893147756342, -7.433330006724137462 ) ) ;
#49335=CARTESIAN_POINT ( 'NONE',  ( 77.38371485743755329, 49.76092087919086282, -14.99339166432857162 ) ) ;
#49341=CARTESIAN_POINT ( 'NONE',  ( 69.35253854976203058, 63.01665765323906498, 13.58811665770852350 ) ) ;
#49343=CARTESIAN_POINT ( 'NONE',  ( 78.90549422596571105, 46.47045305960070039, 12.99985401326297563 ) ) ;
#49352=CARTESIAN_POINT ( 'NONE',  ( 82.57385212973971989, 41.04541115053231692, -1.138833187496895549 ) ) ;
#49360=CARTESIAN_POINT ( 'NONE',  ( 67.40381412284057205, 69.04098650065962772, 3.573880184651055281 ) ) ;
#49361=CARTESIAN_POINT ( 'NONE',  ( 82.81329010676300584, 42.04495716520958126, 5.036686735886401145 ) ) ;
#49369=CARTESIAN_POINT ( 'NONE',  ( 83.65721968253822638, 46.40063887978691781, 10.86318306393037503 ) ) ;
#49373=CARTESIAN_POINT ( 'NONE',  ( 68.50152299929102639, 64.46762139964850746, -12.23471630616243822 ) ) ;
#49382=ORIENTED_EDGE ( 'NONE', *, *, #56085, .T. ) ;
#49387=CARTESIAN_POINT ( 'NONE',  ( 14.21828646722447154, 29.18502408145591431, 5.678558825948277544 ) ) ;
#49396=CARTESIAN_POINT ( 'NONE',  ( 75.75493378409400691, 65.86437009324527025, -14.07593894684413804 ) ) ;
#49398=CARTESIAN_POINT ( 'NONE',  ( 81.49529596843051138, 56.10236560196279498, -16.41626961062114987 ) ) ;
#49399=VERTEX_POINT ( 'NONE', #66919 ) ;
#49405=CARTESIAN_POINT ( 'NONE',  ( 83.66191979497145326, 52.22800872522471138, -14.69070669276292662 ) ) ;
#49406=CARTESIAN_POINT ( 'NONE',  ( 72.18714191131631708, 71.56775394826222225, -5.867817691062866103 ) ) ;
#49410=CARTESIAN_POINT ( 'NONE',  ( 6.214053113703209341, 25.36126292948893024, 6.180339887498949913 ) ) ;
#49413=CARTESIAN_POINT ( 'NONE',  ( 77.95656630038031665, 61.79485276963480089, 16.07049939491896495 ) ) ;
#49421=CARTESIAN_POINT ( 'NONE',  ( 76.57758696453686298, 52.46645809405062266, -15.82665826843820867 ) ) ;
#49433=CARTESIAN_POINT ( 'NONE',  ( 82.43550774211716714, 40.72616915719758879, 3.190364828977913625 ) ) ;
#49435=FACE_OUTER_BOUND ( 'NONE', #42416, .T. ) ;
#49441=CARTESIAN_POINT ( 'NONE',  ( 70.41672140557730586, 61.20692221393646548, -14.84313828059261020 ) ) ;
#49442=CARTESIAN_POINT ( 'NONE',  ( 43.88624854525928498, 27.19860640527296169, 2.839279412974134775 ) ) ;
#49446=CARTESIAN_POINT ( 'NONE',  ( 85.65412827366334625, 48.89905674914069067, -12.59087409094111543 ) ) ;
#49455=CARTESIAN_POINT ( 'NONE',  ( 76.47316661484272515, 51.61210842333346704, -15.65491330287230376 ) ) ;
#49457=ORIENTED_EDGE ( 'NONE', *, *, #72475, .F. ) ;
#49459=CARTESIAN_POINT ( 'NONE',  ( 65.75045340966318008, 69.08842219619184277, 0.01581025732398740752 ) ) ;
#49468=CARTESIAN_POINT ( 'NONE',  ( 88.01292981757310940, 43.79437901572622849, 2.423352920943453892 ) ) ;
#49471=CARTESIAN_POINT ( 'NONE',  ( 76.63557502497172891, 60.94970092050591148, -15.67532736481255107 ) ) ;
#49476=CARTESIAN_POINT ( 'NONE',  ( 80.90448388914862221, 43.66277003455212480, -9.563369884905593921 ) ) ;
#49482=CARTESIAN_POINT ( 'NONE',  ( 88.05604604623943032, 44.30204071979397185, -4.408624695025149087 ) ) ;
#49483=CARTESIAN_POINT ( 'NONE',  ( 66.77752810875767864, 68.40544692769400115, 4.459354299965320401 ) ) ;
#49485=FACE_OUTER_BOUND ( 'NONE', #36968, .T. ) ;
#49486=CARTESIAN_POINT ( 'NONE',  ( 75.44349275752195183, 55.11585462790367984, -16.13645090372341073 ) ) ;
#49493=CARTESIAN_POINT ( 'NONE',  ( 78.94459720937796021, 54.75824911672975759, -16.02467863901235390 ) ) ;
#49501=CARTESIAN_POINT ( 'NONE',  ( 79.41912790878161843, 52.36421636274327085, -15.93798156132412380 ) ) ;
#49506=AXIS2_PLACEMENT_3D ( 'NONE', #14072, #83510, #23147 ) ;
#49507=CARTESIAN_POINT ( 'NONE',  ( 31.10096393961467598, 36.14336893147757479, 7.433330006724141015 ) ) ;
#49511=CARTESIAN_POINT ( 'NONE',  ( 15.40246583222295129, 30.93396525600389424, 2.839279412974139660 ) ) ;
#49518=DIRECTION ( 'NONE',  ( -0.8660254037844378194, -0.5000000000000014433, -0.000000000000000000 ) ) ;
#49519=CARTESIAN_POINT ( 'NONE',  ( 82.56047309644807797, 54.07683023134062239, -15.52634518316282630 ) ) ;
#49520=CARTESIAN_POINT ( 'NONE',  ( 72.27728550995250600, 71.54023409894355723, 5.041877779019897865 ) ) ;
#49521=CARTESIAN_POINT ( 'NONE',  ( 87.45985321408362267, 44.85427673109838764, -6.610136163016259836 ) ) ;
#49524=CARTESIAN_POINT ( 'NONE',  ( 74.87825199367567564, 53.25176599458816185, 16.52284144418170797 ) ) ;
#49526=CARTESIAN_POINT ( 'NONE',  ( 85.26933297508705323, 45.86091332672160803, 9.343335550192509942 ) ) ;
#49530=CARTESIAN_POINT ( 'NONE',  ( 72.84093999290328725, 56.97456911652175648, -16.40692799624908815 ) ) ;
#49532=CARTESIAN_POINT ( 'NONE',  ( 77.05346401475797791, 63.67418989607284630, -14.99496270919825136 ) ) ;
#49540=CARTESIAN_POINT ( 'NONE',  ( 30.25658917092484756, 35.65586893147758474, -7.433330006724137462 ) ) ;
#49541=CARTESIAN_POINT ( 'NONE',  ( 86.30977306730703447, 47.58285218899635538, -10.62438056216880611 ) ) ;
#49546=ORIENTED_EDGE ( 'NONE', *, *, #72238, .T. ) ;
#49565=CARTESIAN_POINT ( 'NONE',  ( 80.22848430713953860, 44.69384781298665388, -11.72783283579514979 ) ) ;
#49567=CARTESIAN_POINT ( 'NONE',  ( 38.03700799836438051, 22.36477965099642518, 1.583844403245330712 ) ) ;
#49576=CARTESIAN_POINT ( 'NONE',  ( 31.79297225648316427, 18.75978393459166682, -1.583844403245396437 ) ) ;
#49585=CARTESIAN_POINT ( 'NONE',  ( 81.24301197013335241, 47.20210463093496145, 12.61345882853937539 ) ) ;
#49595=CARTESIAN_POINT ( 'NONE',  ( 82.65284874209399391, 41.20956459249614312, 2.251177775424070937 ) ) ;
#49597=CARTESIAN_POINT ( 'NONE',  ( 78.43012671350176390, 61.37287260322700888, 16.21548333613125692 ) ) ;
#49602=CARTESIAN_POINT ( 'NONE',  ( 73.51359153202696461, 64.16502688528564136, -13.81845228444169926 ) ) ;
#49607=CARTESIAN_POINT ( 'NONE',  ( 33.07613030564196777, 37.83478043621391151, -8.090169943749479842 ) ) ;
#49611=CARTESIAN_POINT ( 'NONE',  ( 34.14357333472769085, 43.21091486745863364, 7.012934429366973338E-14 ) ) ;
#49617=EDGE_CURVE ( 'NONE', #91729, #44705, #67844, .T. ) ;
#49618=CARTESIAN_POINT ( 'NONE',  ( 86.65718700450617007, 46.39925006966746679, 9.083952274210956190 ) ) ;
#49619=CARTESIAN_POINT ( 'NONE',  ( 17.08077532425043543, 25.56454794089041371, 10.00000000000000355 ) ) ;
#49620=CARTESIAN_POINT ( 'NONE',  ( 82.00684797933710968, 41.19628710175830832, 5.481709446181254997 ) ) ;
#49622=CARTESIAN_POINT ( 'NONE',  ( 87.37955803993382631, 45.91052472906853410, 8.478299845497456744 ) ) ;
#49624=CARTESIAN_POINT ( 'NONE',  ( 37.84453522905105416, 33.80066082961425167, 10.00000000000000533 ) ) ;
#49629=LINE ( 'NONE', #72965, #64633 ) ;
#49632=DIRECTION ( 'NONE',  ( -0.8660254037844379305, -0.5000000000000014433, -0.000000000000000000 ) ) ;
#49633=CARTESIAN_POINT ( 'NONE',  ( 32.66923259237032084, 34.56454794089044213, 10.00000000000000355 ) ) ;
#49639=ORIENTED_EDGE ( 'NONE', *, *, #3307, .T. ) ;
#49643=CARTESIAN_POINT ( 'NONE',  ( 31.98500480842837490, 19.26216523072496400, -2.296566073217252530E-15 ) ) ;
#49645=CARTESIAN_POINT ( 'NONE',  ( 86.41573892179229688, 47.05171444917584012, -10.02785938301615687 ) ) ;
#49650=CARTESIAN_POINT ( 'NONE',  ( 20.49695707787433463, 14.76004757982089188, 5.678558825948272215 ) ) ;
#49655=CARTESIAN_POINT ( 'NONE',  ( 72.18714191131631708, 71.56775394826222225, -5.867817691062866103 ) ) ;
#49669=CARTESIAN_POINT ( 'NONE',  ( 72.71298963066548993, 57.56606450374060557, -16.30620737163571476 ) ) ;
#49670=CARTESIAN_POINT ( 'NONE',  ( 78.21587680839553514, 61.74396432438783222, -15.75068414206376843 ) ) ;
#49674=EDGE_CURVE ( 'NONE', #52768, #26530, #14613, .T. ) ;
#49679=CARTESIAN_POINT ( 'NONE',  ( 35.22902474502244274, 28.84335787977765619, 9.188101187500006262 ) ) ;
#49681=CARTESIAN_POINT ( 'NONE',  ( 66.36121846479309738, 69.42315429199126697, -0.9703253544482470794 ) ) ;
#49682=EDGE_CURVE ( 'NONE', #14203, #53284, #82566, .T. ) ;
#49684=CARTESIAN_POINT ( 'NONE',  ( 73.76584831522593788, 68.38082682530667000, 10.99424229391076402 ) ) ;
#49689=CARTESIAN_POINT ( 'NONE',  ( 78.87565597274867457, 57.06976691274630298, -16.20268086563066845 ) ) ;
#49691=CARTESIAN_POINT ( 'NONE',  ( 83.98748035737914108, 42.88667253378446986, -5.474467086385531367 ) ) ;
#49692=CARTESIAN_POINT ( 'NONE',  ( 78.14496247000307960, 54.23761980304868047, 16.42853692188513293 ) ) ;
#49695=CARTESIAN_POINT ( 'NONE',  ( 68.13387999444950083, 69.36173196781918193, -3.979686392102562920 ) ) ;
#49696=ADVANCED_FACE ( 'NONE', ( #99220 ), #68410, .T. ) ;
#49697=CYLINDRICAL_SURFACE ( 'NONE', #82320, 10.00000000000001066 ) ;
#49708=CARTESIAN_POINT ( 'NONE',  ( 82.28868876057151738, 44.23413057205505794, -9.339634112966722412 ) ) ;
#49714=CARTESIAN_POINT ( 'NONE',  ( 76.14472760179803856, 51.53489781101264100, -15.67783219047871235 ) ) ;
#49716=CARTESIAN_POINT ( 'NONE',  ( 80.29526846451028632, 57.41841621455482425, -16.58920233904881414 ) ) ;
#49717=CARTESIAN_POINT ( 'NONE',  ( 71.63453813518020752, 72.07236434383467838, 0.7172108931481352423 ) ) ;
#49719=FACE_OUTER_BOUND ( 'NONE', #51527, .T. ) ;
#49724=CARTESIAN_POINT ( 'NONE',  ( 68.91580955978653833, 69.84068243732808412, 3.940511651554692740 ) ) ;
#49731=B_SPLINE_SURFACE_WITH_KNOTS ( 'NONE', 3, 1, ( 
 ( #19740, #18733 ),
 ( #41511, #42499 ),
 ( #81074, #10636 ),
 ( #20230, #57209 ),
 ( #4514, #66321 ),
 ( #97254, #95779 ),
 ( #26332, #87702 ),
 ( #95283, #50605 ),
 ( #3545, #35908 ),
 ( #34422, #19255 ),
 ( #12127, #81559 ),
 ( #51101, #73928 ),
 ( #42991, #26827 ),
 ( #50121, #82067 ),
 ( #43507, #35413 ),
 ( #49132, #33946 ),
 ( #12636, #74446 ),
 ( #65805, #88684 ),
 ( #73435, #27331 ),
 ( #27819, #5027 ),
 ( #58213, #11640 ),
 ( #64833, #88186 ),
 ( #57706, #49618 ),
 ( #80571, #65323 ),
 ( #58695, #89191 ),
 ( #96260, #25845 ),
 ( #89669, #11149 ),
 ( #18236, #42018 ),
 ( #4021, #56720 ),
 ( #80066, #72453 ),
 ( #72952, #34904 ) ),
 .UNSPECIFIED., .F., .F., .F.,
 ( 4, 3, 3, 3, 3, 3, 3, 3, 3, 3, 4 ),
 ( 2, 2 ),
 ( 0.000000000000000000, 0.1333490885032313222, 0.3007194338854242699, 0.4699862290244929963, 0.5844252810809240639, 0.6686540514502682386, 0.7354980260655500368, 0.8028463152565734617, 0.8633854507757154906, 0.9437142632667211428, 1.000000000000000000 ),
 ( 0.000000000000000000, 1.000000000000000000 ),
 .UNSPECIFIED. ) ;
#49732=CARTESIAN_POINT ( 'NONE',  ( 22.93021583062070690, 14.20801979619928623, -3.090169943749474069 ) ) ;
#49740=CARTESIAN_POINT ( 'NONE',  ( 81.87873318869407058, 51.48326241843163587, -14.75192784692151626 ) ) ;
#49741=EDGE_LOOP ( 'NONE', ( #12479, #89055, #26118, #28256 ) ) ;
#49748=CARTESIAN_POINT ( 'NONE',  ( 19.85205661636063468, 27.16454794089041869, -10.00000000000000355 ) ) ;
#49749=CARTESIAN_POINT ( 'NONE',  ( 67.96946636730157820, 65.22418645040922058, -10.61429169278184759 ) ) ;
#49750=VECTOR ( 'NONE', #23398, 1000.000000000000114 ) ;
#49752=CARTESIAN_POINT ( 'NONE',  ( 72.30049733009887802, 72.04291962484111878, -3.432230885200083126 ) ) ;
#49754=CARTESIAN_POINT ( 'NONE',  ( 74.22542230801622054, 55.48368813609693007, -16.11996396474174631 ) ) ;
#49758=CARTESIAN_POINT ( 'NONE',  ( 75.00251594304947389, 67.18370992929050090, 12.56202059610710720 ) ) ;
#49765=CARTESIAN_POINT ( 'NONE',  ( 38.30461122658549300, 34.06628583063844928, -9.188101187500006262 ) ) ;
#49768=CARTESIAN_POINT ( 'NONE',  ( 32.31339950491288704, 36.84336893147758474, -7.433330006724137462 ) ) ;
#49769=CARTESIAN_POINT ( 'NONE',  ( 27.64470315295111646, 16.36477965099641452, 1.583844403245364907 ) ) ;
#49775=CARTESIAN_POINT ( 'NONE',  ( 12.79414888559916719, 13.10170272979925166, -7.433330006724141015 ) ) ;
#49777=CARTESIAN_POINT ( 'NONE',  ( 19.43607595823839418, 14.14754757982089473, -5.678558825948275768 ) ) ;
#49785=CARTESIAN_POINT ( 'NONE',  ( 87.50902739619012038, 45.51716134564335903, 6.992071084032383865 ) ) ;
#49790=CARTESIAN_POINT ( 'NONE',  ( 86.32803123799460820, 47.24229282936711627, 10.81726845165080064 ) ) ;
#49792=CARTESIAN_POINT ( 'NONE',  ( 77.34314915561620296, 55.31099856840221918, 16.12525396489078844 ) ) ;
#49796=CARTESIAN_POINT ( 'NONE',  ( 81.82315253837346347, 49.37544138376473768, -13.78991541157006750 ) ) ;
#49799=CARTESIAN_POINT ( 'NONE',  ( 80.49441947199758829, 43.53112923038558790, 9.691460173197548045 ) ) ;
#49808=CARTESIAN_POINT ( 'NONE',  ( 42.14088959202413776, 24.73415679381825427, -6.890680421881970419E-14 ) ) ;
#49812=ORIENTED_EDGE ( 'NONE', *, *, #91875, .T. ) ;
#49819=CARTESIAN_POINT ( 'NONE',  ( 70.30547663914938994, 67.08293681328960645, 10.12933801363482544 ) ) ;
#49825=ORIENTED_EDGE ( 'NONE', *, *, #4201, .F. ) ;
#49827=CARTESIAN_POINT ( 'NONE',  ( 27.86299091144838869, 21.80170272979927404, 7.433330006724137462 ) ) ;
#49834=CARTESIAN_POINT ( 'NONE',  ( 35.83123663242427170, 44.18528772668522464, -1.583844403245329602 ) ) ;
#49842=VECTOR ( 'NONE', #82311, 1000.000000000000114 ) ;
#49848=CARTESIAN_POINT ( 'NONE',  ( 23.04394319889420828, 13.70852965304479554, 1.583844403245364907 ) ) ;
#49854=CARTESIAN_POINT ( 'NONE',  ( 79.60765542401018990, 47.14190884193141784, -13.17992671574433317 ) ) ;
#49855=CARTESIAN_POINT ( 'NONE',  ( 75.97349631671795578, 51.36067909666243025, 16.15326845647728149 ) ) ;
#49865=CARTESIAN_POINT ( 'NONE',  ( 84.80172950927561715, 50.19486025153374698, 13.34007759942641336 ) ) ;
#49872=CARTESIAN_POINT ( 'NONE',  ( 68.89679659267170564, 64.71313860959173780, -12.22090107332434528 ) ) ;
#49874=CARTESIAN_POINT ( 'NONE',  ( 79.06615046322909279, 46.00065692319815724, -12.62335963921513837 ) ) ;
#49880=EDGE_LOOP ( 'NONE', ( #44823, #78526, #87029, #85212 ) ) ;
#49886=CARTESIAN_POINT ( 'NONE',  ( 16.72494223679300873, 27.84336893147755987, -7.433330006724137462 ) ) ;
#49887=CARTESIAN_POINT ( 'NONE',  ( 75.19340432564982279, 67.01774300492178327, 13.18884388031393229 ) ) ;
#49892=FACE_OUTER_BOUND ( 'NONE', #45160, .T. ) ;
#49893=ORIENTED_EDGE ( 'NONE', *, *, #92162, .F. ) ;
#49898=CARTESIAN_POINT ( 'NONE',  ( 81.63517289312954972, 55.69097578121159131, -16.34528168754147259 ) ) ;
#49902=CARTESIAN_POINT ( 'NONE',  ( 71.83275678050461011, 72.56239119006679061, 1.040614184235704842 ) ) ;
#49903=CARTESIAN_POINT ( 'NONE',  ( 84.68632265823056571, 43.86313539936578110, 6.734552681056144685 ) ) ;
#49906=CARTESIAN_POINT ( 'NONE',  ( 72.03955433498997252, 71.50824183410490775, -5.808600603169774779 ) ) ;
#49911=CARTESIAN_POINT ( 'NONE',  ( 5.551812139918021138, 18.90829794293878408, 10.00000000000000355 ) ) ;
#49919=CARTESIAN_POINT ( 'NONE',  ( 79.15819921557465477, 59.82093924937031204, 16.50069780760282256 ) ) ;
#49925=CARTESIAN_POINT ( 'NONE',  ( 84.70734284140858961, 49.82661628013787691, -13.16822936550296319 ) ) ;
#49931=CARTESIAN_POINT ( 'NONE',  ( 77.32261477357617707, 49.49473738394384270, 14.91239470638691422 ) ) ;
#49932=ORIENTED_EDGE ( 'NONE', *, *, #72532, .T. ) ;
#49933=CARTESIAN_POINT ( 'NONE',  ( 74.82759778890250857, 57.94603759221541850, 15.96911003232950499 ) ) ;
#49942=CARTESIAN_POINT ( 'NONE',  ( 84.63373551891548630, 42.05073026052070162, -3.462570873098485436 ) ) ;
#49943=ADVANCED_FACE ( 'NONE', ( #73313 ), #49009, .T. ) ;
#49945=CARTESIAN_POINT ( 'NONE',  ( 73.28532805263516536, 68.06995479673437899, -11.00005841506875370 ) ) ;
#49947=CARTESIAN_POINT ( 'NONE',  ( 88.05115470054576576, 43.61122574602664059, 0.03890336903546996739 ) ) ;
#49948=CARTESIAN_POINT ( 'NONE',  ( 6.527493107231251201, 21.95586893147753216, 7.433330006724141015 ) ) ;
#49950=ORIENTED_EDGE ( 'NONE', *, *, #3463, .F. ) ;
#49958=EDGE_CURVE ( 'NONE', #37182, #18761, #52220, .T. ) ;
#49959=CARTESIAN_POINT ( 'NONE',  ( 78.71005434030972481, 51.00076188309252956, -15.65772236519125826 ) ) ;
#49963=CARTESIAN_POINT ( 'NONE',  ( 85.96821334696042527, 43.30321141303308963, 3.387204527858681313 ) ) ;
#49964=CARTESIAN_POINT ( 'NONE',  ( 88.45040933577318754, 44.05593677119288287, -2.476488480078137933 ) ) ;
#49968=CARTESIAN_POINT ( 'NONE',  ( 66.05101471070410923, 68.71202625984970780, 0.004290391756236853690 ) ) ;
#49972=DIRECTION ( 'NONE',  ( -0.9133924323370958831, 0.1624253398589842745, 0.3732723851572966600 ) ) ;
#49976=CARTESIAN_POINT ( 'NONE',  ( 88.42017002704760387, 43.92753743058676719, 1.721442031696310382 ) ) ;
#49981=CARTESIAN_POINT ( 'NONE',  ( 74.66876074730942037, 61.62064187642321400, -15.14846027550216867 ) ) ;
#49983=DIRECTION ( 'NONE',  ( 0.2702110370271901263, 0.9515975153008180420, -0.1464519181916028867 ) ) ;
#49984=DIRECTION ( 'NONE',  ( -0.4493970231495795775, 0.7783784768652820540, -0.4383711467890876734 ) ) ;
#49985=CARTESIAN_POINT ( 'NONE',  ( 81.05143020228690887, 43.40825155421170223, -9.967878382272422400 ) ) ;
#49987=EDGE_CURVE ( 'NONE', #62487, #10212, #38946, .T. ) ;
#49991=CARTESIAN_POINT ( 'NONE',  ( 88.09812594050896450, 44.33653194584124435, -4.440584375772049341 ) ) ;
#49993=DIRECTION ( 'NONE',  ( 0.5000000000000013323, -0.8660254037844378194, 0.000000000000000000 ) ) ;
#50001=CARTESIAN_POINT ( 'NONE',  ( 75.59167736239344038, 55.94695640115752866, -16.15688945000958299 ) ) ;
#50007=CARTESIAN_POINT ( 'NONE',  ( 73.13476967714908028, 57.39438153525127007, 15.88807208273858684 ) ) ;
#50012=CARTESIAN_POINT ( 'NONE',  ( 75.94843506473843320, 65.47918399976401815, 14.33637728062728200 ) ) ;
#50014=CARTESIAN_POINT ( 'NONE',  ( 31.70236382085744964, 33.70171378149921537, -9.188101187500004485 ) ) ;
#50016=CARTESIAN_POINT ( 'NONE',  ( 76.03008165241378435, 63.51276889911483181, 15.23596077392240211 ) ) ;
#50018=CARTESIAN_POINT ( 'NONE',  ( 17.52000153575897912, 22.06628583063841020, -9.188101187500006262 ) ) ;
#50023=CARTESIAN_POINT ( 'NONE',  ( 84.14312167556933275, 48.98415679381830756, 0.000000000000000000 ) ) ;
#50026=CARTESIAN_POINT ( 'NONE',  ( 72.34554419998197261, 71.56729737182827478, 5.072265668445069764 ) ) ;
#50027=CIRCLE ( 'NONE', #6354, 0.5000000000000004441 ) ;
#50030=CARTESIAN_POINT ( 'NONE',  ( 19.72404941274043466, 33.16126292948895582, -6.180339887498951690 ) ) ;
#50031=VERTEX_POINT ( 'NONE', #6880 ) ;
#50037=CARTESIAN_POINT ( 'NONE',  ( 72.68453300703816922, 57.05733065325770781, -16.38297471568555252 ) ) ;
#50039=CARTESIAN_POINT ( 'NONE',  ( 77.25136647710282034, 63.46566284268146063, -15.11586214491885194 ) ) ;
#50047=CARTESIAN_POINT ( 'NONE',  ( 28.52453836335597614, 34.65586893147758474, -7.433330006724137462 ) ) ;
#50072=ADVANCED_FACE ( 'NONE', ( #37770 ), #29201, .T. ) ;
#50075=VERTEX_POINT ( 'NONE', #37281 ) ;
#50084=CARTESIAN_POINT ( 'NONE',  ( 70.68033699063239794, 69.39733653096790533, -7.416591401506187786 ) ) ;
#50086=CARTESIAN_POINT ( 'NONE',  ( 69.76031522910172100, 62.75377154243565059, -13.30659298224870746 ) ) ;
#50089=CIRCLE ( 'NONE', #84125, 10.00000000000000711 ) ;
#50099=VECTOR ( 'NONE', #564, 1000.000000000000000 ) ;
#50101=CARTESIAN_POINT ( 'NONE',  ( 68.62498439451977106, 69.99363476994645339, -2.580443242845753549 ) ) ;
#50103=CARTESIAN_POINT ( 'NONE',  ( 83.15922154792146159, 52.24841325804966630, 14.83149234656706561 ) ) ;
#50108=CARTESIAN_POINT ( 'NONE',  ( 71.65393590783921240, 64.63887889010254639, -12.86708473997534341 ) ) ;
#50109=CARTESIAN_POINT ( 'NONE',  ( 74.31667694623762088, 55.31426079121899164, 16.60244124719878300 ) ) ;
#50112=CARTESIAN_POINT ( 'NONE',  ( 33.59574554791263523, 38.13478043621391578, 8.090169943749478065 ) ) ;
#50113=CARTESIAN_POINT ( 'NONE',  ( 78.54208217020030247, 47.90658315326027861, 13.93004184109306287 ) ) ;
#50116=CARTESIAN_POINT ( 'NONE',  ( 85.67990461644461675, 43.48540777662389445, -4.634265786033663126 ) ) ;
#50120=ORIENTED_EDGE ( 'NONE', *, *, #55892, .F. ) ;
#50121=CARTESIAN_POINT ( 'NONE',  ( 87.13039101863441260, 46.06611145402069241, 8.900391155234917306 ) ) ;
#50122=CARTESIAN_POINT ( 'NONE',  ( 21.90410768801267949, 17.81029122506294726, 8.090169943749479842 ) ) ;
#50124=CARTESIAN_POINT ( 'NONE',  ( 71.89122079532039322, 72.62093029633255981, -0.6100853850958146696 ) ) ;
#50126=ADVANCED_FACE ( 'NONE', ( #25970 ), #16477, .T. ) ;
#50127=CARTESIAN_POINT ( 'NONE',  ( 87.04534585051717954, 46.05262481000475105, 8.948764308993935046 ) ) ;
#50129=CARTESIAN_POINT ( 'NONE',  ( 29.27874087092374111, 39.83705186507756224, 3.090169943749475401 ) ) ;
#50133=CARTESIAN_POINT ( 'NONE',  ( 72.54776654123371316, 67.64497073380857728, -10.93401973738937549 ) ) ;
#50151=CARTESIAN_POINT ( 'NONE',  ( 31.23567208480136514, 20.96004757982091604, -5.678558825948276656 ) ) ;
#50153=CARTESIAN_POINT ( 'NONE',  ( 86.52156533961138507, 47.40180082335727718, -10.32616759113387062 ) ) ;
#50156=CARTESIAN_POINT ( 'NONE',  ( 13.89352694080530348, 28.99752408145591076, 5.678558825948276656 ) ) ;
#50161=CARTESIAN_POINT ( 'NONE',  ( 72.01497877597556396, 71.50364303677275757, -5.786257741033058011 ) ) ;
#50172=CARTESIAN_POINT ( 'NONE',  ( 65.83577767310526951, 68.92730293486754078, -2.453578508652157097 ) ) ;
#50174=CARTESIAN_POINT ( 'NONE',  ( 72.59642922388725594, 57.37503576641776704, -16.32655392149956342 ) ) ;
#50175=CARTESIAN_POINT ( 'NONE',  ( 77.94354854059760385, 61.39700473696555605, -16.15480247637162847 ) ) ;
#50181=EDGE_LOOP ( 'NONE', ( #5300, #94428, #45319, #81732 ) ) ;
#50182=CARTESIAN_POINT ( 'NONE',  ( 38.36533659613348846, 24.01110640527295104, 2.839279412974134775 ) ) ;
#50193=CARTESIAN_POINT ( 'NONE',  ( 86.54292033101232562, 46.25028892199808439, 8.970843135639702481 ) ) ;
#50197=CARTESIAN_POINT ( 'NONE',  ( 69.97979529158072864, 69.74216827977384980, -5.914717412081216708 ) ) ;
#50208=VERTEX_POINT ( 'NONE', #93519 ) ;
#50209=CARTESIAN_POINT ( 'NONE',  ( 81.83453868260083652, 44.26299598697195847, -9.678769061459140843 ) ) ;
#50210=CARTESIAN_POINT ( 'NONE',  ( 82.70413545112889153, 41.12970673414849188, 1.275000209075848101 ) ) ;
#50213=CARTESIAN_POINT ( 'NONE',  ( 74.50257599732556457, 59.70488952813933281, 15.64583394787582726 ) ) ;
#50216=CARTESIAN_POINT ( 'NONE',  ( 80.49253188860416230, 57.12688299469299125, -16.22935582423522405 ) ) ;
#50222=CARTESIAN_POINT ( 'NONE',  ( 67.66865572057727718, 68.40145999173375913, 5.820033390399663276 ) ) ;
#50225=CARTESIAN_POINT ( 'NONE',  ( 22.16837966976980567, 14.92755873383626053, 6.180339887498953466 ) ) ;
#50233=CARTESIAN_POINT ( 'NONE',  ( 16.01096549046674511, 31.01751292744055988, 6.180339887498949913 ) ) ;
#50240=CARTESIAN_POINT ( 'NONE',  ( 85.86628601408199302, 44.95660682449336321, 8.361449031888060546 ) ) ;
#50241=CARTESIAN_POINT ( 'NONE',  ( 21.39005255714673126, 24.30066082961421969, -10.00000000000000533 ) ) ;
#50242=CARTESIAN_POINT ( 'NONE',  ( 88.21238909966383801, 43.70556102481675964, 0.1923655077720387852 ) ) ;
#50246=CARTESIAN_POINT ( 'NONE',  ( 73.94386985606865892, 54.90338819443267226, -16.13259590105355912 ) ) ;
#50249=CARTESIAN_POINT ( 'NONE',  ( 76.65070268594573122, 58.80663122369263363, 16.45680034700567163 ) ) ;
#50250=CARTESIAN_POINT ( 'NONE',  ( 32.29641253342593643, 23.81029122506296503, 8.090169943749479842 ) ) ;
#50257=CARTESIAN_POINT ( 'NONE',  ( 35.55378427144160014, 29.03085787977765264, 9.188101187500006262 ) ) ;
#50258=EDGE_CURVE ( 'NONE', #12902, #48310, #96969, .T. ) ;
#50260=CARTESIAN_POINT ( 'NONE',  ( 37.50591675755416077, 22.44966523072497111, -2.296566073217252530E-15 ) ) ;
#50266=CARTESIAN_POINT ( 'NONE',  ( 13.56875384759882763, 10.76004757982087767, 5.678558825948272215 ) ) ;
#50267=CARTESIAN_POINT ( 'NONE',  ( 71.83275678050462432, 72.56239119006677640, 1.040614184235684636 ) ) ;
#50268=CARTESIAN_POINT ( 'NONE',  ( 11.52878981408637848, 24.84336893147754921, -7.433330006724137462 ) ) ;
#50273=CARTESIAN_POINT ( 'NONE',  ( 75.08378362262867256, 53.60473078829387106, -16.54206508529750508 ) ) ;
#50275=ORIENTED_EDGE ( 'NONE', *, *, #21817, .F. ) ;
#50279=CARTESIAN_POINT ( 'NONE',  ( 66.72318566906618287, 68.35417501291662745, 4.516870767104322226 ) ) ;
#50280=CARTESIAN_POINT ( 'NONE',  ( 87.36072329576109041, 44.92403384853250259, 6.858028155142555704 ) ) ;
#50286=ORIENTED_EDGE ( 'NONE', *, *, #66944, .F. ) ;
#50287=CARTESIAN_POINT ( 'NONE',  ( 77.57840026120739196, 56.51549017185177348, 16.17678933532221563 ) ) ;
#50289=ORIENTED_EDGE ( 'NONE', *, *, #18310, .T. ) ;
#50290=CARTESIAN_POINT ( 'NONE',  ( 78.08206365161463225, 61.83366292688850763, -15.70979438352861735 ) ) ;
#50291=CARTESIAN_POINT ( 'NONE',  ( 82.46595807734689743, 49.18434068982010388, -13.48834215029216033 ) ) ;
#50297=ORIENTED_EDGE ( 'NONE', *, *, #4205, .T. ) ;
#50302=VERTEX_POINT ( 'NONE', #34547 ) ;
#50309=CARTESIAN_POINT ( 'NONE',  ( 82.92115063973837152, 53.64018987990930043, 15.71948723892795385 ) ) ;
#50312=CARTESIAN_POINT ( 'NONE',  ( 86.87294856589132053, 43.40665088353684808, 1.105523696438083459 ) ) ;
#50318=CARTESIAN_POINT ( 'NONE',  ( 24.12344523961532161, 25.87878583063842086, -9.188101187500006262 ) ) ;
#50321=CARTESIAN_POINT ( 'NONE',  ( 82.63281508726200286, 40.94328431233920895, -3.617117793111280122 ) ) ;
#50330=CARTESIAN_POINT ( 'NONE',  ( 81.29539683296886210, 43.25976067974499273, 9.624898955577574355 ) ) ;
#50331=ORIENTED_EDGE ( 'NONE', *, *, #37082, .F. ) ;
#50339=CARTESIAN_POINT ( 'NONE',  ( 82.79070683882470405, 40.63681047240066846, -1.342339673626402385 ) ) ;
#50341=CARTESIAN_POINT ( 'NONE',  ( 84.78301923744977842, 50.41116426179083021, 13.48115605303108744 ) ) ;
#50345=VERTEX_POINT ( 'NONE', #47 ) ;
#50346=ORIENTED_EDGE ( 'NONE', *, *, #15902, .T. ) ;
#50347=CARTESIAN_POINT ( 'NONE',  ( 74.04232911944542650, 68.62205345152153768, 11.42009053252770912 ) ) ;
#50352=CARTESIAN_POINT ( 'NONE',  ( 88.22000632671871756, 44.27423112938743088, 4.003506518527984781 ) ) ;
#50354=CARTESIAN_POINT ( 'NONE',  ( 73.84430631328980610, 68.30184443197676103, -11.60545323109705507 ) ) ;
#50363=CARTESIAN_POINT ( 'NONE',  ( 68.75905127766452551, 64.69927639754664028, -12.16833701327061945 ) ) ;
#50365=CARTESIAN_POINT ( 'NONE',  ( 81.17232691891706509, 55.55242957854174080, 16.36487835605630536 ) ) ;
#50373=AXIS2_PLACEMENT_3D ( 'NONE', #21978, #92905, #44764 ) ;
#50376=DIRECTION ( 'NONE',  ( 0.3473291852294957405, -0.6015917957689906892, 0.7193398003386545225 ) ) ;
#50378=CARTESIAN_POINT ( 'NONE',  ( 22.90017757337614768, 16.14754757982090183, -5.678558825948276656 ) ) ;
#50379=CARTESIAN_POINT ( 'NONE',  ( 74.86935717915280009, 67.14205582119099347, 12.97785457704837953 ) ) ;
#50384=CARTESIAN_POINT ( 'NONE',  ( 13.94779419600527959, 26.79103043416548147, 8.090169943749478065 ) ) ;
#50390=CARTESIAN_POINT ( 'NONE',  ( 81.42010827217174551, 55.18017053111339010, -15.93332911233570215 ) ) ;
#50392=CARTESIAN_POINT ( 'NONE',  ( 68.79154833403119085, 66.56514279001069667, 9.697512220263618588 ) ) ;
#50396=CARTESIAN_POINT ( 'NONE',  ( 84.81378781617564755, 44.04893954711137383, 6.950746278775451259 ) ) ;
#50397=CARTESIAN_POINT ( 'NONE',  ( 80.33815187331018137, 55.67465446643217319, 16.05710040854216203 ) ) ;
#50399=CARTESIAN_POINT ( 'NONE',  ( 72.29604205201167133, 71.64671137691723857, -5.830803549263603891 ) ) ;
#50402=CARTESIAN_POINT ( 'NONE',  ( 6.396987757676564357, 15.64441083166258295, -10.00000000000000533 ) ) ;
#50414=CARTESIAN_POINT ( 'NONE',  ( 76.65771178043479495, 52.44190810767315725, -15.81497611108756729 ) ) ;
#50423=ORIENTED_EDGE ( 'NONE', *, *, #79298, .F. ) ;
#50429=CARTESIAN_POINT ( 'NONE',  ( 81.91079631343028211, 41.10426679011759887, 3.683705643908186111 ) ) ;
#50430=DIRECTION ( 'NONE',  ( 0.000000000000000000, -0.7457702847286276082, -0.6662031840330557841 ) ) ;
#50438=CARTESIAN_POINT ( 'NONE',  ( 6.089662503932698812, 18.91421378149916421, 9.188101187500008038 ) ) ;
#50439=ORIENTED_EDGE ( 'NONE', *, *, #36678, .F. ) ;
#50455=CARTESIAN_POINT ( 'NONE',  ( 77.82117886139609197, 61.13554303172738003, -15.83944663029401134 ) ) ;
#50456=ORIENTED_EDGE ( 'NONE', *, *, #29825, .F. ) ;
#50460=CARTESIAN_POINT ( 'NONE',  ( 30.01653393904200584, 17.73415679381823296, -6.890680421881970419E-14 ) ) ;
#50462=LINE ( 'NONE', #66171, #1520 ) ;
#50463=CARTESIAN_POINT ( 'NONE',  ( 87.90044328681766217, 44.19652605784722965, 2.801406232019506337 ) ) ;
#50466=CARTESIAN_POINT ( 'NONE',  ( 78.48493553110232313, 60.21799449290400474, -16.03803239114666113 ) ) ;
#50471=CARTESIAN_POINT ( 'NONE',  ( 81.01849461552974674, 43.39542731648039364, -9.975009594712970440 ) ) ;
#50476=FACE_OUTER_BOUND ( 'NONE', #88643, .T. ) ;
#50483=CARTESIAN_POINT ( 'NONE',  ( 84.90983652888880329, 50.15852115595398431, 13.71398460619150406 ) ) ;
#50497=CARTESIAN_POINT ( 'NONE',  ( 38.86330120330953974, 24.29860640527295246, -2.839279412974138328 ) ) ;
#50498=CARTESIAN_POINT ( 'NONE',  ( 80.71202285803703091, 44.87545462257573803, 11.64689240967433292 ) ) ;
#50499=CARTESIAN_POINT ( 'NONE',  ( 75.85623159827970596, 62.55299574685686537, 15.52670894256219469 ) ) ;
#50501=CARTESIAN_POINT ( 'NONE',  ( 20.98410315089673261, 24.06628583063841376, -9.188101187500006262 ) ) ;
#50506=EDGE_CURVE ( 'NONE', #79874, #92910, #55610, .T. ) ;
#50508=EDGE_CURVE ( 'NONE', #77062, #89714, #32664, .T. ) ;
#50514=CARTESIAN_POINT ( 'NONE',  ( 75.21686481362549159, 53.08771132160212858, 16.48832112884387868 ) ) ;
#50515=VERTEX_POINT ( 'NONE', #91702 ) ;
#50519=CARTESIAN_POINT ( 'NONE',  ( 83.50485132091074547, 41.54316576433266306, 0.9957241127150030513 ) ) ;
#50527=CARTESIAN_POINT ( 'NONE',  ( 88.14071703455390150, 44.55363679567808788, -5.002659464432031911 ) ) ;
#50529=CARTESIAN_POINT ( 'NONE',  ( 30.77620441319551503, 35.95586893147757479, 7.433330006724141015 ) ) ;
#50534=VERTEX_POINT ( 'NONE', #7559 ) ;
#50535=CARTESIAN_POINT ( 'NONE',  ( 81.17885442797722817, 42.40402381128041043, 7.623678581642264973 ) ) ;
#50539=CARTESIAN_POINT ( 'NONE',  ( 85.67419379123523981, 48.38599046538906379, -11.71860351056688820 ) ) ;
#50551=EDGE_LOOP ( 'NONE', ( #82964, #66507, #54880, #40296 ) ) ;
#50553=VERTEX_POINT ( 'NONE', #62243 ) ;
#50563=ORIENTED_EDGE ( 'NONE', *, *, #66813, .F. ) ;
#50578=CARTESIAN_POINT ( 'NONE',  ( 82.73648154191296555, 53.32161198284063630, 15.27338507632241793 ) ) ;
#50585=CARTESIAN_POINT ( 'NONE',  ( 79.74169968745719927, 49.12834186041503415, 14.22482900215453760 ) ) ;
#50593=CARTESIAN_POINT ( 'NONE',  ( 70.54855537558694323, 70.85739277034529948, -3.923908426818032424 ) ) ;
#50596=CARTESIAN_POINT ( 'NONE',  ( 15.24017643949430401, 10.92755873383624632, 6.180339887498953466 ) ) ;
#50597=CARTESIAN_POINT ( 'NONE',  ( 41.80956963312145547, 25.10801979619932567, 3.090169943749476733 ) ) ;
#50601=CARTESIAN_POINT ( 'NONE',  ( 80.78918961562681034, 43.20779693872438543, -9.098606657379765039 ) ) ;
#50603=CARTESIAN_POINT ( 'NONE',  ( 67.36468726135395002, 67.68509535240536934, 7.969348504922436405 ) ) ;
#50605=CARTESIAN_POINT ( 'NONE',  ( 87.08280028807568840, 46.42470512669584082, 8.779466583191080531 ) ) ;
#50606=CARTESIAN_POINT ( 'NONE',  ( 39.83529790697233608, 25.12755873383629179, -6.180339887498949025 ) ) ;
#50609=CARTESIAN_POINT ( 'NONE',  ( 87.37996854902368682, 45.84054858551529321, 8.374939902689632731 ) ) ;
#50611=CARTESIAN_POINT ( 'NONE',  ( 32.48073783699224748, 37.49103043416551628, -8.090169943749479842 ) ) ;
#50615=CARTESIAN_POINT ( 'NONE',  ( 67.32446469936046185, 67.76807788068994398, -6.698702025512672797 ) ) ;
#50622=CARTESIAN_POINT ( 'NONE',  ( 87.60525524337998604, 45.45034058462092474, -6.736065127946986308 ) ) ;
#50624=CARTESIAN_POINT ( 'NONE',  ( 74.83655476910678317, 53.51806293180211327, 16.54630480343736210 ) ) ;
#50625=CARTESIAN_POINT ( 'NONE',  ( 74.14312167556930433, 66.30466486950707861, 1.224646799147354045E-15 ) ) ;
#50631=CARTESIAN_POINT ( 'NONE',  ( 67.07163056930700407, 67.06484247801786580, -8.621218654996820163 ) ) ;
#50637=CARTESIAN_POINT ( 'NONE',  ( 34.79119414172389213, 25.80170272979928470, 7.433330006724137462 ) ) ;
#50642=CARTESIAN_POINT ( 'NONE',  ( 19.11131643181922968, 13.96004757982089473, -5.678558825948275768 ) ) ;
#50643=CARTESIAN_POINT ( 'NONE',  ( 68.42755367300264879, 64.43063514657779933, 12.23043961556458470 ) ) ;
#50657=CARTESIAN_POINT ( 'NONE',  ( 65.90562114866830257, 69.02037705693993530, -2.125153001406280939 ) ) ;
#50660=CARTESIAN_POINT ( 'NONE',  ( 78.38505820428797222, 61.21347221756810342, -15.89202726422457879 ) ) ;
#50667=ORIENTED_EDGE ( 'NONE', *, *, #86010, .F. ) ;
#50668=CARTESIAN_POINT ( 'NONE',  ( 38.77491099913230954, 28.10170272979929962, -7.433330006724141015 ) ) ;
#50677=CARTESIAN_POINT ( 'NONE',  ( 77.38135075303371480, 62.12945940828362268, -15.52596300841300092 ) ) ;
#50679=CARTESIAN_POINT ( 'NONE',  ( 74.81832046901196520, 67.48663194201290594, -12.71244991431774984 ) ) ;
#50683=DIRECTION ( 'NONE',  ( 0.4330127018922168558, -0.7499999999999987788, 0.5000000000000039968 ) ) ;
#50689=VECTOR ( 'NONE', #300, 1000.000000000000000 ) ;
#50694=ORIENTED_EDGE ( 'NONE', *, *, #69031, .F. ) ;
#50695=CARTESIAN_POINT ( 'NONE',  ( 82.42287977205688776, 44.22628728383867980, -9.237571607454468037 ) ) ;
#50696=CARTESIAN_POINT ( 'NONE',  ( 83.27976113774722933, 41.54303965256077902, 2.024835421397801039 ) ) ;
#50699=CARTESIAN_POINT ( 'NONE',  ( 79.19548930461120051, 59.90515312544787463, -16.13566294680263624 ) ) ;
#50700=CARTESIAN_POINT ( 'NONE',  ( 74.19664195402195617, 58.24996677738988637, 15.87843237399661334 ) ) ;
#50705=CARTESIAN_POINT ( 'NONE',  ( 72.62263890461544236, 71.39809534012815107, -5.857653296095948647 ) ) ;
#50711=CARTESIAN_POINT ( 'NONE',  ( 69.84362963217853348, 70.73783495060057191, 2.524573071926013768 ) ) ;
#50712=B_SPLINE_CURVE_WITH_KNOTS ( 'NONE', 3,
 ( #53206, #1009, #84159, #83654 ),
 .UNSPECIFIED., .F., .F.,
 ( 4, 4 ),
 ( 0.000000000000000000, 0.3032312338214309122 ),
 .UNSPECIFIED. ) ;
#50715=CARTESIAN_POINT ( 'NONE',  ( 20.43632886220093425, 13.92755873383625698, 6.180339887498953466 ) ) ;
#50729=CARTESIAN_POINT ( 'NONE',  ( 82.89821946049899282, 41.08885103174851849, 3.601454807390346513 ) ) ;
#50730=CARTESIAN_POINT ( 'NONE',  ( 20.69167212271446488, 17.11029122506294087, -8.090169943749478065 ) ) ;
#50731=CARTESIAN_POINT ( 'NONE',  ( 85.29362735876655677, 48.41412782346649379, 12.38048700662148072 ) ) ;
#50733=CARTESIAN_POINT ( 'NONE',  ( 72.04989860578065475, 72.29315785138345518, -3.506402493552649435 ) ) ;
#50735=CARTESIAN_POINT ( 'NONE',  ( 74.23290034432453410, 55.48174697381312370, -16.12021105329591819 ) ) ;
#50738=CARTESIAN_POINT ( 'NONE',  ( 75.26062286730075357, 66.82642578153097190, 12.89509023346212402 ) ) ;
#50741=ADVANCED_FACE ( 'NONE', ( #73379 ), #4977, .T. ) ;
#50750=CARTESIAN_POINT ( 'NONE',  ( 79.04351678514861135, 60.08826646268103389, 16.12134523096112204 ) ) ;
#50751=CARTESIAN_POINT ( 'NONE',  ( 34.12723495145388597, 35.10171378149922106, 9.188101187500008038 ) ) ;
#50755=DIRECTION ( 'NONE',  ( 0.4851478631379963491, -0.8403007481384849875, 0.2419218955996714493 ) ) ;
#50758=CARTESIAN_POINT ( 'NONE',  ( 13.89352694080530171, 28.99752408145591076, 5.678558825948277544 ) ) ;
#50759=CARTESIAN_POINT ( 'NONE',  ( 71.92106615665201730, 72.60175000959985425, 1.189886861346804769 ) ) ;
#50760=CARTESIAN_POINT ( 'NONE',  ( 82.45129306854981621, 53.84777233740990710, 15.85475489262521975 ) ) ;
#50762=AXIS2_PLACEMENT_3D ( 'NONE', #84204, #14750, #86209 ) ;
#50770=CARTESIAN_POINT ( 'NONE',  ( 66.54264984482914258, 68.81226801441182772, 2.258477026830895795 ) ) ;
#50771=CARTESIAN_POINT ( 'NONE',  ( 66.42367604814864990, 68.18713262965796673, 4.499938400593175736 ) ) ;
#50772=CARTESIAN_POINT ( 'NONE',  ( 87.34298713220451305, 45.48433765315401445, 7.112235686424480008 ) ) ;
#50779=EDGE_LOOP ( 'NONE', ( #26028, #80374, #13441, #61453 ) ) ;
#50780=CARTESIAN_POINT ( 'NONE',  ( 80.74781574657599492, 57.21644485803224711, 16.56566952311892749 ) ) ;
#50783=CARTESIAN_POINT ( 'NONE',  ( 87.67818183259522868, 45.22881258881258759, -6.241223674190681692 ) ) ;
#50784=CARTESIAN_POINT ( 'NONE',  ( 80.03738279725816085, 49.90009009011918550, -14.50516081086794706 ) ) ;
#50786=CARTESIAN_POINT ( 'NONE',  ( 81.03246857581767415, 43.63023369003471430, 9.437679533993755143 ) ) ;
#50791=CARTESIAN_POINT ( 'NONE',  ( 73.56986118162708976, 59.18547764286820723, 15.61157655548840495 ) ) ;
#50810=CARTESIAN_POINT ( 'NONE',  ( 71.85869513609316073, 58.67586711399008692, -15.48493562761569287 ) ) ;
#50819=CARTESIAN_POINT ( 'NONE',  ( 82.55707186143240506, 51.89045595487220908, -14.80451076870274107 ) ) ;
#50822=EDGE_CURVE ( 'NONE', #81636, #75751, #27818, .T. ) ;
#50830=EDGE_CURVE ( 'NONE', #56024, #57136, #37583, .T. ) ;
#50833=CARTESIAN_POINT ( 'NONE',  ( 82.80082720015894893, 40.64166234397397659, -1.331724720465388812 ) ) ;
#50835=CARTESIAN_POINT ( 'NONE',  ( 84.35279708572993229, 50.67471669617422236, 13.78338001634371857 ) ) ;
#50839=VERTEX_POINT ( 'NONE', #69984 ) ;
#50842=CARTESIAN_POINT ( 'NONE',  ( 74.27485901263420942, 68.48687493391096837, -11.14965480144356569 ) ) ;
#50843=CARTESIAN_POINT ( 'NONE',  ( 74.34518270076702606, 65.51476795103405948, 13.81701700184060932 ) ) ;
#50859=CARTESIAN_POINT ( 'NONE',  ( 79.48876273271771709, 46.38894273206648222, -12.71961528548989406 ) ) ;
#50861=CARTESIAN_POINT ( 'NONE',  ( 73.31626447649914269, 69.83209129105155455, 9.123803007987715930 ) ) ;
#50865=CARTESIAN_POINT ( 'NONE',  ( 72.51945164430701141, 57.47770362461726279, 16.30230911779761982 ) ) ;
#50873=EDGE_CURVE ( 'NONE', #83096, #49399, #81174, .T. ) ;
#50874=CARTESIAN_POINT ( 'NONE',  ( 31.21402144970675607, 20.94754757982090609, 5.678558825948272215 ) ) ;
#50880=CARTESIAN_POINT ( 'NONE',  ( 68.44064878421174569, 64.54239741235952010, 12.14664289795469543 ) ) ;
#50886=CARTESIAN_POINT ( 'NONE',  ( 81.27316195909862984, 55.43468901134095006, -16.33783760952318431 ) ) ;
#50888=CARTESIAN_POINT ( 'NONE',  ( 68.35453417343931903, 65.67399229982113695, 10.37910612949749911 ) ) ;
#50891=CARTESIAN_POINT ( 'NONE',  ( 83.53995079529126144, 42.42627917222136347, 4.930145434067244814 ) ) ;
#50892=CARTESIAN_POINT ( 'NONE',  ( 79.99648514317578929, 53.62058690794304283, 15.71113301258886530 ) ) ;
#50896=EDGE_LOOP ( 'NONE', ( #79311, #9768, #61364, #29250 ) ) ;
#50898=CARTESIAN_POINT ( 'NONE',  ( 43.97106342183892735, 31.10170272979931028, -7.433330006724141015 ) ) ;
#50903=VERTEX_POINT ( 'NONE', #50193 ) ;
#50904=CARTESIAN_POINT ( 'NONE',  ( 79.11039871569171567, 60.06401293417182075, 16.12737026114500694 ) ) ;
#50906=B_SPLINE_CURVE_WITH_KNOTS ( 'NONE', 3,
 ( #70388, #94725, #997, #9095, #77513, #62779, #7590, #15682, #30893, #93737, #497, #8104, #86651, #70902, #46072, #46575, #31384, #62268, #61781, #38978, #17182, #48084, #86157, #15172, #1509, #93224, #54670, #9614, #32392, #63288, #94231, #55664, #40476, #57676, #12096, #64294, #87167, #87669, #26793, #80538, #10600, #95747, #71908, #33914, #33392, #26300 ),
 .UNSPECIFIED., .F., .F.,
 ( 4, 1, 1, 1, 2, 2, 1, 1, 1, 2, 2, 1, 1, 2, 2, 1, 1, 2, 2, 1, 1, 2, 2, 1, 2, 2, 1, 2, 2, 4 ),
 ( 0.000000000000000000, 0.06249999999998895328, 0.09374999999998358258, 0.1093749999999792943, 0.1171874999999787809, 0.1249999999999782396, 0.1874999999999764910, 0.2187499999999757694, 0.2343749999999754086, 0.2421874999999754086, 0.2499999999999754086, 0.3124999999999897859, 0.3437499999999955036, 0.3593749999999983902, 0.3750000000000012212, 0.4375000000000066613, 0.4687500000000108802, 0.4843750000000129896, 0.5000000000000149880, 0.5625000000000202061, 0.5937500000000215383, 0.6093750000000206501, 0.6250000000000197620, 0.6875000000000135447, 0.7187500000000121014, 0.7500000000000105471, 0.8125000000000075495, 0.8437500000000063283, 0.8750000000000049960, 1.000000000000000000 ),
 .UNSPECIFIED. ) ;
#50908=VERTEX_POINT ( 'NONE', #50679 ) ;
#50913=EDGE_LOOP ( 'NONE', ( #21418, #25166, #88944, #2758 ) ) ;
#50914=EDGE_LOOP ( 'NONE', ( #60354, #94586, #64762, #53151 ) ) ;
#50924=CARTESIAN_POINT ( 'NONE',  ( 82.12375653173634760, 41.12462394345740790, 3.261405856185052521 ) ) ;
#50927=CARTESIAN_POINT ( 'NONE',  ( 82.30224259357629535, 41.51585266698759824, -5.837696018585297963 ) ) ;
#50929=CARTESIAN_POINT ( 'NONE',  ( 29.37675396051999144, 17.36477965099641452, 1.583844403245364907 ) ) ;
#50933=CARTESIAN_POINT ( 'NONE',  ( 76.43229601622785196, 58.36452290443871505, 16.05521737458219533 ) ) ;
#50934=CARTESIAN_POINT ( 'NONE',  ( 7.739928672529463149, 22.65586893147754211, -7.433330006724137462 ) ) ;
#50940=CARTESIAN_POINT ( 'NONE',  ( 78.36279588851795097, 47.41043415324340771, -13.73196331463247688 ) ) ;
#50942=CARTESIAN_POINT ( 'NONE',  ( 70.96429761875693032, 61.15374941679502996, 14.99935025239129871 ) ) ;
#50944=CARTESIAN_POINT ( 'NONE',  ( 70.37934122712871954, 61.23818324669216651, 14.28954007458889386 ) ) ;
#50947=CARTESIAN_POINT ( 'NONE',  ( 88.12308754723774484, 43.81089488678613009, -2.128676964009123651 ) ) ;
#50950=CARTESIAN_POINT ( 'NONE',  ( 66.19182003012738846, 68.79183717905171136, 0.1039918714880866402 ) ) ;
#50951=VERTEX_POINT ( 'NONE', #486 ) ;
#50952=EDGE_CURVE ( 'NONE', #25006, #1813, #24136, .T. ) ;
#50958=CARTESIAN_POINT ( 'NONE',  ( 88.48864216585432985, 44.00423028902886102, 2.007554169862322713 ) ) ;
#50961=ORIENTED_EDGE ( 'NONE', *, *, #72017, .T. ) ;
#50962=CARTESIAN_POINT ( 'NONE',  ( 71.69040520065344424, 62.44079089823191708, -14.09287754070083487 ) ) ;
#50965=CARTESIAN_POINT ( 'NONE',  ( 85.51062282364698319, 48.96702101389664108, -12.23238128493629517 ) ) ;
#50969=CARTESIAN_POINT ( 'NONE',  ( 81.17742577809939064, 43.43109523646555203, -9.910019672670513202 ) ) ;
#50975=CARTESIAN_POINT ( 'NONE',  ( 78.18546057057351106, 52.16385450527234013, 15.57755498089799850 ) ) ;
#50976=DIRECTION ( 'NONE',  ( 0.5000000000000014433, -0.8660254037844378194, 0.000000000000000000 ) ) ;
#50980=CARTESIAN_POINT ( 'NONE',  ( 84.19352825665725959, 50.57172232247530275, 13.77707419306082670 ) ) ;
#50991=CARTESIAN_POINT ( 'NONE',  ( 86.16743810126995129, 43.04331322985106567, -1.056965546583657822 ) ) ;
#50995=CARTESIAN_POINT ( 'NONE',  ( 28.71100085020356474, 39.68290643055189548, 3.479690158560446702E-15 ) ) ;
#50999=CARTESIAN_POINT ( 'NONE',  ( 20.42541317417268942, 33.83396525600390703, -2.839279412974133887 ) ) ;
#51005=VERTEX_POINT ( 'NONE', #11103 ) ;
#51006=CARTESIAN_POINT ( 'NONE',  ( 70.83557099577411975, 60.89137392342752975, 14.54819139492075841 ) ) ;
#51012=CARTESIAN_POINT ( 'NONE',  ( 75.37222269001998143, 53.48600193327490615, 16.03910331961625246 ) ) ;
#51016=ORIENTED_EDGE ( 'NONE', *, *, #92741, .T. ) ;
#51018=CARTESIAN_POINT ( 'NONE',  ( 81.51603451045065185, 42.23037173800174315, -8.032388100303403888 ) ) ;
#51019=CARTESIAN_POINT ( 'NONE',  ( 77.30032487123098406, 63.32994978619627346, -15.17488454575836521 ) ) ;
#51027=CARTESIAN_POINT ( 'NONE',  ( 34.90123498099573851, 22.01110640527294393, 2.839279412974134775 ) ) ;
#51030=CARTESIAN_POINT ( 'NONE',  ( 87.64858773784966672, 45.45714736155468927, 6.714362014711301896 ) ) ;
#51033=CARTESIAN_POINT ( 'NONE',  ( 86.70911053808110580, 46.89117940024963360, 10.21290512048939902 ) ) ;
#51036=CARTESIAN_POINT ( 'NONE',  ( 85.54106661513783649, 48.65811287445264810, 12.45824154186499833 ) ) ;
#51039=CARTESIAN_POINT ( 'NONE',  ( 82.15463706511576447, 40.84277258114416753, 1.595534587534163995 ) ) ;
#51050=CARTESIAN_POINT ( 'NONE',  ( 87.10310940712852812, 46.00011840676027219, -8.174603884307702018 ) ) ;
#51053=CARTESIAN_POINT ( 'NONE',  ( 7.357472841178069878, 27.18080186712591484, 3.090169943749475401 ) ) ;
#51061=CARTESIAN_POINT ( 'NONE',  ( 70.78770575672112386, 64.97714170464311678, 12.24875154412454314 ) ) ;
#51065=CARTESIAN_POINT ( 'NONE',  ( 83.42856800471859913, 47.51705139073896333, 11.98419555216981003 ) ) ;
#51067=CARTESIAN_POINT ( 'NONE',  ( 69.64257305926975050, 62.32707857316431443, -13.51840679933402711 ) ) ;
#51071=CARTESIAN_POINT ( 'NONE',  ( 81.82384807472087118, 49.02608080520630551, 13.57111770008744500 ) ) ;
#51072=CARTESIAN_POINT ( 'NONE',  ( 82.36513698948819240, 40.35680866276053536, -0.9065428034150362357 ) ) ;
#51076=CARTESIAN_POINT ( 'NONE',  ( 76.12676022442599333, 51.56486861732116012, -16.17662836183246711 ) ) ;
#51077=ADVANCED_FACE ( 'NONE', ( #66279 ), #41620, .T. ) ;
#51080=CARTESIAN_POINT ( 'NONE',  ( 79.32243881128263752, 47.71223523376870190, 13.60867400304461050 ) ) ;
#51090=CARTESIAN_POINT ( 'NONE',  ( 29.61202869050421427, 35.83478043621390441, -8.090169943749479842 ) ) ;
#51095=CARTESIAN_POINT ( 'NONE',  ( 83.98302130751108052, 43.28427656522794820, -6.397989684056143211 ) ) ;
#51101=CARTESIAN_POINT ( 'NONE',  ( 87.19358828159984398, 46.06351791880832991, 8.846884648199045742 ) ) ;
#51107=CARTESIAN_POINT ( 'NONE',  ( 86.78549426258130950, 45.83013854792883990, 8.849882187839872572 ) ) ;
#51110=CARTESIAN_POINT ( 'NONE',  ( 42.17466224797323804, 36.30066082961425877, -10.00000000000000533 ) ) ;
#51117=CARTESIAN_POINT ( 'NONE',  ( 68.55506308078156508, 67.87136273880065573, -7.775597205189836991 ) ) ;
#51128=CARTESIAN_POINT ( 'NONE',  ( 11.62691283633230377, 30.21091486745859811, -1.111400068045478839E-16 ) ) ;
#51130=CARTESIAN_POINT ( 'NONE',  ( 67.17471155831628948, 67.15864351149404854, -8.572145057571571414 ) ) ;
#51134=CARTESIAN_POINT ( 'NONE',  ( 78.08206365161463225, 61.83366292688850763, -15.70979438352861735 ) ) ;
#51135=CARTESIAN_POINT ( 'NONE',  ( 28.38624132378439313, 39.49540643055189548, 3.479690158560446702E-15 ) ) ;
#51140=CARTESIAN_POINT ( 'NONE',  ( 11.72364552993787967, 24.95586893147754282, 7.433330006724141015 ) ) ;
#51142=CARTESIAN_POINT ( 'NONE',  ( 70.89819722514211264, 70.25179532443134178, -6.076314343069640245 ) ) ;
#51146=B_SPLINE_CURVE_WITH_KNOTS ( 'NONE', 3,
 ( #66945, #58349, #28448, #28964, #82212, #81702, #66459, #13276, #4667, #76081, #89327, #82709, #97384, #27952, #50750, #43136, #58833, #52731, #83694, #21360, #45142, #89799, #19880, #51244 ),
 .UNSPECIFIED., .F., .F.,
 ( 4, 2, 2, 2, 2, 2, 2, 2, 2, 2, 2, 4 ),
 ( 0.000000000000000000, 0.1249999999999907851, 0.2499999999999815703, 0.3749999999999723554, 0.4374999999999739098, 0.4999999999999754641, 0.5624999999999769074, 0.6249999999999784617, 0.6874999999999799050, 0.7499999999999814593, 0.8749999999999906741, 1.000000000000000000 ),
 .UNSPECIFIED. ) ;
#51149=ORIENTED_EDGE ( 'NONE', *, *, #31981, .T. ) ;
#51155=CARTESIAN_POINT ( 'NONE',  ( 65.93191908977979665, 69.03888066652848465, -2.102623230407007604 ) ) ;
#51158=CARTESIAN_POINT ( 'NONE',  ( 78.26468621063266085, 61.69794584189649811, -15.76854286150912010 ) ) ;
#51162=CARTESIAN_POINT ( 'NONE',  ( 72.21491844529387549, 53.64441083166271085, 0.000000000000000000 ) ) ;
#51168=ORIENTED_EDGE ( 'NONE', *, *, #37013, .T. ) ;
#51172=ORIENTED_EDGE ( 'NONE', *, *, #24311, .T. ) ;
#51177=CARTESIAN_POINT ( 'NONE',  ( 75.74815782865833569, 62.74121906712248631, -15.01347554402796192 ) ) ;
#51183=CARTESIAN_POINT ( 'NONE',  ( 77.35605062658235909, 53.90549147004347930, -16.44166418353362502 ) ) ;
#51190=AXIS2_PLACEMENT_3D ( 'NONE', #35865, #3010, #66766 ) ;
#51192=CARTESIAN_POINT ( 'NONE',  ( 87.11349487006070547, 46.19076519147612458, 8.411924245371466213 ) ) ;
#51200=ORIENTED_EDGE ( 'NONE', *, *, #27516, .T. ) ;
#51201=CARTESIAN_POINT ( 'NONE',  ( 76.71780308168534646, 55.72448719287293528, 16.16777461468364052 ) ) ;
#51203=CARTESIAN_POINT ( 'NONE',  ( 72.57809076984500507, 71.31855580840982611, -5.985130625757507872 ) ) ;
#51207=CARTESIAN_POINT ( 'NONE',  ( 68.30570690293387770, 69.17111502577031956, 4.863477417514607382 ) ) ;
#51208=B_SPLINE_CURVE_WITH_KNOTS ( 'NONE', 3,
 ( #68996, #44694, #61398, #46183, #90871, #68010, #22410 ),
 .UNSPECIFIED., .F., .F.,
 ( 4, 1, 2, 4 ),
 ( 0.000000000000000000, 0.1620005363610098892, 0.2430008045415152085, 0.3240010727220205000 ),
 .UNSPECIFIED. ) ;
#51211=CARTESIAN_POINT ( 'NONE',  ( 10.23294337622180628, 30.00034080476288878, -1.878358725466461243E-16 ) ) ;
#51217=ADVANCED_FACE ( 'NONE', ( #60840 ), #91801, .T. ) ;
#51220=ORIENTED_EDGE ( 'NONE', *, *, #42423, .T. ) ;
#51226=CARTESIAN_POINT ( 'NONE',  ( 85.93706912677129139, 45.09247296462667265, 8.501039739313545951 ) ) ;
#51227=CARTESIAN_POINT ( 'NONE',  ( 25.69932979004302709, 23.03677371833802212, 10.00000000000000533 ) ) ;
#51228=CARTESIAN_POINT ( 'NONE',  ( 85.81856918057869166, 48.58455003273027017, 12.27698013059672455 ) ) ;
#51232=CARTESIAN_POINT ( 'NONE',  ( 74.21788993013733204, 55.48536492223286842, -16.11972369606550259 ) ) ;
#51243=CARTESIAN_POINT ( 'NONE',  ( 72.86910405259972379, 71.04354916989078106, -7.648857478963559942 ) ) ;
#51244=CARTESIAN_POINT ( 'NONE',  ( 78.70150085959764397, 59.83202584994826623, 16.12694553795978081 ) ) ;
#51245=CARTESIAN_POINT ( 'NONE',  ( 31.19238438139944947, 38.98502408145593989, -5.678558825948271327 ) ) ;
#51253=CARTESIAN_POINT ( 'NONE',  ( 11.72364552993787967, 24.95586893147754282, 7.433330006724141015 ) ) ;
#51254=CARTESIAN_POINT ( 'NONE',  ( 71.94719849994383765, 72.57089041204893931, 1.653882010069143815 ) ) ;
#51255=CARTESIAN_POINT ( 'NONE',  ( 82.66013068336778247, 54.08499358714050942, 15.52290316209530019 ) ) ;
#51260=CARTESIAN_POINT ( 'NONE',  ( 85.74058674982732953, 45.55718474559918008, -8.560518791363312729 ) ) ;
#51261=CARTESIAN_POINT ( 'NONE',  ( 27.53097578467762219, 16.86426979415090699, -3.090169943749474069 ) ) ;
#51263=ORIENTED_EDGE ( 'NONE', *, *, #13159, .T. ) ;
#51265=CARTESIAN_POINT ( 'NONE',  ( 67.93373562898584339, 69.81538817605719771, 0.4299488895426710755 ) ) ;
#51273=ORIENTED_EDGE ( 'NONE', *, *, #57176, .F. ) ;
#51275=CARTESIAN_POINT ( 'NONE',  ( 80.48346613340457623, 57.68579040447578166, -16.59506630531065241 ) ) ;
#51277=VERTEX_POINT ( 'NONE', #23347 ) ;
#51278=CARTESIAN_POINT ( 'NONE',  ( 87.69946696010549658, 45.28426313102758627, -6.325214577564480578 ) ) ;
#51279=CARTESIAN_POINT ( 'NONE',  ( 88.50303165573761532, 43.87208881218895584, -0.02088647746843486086 ) ) ;
#51280=CARTESIAN_POINT ( 'NONE',  ( 80.84441418302719740, 43.48202404113703068, 9.388955441769184063 ) ) ;
#51281=ORIENTED_EDGE ( 'NONE', *, *, #74704, .F. ) ;
#51283=CARTESIAN_POINT ( 'NONE',  ( 73.98106629984819449, 60.92745772619367273, 15.22512809013772106 ) ) ;
#51288=CARTESIAN_POINT ( 'NONE',  ( 41.22093855302744458, 25.92755873383628895, 6.180339887498953466 ) ) ;
#51297=CARTESIAN_POINT ( 'NONE',  ( 86.48513059569856409, 43.16329677770136186, 0.5072759017112983271 ) ) ;
#51300=CARTESIAN_POINT ( 'NONE',  ( 76.86804935198983912, 57.06628021550515939, -16.17658353980281305 ) ) ;
#51301=AXIS2_PLACEMENT_3D ( 'NONE', #30026, #60910, #91877 ) ;
#51303=CARTESIAN_POINT ( 'NONE',  ( 77.40115397588131430, 49.73071544000705302, -15.49217368967964426 ) ) ;
#51311=CARTESIAN_POINT ( 'NONE',  ( 71.44228484409906343, 68.27790281458665334, 9.600800115958856296 ) ) ;
#51314=EDGE_CURVE ( 'NONE', #13779, #64640, #17024, .T. ) ;
#51324=EDGE_CURVE ( 'NONE', #24132, #56530, #90079, .T. ) ;
#51334=CARTESIAN_POINT ( 'NONE',  ( 82.16683981089441602, 40.63021946778572868, 3.442904079118366933 ) ) ;
#51335=VERTEX_POINT ( 'NONE', #52037 ) ;
#51339=CARTESIAN_POINT ( 'NONE',  ( 74.44907505376188794, 68.07791596852769089, -11.61944736710526627 ) ) ;
#51342=CARTESIAN_POINT ( 'NONE',  ( 76.59722600259529202, 51.27521344558854111, 16.05611726275148854 ) ) ;
#51343=CARTESIAN_POINT ( 'NONE',  ( 82.01427717811640150, 41.38653749815328098, -5.922201023369847661 ) ) ;
#51345=( BOUNDED_CURVE ( )  B_SPLINE_CURVE ( 2, ( #90668, #7002, #98232, #83051, #21225, #60186, #99224 ),
 .UNSPECIFIED., .F., .T. ) 
 B_SPLINE_CURVE_WITH_KNOTS ( ( 3, 2, 2, 3 ),
 ( 0.9875000000000000444, 0.9899999999999999911, 0.9949999999999999956, 1.000000000000000000 ),
 .UNSPECIFIED. ) 
 CURVE ( )  GEOMETRIC_REPRESENTATION_ITEM ( )  RATIONAL_B_SPLINE_CURVE ( ( 0.9755282581475767101, 0.9755282581475772652, 1.000000000000000000, 0.9510565162951535312, 1.000000000000000000, 0.9510565162951535312, 1.000000000000000000 ) ) 
 REPRESENTATION_ITEM ( '' )  );
#51346=LINE ( 'NONE', #29067, #49842 ) ;
#51351=CARTESIAN_POINT ( 'NONE',  ( 78.96380797632824056, 59.43460744216077529, -16.52597720501995937 ) ) ;
#51356=CARTESIAN_POINT ( 'NONE',  ( 74.14312167556930433, 66.30466486950707861, 1.224646799147354045E-15 ) ) ;
#51357=CARTESIAN_POINT ( 'NONE',  ( 71.63950284402343982, 58.95762851674515304, -15.87121227278351299 ) ) ;
#51358=CARTESIAN_POINT ( 'NONE',  ( 71.94179174019755862, 72.17120852766012717, -1.676876488574577717 ) ) ;
#51362=CARTESIAN_POINT ( 'NONE',  ( 70.33000752277322931, 70.07220943294167625, 5.706326222802051262 ) ) ;
#51363=CARTESIAN_POINT ( 'NONE',  ( 66.11301736082367597, 68.60463451963875059, -4.424701819410488568 ) ) ;
#51364=( BOUNDED_CURVE ( )  B_SPLINE_CURVE ( 2, ( #48347, #80800, #86905, #25548, #11377, #79296, #42227, #9866, #2260, #33142, #56436, #17962, #48858 ),
 .UNSPECIFIED., .F., .T. ) 
 B_SPLINE_CURVE_WITH_KNOTS ( ( 3, 2, 2, 2, 2, 2, 3 ),
 ( 0.08750000000000000833, 0.08999999999999999667, 0.09500000000000000111, 0.1000000000000000056, 0.1049999999999999961, 0.1100000000000000006, 0.1125000000000000028 ),
 .UNSPECIFIED. ) 
 CURVE ( )  GEOMETRIC_REPRESENTATION_ITEM ( )  RATIONAL_B_SPLINE_CURVE ( ( 0.9755282581475768211, 0.9755282581475768211, 1.000000000000000000, 0.9510565162951535312, 1.000000000000000000, 0.9510565162951535312, 1.000000000000000000, 0.9510565162951535312, 1.000000000000000000, 0.9510565162951535312, 1.000000000000000000, 0.9755282581475768211, 0.9755282581475768211 ) ) 
 REPRESENTATION_ITEM ( '' )  );
#51370=CARTESIAN_POINT ( 'NONE',  ( 24.44820476603448611, 26.06628583063842086, -9.188101187500006262 ) ) ;
#51372=CARTESIAN_POINT ( 'NONE',  ( 83.81305692926204642, 51.81190264249386956, -14.87427321595085417 ) ) ;
#51373=CARTESIAN_POINT ( 'NONE',  ( 76.55703705082244426, 63.73850827144991626, 14.88124462962344552 ) ) ;
#51385=ORIENTED_EDGE ( 'NONE', *, *, #91274, .T. ) ;
#51386=CARTESIAN_POINT ( 'NONE',  ( 70.86876320951611774, 70.15810021654870354, 6.178032208043940265 ) ) ;
#51388=CARTESIAN_POINT ( 'NONE',  ( 85.22997224006158490, 42.06997850247606152, -1.831231488640648664 ) ) ;
#51390=CARTESIAN_POINT ( 'NONE',  ( 85.92346940974357494, 46.00060071795214611, 9.032556752206142292 ) ) ;
#51399=CARTESIAN_POINT ( 'NONE',  ( 8.916318567990060728, 28.08080186712591342, -3.090169943749475845 ) ) ;
#51417=CARTESIAN_POINT ( 'NONE',  ( 81.20875893632040743, 42.29378956363321862, -7.416406876933310244 ) ) ;
#51420=CARTESIAN_POINT ( 'NONE',  ( 88.37416949021037738, 43.79857776338975839, 0.1607882160166531627 ) ) ;
#51423=ORIENTED_EDGE ( 'NONE', *, *, #26875, .F. ) ;
#51429=LINE ( 'NONE', #220, #87061 ) ;
#51432=CARTESIAN_POINT ( 'NONE',  ( 72.34345819658318533, 68.24918517509843241, -10.24609853730615328 ) ) ;
#51435=CARTESIAN_POINT ( 'NONE',  ( 77.01662391835196786, 61.79474988883485764, 15.54209892090687362 ) ) ;
#51436=CARTESIAN_POINT ( 'NONE',  ( 14.11662529016922640, 10.01110640527290663, 2.839279412974134775 ) ) ;
#51440=ORIENTED_EDGE ( 'NONE', *, *, #77637, .T. ) ;
#51445=CARTESIAN_POINT ( 'NONE',  ( 82.21190057601546641, 49.98264421458685547, -14.46497528049439474 ) ) ;
#51447=CARTESIAN_POINT ( 'NONE',  ( 84.46833194923661381, 42.11454976261988037, 1.216645073941585720 ) ) ;
#51448=CARTESIAN_POINT ( 'NONE',  ( 88.36865033182888851, 43.96674011622069855, -2.220889795100837283 ) ) ;
#51449=ORIENTED_EDGE ( 'NONE', *, *, #10130, .F. ) ;
#51451=CARTESIAN_POINT ( 'NONE',  ( 76.74769370342797004, 61.59959995924427290, -15.56961045695145351 ) ) ;
#51462=CARTESIAN_POINT ( 'NONE',  ( 88.05378287308985819, 43.82556038557744671, 2.467578420128283767 ) ) ;
#51469=CARTESIAN_POINT ( 'NONE',  ( 85.49318370521093868, 48.99722645306705715, -12.73116331006621493 ) ) ;
#51477=CARTESIAN_POINT ( 'NONE',  ( 79.57426776854913442, 46.24084366570346560, -13.18946159588284139 ) ) ;
#51479=CARTESIAN_POINT ( 'NONE',  ( 77.87326056917984829, 50.90737332642450497, 15.27958365935661611 ) ) ;
#51481=CARTESIAN_POINT ( 'NONE',  ( 80.14583156672975406, 53.55993809145104478, -15.68071144708088660 ) ) ;
#51482=DIRECTION ( 'NONE',  ( 0.5840252505817197237, 0.000000000000000000, -0.8117354905897360418 ) ) ;
#51493=CARTESIAN_POINT ( 'NONE',  ( 4.600586583810874153, 20.84336893147753500, -7.433330006724137462 ) ) ;
#51499=CARTESIAN_POINT ( 'NONE',  ( 75.91719666336339856, 65.48793379249461566, 14.32281418338180856 ) ) ;
#51503=CARTESIAN_POINT ( 'NONE',  ( 40.59535201087842182, 25.29860640527295601, -2.839279412974138328 ) ) ;
#51505=DIRECTION ( 'NONE',  ( 0.000000000000000000, 0.6050222638427527055, 0.7962085532412914723 ) ) ;
#51507=CARTESIAN_POINT ( 'NONE',  ( 23.58217936225004863, 25.56628583063841376, 9.188101187500006262 ) ) ;
#51508=CARTESIAN_POINT ( 'NONE',  ( 6.430760413625676186, 27.21091486745858390, -1.111400068045478839E-16 ) ) ;
#51512=CARTESIAN_POINT ( 'NONE',  ( 70.83041700687917341, 60.97177786998932447, 15.04209849889492823 ) ) ;
#51517=CARTESIAN_POINT ( 'NONE',  ( 87.40678246761487458, 44.84425702272720571, -6.651126967624185760 ) ) ;
#51519=CARTESIAN_POINT ( 'NONE',  ( 70.02414138031360835, 62.78214778883172187, 13.38063900663788885 ) ) ;
#51521=CARTESIAN_POINT ( 'NONE',  ( 86.81641918289878390, 45.77657501471897916, -8.750901752256119437 ) ) ;
#51523=ORIENTED_EDGE ( 'NONE', *, *, #50830, .T. ) ;
#51524=DIRECTION ( 'NONE',  ( 0.3940053768033583426, -0.6824373310787393843, 0.6156614753256619554 ) ) ;
#51525=CARTESIAN_POINT ( 'NONE',  ( 82.97960392506115568, 41.21894294556930305, 0.3178262756287024704 ) ) ;
#51527=EDGE_LOOP ( 'NONE', ( #26171, #67495, #83165, #4794 ) ) ;
#51538=CARTESIAN_POINT ( 'NONE',  ( 33.58239374649102871, 42.49540643055190259, 3.479690158560446702E-15 ) ) ;
#51548=CARTESIAN_POINT ( 'NONE',  ( 85.30407614177579489, 48.45294084599412088, 12.40582119231524949 ) ) ;
#51550=CARTESIAN_POINT ( 'NONE',  ( 72.57276282155493163, 61.54530475149964985, -14.72551858661936031 ) ) ;
#51551=CARTESIAN_POINT ( 'NONE',  ( 82.38478773084463569, 40.37679422933422302, 1.032346012429565807 ) ) ;
#51553=CARTESIAN_POINT ( 'NONE',  ( 76.91165928263828278, 63.32913628365751180, -15.47028109333149715 ) ) ;
#51554=CARTESIAN_POINT ( 'NONE',  ( 78.92848498041493599, 59.73641368792644357, 16.49589861780994227 ) ) ;
#51563=EDGE_CURVE ( 'NONE', #5854, #56559, #63619, .T. ) ;
#51564=CARTESIAN_POINT ( 'NONE',  ( 87.00169912441755571, 45.80253757415765392, -8.636720921146656238 ) ) ;
#51565=EDGE_CURVE ( 'NONE', #64000, #38047, #41303, .T. ) ;
#51566=CARTESIAN_POINT ( 'NONE',  ( 71.41016749218992743, 59.45273978182970609, 15.19346469599747174 ) ) ;
#51570=ORIENTED_EDGE ( 'NONE', *, *, #73902, .T. ) ;
#51573=B_SPLINE_CURVE_WITH_KNOTS ( 'NONE', 3,
 ( #413, #30816, #38397, #62190, #24704, #8517, #31792, #39386, #55096, #40390, #86083, #16605, #39882, #70818, #32307 ),
 .UNSPECIFIED., .F., .F.,
 ( 4, 2, 2, 2, 1, 2, 2, 4 ),
 ( 0.02192660554268253612, 0.1441857798498459853, 0.2664449541570094726, 0.5109633027713375020, 0.6332224770785018775, 0.6943520642320850644, 0.7554816513856682514, 1.000000000000000000 ),
 .UNSPECIFIED. ) ;
#51579=CARTESIAN_POINT ( 'NONE',  ( 84.10316667629699339, 50.25482096114932773, 13.62407874060527213 ) ) ;
#51581=CARTESIAN_POINT ( 'NONE',  ( 69.60117505803954430, 62.41877665539861653, -13.45126974014724475 ) ) ;
#51586=CARTESIAN_POINT ( 'NONE',  ( 82.60448357664856189, 52.47690334010501800, 14.99630412890038933 ) ) ;
#51587=CARTESIAN_POINT ( 'NONE',  ( 82.22603995272856992, 41.23397994388041354, -3.464870737315245641 ) ) ;
#51591=CARTESIAN_POINT ( 'NONE',  ( 71.86232962023154869, 72.24313703945740883, 3.263832247265275210 ) ) ;
#51594=CARTESIAN_POINT ( 'NONE',  ( 80.71439172754905655, 53.75030299096716391, 15.68586089724884047 ) ) ;
#51598=FACE_OUTER_BOUND ( 'NONE', #82244, .T. ) ;
#51599=CARTESIAN_POINT ( 'NONE',  ( 77.69476712368373228, 61.97275371516123244, 15.64124197209477707 ) ) ;
#51602=CARTESIAN_POINT ( 'NONE',  ( 71.47384123275855927, 72.35069954344790233, 1.100233114707630300 ) ) ;
#51603=AXIS2_PLACEMENT_3D ( 'NONE', #95754, #18708, #65782 ) ;
#51607=CARTESIAN_POINT ( 'NONE',  ( 16.16012747849099540, 9.734156793818206310, 1.333680081654574804E-15 ) ) ;
#51611=CARTESIAN_POINT ( 'NONE',  ( 72.12859001842100781, 72.20979474176914437, 3.988024951247655991 ) ) ;
#51614=CARTESIAN_POINT ( 'NONE',  ( 71.01399855574825892, 72.00622678233665397, 1.913033562013090272 ) ) ;
#51620=CARTESIAN_POINT ( 'NONE',  ( 71.66369827319218189, 72.02185750324218816, -1.551229696566575056 ) ) ;
#51623=EDGE_CURVE ( 'NONE', #50345, #12913, #89422, .T. ) ;
#51624=CARTESIAN_POINT ( 'NONE',  ( 87.34667321826604791, 45.97495992385612595, 8.598559468654661586 ) ) ;
#51627=CARTESIAN_POINT ( 'NONE',  ( 6.852252633650415703, 22.14336893147753571, 7.433330006724141015 ) ) ;
#51631=CARTESIAN_POINT ( 'NONE',  ( 73.25272225934853054, 63.87170619894617829, 13.86221949118336916 ) ) ;
#51632=CARTESIAN_POINT ( 'NONE',  ( 73.77985862123976801, 67.40099183159448160, -11.80460429102062925 ) ) ;
#51633=B_SPLINE_SURFACE_WITH_KNOTS ( 'NONE', 3, 1, ( 
 ( #52624, #28851 ),
 ( #53136, #98261 ),
 ( #45524, #76455 ),
 ( #29841, #75973 ),
 ( #68827, #38422 ),
 ( #60215, #84580 ),
 ( #82600, #74962 ),
 ( #13166, #61227 ),
 ( #5545, #92192 ),
 ( #14143, #59730 ),
 ( #36430, #22745 ),
 ( #52132, #53624 ),
 ( #37423, #67337 ),
 ( #21253, #83082 ),
 ( #13652, #15119 ),
 ( #46013, #69337 ),
 ( #76929, #44524 ),
 ( #75455, #68331 ),
 ( #60711, #6040 ),
 ( #100258, #91179 ),
 ( #36936, #61726 ),
 ( #67848, #98769 ),
 ( #83582, #6549 ),
 ( #99256, #45031 ),
 ( #85074, #93170 ),
 ( #63238, #9041 ),
 ( #69831, #10050 ),
 ( #16139, #94180 ),
 ( #17133, #46520 ),
 ( #77457, #47037 ),
 ( #944, #40423 ) ),
 .UNSPECIFIED., .F., .F., .F.,
 ( 4, 3, 3, 3, 3, 3, 3, 3, 3, 3, 4 ),
 ( 2, 2 ),
 ( 0.000000000000000000, 0.1122669598086646486, 0.2243161639709420618, 0.3396355846219054064, 0.4553962076585019170, 0.5677860799922325175, 0.6749047109689453317, 0.7773884377078321695, 0.8775581155834190072, 0.9782364162377876760, 1.000000000000000000 ),
 ( 0.000000000000000000, 1.000000000000000000 ),
 .UNSPECIFIED. ) ;
#51640=B_SPLINE_CURVE_WITH_KNOTS ( 'NONE', 3,
 ( #26142, #94568, #57020, #48436, #18048, #64134, #79384, #72258, #26639, #2350 ),
 .UNSPECIFIED., .F., .F.,
 ( 4, 2, 2, 2, 4 ),
 ( 0.000000000000000000, 0.1244049413672969895, 0.2488098827345939235, 0.3732148241018908852, 0.4976197654691878469 ),
 .UNSPECIFIED. ) ;
#51649=ORIENTED_EDGE ( 'NONE', *, *, #81877, .F. ) ;
#51653=CARTESIAN_POINT ( 'NONE',  ( 25.47001115121704373, 36.74646525600391556, 2.839279412974139660 ) ) ;
#51658=CARTESIAN_POINT ( 'NONE',  ( 19.86428432551159418, 29.65586893147756342, -7.433330006724137462 ) ) ;
#51661=CARTESIAN_POINT ( 'NONE',  ( 16.19390013444010279, 21.30066082961420904, -10.00000000000000533 ) ) ;
#51663=ORIENTED_EDGE ( 'NONE', *, *, #74586, .F. ) ;
#51666=EDGE_CURVE ( 'NONE', #54888, #63156, #76113, .T. ) ;
#51674=VERTEX_POINT ( 'NONE', #38179 ) ;
#51675=CARTESIAN_POINT ( 'NONE',  ( 66.47396703475773450, 68.78583434973192823, -2.171907785482437347 ) ) ;
#51688=ORIENTED_EDGE ( 'NONE', *, *, #12703, .F. ) ;
#51692=CARTESIAN_POINT ( 'NONE',  ( 75.01075065425354182, 66.36200818202817686, -13.12054805335453622 ) ) ;
#51695=CARTESIAN_POINT ( 'NONE',  ( 81.50870630197763944, 56.04945151212235999, 16.05838072277431650 ) ) ;
#51701=CARTESIAN_POINT ( 'NONE',  ( 71.36058271582115253, 63.95108385012159147, -13.16758000239697957 ) ) ;
#51709=EDGE_CURVE ( 'NONE', #19318, #95962, #88169, .T. ) ;
#51720=CARTESIAN_POINT ( 'NONE',  ( 88.05889915941182267, 44.40447472371889148, 4.714184461739164611 ) ) ;
#51721=CARTESIAN_POINT ( 'NONE',  ( 86.87034215171701135, 45.69404419005449824, 7.858360242176417820 ) ) ;
#51723=CARTESIAN_POINT ( 'NONE',  ( 73.04277380876571613, 70.56196896876863889, 7.835544939490339367 ) ) ;
#51730=CARTESIAN_POINT ( 'NONE',  ( 80.49625421685304616, 49.43199229230145875, 14.16045356324821292 ) ) ;
#51731=CARTESIAN_POINT ( 'NONE',  ( 73.71083753633998015, 69.42096255681319406, -9.886876304414311534 ) ) ;
#51735=CARTESIAN_POINT ( 'NONE',  ( 71.64460139743449929, 72.06580075763625359, -0.2659531731967009760 ) ) ;
#51738=CARTESIAN_POINT ( 'NONE',  ( 14.54318666465499632, 27.13478043621387314, 8.090169943749478065 ) ) ;
#51743=CARTESIAN_POINT ( 'NONE',  ( 72.27876543856895353, 72.05160118724565166, -3.335218298938914749 ) ) ;
#51747=VECTOR ( 'NONE', #25133, 1000.000000000000000 ) ;
#51748=CARTESIAN_POINT ( 'NONE',  ( 66.48609986787805326, 67.91412938167108848, -6.639081268635919741 ) ) ;
#51752=CARTESIAN_POINT ( 'NONE',  ( 20.44528175232247591, 34.73705186507753950, -3.090169943749475845 ) ) ;
#51753=CARTESIAN_POINT ( 'NONE',  ( 85.21216800587870921, 49.06579667261281230, 12.45646816431239223 ) ) ;
#51768=CARTESIAN_POINT ( 'NONE',  ( 40.74993669414823927, 32.03085787977766330, 9.188101187500006262 ) ) ;
#51776=CARTESIAN_POINT ( 'NONE',  ( 19.20273687360401027, 16.80170272979925628, 7.433330006724137462 ) ) ;
#51778=CARTESIAN_POINT ( 'NONE',  ( 82.75953659669094975, 53.91263660082293541, 15.45461559304629340 ) ) ;
#51789=CARTESIAN_POINT ( 'NONE',  ( 68.52305094706389355, 70.17018868913098117, -0.3349893018502964059 ) ) ;
#51790=FACE_OUTER_BOUND ( 'NONE', #18823, .T. ) ;
#51799=CARTESIAN_POINT ( 'NONE',  ( 88.07576543976308869, 43.78748546321877910, -2.154750241475199335 ) ) ;
#51800=CARTESIAN_POINT ( 'NONE',  ( 80.44110801039052205, 57.53904330600535388, -16.59063950305211677 ) ) ;
#51804=ORIENTED_EDGE ( 'NONE', *, *, #78524, .T. ) ;
#51806=CARTESIAN_POINT ( 'NONE',  ( 74.78917493913915848, 64.52558641573418186, 14.02150606163593949 ) ) ;
#51812=CARTESIAN_POINT ( 'NONE',  ( 41.80956963312145547, 25.10801979619932567, 3.090169943749476733 ) ) ;
#51814=ORIENTED_EDGE ( 'NONE', *, *, #25001, .T. ) ;
#51816=EDGE_CURVE ( 'NONE', #75490, #45639, #30009, .T. ) ;
#51826=LINE ( 'NONE', #83243, #94981 ) ;
#51830=CARTESIAN_POINT ( 'NONE',  ( 79.98829826350832661, 44.59498145193617802, 11.76229303994366049 ) ) ;
#51833=ORIENTED_EDGE ( 'NONE', *, *, #33898, .F. ) ;
#51835=CARTESIAN_POINT ( 'NONE',  ( 78.86497519275886248, 53.26976081405998542, -15.76972371277651064 ) ) ;
#51838=CARTESIAN_POINT ( 'NONE',  ( 79.43760634492710437, 46.26763820643595437, 12.65635740753111449 ) ) ;
#51859=CARTESIAN_POINT ( 'NONE',  ( 82.10527917775937112, 41.44314374168844495, -5.931418479470229599 ) ) ;
#51865=ORIENTED_EDGE ( 'NONE', *, *, #55148, .F. ) ;
#51872=FACE_OUTER_BOUND ( 'NONE', #58180, .T. ) ;
#51874=CARTESIAN_POINT ( 'NONE',  ( 71.63738353716577478, 58.87189805328393533, -15.39703515908747811 ) ) ;
#51885=CARTESIAN_POINT ( 'NONE',  ( 29.48197064213787044, 19.94754757982090609, 5.678558825948272215 ) ) ;
#51887=DIRECTION ( 'NONE',  ( -0.3940053768033626169, 0.6824373310787468228, 0.6156614753256509642 ) ) ;
#51889=CARTESIAN_POINT ( 'NONE',  ( 81.67891891309422192, 41.47871809714329316, -5.216020542643499347 ) ) ;
#51891=CARTESIAN_POINT ( 'NONE',  ( 68.54052320776597185, 64.24254624729013585, 11.78809861305686901 ) ) ;
#51897=CARTESIAN_POINT ( 'NONE',  ( 2.730238736670421940, 24.68290643055184930, 3.479690158560446702E-15 ) ) ;
#51901=EDGE_CURVE ( 'NONE', #42456, #52395, #48675, .T. ) ;
#51911=CARTESIAN_POINT ( 'NONE',  ( 12.48001537019352192, 22.90829794293879473, 10.00000000000000355 ) ) ;
#51921=CARTESIAN_POINT ( 'NONE',  ( 74.71494119846802562, 53.60965191683258269, 16.08410365026011846 ) ) ;
#51928=ORIENTED_EDGE ( 'NONE', *, *, #6611, .T. ) ;
#51931=CARTESIAN_POINT ( 'NONE',  ( 82.05352392983871823, 53.80490633333712225, 15.54385313613422426 ) ) ;
#51940=CARTESIAN_POINT ( 'NONE',  ( 29.42114147039228200, 17.39040679176983772, 1.333680081654574804E-15 ) ) ;
#51943=CARTESIAN_POINT ( 'NONE',  ( 76.51060883434578841, 58.77893196432874134, 16.01845725252526265 ) ) ;
#51944=CARTESIAN_POINT ( 'NONE',  ( 12.93244592517074487, 8.262165230724926701, -2.296566073217252530E-15 ) ) ;
#51954=CARTESIAN_POINT ( 'NONE',  ( 86.99204085828590394, 44.40222714392293568, 5.125783883892307990 ) ) ;
#51956=( BOUNDED_CURVE ( )  B_SPLINE_CURVE ( 2, ( #77999, #8592, #62260, #1, #80410, #93216, #39456, #92721, #88027, #70381, #61773, #62770, #93729 ),
 .UNSPECIFIED., .F., .T. ) 
 B_SPLINE_CURVE_WITH_KNOTS ( ( 3, 2, 2, 2, 2, 2, 3 ),
 ( 0.3375000000000000222, 0.3400000000000000244, 0.3449999999999999734, 0.3499999999999999778, 0.3549999999999999822, 0.3599999999999999867, 0.3624999999999999889 ),
 .UNSPECIFIED. ) 
 CURVE ( )  GEOMETRIC_REPRESENTATION_ITEM ( )  RATIONAL_B_SPLINE_CURVE ( ( 0.9755282581475768211, 0.9755282581475768211, 1.000000000000000000, 0.9510565162951535312, 1.000000000000000000, 0.9510565162951535312, 1.000000000000000000, 0.9510565162951535312, 1.000000000000000000, 0.9510565162951535312, 1.000000000000000000, 0.9755282581475768211, 0.9755282581475768211 ) ) 
 REPRESENTATION_ITEM ( '' )  );
#51959=CARTESIAN_POINT ( 'NONE',  ( 73.36977505992142312, 62.78772663851135860, -14.42615283414499316 ) ) ;
#51964=CARTESIAN_POINT ( 'NONE',  ( 83.44519214171087640, 44.67505360890212529, -9.064355971954283220 ) ) ;
#51965=EDGE_CURVE ( 'NONE', #24162, #41583, #27404, .T. ) ;
#51968=CARTESIAN_POINT ( 'NONE',  ( 75.99625379708062667, 65.54331796600069993, 13.91730801885865354 ) ) ;
#51973=CYLINDRICAL_SURFACE ( 'NONE', #72342, 10.00000000000001066 ) ;
#51974=CARTESIAN_POINT ( 'NONE',  ( 85.67156739209939076, 48.86885130997027460, -12.09209206581120455 ) ) ;
#51976=CARTESIAN_POINT ( 'NONE',  ( 86.21810832699266314, 43.22812469855217188, 2.504907440873156421 ) ) ;
#51978=CARTESIAN_POINT ( 'NONE',  ( 84.84478398652468911, 48.04838981413973187, 11.80738860868059703 ) ) ;
#51985=CARTESIAN_POINT ( 'NONE',  ( 78.91055811150361876, 55.69949448062589425, 16.11633552490014765 ) ) ;
#51991=CARTESIAN_POINT ( 'NONE',  ( 84.95191157424133621, 50.11551264433204267, 13.67402201518260441 ) ) ;
#51998=CARTESIAN_POINT ( 'NONE',  ( 7.290083236948966317, 25.18502408145589655, 5.678558825948277544 ) ) ;
#51999=CARTESIAN_POINT ( 'NONE',  ( 67.66477494612622934, 65.93994996590180335, 10.43000742999573838 ) ) ;
#52002=CARTESIAN_POINT ( 'NONE',  ( 83.98768872710463995, 42.26923717846278095, -3.638105868026994649 ) ) ;
#52005=CARTESIAN_POINT ( 'NONE',  ( 80.07887604596260189, 44.31141191799963508, 11.46520868211218414 ) ) ;
#52006=CARTESIAN_POINT ( 'NONE',  ( 38.63056705113294953, 37.70171378149921537, -9.188101187500004485 ) ) ;
#52008=FACE_OUTER_BOUND ( 'NONE', #83232, .T. ) ;
#52010=CARTESIAN_POINT ( 'NONE',  ( 20.80007953598619963, 32.98502408145593279, -5.678558825948271327 ) ) ;
#52011=B_SPLINE_CURVE_WITH_KNOTS ( 'NONE', 3,
 ( #83475, #21162, #75866, #67742, #14041, #51030, #5448, #81986, #6445, #97669, #90597, #37324, #28236, #99148, #29735, #60610, #91564, #83981, #59112, #20653, #58623, #43434, #84474, #55016 ),
 .UNSPECIFIED., .F., .F.,
 ( 4, 2, 2, 2, 2, 2, 2, 2, 2, 2, 2, 4 ),
 ( 0.000000000000000000, 0.1250000000000062450, 0.2500000000000124900, 0.3750000000000187628, 0.4375000000000228151, 0.5000000000000268674, 0.5625000000000308642, 0.6250000000000348610, 0.6875000000000388578, 0.7500000000000429656, 0.8750000000000215383, 1.000000000000000000 ),
 .UNSPECIFIED. ) ;
#52025=CARTESIAN_POINT ( 'NONE',  ( 85.18019808382288716, 46.01488486704433001, -10.22134979624012452 ) ) ;
#52028=CARTESIAN_POINT ( 'NONE',  ( 81.41513720620088179, 41.93548059953372587, -7.650316833348846934 ) ) ;
#52030=CARTESIAN_POINT ( 'NONE',  ( 87.65749775821140588, 44.27781399121202810, 3.602933735144415728 ) ) ;
#52034=CARTESIAN_POINT ( 'NONE',  ( 84.64741752562134991, 50.25350151326510684, 13.85721388315136693 ) ) ;
#52037=CARTESIAN_POINT ( 'NONE',  ( 88.33748333995926316, 44.07075497373335793, -2.898134731201833070 ) ) ;
#52038=CARTESIAN_POINT ( 'NONE',  ( 36.24780089259745353, 32.87878583063844218, -9.188101187500006262 ) ) ;
#52039=CARTESIAN_POINT ( 'NONE',  ( 80.35194745355103407, 44.33500143762700674, 11.34211166093983358 ) ) ;
#52040=CARTESIAN_POINT ( 'NONE',  ( 71.50101329703264241, 60.99057979258904538, -14.67061923267852919 ) ) ;
#52052=CARTESIAN_POINT ( 'NONE',  ( 82.45869220239580955, 40.41366995031415144, 0.9483679617909533954 ) ) ;
#52054=CARTESIAN_POINT ( 'NONE',  ( 77.07149570696485341, 63.73492570656748057, -15.36167024187155228 ) ) ;
#52055=CARTESIAN_POINT ( 'NONE',  ( 78.87398835131222086, 59.62348996268822532, 16.50394892759813459 ) ) ;
#52064=CARTESIAN_POINT ( 'NONE',  ( 34.04375301561599798, 21.78380873178788946, -6.180339887498949025 ) ) ;
#52065=CARTESIAN_POINT ( 'NONE',  ( 13.51707852204697069, 30.73705186507753240, -3.090169943749475845 ) ) ;
#52073=CARTESIAN_POINT ( 'NONE',  ( 67.06678242535858203, 68.82311105335894297, -3.689783056880661771 ) ) ;
#52075=CARTESIAN_POINT ( 'NONE',  ( 69.50673298128731403, 63.05023952497469963, -13.62172798439030608 ) ) ;
#52079=CARTESIAN_POINT ( 'NONE',  ( 82.21065643673749435, 50.51336489522484641, 14.24654085560588435 ) ) ;
#52083=EDGE_CURVE ( 'NONE', #40804, #50302, #20476, .T. ) ;
#52086=CARTESIAN_POINT ( 'NONE',  ( 79.69316575823049220, 48.95429064770711847, 14.15326268420492006 ) ) ;
#52087=CARTESIAN_POINT ( 'NONE',  ( 69.54162092933202644, 70.29952225041016334, -3.646433943178841286 ) ) ;
#52092=EDGE_CURVE ( 'NONE', #7443, #47283, #3618, .T. ) ;
#52095=CARTESIAN_POINT ( 'NONE',  ( 73.59487243717410365, 69.71703543845904960, -9.441731441278315984 ) ) ;
#52098=CARTESIAN_POINT ( 'NONE',  ( 40.84394904227130496, 31.78052372038643725, -10.00000000000000355 ) ) ;
#52101=CARTESIAN_POINT ( 'NONE',  ( 72.06396613292808695, 72.31755342346831128, 3.440598478083119804 ) ) ;
#52104=CARTESIAN_POINT ( 'NONE',  ( 81.49351603733306604, 42.61972550722757092, -7.674745181728958698 ) ) ;
#52106=CARTESIAN_POINT ( 'NONE',  ( 72.09026212718839588, 72.27200742537389999, -1.505500128747980337 ) ) ;
#52108=CARTESIAN_POINT ( 'NONE',  ( 28.47099635789628280, 18.29860640527293114, -2.839279412974138328 ) ) ;
#52111=CARTESIAN_POINT ( 'NONE',  ( 12.70933400901951416, 9.198606405272903075, 2.839279412974134775 ) ) ;
#52115=CARTESIAN_POINT ( 'NONE',  ( 72.32152639495393487, 60.34245158586753632, 15.08100388408858272 ) ) ;
#52116=CARTESIAN_POINT ( 'NONE',  ( 74.42984188155799075, 67.24162272381263961, -12.24555194031338701 ) ) ;
#52118=CARTESIAN_POINT ( 'NONE',  ( 74.26842774264412128, 57.07890938945873671, -16.02166782049268789 ) ) ;
#52122=VERTEX_POINT ( 'NONE', #92680 ) ;
#52125=ADVANCED_FACE ( 'NONE', ( #23232 ), #60295, .T. ) ;
#52132=CARTESIAN_POINT ( 'NONE',  ( 79.15299089334158111, 45.92879069919392521, -13.14368370819105714 ) ) ;
#52135=DIRECTION ( 'NONE',  ( 0.4827766168686632997, 0.5834231310750495059, -0.6531035050674843800 ) ) ;
#52139=CARTESIAN_POINT ( 'NONE',  ( 26.24098094315136009, 17.01110640527292972, 2.839279412974134775 ) ) ;
#52140=CARTESIAN_POINT ( 'NONE',  ( 76.51987890029035100, 63.61070592637643983, 14.91914813192731337 ) ) ;
#52141=CARTESIAN_POINT ( 'NONE',  ( 71.31409814852831630, 70.28103913945014369, -6.532773565772590274 ) ) ;
#52142=CARTESIAN_POINT ( 'NONE',  ( 75.31048316780064056, 66.81495650182517920, -12.93102085071238072 ) ) ;
#52147=ORIENTED_EDGE ( 'NONE', *, *, #72532, .F. ) ;
#52148=CARTESIAN_POINT ( 'NONE',  ( 70.34454795188869980, 61.29844696716961749, 14.78467410895967760 ) ) ;
#52151=CARTESIAN_POINT ( 'NONE',  ( 66.12920851151632462, 68.57659062400610139, -2.240737289274019606 ) ) ;
#52156=VECTOR ( 'NONE', #2763, 1000.000000000000000 ) ;
#52166=CARTESIAN_POINT ( 'NONE',  ( 75.32621823817197537, 66.64820785908354139, -13.05086397426676648 ) ) ;
#52169=CARTESIAN_POINT ( 'NONE',  ( 81.68833537920569654, 55.69874641368435420, 15.98167401408987587 ) ) ;
#52171=CARTESIAN_POINT ( 'NONE',  ( 71.16602909547167144, 66.01008435473005420, 11.62282365756693103 ) ) ;
#52173=CARTESIAN_POINT ( 'NONE',  ( 87.43576499144317893, 45.00137247461037049, 6.922634181320210800 ) ) ;
#52174=ORIENTED_EDGE ( 'NONE', *, *, #4780, .T. ) ;
#52179=CARTESIAN_POINT ( 'NONE',  ( 76.13068126100937150, 51.50493480594106899, -15.67342808751774008 ) ) ;
#52182=EDGE_CURVE ( 'NONE', #69479, #65130, #39807, .T. ) ;
#52188=CARTESIAN_POINT ( 'NONE',  ( 86.21660337353470993, 44.60933949929385989, 6.554422449840823006 ) ) ;
#52191=B_SPLINE_CURVE_WITH_KNOTS ( 'NONE', 3,
 ( #39132, #91906, #68060, #22462, #21962, #44746, #52855, #76191, #53357, #14854 ),
 .UNSPECIFIED., .F., .F.,
 ( 4, 2, 2, 2, 4 ),
 ( 0.000000000000000000, 0.2500000000000000000, 0.5000000000000000000, 0.7500000000000000000, 1.000000000000000000 ),
 .UNSPECIFIED. ) ;
#52192=CARTESIAN_POINT ( 'NONE',  ( 72.99805664120070503, 70.78149395872682703, 8.185774945494653565 ) ) ;
#52194=VERTEX_POINT ( 'NONE', #22009 ) ;
#52195=CARTESIAN_POINT ( 'NONE',  ( 76.70704513412616166, 55.66840412848188890, 16.16585368749594664 ) ) ;
#52197=CARTESIAN_POINT ( 'NONE',  ( 72.63019387209214983, 71.43162966861650887, -5.787168193185468823 ) ) ;
#52202=CARTESIAN_POINT ( 'NONE',  ( 70.92638144461730576, 71.59949221093340554, 0.8533387835500414464 ) ) ;
#52207=AXIS2_PLACEMENT_3D ( 'NONE', #36065, #77582, #31950 ) ;
#52210=CARTESIAN_POINT ( 'NONE',  ( 23.91155070014810136, 29.50829794293881392, -10.00000000000000355 ) ) ;
#52214=CARTESIAN_POINT ( 'NONE',  ( 71.04154053766541210, 69.33027533991680968, -8.669517590967728893 ) ) ;
#52216=CARTESIAN_POINT ( 'NONE',  ( 72.05072980389924453, 71.77788221706620675, -3.931438730150958349 ) ) ;
#52220=B_SPLINE_CURVE_WITH_KNOTS ( 'NONE', 3,
 ( #58578, #95149, #10504, #79943, #2419, #34785, #88066, #65201, #89077, #11523 ),
 .UNSPECIFIED., .F., .F.,
 ( 4, 2, 2, 2, 4 ),
 ( 0.000000000000000000, 0.0002622400424272841352, 0.0005244800848545682704, 0.0007867201272818524597, 0.001048960169709136541 ),
 .UNSPECIFIED. ) ;
#52222=CARTESIAN_POINT ( 'NONE',  ( 66.71298768300009385, 67.40120186928047019, -6.723713196347710586 ) ) ;
#52223=CARTESIAN_POINT ( 'NONE',  ( 72.73113476598997806, 70.26322447592292519, -8.050895442633969168 ) ) ;
#52227=CARTESIAN_POINT ( 'NONE',  ( 30.56436172585706146, 22.81029122506296147, 8.090169943749479842 ) ) ;
#52230=LINE ( 'NONE', #6137, #66209 ) ;
#52231=FACE_OUTER_BOUND ( 'NONE', #75829, .T. ) ;
#52241=CARTESIAN_POINT ( 'NONE',  ( 84.55537670905214043, 50.62155581810766591, -14.09136642048689936 ) ) ;
#52246=CARTESIAN_POINT ( 'NONE',  ( 33.90715327291019321, 42.68290643055189548, 3.479690158560446702E-15 ) ) ;
#52249=ADVANCED_FACE ( 'NONE', ( #69914 ), #70424, .T. ) ;
#52253=CARTESIAN_POINT ( 'NONE',  ( 16.17646586176480739, 17.84335787977762067, 9.188101187500006262 ) ) ;
#52255=CARTESIAN_POINT ( 'NONE',  ( 82.61367695794857013, 54.13558619510798309, 15.54525242622692716 ) ) ;
#52256=CARTESIAN_POINT ( 'NONE',  ( 71.39729339694994792, 59.37714758514961488, 15.71381503284779235 ) ) ;
#52261=CARTESIAN_POINT ( 'NONE',  ( 79.96327294300282063, 46.17232751745272168, -12.99524731289856483 ) ) ;
#52263=CARTESIAN_POINT ( 'NONE',  ( 74.99593504773368124, 53.54266265287736815, -16.54118947238006854 ) ) ;
#52264=CARTESIAN_POINT ( 'NONE',  ( 81.43085985942128957, 41.98340591695951218, 7.714366660622415495 ) ) ;
#52266=CARTESIAN_POINT ( 'NONE',  ( 81.99104559367746958, 58.71166190940888185, -0.01744974835124876722 ) ) ;
#52268=CARTESIAN_POINT ( 'NONE',  ( 72.52170310386408403, 57.33936031854678106, 16.32555210529406153 ) ) ;
#52274=ORIENTED_EDGE ( 'NONE', *, *, #64311, .T. ) ;
#52276=CARTESIAN_POINT ( 'NONE',  ( 84.14312167556933275, 48.98415679381830756, 0.000000000000000000 ) ) ;
#52277=CARTESIAN_POINT ( 'NONE',  ( 80.41409615687595647, 57.98253562157035645, -16.60360993379744343 ) ) ;
#52283=CARTESIAN_POINT ( 'NONE',  ( 74.66885986973987599, 63.97112931501096256, 14.24837920079651887 ) ) ;
#52293=ORIENTED_EDGE ( 'NONE', *, *, #44210, .T. ) ;
#52294=CARTESIAN_POINT ( 'NONE',  ( 73.43067314555278813, 69.84183981607019120, 9.192079101480102210 ) ) ;
#52303=AXIS2_PLACEMENT_3D ( 'NONE', #60315, #69432, #13264 ) ;
#52305=CARTESIAN_POINT ( 'NONE',  ( 72.70796915197145438, 58.43460131349139175, -15.66698973594322197 ) ) ;
#52306=CARTESIAN_POINT ( 'NONE',  ( 30.83758659773572575, 40.73705186507756082, -3.090169943749475845 ) ) ;
#52314=CARTESIAN_POINT ( 'NONE',  ( 75.40682597281998767, 54.41795888520695001, -16.12013989205779296 ) ) ;
#52316=CARTESIAN_POINT ( 'NONE',  ( 79.70436563710978817, 46.00489109485927486, 12.97891914157378679 ) ) ;
#52319=VERTEX_POINT ( 'NONE', #13389 ) ;
#52336=CARTESIAN_POINT ( 'NONE',  ( 69.94542627262927681, 71.02953153408785170, -0.005637359706063728958 ) ) ;
#52339=CARTESIAN_POINT ( 'NONE',  ( 81.85412157328340754, 41.19605074857211946, -5.694832249283913406 ) ) ;
#52340=CYLINDRICAL_SURFACE ( 'NONE', #17144, 16.60714546451156792 ) ;
#52342=CARTESIAN_POINT ( 'NONE',  ( 68.48351335520325733, 64.33043610559428771, -12.33486862999595601 ) ) ;
#52350=CARTESIAN_POINT ( 'NONE',  ( 68.72758243515100673, 68.85043676914649780, -7.310471056669800127 ) ) ;
#52352=CARTESIAN_POINT ( 'NONE',  ( 71.90368585207026797, 59.31677128024832513, -15.31322431433719800 ) ) ;
#52357=CARTESIAN_POINT ( 'NONE',  ( 73.13084643241136007, 57.37954916538377148, 15.88987484405033435 ) ) ;
#52358=CARTESIAN_POINT ( 'NONE',  ( 71.07628154480391913, 71.06296950484041020, 4.311319492879813531 ) ) ;
#52359=CARTESIAN_POINT ( 'NONE',  ( 66.13815982364135948, 68.48623413791136727, -4.821830553978275091 ) ) ;
#52367=CARTESIAN_POINT ( 'NONE',  ( 28.47099635789628280, 18.29860640527293114, -2.839279412974138328 ) ) ;
#52369=CARTESIAN_POINT ( 'NONE',  ( 83.82342001511069896, 52.04024975599947567, -14.96847033955516260 ) ) ;
#52373=CARTESIAN_POINT ( 'NONE',  ( 88.13962338646859962, 43.88173199026378057, 2.505344897735778620 ) ) ;
#52376=CARTESIAN_POINT ( 'NONE',  ( 69.03268662160444080, 64.48878135178121340, 12.45710446990803000 ) ) ;
#52380=DIRECTION ( 'NONE',  ( -0.3473291852295006810, 0.6015917957689992379, 0.7193398003386451967 ) ) ;
#52384=CARTESIAN_POINT ( 'NONE',  ( 70.37731676418549398, 69.40210544723913699, 7.051632179388870547 ) ) ;
#52386=ADVANCED_FACE ( 'NONE', ( #13152 ), #65919, .T. ) ;
#52389=DIRECTION ( 'NONE',  ( -0.3473291852295006810, 0.6015917957689992379, 0.7193398003386451967 ) ) ;
#52390=CARTESIAN_POINT ( 'NONE',  ( 68.62404369657433278, 69.88680614121496149, 3.169402490526867844 ) ) ;
#52391=FACE_OUTER_BOUND ( 'NONE', #75244, .T. ) ;
#52393=CARTESIAN_POINT ( 'NONE',  ( 17.56085832715719164, 11.10801979619927948, 3.090169943749476733 ) ) ;
#52394=CARTESIAN_POINT ( 'NONE',  ( 83.73797956718067326, 47.25317760063183670, 12.19094957233783738 ) ) ;
#52395=VERTEX_POINT ( 'NONE', #35819 ) ;
#52396=CARTESIAN_POINT ( 'NONE',  ( 79.14312167556931854, 57.64441083166269664, 0.000000000000000000 ) ) ;
#52397=CARTESIAN_POINT ( 'NONE',  ( 86.35458572345136474, 46.97350791603361131, -10.52386536561717811 ) ) ;
#52398=CARTESIAN_POINT ( 'NONE',  ( 80.47941278984953328, 45.63198079188786238, -11.75349558557117469 ) ) ;
#52403=CARTESIAN_POINT ( 'NONE',  ( 74.81496871025450446, 53.36391971156190550, 16.05853747727076453 ) ) ;
#52407=CARTESIAN_POINT ( 'NONE',  ( 67.34378090123340144, 69.79098680214323736, 2.519322243948931561 ) ) ;
#52408=CARTESIAN_POINT ( 'NONE',  ( 81.62852022226142878, 42.64977674016488152, -7.599251380822039437 ) ) ;
#52415=CARTESIAN_POINT ( 'NONE',  ( 76.20055470335279324, 65.09253202017347917, 14.18943646504600054 ) ) ;
#52418=CARTESIAN_POINT ( 'NONE',  ( 82.66777534764520396, 40.88273136510965600, 3.288167606857240521 ) ) ;
#52420=ADVANCED_FACE ( 'NONE', ( #84455 ), #53054, .T. ) ;
#52422=CARTESIAN_POINT ( 'NONE',  ( 66.75966942117048575, 68.13366762939419630, -5.218020817821980017 ) ) ;
#52426=CARTESIAN_POINT ( 'NONE',  ( 8.697374518098678564, 25.99752408145590366, 5.678558825948277544 ) ) ;
#52434=CARTESIAN_POINT ( 'NONE',  ( 79.79559376127615167, 44.73722406975080190, 11.30977224791904057 ) ) ;
#52441=CARTESIAN_POINT ( 'NONE',  ( 72.49894385216839510, 63.03176572407281952, -14.06401512292728206 ) ) ;
#52458=ADVANCED_FACE ( 'NONE', ( #61843 ), #97524, .T. ) ;
#52463=CARTESIAN_POINT ( 'NONE',  ( 84.20940321838243392, 46.16460512702312258, 10.34873203983212164 ) ) ;
#52469=CARTESIAN_POINT ( 'NONE',  ( 79.07729678290289144, 56.72051478397521862, 16.18859796109226679 ) ) ;
#52472=PLANE ( 'NONE',  #64723 ) ;
#52476=CARTESIAN_POINT ( 'NONE',  ( 84.43483225515912238, 50.68154273191345283, 13.76020688952911364 ) ) ;
#52485=CARTESIAN_POINT ( 'NONE',  ( 68.22205435738101187, 65.90345407221148832, 10.80313017757570826 ) ) ;
#52492=CARTESIAN_POINT ( 'NONE',  ( 40.74993669414823216, 32.03085787977766330, 9.188101187500006262 ) ) ;
#52494=FACE_BOUND ( 'NONE', #25546, .T. ) ;
#52496=CARTESIAN_POINT ( 'NONE',  ( 22.44070990177030112, 31.14336893147756413, 7.433330006724141015 ) ) ;
#52501=CARTESIAN_POINT ( 'NONE',  ( 70.58272931436614783, 60.86286632090516235, 14.50022832024369279 ) ) ;
#52502=CARTESIAN_POINT ( 'NONE',  ( 75.80192922086310148, 65.84738460970490337, -14.09986028324621898 ) ) ;
#52504=CARTESIAN_POINT ( 'NONE',  ( 22.01921768174555893, 36.21091486745860522, -1.111400068045478839E-16 ) ) ;
#52506=CARTESIAN_POINT ( 'NONE',  ( 75.15191903146568109, 52.97183600650499358, -16.48001256439864903 ) ) ;
#52523=CARTESIAN_POINT ( 'NONE',  ( 33.72069078606260462, 37.65586893147758474, -7.433330006724137462 ) ) ;
#52530=CARTESIAN_POINT ( 'NONE',  ( 81.09122451980682911, 42.49663464562407711, 7.855986980898610916 ) ) ;
#52535=CARTESIAN_POINT ( 'NONE',  ( 68.51164798075079432, 68.66491985411187216, 7.416875103192704266 ) ) ;
#52538=CARTESIAN_POINT ( 'NONE',  ( 77.23555989339968164, 62.99091516456967099, -15.27956704681999156 ) ) ;
#52543=CARTESIAN_POINT ( 'NONE',  ( 31.37760429443829224, 33.51421378149921537, -9.188101187500004485 ) ) ;
#52545=ORIENTED_EDGE ( 'NONE', *, *, #87317, .F. ) ;
#52547=CARTESIAN_POINT ( 'NONE',  ( 74.09769653082098273, 68.87686179987508694, -11.21282387169916284 ) ) ;
#52551=CARTESIAN_POINT ( 'NONE',  ( 21.91939736263385541, 14.78380873178786636, -6.180339887498949025 ) ) ;
#52560=CARTESIAN_POINT ( 'NONE',  ( 83.31942950123568892, 47.18081731595467687, 11.75718208460381220 ) ) ;
#52567=CARTESIAN_POINT ( 'NONE',  ( 82.28788541374279930, 41.26664830668678974, -3.453415047302514029 ) ) ;
#52571=CARTESIAN_POINT ( 'NONE',  ( 72.00818181938288376, 72.30390281540809383, 3.363530094501221424 ) ) ;
#52577=CARTESIAN_POINT ( 'NONE',  ( 82.71327011143105779, 53.60354310397067934, -15.74390733313335566 ) ) ;
#52581=CARTESIAN_POINT ( 'NONE',  ( 77.71677981826302073, 61.99014014597172206, 15.64018103715309316 ) ) ;
#52588=CARTESIAN_POINT ( 'NONE',  ( 79.58936028502597537, 59.22294857574253513, 16.56770033466462166 ) ) ;
#52589=CARTESIAN_POINT ( 'NONE',  ( 43.71482552144721723, 26.20801979619932354, -3.090169943749474069 ) ) ;
#52591=CARTESIAN_POINT ( 'NONE',  ( 82.67645095449901760, 54.06173429938865382, 15.51329239322386577 ) ) ;
#52592=CARTESIAN_POINT ( 'NONE',  ( 72.26106983447931498, 71.98033296937877878, 3.564000903169437517 ) ) ;
#52595=CARTESIAN_POINT ( 'NONE',  ( 81.34288284027337568, 42.53142883239708993, -7.672663453570639724 ) ) ;
#52597=CARTESIAN_POINT ( 'NONE',  ( 40.45322629432754269, 23.75978393459168458, -1.583844403245396437 ) ) ;
#52600=CARTESIAN_POINT ( 'NONE',  ( 19.06802872841732110, 31.98502408145592568, -5.678558825948271327 ) ) ;
#52603=CARTESIAN_POINT ( 'NONE',  ( 43.20833262110986084, 30.11029122506297995, -8.090169943749478065 ) ) ;
#52608=CARTESIAN_POINT ( 'NONE',  ( 73.58277243495972186, 65.12260290344103453, 13.28827523339052696 ) ) ;
#52612=CARTESIAN_POINT ( 'NONE',  ( 87.77567103309253582, 45.10408226285451150, -6.743331934586553444 ) ) ;
#52622=ORIENTED_EDGE ( 'NONE', *, *, #64617, .F. ) ;
#52624=CARTESIAN_POINT ( 'NONE',  ( 79.36263291412585374, 45.67866562560195831, -12.88899626214226579 ) ) ;
#52625=LINE ( 'NONE', #59214, #2291 ) ;
#52631=CARTESIAN_POINT ( 'NONE',  ( 16.40018271037384068, 27.65586893147755987, -7.433330006724137462 ) ) ;
#52632=CARTESIAN_POINT ( 'NONE',  ( 75.82607876426669691, 58.94255996486501914, 15.94889058982140995 ) ) ;
#52640=ORIENTED_EDGE ( 'NONE', *, *, #45134, .F. ) ;
#52641=CARTESIAN_POINT ( 'NONE',  ( 72.51499028565849869, 68.19712414860103422, 10.98850085807369048 ) ) ;
#52643=CARTESIAN_POINT ( 'NONE',  ( 68.16895862681424489, 70.45982571230283042, -0.9782046817701681718 ) ) ;
#52646=CARTESIAN_POINT ( 'NONE',  ( 81.43364589948765797, 55.81991725365188017, 16.38199963144059268 ) ) ;
#52655=B_SPLINE_CURVE_WITH_KNOTS ( 'NONE', 3,
 ( #60346, #58370, #14271, #75094, #76101, #98396, #59349, #13771, #27971, #19899 ),
 .UNSPECIFIED., .F., .F.,
 ( 4, 2, 2, 2, 4 ),
 ( 0.000000000000000000, 0.0002622400424272964409, 0.0005244800848545928817, 0.0007867201272818888889, 0.001048960169709184896 ),
 .UNSPECIFIED. ) ;
#52660=EDGE_LOOP ( 'NONE', ( #77090, #4541, #94445, #64234 ) ) ;
#52663=CARTESIAN_POINT ( 'NONE',  ( 67.00504814593276137, 67.59751109484044207, 6.664452144992148774 ) ) ;
#52666=CARTESIAN_POINT ( 'NONE',  ( 81.43364589948765797, 55.81991725365188017, 16.38199963144059268 ) ) ;
#52669=CARTESIAN_POINT ( 'NONE',  ( 87.62362232749241286, 45.09856358269392729, 6.901305344596347702 ) ) ;
#52673=CARTESIAN_POINT ( 'NONE',  ( 76.04118372992293473, 51.31859880959181197, -16.13611964362921114 ) ) ;
#52682=CARTESIAN_POINT ( 'NONE',  ( 87.80215979260032100, 44.26138434534234278, 4.729176973005308149 ) ) ;
#52684=ADVANCED_FACE ( 'NONE', ( #66289 ), #66780, .T. ) ;
#52685=CARTESIAN_POINT ( 'NONE',  ( 87.92881912668997302, 44.04200394344634617, -1.750241744287725609 ) ) ;
#52688=CARTESIAN_POINT ( 'NONE',  ( 73.03196327561725809, 66.92845420574971627, -11.83911326526495067 ) ) ;
#52693=CARTESIAN_POINT ( 'NONE',  ( 80.15658303621371772, 48.28644400875573695, 13.66130757313470312 ) ) ;
#52702=FACE_BOUND ( 'NONE', #1500, .T. ) ;
#52703=CARTESIAN_POINT ( 'NONE',  ( 22.83062064355499032, 21.38052372038641380, 10.00000000000000533 ) ) ;
#52704=CARTESIAN_POINT ( 'NONE',  ( 86.10128179547638183, 47.01522930412662760, 10.71950609365847917 ) ) ;
#52706=CARTESIAN_POINT ( 'NONE',  ( 70.56976607031667470, 69.33912239971135705, -8.253513271727511480 ) ) ;
#52709=CARTESIAN_POINT ( 'NONE',  ( 72.30143066935100649, 72.00106423939931233, -3.615897486538043548 ) ) ;
#52712=ORIENTED_EDGE ( 'NONE', *, *, #670, .T. ) ;
#52714=CARTESIAN_POINT ( 'NONE',  ( 66.77293986438145623, 68.13932227484529847, -6.519502098149898117 ) ) ;
#52715=CARTESIAN_POINT ( 'NONE',  ( 72.64601778605843663, 70.71744408260791204, -7.969226289351840187 ) ) ;
#52719=CARTESIAN_POINT ( 'NONE',  ( 22.60804823384966156, 31.79103043416549923, 8.090169943749478065 ) ) ;
#52720=CARTESIAN_POINT ( 'NONE',  ( 85.91498916281075537, 48.46192805135255099, 12.13455285288522667 ) ) ;
#52722=CARTESIAN_POINT ( 'NONE',  ( 71.94430347986846641, 71.72799717812090137, -3.886761019894646729 ) ) ;
#52727=CARTESIAN_POINT ( 'NONE',  ( 76.26946404230703536, 64.97317754398874001, 14.67006731301516176 ) ) ;
#52730=CARTESIAN_POINT ( 'NONE',  ( 72.57773168451072365, 70.69087215581753014, -7.948841485240758509 ) ) ;
#52731=CARTESIAN_POINT ( 'NONE',  ( 78.91212607377818244, 60.09823531620596526, 16.11286148787682393 ) ) ;
#52739=CARTESIAN_POINT ( 'NONE',  ( 19.11131643181922968, 13.96004757982089473, -5.678558825948276656 ) ) ;
#52741=CARTESIAN_POINT ( 'NONE',  ( 71.81391265307100014, 59.05408711125518550, 15.37230141137981754 ) ) ;
#52745=VERTEX_POINT ( 'NONE', #13103 ) ;
#52746=CARTESIAN_POINT ( 'NONE',  ( 86.41880224017843659, 45.50969932908875393, -7.944645677213507895 ) ) ;
#52748=CARTESIAN_POINT ( 'NONE',  ( 81.46654924364905526, 42.47797946394854307, 7.469209086924764485 ) ) ;
#52753=CARTESIAN_POINT ( 'NONE',  ( 20.44528175232247591, 34.73705186507753950, -3.090169943749475845 ) ) ;
#52761=CARTESIAN_POINT ( 'NONE',  ( 71.93357406896315354, 69.69179662921422391, 8.874436160946375551 ) ) ;
#52762=CARTESIAN_POINT ( 'NONE',  ( 80.39015929397758953, 57.47250276623566378, -16.58917374605577777 ) ) ;
#52763=CARTESIAN_POINT ( 'NONE',  ( 67.84059961315651321, 69.51487248268222174, -4.691999901035240228 ) ) ;
#52764=EDGE_LOOP ( 'NONE', ( #76377, #55768, #96495, #91666 ) ) ;
#52768=VERTEX_POINT ( 'NONE', #36368 ) ;
#52772=VERTEX_POINT ( 'NONE', #11115 ) ;
#52780=CARTESIAN_POINT ( 'NONE',  ( 83.32631514680937812, 52.40275339355609674, 14.85530416217961047 ) ) ;
#52783=ORIENTED_EDGE ( 'NONE', *, *, #93713, .T. ) ;
#52784=CARTESIAN_POINT ( 'NONE',  ( 78.48876124178367775, 51.94357913415533545, -15.95536876511241964 ) ) ;
#52785=CARTESIAN_POINT ( 'NONE',  ( 83.05016518402850068, 42.76510943801325482, -6.363870132515760503 ) ) ;
#52790=DIRECTION ( 'NONE',  ( 0.1710100716628310258, -0.2961981327260192476, 0.9396926207859104263 ) ) ;
#52793=CARTESIAN_POINT ( 'NONE',  ( 75.09455210346366982, 57.68713258346969042, -16.03622425841626509 ) ) ;
#52796=CARTESIAN_POINT ( 'NONE',  ( 67.14666838648643932, 66.78363720521792857, 8.171468515940333077 ) ) ;
#52799=LINE ( 'NONE', #55780, #56099 ) ;
#52803=CARTESIAN_POINT ( 'NONE',  ( 74.51860651786539336, 54.69479437051430892, -16.14050065589297844 ) ) ;
#52805=CARTESIAN_POINT ( 'NONE',  ( 85.72891561183703857, 43.80477521659179274, 6.542285751333638544 ) ) ;
#52806=CARTESIAN_POINT ( 'NONE',  ( 79.69883455371483194, 45.99209036072507928, 12.97227174178035192 ) ) ;
#52808=CARTESIAN_POINT ( 'NONE',  ( 79.41561859137864587, 54.73972641915754878, -16.40726218708634931 ) ) ;
#52810=ORIENTED_EDGE ( 'NONE', *, *, #84255, .T. ) ;
#52814=CYLINDRICAL_SURFACE ( 'NONE', #22445, 10.00000000000001066 ) ;
#52827=CARTESIAN_POINT ( 'NONE',  ( 72.78342027449815532, 68.81891707817121073, 9.930820707867006547 ) ) ;
#52836=CARTESIAN_POINT ( 'NONE',  ( 81.98204644740465596, 41.14170829992954026, -5.380964918555401155 ) ) ;
#52837=B_SPLINE_CURVE_WITH_KNOTS ( 'NONE', 3,
 ( #26166, #82772, #13339, #44696, #36606, #80407, #20440, #4741 ),
 .UNSPECIFIED., .F., .F.,
 ( 4, 2, 2, 4 ),
 ( 0.1732562812666568475, 0.5866281406333284654, 0.7933140703166642327, 1.000000000000000000 ),
 .UNSPECIFIED. ) ;
#52843=B_SPLINE_CURVE_WITH_KNOTS ( 'NONE', 3,
 ( #17595, #39864, #70801, #94133, #1410, #63192, #48504, #10007, #33291, #64193 ),
 .UNSPECIFIED., .F., .F.,
 ( 4, 2, 2, 2, 4 ),
 ( 0.000000000000000000, 0.0002622400424272842436, 0.0005244800848545684872, 0.0007867201272818526766, 0.001048960169709136974 ),
 .UNSPECIFIED. ) ;
#52848=CARTESIAN_POINT ( 'NONE',  ( 3.540199675970839177, 23.81751292744053217, -6.180339887498951690 ) ) ;
#52850=CARTESIAN_POINT ( 'NONE',  ( 71.86919472611239712, 59.31234992600734302, -15.30864741555868846 ) ) ;
#52851=CARTESIAN_POINT ( 'NONE',  ( 84.06604358195920668, 51.46910565605918464, 14.65639964578790533 ) ) ;
#52855=CARTESIAN_POINT ( 'NONE',  ( 74.02416338248266925, 55.20782277953769324, 16.12359275168059369 ) ) ;
#52857=CARTESIAN_POINT ( 'NONE',  ( 66.08289746408667042, 68.56685657833568825, -4.488094959726262267 ) ) ;
#52863=CARTESIAN_POINT ( 'NONE',  ( 20.18904385193075868, 29.84336893147756342, -7.433330006724137462 ) ) ;
#52864=FACE_OUTER_BOUND ( 'NONE', #39070, .T. ) ;
#52866=CARTESIAN_POINT ( 'NONE',  ( 75.18533445981178431, 53.54581650303052243, -16.05318290065117282 ) ) ;
#52867=CARTESIAN_POINT ( 'NONE',  ( 88.45605923504750479, 44.01628325393264873, 2.215908606781754830 ) ) ;
#52876=ORIENTED_EDGE ( 'NONE', *, *, #45220, .T. ) ;
#52879=B_SPLINE_CURVE_WITH_KNOTS ( 'NONE', 3,
 ( #46658, #60844, #83714, #91806, #6171, #29474, #69953, #84219, #77585, #53746, #78, #14272, #15246, #60347, #45648, #28988, #46142, #76576, #59863, #7157, #92313, #38044, #76102, #21380 ),
 .UNSPECIFIED., .F., .F.,
 ( 4, 2, 2, 2, 2, 2, 2, 2, 2, 2, 2, 4 ),
 ( 0.000000000000000000, 0.1249999999999653333, 0.2499999999999306666, 0.3749999999998959721, 0.4374999999999003020, 0.4999999999999046318, 0.5624999999999089617, 0.6249999999999132916, 0.6874999999999176215, 0.7499999999999218403, 0.8749999999999609201, 1.000000000000000000 ),
 .UNSPECIFIED. ) ;
#52889=CARTESIAN_POINT ( 'NONE',  ( 19.46611421548295695, 12.20801979619928090, -3.090169943749474069 ) ) ;
#52890=CARTESIAN_POINT ( 'NONE',  ( 83.97117539556700194, 48.10897359057201328, 12.72530908371034464 ) ) ;
#52901=CARTESIAN_POINT ( 'NONE',  ( 21.19816502305182837, 13.20801979619928268, -3.090169943749474069 ) ) ;
#52907=CARTESIAN_POINT ( 'NONE',  ( 81.53796252524934118, 42.62971458812653935, -7.650143360278183202 ) ) ;
#52912=CARTESIAN_POINT ( 'NONE',  ( 81.12979385446129754, 48.93447223002202406, 13.74866293976100806 ) ) ;
#52916=EDGE_LOOP ( 'NONE', ( #88353, #20142, #72490, #65575 ) ) ;
#52923=CARTESIAN_POINT ( 'NONE',  ( 82.74206721279597332, 53.66691124579689642, -15.75745978315255869 ) ) ;
#52925=CARTESIAN_POINT ( 'NONE',  ( 66.18410330236099526, 68.78720517270650703, 0.1136469981348479652 ) ) ;
#52926=CARTESIAN_POINT ( 'NONE',  ( 14.44441505419593064, 16.84335787977761711, 9.188101187500006262 ) ) ;
#52928=CARTESIAN_POINT ( 'NONE',  ( 80.74781574657599492, 57.21644485803225422, 16.56566952311892749 ) ) ;
#52934=CARTESIAN_POINT ( 'NONE',  ( 79.73556474071195055, 44.84470626076887356, 11.43605411104022096 ) ) ;
#52942=CARTESIAN_POINT ( 'NONE',  ( 86.70911053808110580, 46.89117940024963360, 10.21290512048939547 ) ) ;
#52950=CARTESIAN_POINT ( 'NONE',  ( 72.12653191652874796, 72.33473008883520095, 0.9717078169766214524 ) ) ;
#52951=CARTESIAN_POINT ( 'NONE',  ( 72.99805664120070503, 70.78149395872682703, 8.185774945494646460 ) ) ;
#52963=CARTESIAN_POINT ( 'NONE',  ( 83.32045823979383670, 44.28835298952803612, 8.667801982703636554 ) ) ;
#52968=DIRECTION ( 'NONE',  ( -0.4755282581475737680, 0.8236391035463299648, -0.3090169943749573878 ) ) ;
#52969=CARTESIAN_POINT ( 'NONE',  ( 75.58214075417596689, 65.23491603964201602, 14.35294216029143399 ) ) ;
#52970=B_SPLINE_CURVE_WITH_KNOTS ( 'NONE', 3,
 ( #47125, #86196, #24827, #17223, #2554, #48131, #32436, #94272, #33437, #8141, #69922, #98770, #58239, #13167, #29352, #6550 ),
 .UNSPECIFIED., .F., .F.,
 ( 4, 1, 2, 2, 2, 1, 2, 2, 4 ),
 ( 0.000000000000000000, 0.1250000000000044964, 0.1875000000000050238, 0.2500000000000055511, 0.5000000000000083267, 0.6250000000000118794, 0.6875000000000123235, 0.7500000000000108802, 1.000000000000000000 ),
 .UNSPECIFIED. ) ;
#52972=VECTOR ( 'NONE', #39377, 1000.000000000000114 ) ;
#52973=CARTESIAN_POINT ( 'NONE',  ( 76.68665551218811061, 54.72605516139766024, -16.09894948477438703 ) ) ;
#52980=CARTESIAN_POINT ( 'NONE',  ( 70.65108737845197595, 70.93011541185489932, 3.799750337262588040 ) ) ;
#52984=CARTESIAN_POINT ( 'NONE',  ( 82.15581729306063608, 41.47318868828376281, -5.933381251846729931 ) ) ;
#52987=CARTESIAN_POINT ( 'NONE',  ( 3.479571460297436136, 22.98502408145589726, -5.678558825948271327 ) ) ;
#52988=CARTESIAN_POINT ( 'NONE',  ( 68.12716324602396867, 65.77153025955813348, 10.88064167488197143 ) ) ;
#52989=CYLINDRICAL_SURFACE ( 'NONE', #88948, 10.00000000000001066 ) ;
#52991=CARTESIAN_POINT ( 'NONE',  ( 85.28284199416806644, 42.68018856290509433, -2.168919532025619379 ) ) ;
#52998=CARTESIAN_POINT ( 'NONE',  ( 29.31840136419365805, 25.43085787977764056, -9.188101187500008038 ) ) ;
#53004=CARTESIAN_POINT ( 'NONE',  ( 70.36717637110562862, 61.12986366949047579, 14.33409245634332585 ) ) ;
#53011=CARTESIAN_POINT ( 'NONE',  ( 73.10017469210082197, 69.78597432261236122, 9.621008654245756020 ) ) ;
#53022=CARTESIAN_POINT ( 'NONE',  ( 41.28156676870083430, 26.76004757982093452, 5.678558825948272215 ) ) ;
#53024=CARTESIAN_POINT ( 'NONE',  ( 72.95814459691263210, 63.22145188874699073, -14.59938505178614498 ) ) ;
#53028=ORIENTED_EDGE ( 'NONE', *, *, #45266, .T. ) ;
#53040=CARTESIAN_POINT ( 'NONE',  ( 77.11998379669407200, 62.91817058770694615, -15.28160261259852959 ) ) ;
#53043=EDGE_LOOP ( 'NONE', ( #25602, #65755, #41707, #82758, #39462, #48321 ) ) ;
#53046=CARTESIAN_POINT ( 'NONE',  ( 35.86231599663030067, 42.74646525600393687, 2.839279412974139660 ) ) ;
#53049=ORIENTED_EDGE ( 'NONE', *, *, #95857, .F. ) ;
#53052=CARTESIAN_POINT ( 'NONE',  ( 74.16736989203016606, 68.80940149631990721, -11.31408104362165545 ) ) ;
#53054=B_SPLINE_SURFACE_WITH_KNOTS ( 'NONE', 3, 1, ( 
 ( #52506, #53986 ),
 ( #21142, #91547 ),
 ( #92066, #76335 ),
 ( #67214, #44405 ),
 ( #37305, #68205 ),
 ( #22616, #24103 ),
 ( #94048, #2326 ),
 ( #16503, #47398 ),
 ( #78324, #24601 ),
 ( #71227, #48411 ),
 ( #25096, #9924 ),
 ( #40785, #96422 ),
 ( #77314, #23589 ),
 ( #31197, #93033 ),
 ( #20896, #67465 ),
 ( #4171, #65975 ),
 ( #12292, #75089 ),
 ( #6166, #74092 ),
 ( #52263, #29467 ),
 ( #27966, #89816 ),
 ( #37063, #60342 ),
 ( #50273, #58365 ),
 ( #89342, #58846 ),
 ( #4685, #82226 ),
 ( #14760, #71 ),
 ( #45642, #30459 ),
 ( #31945, #38038 ),
 ( #15744, #61351 ),
 ( #77578, #83709 ),
 ( #29962, #31446 ),
 ( #23847, #91799 ) ),
 .UNSPECIFIED., .F., .F., .F.,
 ( 4, 3, 3, 3, 3, 3, 3, 3, 3, 3, 4 ),
 ( 2, 2 ),
 ( 0.000000000000000000, 0.1122669598086783738, 0.2243161639709696786, 0.3396355846219157870, 0.4553962076585107988, 0.5677860799922528345, 0.6749047109689648716, 0.7773884377078369434, 0.8775581155834392133, 0.9782364162377953365, 1.000000000000000000 ),
 ( 0.000000000000000000, 1.000000000000000000 ),
 .UNSPECIFIED. ) ;
#53062=CYLINDRICAL_SURFACE ( 'NONE', #49506, 10.00000000000001066 ) ;
#53068=CARTESIAN_POINT ( 'NONE',  ( 67.12420765758699304, 68.84019135822225621, -3.751863413797577707 ) ) ;
#53075=CARTESIAN_POINT ( 'NONE',  ( 72.62183550608976645, 66.39385476340312664, 12.02826447586101644 ) ) ;
#53080=CARTESIAN_POINT ( 'NONE',  ( 71.72870690310715247, 72.16142621409359492, 3.283488654313281963 ) ) ;
#53081=CARTESIAN_POINT ( 'NONE',  ( 84.68957885917166095, 45.88504986743041059, 9.714594249952936522 ) ) ;
#53082=CARTESIAN_POINT ( 'NONE',  ( 87.33294734268929460, 44.88192199842171703, 6.808005391826775110 ) ) ;
#53085=CARTESIAN_POINT ( 'NONE',  ( 82.69574664279603837, 54.03060105484253484, -15.86596363536033039 ) ) ;
#53090=CARTESIAN_POINT ( 'NONE',  ( 66.44089328032605124, 67.93038546761928842, 6.554334301446774091 ) ) ;
#53093=CARTESIAN_POINT ( 'NONE',  ( 73.41757211889691348, 69.17622104212573220, -9.975606977152791544 ) ) ;
#53095=CARTESIAN_POINT ( 'NONE',  ( 1.988115337714555064, 24.08080186712590276, -3.090169943749475845 ) ) ;
#53096=CARTESIAN_POINT ( 'NONE',  ( 41.55205903992003158, 29.15404122711137447, 8.090169943749479842 ) ) ;
#53100=CARTESIAN_POINT ( 'NONE',  ( 71.78913936505468030, 72.20160104369585952, 3.260718063500208430 ) ) ;
#53101=EDGE_CURVE ( 'NONE', #36219, #9880, #84393, .T. ) ;
#53111=CARTESIAN_POINT ( 'NONE',  ( 18.86656744736070124, 32.93396525600390845, 2.839279412974139660 ) ) ;
#53114=CARTESIAN_POINT ( 'NONE',  ( 45.82169850708434922, 28.58380873178791504, 6.180339887498953466 ) ) ;
#53116=CARTESIAN_POINT ( 'NONE',  ( 77.33488381500329467, 63.19222936695796733, 15.59520410795408196 ) ) ;
#53128=ORIENTED_EDGE ( 'NONE', *, *, #74241, .T. ) ;
#53136=CARTESIAN_POINT ( 'NONE',  ( 79.32826970724438809, 45.68448480011694812, -12.90705109908815906 ) ) ;
#53142=CARTESIAN_POINT ( 'NONE',  ( 22.66683848874176022, 18.80170272979926693, 7.433330006724137462 ) ) ;
#53143=CARTESIAN_POINT ( 'NONE',  ( 75.31615383312099254, 56.31091532350969686, 16.14109913096982396 ) ) ;
#53144=CARTESIAN_POINT ( 'NONE',  ( 71.17509266960550462, 70.27285362950316028, -6.380606852064568457 ) ) ;
#53151=ORIENTED_EDGE ( 'NONE', *, *, #61268, .F. ) ;
#53153=CARTESIAN_POINT ( 'NONE',  ( 79.14672556360194733, 50.15886727742795870, -14.80520554370081854 ) ) ;
#53169=CARTESIAN_POINT ( 'NONE',  ( 79.37503556926780846, 45.76590238620419626, 12.94519473234442231 ) ) ;
#53176=CARTESIAN_POINT ( 'NONE',  ( 66.72442129515968645, 67.86934472784028571, 6.990068089071483470 ) ) ;
#53181=CARTESIAN_POINT ( 'NONE',  ( 71.53524002805265525, 66.98255073825953332, 10.96953089586062546 ) ) ;
#53182=VERTEX_POINT ( 'NONE', #81297 ) ;
#53186=CARTESIAN_POINT ( 'NONE',  ( 76.07519723137014012, 51.47020756999099689, -16.16347409184471573 ) ) ;
#53187=VECTOR ( 'NONE', #97494, 1000.000000000000114 ) ;
#53197=CARTESIAN_POINT ( 'NONE',  ( 80.25013155102732298, 44.94815484363307689, -11.26109297976839052 ) ) ;
#53199=CARTESIAN_POINT ( 'NONE',  ( 72.87908800440395396, 70.94240749453250316, 7.824389999597036294 ) ) ;
#53206=CARTESIAN_POINT ( 'NONE',  ( 87.97782240006738164, 43.76496563450900368, 2.369043524150745927 ) ) ;
#53207=CARTESIAN_POINT ( 'NONE',  ( 79.88561257828403939, 47.45582108751673189, 13.26507963048562289 ) ) ;
#53215=LINE ( 'NONE', #85152, #54996 ) ;
#53218=CARTESIAN_POINT ( 'NONE',  ( 30.27384506023333444, 17.28848085856232331, 1.475505719884397138E-15 ) ) ;
#53221=CARTESIAN_POINT ( 'NONE',  ( 16.60635795911645829, 31.36126292948894445, 6.180339887498949913 ) ) ;
#53226=CARTESIAN_POINT ( 'NONE',  ( 66.90909321514121189, 68.17756947893454367, -6.600776075520579766 ) ) ;
#53227=CARTESIAN_POINT ( 'NONE',  ( 73.09402281141575486, 70.66127457103814891, -7.741035114144303897 ) ) ;
#53231=CARTESIAN_POINT ( 'NONE',  ( 19.12865694409072503, 32.81751292744056769, -6.180339887498951690 ) ) ;
#53232=CARTESIAN_POINT ( 'NONE',  ( 76.88190494917691353, 52.40768971240707685, 16.25993826842571366 ) ) ;
#53234=CARTESIAN_POINT ( 'NONE',  ( 72.13262339782576760, 71.82946044270117625, -3.914888389595029938 ) ) ;
#53243=CARTESIAN_POINT ( 'NONE',  ( 67.72263284813347184, 69.74190012044236653, -3.715451582779847328 ) ) ;
#53245=CARTESIAN_POINT ( 'NONE',  ( 35.77750112005064409, 38.84336893147759184, -7.433330006724137462 ) ) ;
#53252=CARTESIAN_POINT ( 'NONE',  ( 14.52983486323338802, 31.49540643055186706, 3.479690158560446702E-15 ) ) ;
#53254=CARTESIAN_POINT ( 'NONE',  ( 72.03620616349491002, 59.26415205210582826, 15.85034427342174901 ) ) ;
#53260=CARTESIAN_POINT ( 'NONE',  ( 81.64803324908639581, 42.02089059119690972, 7.567395689010925075 ) ) ;
#53263=CARTESIAN_POINT ( 'NONE',  ( 72.62492194693132319, 71.47378110219968050, -5.675874693310046126 ) ) ;
#53269=ORIENTED_EDGE ( 'NONE', *, *, #33961, .F. ) ;
#53274=CARTESIAN_POINT ( 'NONE',  ( 69.35253854976203058, 63.01665765323906498, 13.58811665770852350 ) ) ;
#53275=CARTESIAN_POINT ( 'NONE',  ( 81.49862395535369330, 59.56456120573196245, 0.1209609477998291605 ) ) ;
#53276=CARTESIAN_POINT ( 'NONE',  ( 69.19273132923471792, 69.74333897986481645, -6.091390803950828214 ) ) ;
#53283=CARTESIAN_POINT ( 'NONE',  ( 75.00226567582841142, 65.52623940974007155, 13.57230656279164727 ) ) ;
#53284=VERTEX_POINT ( 'NONE', #66546 ) ;
#53289=CARTESIAN_POINT ( 'NONE',  ( 36.70787689013189947, 33.14441083166263979, 10.00000000000000533 ) ) ;
#53291=CARTESIAN_POINT ( 'NONE',  ( 83.13520543127567919, 52.15262426605146118, 14.79738518802719049 ) ) ;
#53294=CARTESIAN_POINT ( 'NONE',  ( 73.67505968516064740, 69.57270177156178192, 9.668646285131167417 ) ) ;
#53296=CARTESIAN_POINT ( 'NONE',  ( 82.31933756389703660, 53.70313499084333841, 15.83617117143144526 ) ) ;
#53302=CARTESIAN_POINT ( 'NONE',  ( 69.80658768130543024, 67.27183608565839279, 9.609976433168107235 ) ) ;
#53305=CARTESIAN_POINT ( 'NONE',  ( 78.02686697169625063, 47.82505017202286979, 14.03973303039792597 ) ) ;
#53308=CARTESIAN_POINT ( 'NONE',  ( 71.69449150190311570, 68.87257317924374433, 9.071537784185924380 ) ) ;
#53310=CARTESIAN_POINT ( 'NONE',  ( 79.10360752189127709, 45.94674753059116057, 13.17468094630847375 ) ) ;
#53332=CARTESIAN_POINT ( 'NONE',  ( 74.03799347921402330, 64.05404633756495514, 14.51082138824052414 ) ) ;
#53335=CARTESIAN_POINT ( 'NONE',  ( 81.89176746338951318, 41.27503766206196190, -5.828951561110701007 ) ) ;
#53337=FACE_OUTER_BOUND ( 'NONE', #3567, .T. ) ;
#53349=CARTESIAN_POINT ( 'NONE',  ( 12.53574365251957090, 15.43677371833799938, -10.00000000000000355 ) ) ;
#53351=CARTESIAN_POINT ( 'NONE',  ( 71.67479916869325507, 58.94068462711909007, -15.88111808811495607 ) ) ;
#53352=DIRECTION ( 'NONE',  ( -0.9563064286990893281, 0.2923662333936558611, 0.000000000000000000 ) ) ;
#53357=CARTESIAN_POINT ( 'NONE',  ( 74.23329481810236530, 55.36962176604209418, 16.12301265312518339 ) ) ;
#53360=ORIENTED_EDGE ( 'NONE', *, *, #15013, .F. ) ;
#53364=CARTESIAN_POINT ( 'NONE',  ( 33.66714878060290772, 21.29860640527294180, -2.839279412974138328 ) ) ;
#53370=CARTESIAN_POINT ( 'NONE',  ( 68.48051572044573732, 64.33975350462213783, 12.32598567578913773 ) ) ;
#53383=DIRECTION ( 'NONE',  ( -0.5840252505817192796, 0.000000000000000000, 0.8117354905897362638 ) ) ;
#53384=CARTESIAN_POINT ( 'NONE',  ( 66.86954601471772719, 67.94335577711918006, 5.821787759504553073 ) ) ;
#53387=PLANE ( 'NONE',  #12655 ) ;
#53390=CARTESIAN_POINT ( 'NONE',  ( 86.55657754374946933, 47.30628205130771136, -10.74852006680811023 ) ) ;
#53391=CARTESIAN_POINT ( 'NONE',  ( 84.82053053956542499, 45.10610155585538905, -8.666442846737737682 ) ) ;
#53392=VERTEX_POINT ( 'NONE', #80814 ) ;
#53396=CARTESIAN_POINT ( 'NONE',  ( 79.38118373144868656, 59.76411540931838573, -16.16477398176405345 ) ) ;
#53398=CARTESIAN_POINT ( 'NONE',  ( 75.22798512741415777, 53.64680820920216320, -16.53898548151806835 ) ) ;
#53399=CARTESIAN_POINT ( 'NONE',  ( 69.95047170429380401, 62.88811978159139215, 13.86734351276082045 ) ) ;
#53404=CARTESIAN_POINT ( 'NONE',  ( 81.64670023727850889, 42.65128533460878657, -7.584980231169037523 ) ) ;
#53408=CARTESIAN_POINT ( 'NONE',  ( 81.98602009217056263, 53.23458893094329625, 15.38303897364004236 ) ) ;
#53410=CARTESIAN_POINT ( 'NONE',  ( 69.86600153435685456, 70.48283808624711355, 3.777498432527079064 ) ) ;
#53412=ORIENTED_EDGE ( 'NONE', *, *, #24343, .F. ) ;
#53414=CARTESIAN_POINT ( 'NONE',  ( 82.36208054384441368, 41.26681451557220015, 3.281558084501622563 ) ) ;
#53417=CARTESIAN_POINT ( 'NONE',  ( 82.75931229668888989, 53.79267046329768220, -15.79052045153009409 ) ) ;
#53419=CARTESIAN_POINT ( 'NONE',  ( 15.78914702631840328, 24.51421378149918695, -9.188101187500004485 ) ) ;
#53423=ORIENTED_EDGE ( 'NONE', *, *, #10509, .F. ) ;
#53428=CARTESIAN_POINT ( 'NONE',  ( 81.73013690182854418, 46.02429500294771714, -11.48451531274605486 ) ) ;
#53438=CARTESIAN_POINT ( 'NONE',  ( 82.67540033522136866, 44.72113521480816445, -9.646895689004646002 ) ) ;
#53441=CARTESIAN_POINT ( 'NONE',  ( 76.27486002672000609, 65.07516076971148777, 14.62441312286923889 ) ) ;
#53452=CARTESIAN_POINT ( 'NONE',  ( 68.61869731438623887, 66.71998516903308030, 10.18785472861651975 ) ) ;
#53456=PLANE ( 'NONE',  #92052 ) ;
#53459=CYLINDRICAL_SURFACE ( 'NONE', #1208, 16.60714546451156792 ) ;
#53461=CARTESIAN_POINT ( 'NONE',  ( 77.76328872507745871, 54.37645632513159910, -16.02018328028568561 ) ) ;
#53463=CARTESIAN_POINT ( 'NONE',  ( 68.54569597095012057, 64.23358675863970291, -12.43730015513902742 ) ) ;
#53468=CARTESIAN_POINT ( 'NONE',  ( 66.31795133325435643, 69.20145725284447735, 2.477662600225432055 ) ) ;
#53469=CARTESIAN_POINT ( 'NONE',  ( 67.91650730281627091, 67.19912629719564734, 8.215611842121816721 ) ) ;
#53477=CARTESIAN_POINT ( 'NONE',  ( 82.30224259357629535, 41.51585266698759824, -5.837696018585297963 ) ) ;
#53479=CARTESIAN_POINT ( 'NONE',  ( 13.34262526062736676, 23.10171378149917842, 9.188101187500008038 ) ) ;
#53480=CARTESIAN_POINT ( 'NONE',  ( 74.83829975255316924, 60.29844347012056005, -16.01251099248637644 ) ) ;
#53487=CARTESIAN_POINT ( 'NONE',  ( 35.85928575902275384, 36.10171378149922106, 9.188101187500008038 ) ) ;
#53488=CARTESIAN_POINT ( 'NONE',  ( 33.05130250568083738, 42.58029201028044497, 1.583844403245397769 ) ) ;
#53490=VERTEX_POINT ( 'NONE', #37130 ) ;
#53491=CARTESIAN_POINT ( 'NONE',  ( 33.29248241878940462, 22.14754757982091604, -5.678558825948276656 ) ) ;
#53492=CARTESIAN_POINT ( 'NONE',  ( 77.86555730066851311, 62.20866292688850052, -15.95979438352862090 ) ) ;
#53497=CARTESIAN_POINT ( 'NONE',  ( 84.78071699792324978, 50.02262005461608396, -13.67739062443489750 ) ) ;
#53504=ORIENTED_EDGE ( 'NONE', *, *, #9251, .T. ) ;
#53505=CARTESIAN_POINT ( 'NONE',  ( 78.41477381122238910, 47.32040575024743134, -14.22103711499937617 ) ) ;
#53506=CARTESIAN_POINT ( 'NONE',  ( 35.92184506804998279, 29.24335787977765477, -9.188101187500008038 ) ) ;
#53510=ORIENTED_EDGE ( 'NONE', *, *, #72967, .F. ) ;
#53514=CARTESIAN_POINT ( 'NONE',  ( 84.82554225155547556, 50.21385520134798242, 13.77498508261128407 ) ) ;
#53518=CARTESIAN_POINT ( 'NONE',  ( 42.37730965384162829, 25.26216523072498532, -2.296566073217252530E-15 ) ) ;
#53519=CARTESIAN_POINT ( 'NONE',  ( 81.27316195909862984, 55.43468901134095006, -16.33783760952318076 ) ) ;
#53526=CARTESIAN_POINT ( 'NONE',  ( 72.13789110140854177, 72.31505540346954319, -1.296595641072646243 ) ) ;
#53532=CARTESIAN_POINT ( 'NONE',  ( 78.40196830515944271, 59.44234872728634400, -16.13643701924537055 ) ) ;
#53542=EDGE_LOOP ( 'NONE', ( #70114, #17661, #34263, #23984 ) ) ;
#53544=CARTESIAN_POINT ( 'NONE',  ( 74.13858531873714242, 68.40778981217252408, -11.66187469989377767 ) ) ;
#53545=DIRECTION ( 'NONE',  ( 0.7905172007421661373, 0.000000000000000000, -0.6124398381316893403 ) ) ;
#53548=CARTESIAN_POINT ( 'NONE',  ( 32.81602777569660390, 24.11029122506295863, -8.090169943749478065 ) ) ;
#53562=CARTESIAN_POINT ( 'NONE',  ( 69.92518591997227873, 62.80814789249908614, -13.33122127648681499 ) ) ;
#53566=CARTESIAN_POINT ( 'NONE',  ( 72.93513805092823077, 67.35904576704696467, 11.40243080045951629 ) ) ;
#53567=CARTESIAN_POINT ( 'NONE',  ( 82.26825361666672620, 40.74351925651850337, -3.658449855531767714 ) ) ;
#53570=CARTESIAN_POINT ( 'NONE',  ( 81.50940192328098988, 59.54589321767952725, 0.1873032967079516220 ) ) ;
#53571=CARTESIAN_POINT ( 'NONE',  ( 78.14015596324891533, 47.79605781560270117, 14.53813849190288465 ) ) ;
#53574=CARTESIAN_POINT ( 'NONE',  ( 82.39556149134112673, 53.49063599510539291, -15.76428462505607975 ) ) ;
#53580=LINE ( 'NONE', #51602, #15794 ) ;
#53582=CARTESIAN_POINT ( 'NONE',  ( 67.63343560358070761, 69.65666620391252195, -0.2166577581527749097 ) ) ;
#53584=CARTESIAN_POINT ( 'NONE',  ( 76.00333185707168582, 51.30992116068062359, 16.13885810330130255 ) ) ;
#53586=EDGE_CURVE ( 'NONE', #29851, #16015, #21933, .T. ) ;
#53587=CARTESIAN_POINT ( 'NONE',  ( 69.42144788871625849, 62.89730317705431872, 13.10748580973936939 ) ) ;
#53590=CARTESIAN_POINT ( 'NONE',  ( 71.94524616390265237, 71.98672967291759051, 2.832588148037977760 ) ) ;
#53596=CARTESIAN_POINT ( 'NONE',  ( 82.87264987968924856, 49.76174821331473197, -13.67541387821871446 ) ) ;
#53599=CARTESIAN_POINT ( 'NONE',  ( 26.36427918851389762, 18.14754757982090538, -5.678558825948275768 ) ) ;
#53602=CARTESIAN_POINT ( 'NONE',  ( 6.569006713621681648, 25.83396525600388216, -2.839279412974133887 ) ) ;
#53607=CARTESIAN_POINT ( 'NONE',  ( 72.04273812837081437, 59.28583566120335746, 15.34548535902080246 ) ) ;
#53611=CARTESIAN_POINT ( 'NONE',  ( 87.70720954677142345, 45.31332896125894649, -6.372777740749068442 ) ) ;
#53617=CARTESIAN_POINT ( 'NONE',  ( 77.07955643721723504, 49.57937043545834399, 15.50364152264906004 ) ) ;
#53622=ORIENTED_EDGE ( 'NONE', *, *, #90259, .F. ) ;
#53624=CARTESIAN_POINT ( 'NONE',  ( 79.06748585747224922, 46.07688976562260308, -12.67383739758977335 ) ) ;
#53625=EDGE_CURVE ( 'NONE', #43189, #70075, #73573, .T. ) ;
#53630=CARTESIAN_POINT ( 'NONE',  ( 24.39888929631063519, 19.80170272979926693, 7.433330006724137462 ) ) ;
#53640=CARTESIAN_POINT ( 'NONE',  ( 67.91983461438699976, 65.33094372862520061, -10.47544803142360337 ) ) ;
#53656=CARTESIAN_POINT ( 'NONE',  ( 66.84316555279445993, 67.52164038403083168, 6.631609150140850950 ) ) ;
#53658=CARTESIAN_POINT ( 'NONE',  ( 87.20272978483724557, 43.17595422555252327, -1.293722201381849679 ) ) ;
#53660=CARTESIAN_POINT ( 'NONE',  ( 81.17432035541970947, 55.57579169957366361, 16.36820043613993292 ) ) ;
#53662=CARTESIAN_POINT ( 'NONE',  ( 72.47531805799239635, 69.29348212587751732, 9.109228493206927624 ) ) ;
#53671=CARTESIAN_POINT ( 'NONE',  ( 76.02744352951765450, 65.34233732453844823, -14.42760839744433632 ) ) ;
#53677=CARTESIAN_POINT ( 'NONE',  ( 87.76435223195018409, 44.22492802364795494, 4.686297260842066770 ) ) ;
#53687=CARTESIAN_POINT ( 'NONE',  ( 83.83627951286173641, 51.93148169815736281, 14.52308898787406655 ) ) ;
#53695=CARTESIAN_POINT ( 'NONE',  ( 74.02137029423680303, 55.08862506472077314, 16.60352351745309107 ) ) ;
#53696=ADVANCED_FACE ( 'NONE', ( #11129 ), #63302, .T. ) ;
#53697=CARTESIAN_POINT ( 'NONE',  ( 25.97889144642132919, 17.12755873383626692, -6.180339887498949025 ) ) ;
#53700=DIRECTION ( 'NONE',  ( 0.4851478631379963491, -0.8403007481384849875, 0.2419218955996714493 ) ) ;
#53707=CARTESIAN_POINT ( 'NONE',  ( 81.30818518503046732, 58.89441083166271085, 0.000000000000000000 ) ) ;
#53708=CARTESIAN_POINT ( 'NONE',  ( 72.88378191513223214, 70.30562453083473429, -8.123734786539317909 ) ) ;
#53713=CARTESIAN_POINT ( 'NONE',  ( 27.28458541428561901, 34.49103043416550918, -8.090169943749479842 ) ) ;
#53714=CARTESIAN_POINT ( 'NONE',  ( 78.07911708839047549, 58.44437905099346864, 16.56270159866548042 ) ) ;
#53717=CARTESIAN_POINT ( 'NONE',  ( 73.08094384907833785, 54.14441083166272506, 0.000000000000000000 ) ) ;
#53721=CARTESIAN_POINT ( 'NONE',  ( 35.06352437372438402, 42.01751292744059185, 6.180339887498949913 ) ) ;
#53725=CARTESIAN_POINT ( 'NONE',  ( 66.50602851107427682, 67.82027345181231226, 6.844793838059969104 ) ) ;
#53727=CARTESIAN_POINT ( 'NONE',  ( 41.60632629512001301, 26.94754757982092741, 5.678558825948272215 ) ) ;
#53734=CARTESIAN_POINT ( 'NONE',  ( 19.94606896448370392, 26.91421378149918553, 9.188101187500008038 ) ) ;
#53735=CARTESIAN_POINT ( 'NONE',  ( 6.588875291771465470, 26.73705186507752174, -3.090169943749475845 ) ) ;
#53736=CARTESIAN_POINT ( 'NONE',  ( 71.52294418693975331, 59.11029950019791812, 15.31128158434694519 ) ) ;
#53741=CARTESIAN_POINT ( 'NONE',  ( 81.43393898548352183, 42.46093713096067290, 7.472239458194745332 ) ) ;
#53745=CARTESIAN_POINT ( 'NONE',  ( 72.35257617177605027, 71.70739429922333841, -5.765621772327581773 ) ) ;
#53746=CARTESIAN_POINT ( 'NONE',  ( 77.01650215582269254, 63.78770094747507358, 14.95761047872078642 ) ) ;
#53755=CARTESIAN_POINT ( 'NONE',  ( 30.82863370761418409, 19.92755873383627119, 6.180339887498953466 ) ) ;
#53756=CARTESIAN_POINT ( 'NONE',  ( 80.19730562280793151, 57.80653512312768072, 16.60264294324889178 ) ) ;
#53762=CARTESIAN_POINT ( 'NONE',  ( 74.39841895140679640, 68.21392270468032848, 11.45628786500076579 ) ) ;
#53766=DIRECTION ( 'NONE',  ( -0.8660254037844379305, -0.5000000000000014433, -0.000000000000000000 ) ) ;
#53771=CARTESIAN_POINT ( 'NONE',  ( 83.63039906669357038, 52.33209546183138627, 14.75250088251173075 ) ) ;
#53772=EDGE_LOOP ( 'NONE', ( #53510, #61501, #22655, #13869 ) ) ;
#53774=CARTESIAN_POINT ( 'NONE',  ( 87.13197742215592712, 46.34264934104920997, 8.620802749433925882 ) ) ;
#53779=CARTESIAN_POINT ( 'NONE',  ( 73.99515186948657686, 54.97541550358009488, -16.60506967685200763 ) ) ;
#53783=CARTESIAN_POINT ( 'NONE',  ( 69.36291866569143849, 66.30083069348447111, 10.37424756039578710 ) ) ;
#53787=CARTESIAN_POINT ( 'NONE',  ( 69.12385011120056788, 65.62576829796853417, -10.87672581319109000 ) ) ;
#53788=CARTESIAN_POINT ( 'NONE',  ( 78.61683564465192831, 47.48530518036562142, 14.24614870575583048 ) ) ;
#53791=CARTESIAN_POINT ( 'NONE',  ( 84.58391814946246257, 42.10937633166320637, 0.1196556675772392914 ) ) ;
#53792=CARTESIAN_POINT ( 'NONE',  ( 87.71554304996901408, 45.29005973903561966, -7.157883044737483047 ) ) ;
#53794=CARTESIAN_POINT ( 'NONE',  ( 79.47004366810152476, 45.79327920381835071, 12.92587503265258064 ) ) ;
#53800=CARTESIAN_POINT ( 'NONE',  ( 72.29498584114780613, 71.54824044162640462, 5.047338649552161272 ) ) ;
#53810=CARTESIAN_POINT ( 'NONE',  ( 68.52062231897753009, 66.34521348645475314, -9.781991027147515894 ) ) ;
#53812=CARTESIAN_POINT ( 'NONE',  ( 72.17391747568852622, 67.01067792759801023, 11.32486803574759904 ) ) ;
#53815=CARTESIAN_POINT ( 'NONE',  ( 72.21491844529387549, 53.64441083166271085, 0.000000000000000000 ) ) ;
#53830=CARTESIAN_POINT ( 'NONE',  ( 14.46184932687122604, 20.30066082961420904, -10.00000000000000533 ) ) ;
#53833=DIRECTION ( 'NONE',  ( 0.2837547813814350617, 0.9281390619545438758, 0.2409172175609567979 ) ) ;
#53837=CARTESIAN_POINT ( 'NONE',  ( 72.79159666541453078, 57.09351760226002881, 16.38642577662735533 ) ) ;
#53838=CARTESIAN_POINT ( 'NONE',  ( 70.90848803616628970, 68.75243874516947074, 9.337650187172339855 ) ) ;
#53840=EDGE_LOOP ( 'NONE', ( #13800, #76123, #55886, #71632 ) ) ;
#53845=CARTESIAN_POINT ( 'NONE',  ( 33.10845880387886808, 31.06628583063843863, -9.188101187500006262 ) ) ;
#53849=CARTESIAN_POINT ( 'NONE',  ( 88.48648755238653507, 43.99326657310299282, 1.937087981213223786 ) ) ;
#53851=CARTESIAN_POINT ( 'NONE',  ( 69.02454561260198318, 64.16955637294137205, 12.06084141314768132 ) ) ;
#53856=CARTESIAN_POINT ( 'NONE',  ( 9.022134044517839513, 26.18502408145590010, 5.678558825948276656 ) ) ;
#53861=AXIS2_PLACEMENT_3D ( 'NONE', #66827, #34925, #74465 ) ;
#53862=CARTESIAN_POINT ( 'NONE',  ( 71.61987371496262256, 72.44464069648769566, 0.9664813023029465988 ) ) ;
#53865=PLANE ( 'NONE',  #67159 ) ;
#53868=ORIENTED_EDGE ( 'NONE', *, *, #16470, .F. ) ;
#53880=CARTESIAN_POINT ( 'NONE',  ( 74.89047242489884582, 53.29799059985631260, -16.52631573936391618 ) ) ;
#53882=CARTESIAN_POINT ( 'NONE',  ( 69.44224152808193651, 62.71418222078327176, 13.79865581567335298 ) ) ;
#53887=CARTESIAN_POINT ( 'NONE',  ( 81.25434452997238566, 42.43560832920070425, -7.602236268904982275 ) ) ;
#53892=CARTESIAN_POINT ( 'NONE',  ( 73.93846185904290280, 63.82218318657452727, 14.12196739231004905 ) ) ;
#53894=CARTESIAN_POINT ( 'NONE',  ( 70.00673748363735172, 70.63212956676815679, 3.539627672355045274 ) ) ;
#53895=CARTESIAN_POINT ( 'NONE',  ( 87.90004739103230236, 45.00901072816739656, 6.408389154966706691 ) ) ;
#53898=CARTESIAN_POINT ( 'NONE',  ( 83.02255207477764998, 48.37928522878374338, 12.76191819685389817 ) ) ;
#53899=B_SPLINE_CURVE_WITH_KNOTS ( 'NONE', 3,
 ( #85317, #77695, #37173, #14384, #15862, #22475, #61463, #21974, #98995, #6778, #92412, #46246, #177, #7265, #22961, #77170 ),
 .UNSPECIFIED., .F., .F.,
 ( 4, 1, 2, 2, 2, 1, 2, 2, 4 ),
 ( 0.000000000000000000, 0.1249999999999957812, 0.1874999999999948097, 0.2499999999999938383, 0.4999999999999990008, 0.6250000000000004441, 0.6875000000000009992, 0.7500000000000015543, 1.000000000000000000 ),
 .UNSPECIFIED. ) ;
#53901=EDGE_CURVE ( 'NONE', #93491, #68256, #6987, .T. ) ;
#53902=LINE ( 'NONE', #7318, #48499 ) ;
#53903=CARTESIAN_POINT ( 'NONE',  ( 69.14012651450867963, 68.42618068722562441, -7.476854798959941206 ) ) ;
#53905=CARTESIAN_POINT ( 'NONE',  ( 74.66924941948499850, 57.12397588965591666, -16.51158835550184989 ) ) ;
#53906=CARTESIAN_POINT ( 'NONE',  ( 17.58072690530697813, 12.01110640527291373, 2.839279412974134775 ) ) ;
#53909=ORIENTED_EDGE ( 'NONE', *, *, #91401, .T. ) ;
#53918=CARTESIAN_POINT ( 'NONE',  ( 74.51634471081780475, 62.42820743237073344, -14.86162480667644736 ) ) ;
#53923=CARTESIAN_POINT ( 'NONE',  ( 73.02433024948126672, 69.66517378990661769, 9.714162469163332148 ) ) ;
#53924=CARTESIAN_POINT ( 'NONE',  ( 72.70196728203136161, 70.94362825444909504, 7.654249537423017280 ) ) ;
#53926=CARTESIAN_POINT ( 'NONE',  ( 87.97782240006738164, 43.76496563450897526, 2.369043524150738822 ) ) ;
#53946=DIRECTION ( 'NONE',  ( 0.000000000000000000, -0.6788029332000725669, -0.7343204871709475556 ) ) ;
#53948=CIRCLE ( 'NONE', #24817, 10.00000000000001066 ) ;
#53955=CARTESIAN_POINT ( 'NONE',  ( 71.25780773284164127, 62.14891183765285376, 14.64422194484298423 ) ) ;
#53958=CARTESIAN_POINT ( 'NONE',  ( 70.39480543937862933, 70.64432371323627535, 4.229459436019878282 ) ) ;
#53962=CARTESIAN_POINT ( 'NONE',  ( 75.08718269694753644, 62.23679730563473811, 15.49738829792160821 ) ) ;
#53965=CARTESIAN_POINT ( 'NONE',  ( 15.07467606819624173, 24.10171378149917842, 9.188101187500008038 ) ) ;
#53967=FACE_OUTER_BOUND ( 'NONE', #50914, .T. ) ;
#53968=CARTESIAN_POINT ( 'NONE',  ( 66.06006929221051394, 68.60032979153189103, 1.840660791566505861 ) ) ;
#53975=CARTESIAN_POINT ( 'NONE',  ( 66.51358226907667870, 69.48844138931383441, 1.167001339294358120 ) ) ;
#53976=EDGE_LOOP ( 'NONE', ( #1714, #13968, #89421, #33380 ) ) ;
#53977=CARTESIAN_POINT ( 'NONE',  ( 27.11724708220625857, 33.84336893147757763, -7.433330006724137462 ) ) ;
#53983=CARTESIAN_POINT ( 'NONE',  ( 78.91121342772640901, 49.10958624234372394, 14.40725116606144240 ) ) ;
#53986=CARTESIAN_POINT ( 'NONE',  ( 75.20389695419315501, 52.88180760346909892, -15.99093876381489032 ) ) ;
#53990=CARTESIAN_POINT ( 'NONE',  ( 30.86762485498029207, 38.79752408145593989, -5.678558825948271327 ) ) ;
#53995=CARTESIAN_POINT ( 'NONE',  ( 86.31423836152910667, 46.99325454369051869, -10.02800889789844163 ) ) ;
#54001=DIRECTION ( 'NONE',  ( -0.8660254037844379305, -0.5000000000000014433, -0.000000000000000000 ) ) ;
#54002=CARTESIAN_POINT ( 'NONE',  ( 81.40599722213572420, 56.18777044664494014, -16.43392898140639602 ) ) ;
#54006=ORIENTED_EDGE ( 'NONE', *, *, #10932, .F. ) ;
#54021=AXIS2_PLACEMENT_3D ( 'NONE', #39785, #33220, #70716 ) ;
#54024=CARTESIAN_POINT ( 'NONE',  ( 70.40687273385728417, 61.02326734534213415, -14.91946605292216610 ) ) ;
#54025=CARTESIAN_POINT ( 'NONE',  ( 41.82943821127123840, 26.01110640527295814, 2.839279412974134775 ) ) ;
#54029=CARTESIAN_POINT ( 'NONE',  ( 74.17344901341724039, 68.45477986254626046, -11.63824756869785659 ) ) ;
#54030=CARTESIAN_POINT ( 'NONE',  ( 74.63372018211819636, 63.10719506861975248, -14.60809168671694636 ) ) ;
#54033=CARTESIAN_POINT ( 'NONE',  ( 73.13649863228465620, 65.99558131849060771, 12.57961139238893189 ) ) ;
#54041=ORIENTED_EDGE ( 'NONE', *, *, #79193, .T. ) ;
#54046=CARTESIAN_POINT ( 'NONE',  ( 69.34600056039464278, 71.16434039272530754, -0.2959734442564417867 ) ) ;
#54048=CARTESIAN_POINT ( 'NONE',  ( 69.99185448575823898, 62.80507302648442902, -13.35615040175713375 ) ) ;
#54050=VERTEX_POINT ( 'NONE', #49483 ) ;
#54057=EDGE_CURVE ( 'NONE', #35085, #86588, #64188, .T. ) ;
#54060=CARTESIAN_POINT ( 'NONE',  ( 83.25709734292261999, 43.34571608306740842, 7.235311536896932516 ) ) ;
#54064=CARTESIAN_POINT ( 'NONE',  ( 70.39887500514583962, 61.01293241302482784, -14.92214395283775730 ) ) ;
#54065=CARTESIAN_POINT ( 'NONE',  ( 82.75425455800102270, 53.83811729049745054, -15.80404254388376550 ) ) ;
#54067=CARTESIAN_POINT ( 'NONE',  ( 73.98570270871888965, 68.92876820612470112, -11.10152750440662750 ) ) ;
#54074=CARTESIAN_POINT ( 'NONE',  ( 73.71953624722927145, 69.45002187000606853, -9.858408069665332008 ) ) ;
#54075=CARTESIAN_POINT ( 'NONE',  ( 76.60151444110638863, 51.30487137736207615, 16.06220798441930953 ) ) ;
#54086=CARTESIAN_POINT ( 'NONE',  ( 87.92795318006373861, 43.94156286934877897, 0.4729106731310683265 ) ) ;
#54091=CARTESIAN_POINT ( 'NONE',  ( 21.92109465949963720, 30.84336893147756697, -7.433330006724137462 ) ) ;
#54094=CARTESIAN_POINT ( 'NONE',  ( 10.59179830548347745, 18.06628583063839599, -9.188101187500006262 ) ) ;
#54096=CARTESIAN_POINT ( 'NONE',  ( 77.33081447068806824, 63.24619402228064047, 15.57729104808880294 ) ) ;
#54099=CARTESIAN_POINT ( 'NONE',  ( 73.78463575287290155, 65.88767259777996799, 12.89433537800410434 ) ) ;
#54102=CARTESIAN_POINT ( 'NONE',  ( 87.74379322371484591, 45.04902437494477851, -6.671288900681476619 ) ) ;
#54108=CARTESIAN_POINT ( 'NONE',  ( 82.55952364350828532, 54.17540112820317688, 15.56538284540774697 ) ) ;
#54109=VERTEX_POINT ( 'NONE', #1900 ) ;
#54112=CARTESIAN_POINT ( 'NONE',  ( 70.90260330370475117, 68.90363874238359188, -8.343585586704856283 ) ) ;
#54115=CARTESIAN_POINT ( 'NONE',  ( 66.23755376128818284, 69.21869211729334381, -2.080742945835972968 ) ) ;
#54119=CARTESIAN_POINT ( 'NONE',  ( 25.58005199048888656, 32.95586893147756768, 7.433330006724141015 ) ) ;
#54121=FACE_OUTER_BOUND ( 'NONE', #40171, .T. ) ;
#54123=CARTESIAN_POINT ( 'NONE',  ( 81.97896201599648691, 58.73259127988954731, -0.1545084971874724766 ) ) ;
#54128=CARTESIAN_POINT ( 'NONE',  ( 67.80942915694498652, 65.50210952888220106, 10.23305949600108633 ) ) ;
#54129=CARTESIAN_POINT ( 'NONE',  ( 68.10110334728497605, 66.09131973784090519, -10.53698601666638979 ) ) ;
#54139=ORIENTED_EDGE ( 'NONE', *, *, #36778, .T. ) ;
#54145=CARTESIAN_POINT ( 'NONE',  ( 66.53750495837353185, 67.82509315316526965, 6.869996715873302406 ) ) ;
#54146=CARTESIAN_POINT ( 'NONE',  ( 34.57290638322662346, 20.36477965099641452, 1.583844403245330712 ) ) ;
#54149=CARTESIAN_POINT ( 'NONE',  ( 86.27154027830852101, 42.80277227827716757, -2.586754297940185854 ) ) ;
#54151=CARTESIAN_POINT ( 'NONE',  ( 78.64512151719945621, 48.80906647027654088, -14.34982556509240403 ) ) ;
#54152=CARTESIAN_POINT ( 'NONE',  ( 70.37793518914109825, 63.81744015580922991, 12.87794577580022981 ) ) ;
#54157=VERTEX_POINT ( 'NONE', #88055 ) ;
#54159=ORIENTED_EDGE ( 'NONE', *, *, #44208, .T. ) ;
#54160=CARTESIAN_POINT ( 'NONE',  ( 83.76771450586321066, 41.67386438877598209, 0.3050775560854859791 ) ) ;
#54161=VECTOR ( 'NONE', #95315, 1000.000000000000114 ) ;
#54169=CARTESIAN_POINT ( 'NONE',  ( 28.90303340214877181, 40.18528772668521043, -1.583844403245329602 ) ) ;
#54171=CARTESIAN_POINT ( 'NONE',  ( 72.64591869506153898, 70.77312924948247996, 7.138500078990828612 ) ) ;
#54172=CARTESIAN_POINT ( 'NONE',  ( 73.53472180018071924, 66.80482608298828495, -12.17997313596818287 ) ) ;
#54186=EDGE_CURVE ( 'NONE', #85355, #38035, #22073, .T. ) ;
#54189=CARTESIAN_POINT ( 'NONE',  ( 73.91518305203547357, 55.21146187366786506, 16.12241119387309496 ) ) ;
#54192=CARTESIAN_POINT ( 'NONE',  ( 28.04762285228751395, 28.14441083166262203, 10.00000000000000533 ) ) ;
#54200=CARTESIAN_POINT ( 'NONE',  ( 72.51946054628299976, 70.67701989327743206, -7.917356521280768611 ) ) ;
#54204=CARTESIAN_POINT ( 'NONE',  ( 75.37843707191281339, 53.50823561223473490, 16.04097401286667335 ) ) ;
#54206=CARTESIAN_POINT ( 'NONE',  ( 27.78891098193510345, 37.81751292744058190, -6.180339887498951690 ) ) ;
#54207=CARTESIAN_POINT ( 'NONE',  ( 77.40556785558190711, 54.71814905221435055, 16.53596348862507881 ) ) ;
#54214=DIRECTION ( 'NONE',  ( 0.4972609476841349796, -0.8612812260087746585, 0.1045284632676570652 ) ) ;
#54217=CARTESIAN_POINT ( 'NONE',  ( 66.63481606961637738, 67.83260985918037989, 6.962306014892454264 ) ) ;
#54227=CARTESIAN_POINT ( 'NONE',  ( 16.80975711337266176, 31.74646525600390135, 2.839279412974139660 ) ) ;
#54228=CARTESIAN_POINT ( 'NONE',  ( 9.459751770947381289, 21.16454794089040092, -10.00000000000000355 ) ) ;
#54233=CARTESIAN_POINT ( 'NONE',  ( 76.68960682072659552, 58.66400703976827202, -16.06550202522544168 ) ) ;
#54234=CARTESIAN_POINT ( 'NONE',  ( 81.26997250612254220, 42.40853988048920087, 7.543452372214260571 ) ) ;
#54236=CARTESIAN_POINT ( 'NONE',  ( 72.63217277574858599, 71.42405857463968744, -5.808642681096034543 ) ) ;
#54237=CARTESIAN_POINT ( 'NONE',  ( 22.08843299157899764, 31.49103043416549852, -8.090169943749479842 ) ) ;
#54241=CARTESIAN_POINT ( 'NONE',  ( 83.82495796739634386, 42.53198561061005734, -4.832817608612280047 ) ) ;
#54257=CARTESIAN_POINT ( 'NONE',  ( 30.03287232231581072, 25.84335787977764554, 9.188101187500006262 ) ) ;
#54259=CARTESIAN_POINT ( 'NONE',  ( 78.26456671038654633, 47.45118235465228196, -13.78252656109451380 ) ) ;
#54261=EDGE_CURVE ( 'NONE', #36219, #13677, #100058, .T. ) ;
#54267=ORIENTED_EDGE ( 'NONE', *, *, #89319, .F. ) ;
#54270=CARTESIAN_POINT ( 'NONE',  ( 87.10930705799060547, 46.39120889860887331, 8.709784027055659905 ) ) ;
#54280=CARTESIAN_POINT ( 'NONE',  ( 71.66380185985713069, 70.75815305948317757, 6.002177236114092373 ) ) ;
#54282=CARTESIAN_POINT ( 'NONE',  ( 67.68246526915767447, 66.80505248408825025, 8.573265321495291857 ) ) ;
#54284=CARTESIAN_POINT ( 'NONE',  ( 77.94364930070486253, 48.08271769344008817, 14.18973355224276212 ) ) ;
#54288=CARTESIAN_POINT ( 'NONE',  ( 83.97040189252935249, 41.78422930658946655, -0.6732071361253898489 ) ) ;
#54292=FACE_OUTER_BOUND ( 'NONE', #26905, .T. ) ;
#54293=CARTESIAN_POINT ( 'NONE',  ( 83.79462322672901564, 52.11981396736175043, -14.61821130395286872 ) ) ;
#54294=CARTESIAN_POINT ( 'NONE',  ( 68.48117590867735771, 65.15193093079356856, -10.98008167408246649 ) ) ;
#54297=( BOUNDED_CURVE ( )  B_SPLINE_CURVE ( 2, ( #71328, #17100, #79456, #95158, #87080, #77922, #78428, #38897, #23688, #70300, #54583, #15590, #63207 ),
 .UNSPECIFIED., .F., .T. ) 
 B_SPLINE_CURVE_WITH_KNOTS ( ( 3, 2, 2, 2, 2, 2, 3 ),
 ( 0.03750000000000000555, 0.04000000000000000083, 0.04499999999999999833, 0.05000000000000000278, 0.05500000000000000028, 0.05999999999999999778, 0.06250000000000000000 ),
 .UNSPECIFIED. ) 
 CURVE ( )  GEOMETRIC_REPRESENTATION_ITEM ( )  RATIONAL_B_SPLINE_CURVE ( ( 0.9755282581475768211, 0.9755282581475768211, 1.000000000000000000, 0.9510565162951535312, 1.000000000000000000, 0.9510565162951535312, 1.000000000000000000, 0.9510565162951535312, 1.000000000000000000, 0.9510565162951535312, 1.000000000000000000, 0.9755282581475768211, 0.9755282581475768211 ) ) 
 REPRESENTATION_ITEM ( '' )  );
#54299=CARTESIAN_POINT ( 'NONE',  ( 72.19696248574352637, 71.49523067816146238, 5.038491395661391259 ) ) ;
#54307=CARTESIAN_POINT ( 'NONE',  ( 85.72318707267324100, 48.45004672980276439, -11.74706068800014513 ) ) ;
#54308=VERTEX_POINT ( 'NONE', #84408 ) ;
#54309=CARTESIAN_POINT ( 'NONE',  ( 70.84135035934207281, 62.78096507068896415, 13.67032215614803370 ) ) ;
#54321=CARTESIAN_POINT ( 'NONE',  ( 20.76088743254790003, 12.39040679176982529, 1.333680081654574804E-15 ) ) ;
#54322=ADVANCED_FACE ( 'NONE', ( #15960 ), #63064, .T. ) ;
#54325=CARTESIAN_POINT ( 'NONE',  ( 15.99984526765731907, 17.43677371833800649, -10.00000000000000355 ) ) ;
#54332=CARTESIAN_POINT ( 'NONE',  ( 73.10143609569175283, 57.30672121060334945, 15.89779801809523896 ) ) ;
#54333=CARTESIAN_POINT ( 'NONE',  ( 71.48351530877290827, 69.86829643969724657, 8.246344044914554416 ) ) ;
#54334=CARTESIAN_POINT ( 'NONE',  ( 13.59582392308679033, 19.80066082961420548, 10.00000000000000533 ) ) ;
#54340=CARTESIAN_POINT ( 'NONE',  ( 28.71100085020356474, 39.68290643055189548, 3.479690158560446702E-15 ) ) ;
#54346=CARTESIAN_POINT ( 'NONE',  ( 66.48422118441082773, 68.76807364154430502, 2.317831917423630816 ) ) ;
#54351=CARTESIAN_POINT ( 'NONE',  ( 10.26584248093601737, 14.43085787977761036, -9.188101187500008038 ) ) ;
#54359=CARTESIAN_POINT ( 'NONE',  ( 73.76584831522595209, 68.38082682530665579, 10.99424229391075514 ) ) ;
#54368=CARTESIAN_POINT ( 'NONE',  ( 87.27117856089937220, 44.98890866680353895, -6.231534082530021834 ) ) ;
#54371=CARTESIAN_POINT ( 'NONE',  ( 79.31081143133005185, 59.61002059306027689, -16.52811874246032886 ) ) ;
#54373=CARTESIAN_POINT ( 'NONE',  ( 70.01938104327861367, 62.76876530535373178, 13.38671266457854792 ) ) ;
#54384=EDGE_CURVE ( 'NONE', #27648, #36202, #91523, .T. ) ;
#54385=CARTESIAN_POINT ( 'NONE',  ( 70.12552833076205161, 70.75604929650035047, 3.338328085167999060 ) ) ;
#54388=CARTESIAN_POINT ( 'NONE',  ( 81.62619352285597074, 44.78313946143589419, 10.36055733450182537 ) ) ;
#54393=CARTESIAN_POINT ( 'NONE',  ( 82.87565756262195293, 53.54239330764043814, -15.33588095777717086 ) ) ;
#54397=CARTESIAN_POINT ( 'NONE',  ( 11.20403028766721398, 24.65586893147754921, -7.433330006724137462 ) ) ;
#54398=VECTOR ( 'NONE', #79792, 1000.000000000000114 ) ;
#54400=CARTESIAN_POINT ( 'NONE',  ( 80.31556117237309422, 57.81632953744806969, 16.60139635717627726 ) ) ;
#54402=ORIENTED_EDGE ( 'NONE', *, *, #55837, .F. ) ;
#54433=DIRECTION ( 'NONE',  ( 0.8660254037844377084, 0.5000000000000015543, -0.000000000000000000 ) ) ;
#54437=ORIENTED_EDGE ( 'NONE', *, *, #18434, .T. ) ;
#54442=CARTESIAN_POINT ( 'NONE',  ( 80.45486823626444561, 57.11063749423583147, -16.22959712110212749 ) ) ;
#54450=CARTESIAN_POINT ( 'NONE',  ( 68.14689968819119770, 67.57311714285278015, 7.858381336759803659 ) ) ;
#54454=CARTESIAN_POINT ( 'NONE',  ( 81.93667712306067585, 41.32900906425540200, -5.893600489608231463 ) ) ;
#54457=CARTESIAN_POINT ( 'NONE',  ( 17.70402515066951565, 13.14754757982089295, -5.678558825948276656 ) ) ;
#54460=DIRECTION ( 'NONE',  ( 0.5000000000000013323, -0.8660254037844378194, 0.000000000000000000 ) ) ;
#54461=CARTESIAN_POINT ( 'NONE',  ( 8.802591199716557568, 28.58029201028040589, 1.583844403245363353 ) ) ;
#54469=CARTESIAN_POINT ( 'NONE',  ( 67.15292568697987008, 69.89524710907804206, 0.3341031261128851182 ) ) ;
#54474=CARTESIAN_POINT ( 'NONE',  ( 81.05125564046635134, 47.50520864145833855, 13.45574471257056359 ) ) ;
#54478=CARTESIAN_POINT ( 'NONE',  ( 75.75917444283010127, 65.12044684595205979, -14.46054081031674876 ) ) ;
#54486=CARTESIAN_POINT ( 'NONE',  ( 37.11382629638189457, 33.37878583063844218, 9.188101187500006262 ) ) ;
#54490=VERTEX_POINT ( 'NONE', #83739 ) ;
#54495=CYLINDRICAL_SURFACE ( 'NONE', #38854, 16.60714546451156792 ) ;
#54497=CARTESIAN_POINT ( 'NONE',  ( 80.29271997359656154, 44.85105216242119042, 11.15187779989279093 ) ) ;
#54498=CARTESIAN_POINT ( 'NONE',  ( 84.88427240234526039, 50.06337035240281352, -13.24819347122077851 ) ) ;
#54499=CARTESIAN_POINT ( 'NONE',  ( 81.36199125831662116, 55.41608345602817565, -16.32668456146280889 ) ) ;
#54502=ORIENTED_EDGE ( 'NONE', *, *, #69283, .T. ) ;
#54503=CARTESIAN_POINT ( 'NONE',  ( 81.29827136372979624, 55.78681482234479461, 16.38844377500790017 ) ) ;
#54517=CARTESIAN_POINT ( 'NONE',  ( 70.56938734894262666, 60.79602815012135864, -14.52576355119476581 ) ) ;
#54526=CARTESIAN_POINT ( 'NONE',  ( 72.42579240007300712, 63.30198422945165504, 13.90833229552876738 ) ) ;
#54534=CARTESIAN_POINT ( 'NONE',  ( 65.97662824784276836, 68.66983059223240105, -0.2190663313023521186 ) ) ;
#54536=FACE_OUTER_BOUND ( 'NONE', #94675, .T. ) ;
#54543=CARTESIAN_POINT ( 'NONE',  ( 69.85780038398088720, 62.79618712063587793, -13.31498138799742570 ) ) ;
#54557=CARTESIAN_POINT ( 'NONE',  ( 82.35285118013293015, 53.50770157854819331, -15.77620284334257938 ) ) ;
#54559=CARTESIAN_POINT ( 'NONE',  ( 70.70420039156243774, 71.94848598797803163, 6.061257734329015641E-06 ) ) ;
#54563=EDGE_CURVE ( 'NONE', #94602, #8880, #42179, .T. ) ;
#54566=VECTOR ( 'NONE', #39587, 1000.000000000000000 ) ;
#54567=CARTESIAN_POINT ( 'NONE',  ( 78.08841283195533833, 61.93109719521473977, 15.70046319500454857 ) ) ;
#54568=CARTESIAN_POINT ( 'NONE',  ( 73.14143739346300777, 69.59972439283021117, -9.872010100564622803 ) ) ;
#54569=CARTESIAN_POINT ( 'NONE',  ( 75.96574207184018235, 51.41514783579079761, 15.67647344538899645 ) ) ;
#54582=CARTESIAN_POINT ( 'NONE',  ( 88.54102397196729157, 43.89880672352619229, -0.3772737106920460159 ) ) ;
#54583=CARTESIAN_POINT ( 'NONE',  ( 4.856824484202590497, 25.73705186507751819, -3.090169943749475845 ) ) ;
#54589=CARTESIAN_POINT ( 'NONE',  ( 31.56043161122053320, 21.14754757982091249, -5.678558825948275768 ) ) ;
#54592=CARTESIAN_POINT ( 'NONE',  ( 10.91775413003093931, 21.70171378149917985, -9.188101187500004485 ) ) ;
#54594=CARTESIAN_POINT ( 'NONE',  ( 77.31919379202844311, 63.29706486701976331, 15.55867855103717545 ) ) ;
#54600=CARTESIAN_POINT ( 'NONE',  ( 75.25638032370783037, 56.77384408695551343, -16.10482308988691358 ) ) ;
#54606=CIRCLE ( 'NONE', #10987, 15.60714546451148799 ) ;
#54607=CARTESIAN_POINT ( 'NONE',  ( 82.08557581956762306, 54.06085729471828927, 15.60977446998290574 ) ) ;
#54612=VERTEX_POINT ( 'NONE', #24396 ) ;
#54621=CARTESIAN_POINT ( 'NONE',  ( 21.45803809350889324, 35.49540643055188127, 3.479690158560446702E-15 ) ) ;
#54623=CARTESIAN_POINT ( 'NONE',  ( 84.65437100661064562, 50.51450566574431633, -13.57843829959869808 ) ) ;
#54632=CARTESIAN_POINT ( 'NONE',  ( 67.63975743122908568, 65.85389184688227715, 10.50638905972799719 ) ) ;
#54633=CARTESIAN_POINT ( 'NONE',  ( 67.78035058596742601, 65.61037735967913420, -10.84149385423511802 ) ) ;
#54653=CARTESIAN_POINT ( 'NONE',  ( 66.82165646262005509, 67.51089840573428091, 6.628743624060557060 ) ) ;
#54665=CARTESIAN_POINT ( 'NONE',  ( 76.00688113039353766, 65.27918228371470377, -14.45284717766215721 ) ) ;
#54670=CARTESIAN_POINT ( 'NONE',  ( 84.97959890569808294, 43.76174631704970608, -6.205910672392634275 ) ) ;
#54671=CARTESIAN_POINT ( 'NONE',  ( 43.23316042107100543, 25.36477965099643583, 1.583844403245330712 ) ) ;
#54674=CARTESIAN_POINT ( 'NONE',  ( 72.54292141210436284, 70.69116050516647931, 7.176139523292191846 ) ) ;
#54675=CARTESIAN_POINT ( 'NONE',  ( 73.11768136168076637, 66.90819131663745623, -11.89771565002191345 ) ) ;
#54681=CARTESIAN_POINT ( 'NONE',  ( 83.58343668721781228, 51.99607003748921130, 15.00733587213922604 ) ) ;
#54691=CARTESIAN_POINT ( 'NONE',  ( 73.80173605198457665, 55.24307582110920833, 16.12032811712526481 ) ) ;
#54694=CARTESIAN_POINT ( 'NONE',  ( 26.14792707536646432, 33.83478043621389020, -8.090169943749479842 ) ) ;
#54702=CARTESIAN_POINT ( 'NONE',  ( 70.96429761875693032, 61.15374941679502996, 14.99935025239130226 ) ) ;
#54710=CARTESIAN_POINT ( 'NONE',  ( 27.45223038363779722, 27.80066082961423035, 10.00000000000000533 ) ) ;
#54711=CARTESIAN_POINT ( 'NONE',  ( 33.32035334334607057, 27.43677371833803846, -10.00000000000000355 ) ) ;
#54712=CARTESIAN_POINT ( 'NONE',  ( 84.83247989926988453, 42.35328799155462320, -1.743318450112538942 ) ) ;
#54714=LINE ( 'NONE', #47623, #57293 ) ;
#54719=EDGE_CURVE ( 'NONE', #25562, #79014, #55160, .T. ) ;
#54721=FACE_OUTER_BOUND ( 'NONE', #92456, .T. ) ;
#54725=CARTESIAN_POINT ( 'NONE',  ( 66.97748580466556234, 68.05911003901715617, 6.908000617270682042 ) ) ;
#54733=CARTESIAN_POINT ( 'NONE',  ( 20.98529944902502820, 27.51421378149918695, -9.188101187500004485 ) ) ;
#54738=CARTESIAN_POINT ( 'NONE',  ( 9.991594722369004700, 23.95586893147753926, 7.433330006724141015 ) ) ;
#54740=CARTESIAN_POINT ( 'NONE',  ( 75.20199238159069921, 59.20172555882615484, -15.83912561188805590 ) ) ;
#54745=CARTESIAN_POINT ( 'NONE',  ( 72.52145085236621469, 71.52933981707218436, -5.380113948530985013 ) ) ;
#54747=LINE ( 'NONE', #85210, #46850 ) ;
#54748=ORIENTED_EDGE ( 'NONE', *, *, #57167, .T. ) ;
#54752=CARTESIAN_POINT ( 'NONE',  ( 85.89759834047637810, 43.04820835652777333, -2.464790169128945774 ) ) ;
#54756=CARTESIAN_POINT ( 'NONE',  ( 72.08021828965947009, 72.40975849880194914, -3.082927075499598324 ) ) ;
#54757=CARTESIAN_POINT ( 'NONE',  ( 72.82235704132158105, 56.84590537091418128, -15.94416503159311027 ) ) ;
#54758=CARTESIAN_POINT ( 'NONE',  ( 76.88601853014658616, 63.69663891124154276, 15.33692311465240543 ) ) ;
#54761=AXIS2_PLACEMENT_3D ( 'NONE', #84090, #44015, #14140 ) ;
#54773=CARTESIAN_POINT ( 'NONE',  ( 31.05164846989082506, 29.87878583063843507, -9.188101187500006262 ) ) ;
#54778=ORIENTED_EDGE ( 'NONE', *, *, #62450, .T. ) ;
#54783=VERTEX_POINT ( 'NONE', #73387 ) ;
#54786=CARTESIAN_POINT ( 'NONE',  ( 87.13645712923818110, 46.25687745756817293, 8.491008164162357374 ) ) ;
#54796=B_SPLINE_CURVE_WITH_KNOTS ( 'NONE', 3,
 ( #77112, #30519, #22909, #75147, #127, #38095, #52808, #67520, #98450, #5725, #59912, #30016, #99936, #69006, #68022, #61408 ),
 .UNSPECIFIED., .F., .F.,
 ( 4, 1, 2, 2, 2, 1, 2, 2, 4 ),
 ( 0.000000000000000000, 0.1250000000000056344, 0.1875000000000079103, 0.2500000000000102141, 0.5000000000000087708, 0.6250000000000062172, 0.6875000000000045519, 0.7500000000000028866, 1.000000000000000000 ),
 .UNSPECIFIED. ) ;
#54798=AXIS2_PLACEMENT_3D ( 'NONE', #45561, #30377, #91212 ) ;
#54801=CARTESIAN_POINT ( 'NONE',  ( 77.00910850481051284, 63.69207575539577704, -14.97815254220547487 ) ) ;
#54802=CARTESIAN_POINT ( 'NONE',  ( 78.56719005003022005, 47.98515344134878546, 13.96283253221395881 ) ) ;
#54806=CARTESIAN_POINT ( 'NONE',  ( 82.96321432696582576, 41.33265327218170171, -1.885893662060450060 ) ) ;
#54807=CARTESIAN_POINT ( 'NONE',  ( 87.78256729009754622, 45.12882416216076820, -6.783508070075447982 ) ) ;
#54810=CARTESIAN_POINT ( 'NONE',  ( 83.69613447051490596, 51.47860253839341738, -14.37487551769288352 ) ) ;
#54812=ORIENTED_EDGE ( 'NONE', *, *, #5762, .T. ) ;
#54814=CARTESIAN_POINT ( 'NONE',  ( 72.35414581608256412, 71.76618622507949397, 5.628474724962970299 ) ) ;
#54823=CARTESIAN_POINT ( 'NONE',  ( 72.39118694979968893, 67.66586127011399299, 10.85488035418265085 ) ) ;
#54825=DIRECTION ( 'NONE',  ( 0.8660254037844379305, 0.5000000000000014433, 0.000000000000000000 ) ) ;
#54831=CARTESIAN_POINT ( 'NONE',  ( 45.60499120716188060, 26.73415679381826138, -6.890680421881970419E-14 ) ) ;
#54834=VECTOR ( 'NONE', #87337, 1000.000000000000114 ) ;
#54836=CARTESIAN_POINT ( 'NONE',  ( 87.97974684949012669, 44.79880412219662844, 4.785089242980530955 ) ) ;
#54840=CARTESIAN_POINT ( 'NONE',  ( 15.49551970000783996, 14.11029122506293021, -8.090169943749478065 ) ) ;
#54841=CARTESIAN_POINT ( 'NONE',  ( 81.90250264543212211, 49.37766992099674468, -14.25890439565079681 ) ) ;
#54842=CARTESIAN_POINT ( 'NONE',  ( 71.86082717042363299, 59.56791737868546477, -15.73637609511307289 ) ) ;
#54843=CARTESIAN_POINT ( 'NONE',  ( 74.04309036720468384, 54.83868394417908831, -16.13477068996618513 ) ) ;
#54847=CARTESIAN_POINT ( 'NONE',  ( 10.89475974595093000, 11.45404122711131478, -8.090169943749478065 ) ) ;
#54851=CARTESIAN_POINT ( 'NONE',  ( 11.88462290154380874, 22.56454794089039950, 10.00000000000000355 ) ) ;
#54853=ADVANCED_FACE ( 'NONE', ( #72404 ), #20187, .T. ) ;
#54860=CARTESIAN_POINT ( 'NONE',  ( 35.77386594998528579, 21.44966523072496756, -2.296566073217252530E-15 ) ) ;
#54865=CARTESIAN_POINT ( 'NONE',  ( 66.53410914940803877, 68.80543330372941568, 2.269385016797728305 ) ) ;
#54870=CARTESIAN_POINT ( 'NONE',  ( 9.185703322462064335, 20.70171378149917274, -9.188101187500004485 ) ) ;
#54873=CARTESIAN_POINT ( 'NONE',  ( 88.27455224169976589, 44.26958888746147380, -1.928006731073693469 ) ) ;
#54875=DIRECTION ( 'NONE',  ( -0.8660254037844378194, -0.5000000000000013323, -0.000000000000000000 ) ) ;
#54880=ORIENTED_EDGE ( 'NONE', *, *, #45815, .T. ) ;
#54884=CARTESIAN_POINT ( 'NONE',  ( 72.77371579809937430, 70.82568240960111439, 7.174012581183236925 ) ) ;
#54886=CARTESIAN_POINT ( 'NONE',  ( 70.07366985589914066, 68.21750869337182621, 9.404999606781979438 ) ) ;
#54888=VERTEX_POINT ( 'NONE', #80521 ) ;
#54889=CARTESIAN_POINT ( 'NONE',  ( 68.69988281822412546, 63.95555916913097150, -12.08471377653384771 ) ) ;
#54890=CARTESIAN_POINT ( 'NONE',  ( 79.42902015582541253, 59.13724458665812023, -16.22739499525147266 ) ) ;
#54891=EDGE_CURVE ( 'NONE', #41027, #50534, #83652, .T. ) ;
#54893=CARTESIAN_POINT ( 'NONE',  ( 69.50649804366692308, 62.68264628211643696, 13.83822202275866786 ) ) ;
#54894=ORIENTED_EDGE ( 'NONE', *, *, #57248, .F. ) ;
#54902=VERTEX_POINT ( 'NONE', #68751 ) ;
#54905=CARTESIAN_POINT ( 'NONE',  ( 71.12899601204873079, 71.68446395904118162, 1.608505432448458894 ) ) ;
#54906=ORIENTED_EDGE ( 'NONE', *, *, #10419, .F. ) ;
#54909=CARTESIAN_POINT ( 'NONE',  ( 82.76870359366968444, 47.59112932736264412, 12.29198334313100105 ) ) ;
#54914=CARTESIAN_POINT ( 'NONE',  ( 82.48332016352127027, 53.47388482021811740, -15.74481631320922048 ) ) ;
#54917=CARTESIAN_POINT ( 'NONE',  ( 19.94606896448370392, 26.91421378149918553, 9.188101187500008038 ) ) ;
#54926=CARTESIAN_POINT ( 'NONE',  ( 69.95523204135938045, 62.90150226501648234, 13.86126985460704297 ) ) ;
#54927=CARTESIAN_POINT ( 'NONE',  ( 84.79359905062281655, 45.64121975909452544, -9.352143619951702291 ) ) ;
#54933=CARTESIAN_POINT ( 'NONE',  ( 74.87331927037790535, 66.80950769484920215, -13.20416362156882784 ) ) ;
#54942=CARTESIAN_POINT ( 'NONE',  ( 75.60565924420463091, 65.54105765176767306, 13.80443174476947732 ) ) ;
#54947=DIRECTION ( 'NONE',  ( 0.2588190451024995897, 0.9659258262890739744, 0.000000000000000000 ) ) ;
#54949=CARTESIAN_POINT ( 'NONE',  ( 81.89789973039891890, 46.67758023279904478, -11.97137090468010356 ) ) ;
#54950=CARTESIAN_POINT ( 'NONE',  ( 22.61461015039527922, 36.55466486950700755, 7.012934429366973338E-14 ) ) ;
#54953=CARTESIAN_POINT ( 'NONE',  ( 74.09829895435802882, 68.37032454858436381, -11.67432565205426620 ) ) ;
#54955=DIRECTION ( 'NONE',  ( -0.5778974349098193741, -0.4186690413702516822, -0.7005360722495063142 ) ) ;
#54957=DIRECTION ( 'NONE',  ( -0.06958655048002569676, 0.1205274409548614395, -0.9902680687415721383 ) ) ;
#54959=CARTESIAN_POINT ( 'NONE',  ( 29.54281338067077911, 40.55466486950702176, -1.111400068045478839E-16 ) ) ;
#54974=CARTESIAN_POINT ( 'NONE',  ( 75.35150063214643978, 63.77177416529143983, 14.96501676786058255 ) ) ;
#54978=CARTESIAN_POINT ( 'NONE',  ( 19.43607595823839418, 14.14754757982089473, -5.678558825948276656 ) ) ;
#54984=CARTESIAN_POINT ( 'NONE',  ( 30.01653393904200584, 17.73415679381823296, -6.890680421881970419E-14 ) ) ;
#54985=DIRECTION ( 'NONE',  ( -0.9364604334398972663, 0.2023802897980892801, 0.2865031848039413243 ) ) ;
#54992=CARTESIAN_POINT ( 'NONE',  ( 82.04273294443818543, 51.69458978218974465, 15.23912461881878677 ) ) ;
#54996=VECTOR ( 'NONE', #84650, 1000.000000000000114 ) ;
#55000=CARTESIAN_POINT ( 'NONE',  ( 73.57121657643290291, 69.82745460598127352, 9.896087309288359890 ) ) ;
#55002=CARTESIAN_POINT ( 'NONE',  ( 34.13026518906141860, 41.74646525600392977, 2.839279412974139660 ) ) ;
#55006=CARTESIAN_POINT ( 'NONE',  ( 86.74085627840248947, 44.04483152046088179, -5.761820014970100878 ) ) ;
#55008=CARTESIAN_POINT ( 'NONE',  ( 86.50129422937833112, 47.15573905589064196, -10.08535824937341374 ) ) ;
#55011=CARTESIAN_POINT ( 'NONE',  ( 84.95458848507411176, 44.42387911948991075, -8.356648915091495766 ) ) ;
#55012=CARTESIAN_POINT ( 'NONE',  ( 84.43319883474627829, 44.99437554259058913, -9.553074584682860859 ) ) ;
#55016=CARTESIAN_POINT ( 'NONE',  ( 87.10115137904762150, 45.28340438443854055, 6.995308688534716879 ) ) ;
#55018=CARTESIAN_POINT ( 'NONE',  ( 77.16396432587895049, 49.58440764469271045, -14.97671560787508405 ) ) ;
#55019=ORIENTED_EDGE ( 'NONE', *, *, #16168, .F. ) ;
#55020=CARTESIAN_POINT ( 'NONE',  ( 87.20555836939593064, 45.98127448902955905, -8.722945138008007859 ) ) ;
#55021=CARTESIAN_POINT ( 'NONE',  ( 78.65113419757746271, 50.64782171794184507, 15.07795987699981666 ) ) ;
#55026=CARTESIAN_POINT ( 'NONE',  ( 69.81243019392553606, 62.22010195957141576, -13.63492759933605392 ) ) ;
#55027=CARTESIAN_POINT ( 'NONE',  ( 82.24318726465129714, 40.84802034143084626, 1.047704164177056585 ) ) ;
#55032=CARTESIAN_POINT ( 'NONE',  ( 70.58053732654904877, 60.72247144732425994, -14.55979615259335169 ) ) ;
#55033=CARTESIAN_POINT ( 'NONE',  ( 35.53452623260358223, 35.91421378149921395, 9.188101187500008038 ) ) ;
#55043=CARTESIAN_POINT ( 'NONE',  ( 80.71386657632071149, 43.15011696034207489, 9.894852039748123218 ) ) ;
#55047=ORIENTED_EDGE ( 'NONE', *, *, #5707, .T. ) ;
#55051=CARTESIAN_POINT ( 'NONE',  ( 81.94845728006144725, 58.78542703240049150, -0.2795964517353725087 ) ) ;
#55063=CARTESIAN_POINT ( 'NONE',  ( 84.80172950927561715, 50.19486025153374698, 13.34007759942641336 ) ) ;
#55066=CARTESIAN_POINT ( 'NONE',  ( 74.24116255903008721, 68.58322516222325760, 11.55893809163644725 ) ) ;
#55068=CARTESIAN_POINT ( 'NONE',  ( 74.13561708490506419, 68.62084109673111243, 10.97025690930964892 ) ) ;
#55078=CARTESIAN_POINT ( 'NONE',  ( 78.31072776954091808, 61.54348912244275027, 15.80414048699106999 ) ) ;
#55080=CARTESIAN_POINT ( 'NONE',  ( 76.35565666213805969, 51.40178206308662823, 15.62279043926746347 ) ) ;
#55084=EDGE_CURVE ( 'NONE', #81557, #36092, #80713, .T. ) ;
#55092=CARTESIAN_POINT ( 'NONE',  ( 88.42339661562220954, 43.82656006556687345, 0.1181016345699151954 ) ) ;
#55095=CARTESIAN_POINT ( 'NONE',  ( 71.99279863978298977, 71.74937481526245620, -3.912420615770861865 ) ) ;
#55096=CARTESIAN_POINT ( 'NONE',  ( 70.17810782877538145, 70.93619788462370934, -4.492011057286514841 ) ) ;
#55098=CARTESIAN_POINT ( 'NONE',  ( 28.77833178495667710, 28.56628583063842441, 9.188101187500006262 ) ) ;
#55101=CARTESIAN_POINT ( 'NONE',  ( 9.725772901699041739, 17.56628583063838889, 9.188101187500006262 ) ) ;
#55103=CARTESIAN_POINT ( 'NONE',  ( 76.70245435708865500, 63.85979508024991702, 14.86777658481231867 ) ) ;
#55106=CARTESIAN_POINT ( 'NONE',  ( 69.38743239535708085, 62.82953552710814193, -13.71264069967795329 ) ) ;
#55112=CARTESIAN_POINT ( 'NONE',  ( 77.17192383615090989, 49.30585512036960694, 15.39194763320842441 ) ) ;
#55117=CARTESIAN_POINT ( 'NONE',  ( 71.40939848415580116, 68.88699701054706281, -8.787086014537564438 ) ) ;
#55121=CARTESIAN_POINT ( 'NONE',  ( 72.46511837996447980, 71.56249752072032777, 6.234640293157904800 ) ) ;
#55125=CARTESIAN_POINT ( 'NONE',  ( 30.72569264534336142, 26.24335787977765122, -9.188101187500008038 ) ) ;
#55127=CARTESIAN_POINT ( 'NONE',  ( 74.84872400778056090, 66.80276697526576868, -13.19923776164384677 ) ) ;
#55134=CARTESIAN_POINT ( 'NONE',  ( 68.07556148176628597, 65.74332760699670075, 10.87905400252346588 ) ) ;
#55135=CARTESIAN_POINT ( 'NONE',  ( 68.04520307338094653, 65.58168358224989447, -10.28824799336666374 ) ) ;
#55139=CARTESIAN_POINT ( 'NONE',  ( 69.93330931759959412, 71.50341667604121199, 8.155205941333377477E-06 ) ) ;
#55142=CARTESIAN_POINT ( 'NONE',  ( 69.81582973455007846, 63.14295414310246457, -13.67321376818635059 ) ) ;
#55145=ORIENTED_EDGE ( 'NONE', *, *, #92202, .T. ) ;
#55148=EDGE_CURVE ( 'NONE', #43596, #17546, #78154, .T. ) ;
#55152=CARTESIAN_POINT ( 'NONE',  ( 79.90892646165700341, 44.66511174005920992, -11.18539793377209257 ) ) ;
#55156=CARTESIAN_POINT ( 'NONE',  ( 83.36082971782188622, 47.63437754184118944, -12.10617920438150463 ) ) ;
#55160=B_SPLINE_CURVE_WITH_KNOTS ( 'NONE', 3,
 ( #99793, #21779, #7073, #91718, #46056, #54152, #15666, #77495, #76972, #61265, #13690, #98810, #68375, #69376, #51061, #83625, #8088, #44564, #60260, #29391, #52171, #6592, #30879, #69869, #14190, #53181, #92234, #45075, #7575, #22785, #21297, #75499, #76014, #61766, #92713, #23263, #37466, #99300, #59771, #53662, #85114, #6083, #84136, #36976, #28894, #29880 ),
 .UNSPECIFIED., .F., .F.,
 ( 4, 1, 1, 1, 2, 2, 1, 1, 1, 2, 2, 1, 1, 2, 2, 1, 1, 2, 2, 1, 1, 2, 2, 1, 2, 2, 1, 2, 2, 4 ),
 ( 0.000000000000000000, 0.06249999999998717692, 0.09374999999998123723, 0.1093749999999801131, 0.1171874999999796552, 0.1249999999999792111, 0.1874999999999961142, 0.2187500000000023037, 0.2343750000000030809, 0.2421875000000033862, 0.2500000000000036637, 0.3125000000000207057, 0.3437500000000268119, 0.3593750000000282552, 0.3750000000000296430, 0.4375000000000286993, 0.4687500000000277001, 0.4843750000000258127, 0.5000000000000238698, 0.5625000000000197620, 0.5937500000000172085, 0.6093750000000150990, 0.6250000000000129896, 0.6875000000000106581, 0.7187500000000082157, 0.7500000000000056621, 0.8125000000000015543, 0.8437500000000018874, 0.8750000000000021094, 1.000000000000000000 ),
 .UNSPECIFIED. ) ;
#55166=LINE ( 'NONE', #3388, #62869 ) ;
#55168=CARTESIAN_POINT ( 'NONE',  ( 20.07045957425421179, 33.36126292948895866, 6.180339887498949913 ) ) ;
#55171=CARTESIAN_POINT ( 'NONE',  ( 88.02768100692024689, 44.78812371456486119, 4.666884733071423597 ) ) ;
#55179=CARTESIAN_POINT ( 'NONE',  ( 73.07159975088246995, 72.16059528448882077, 0.000000000000000000 ) ) ;
#55184=DIRECTION ( 'NONE',  ( -0.8660254037844377084, -0.5000000000000014433, -0.000000000000000000 ) ) ;
#55186=CARTESIAN_POINT ( 'NONE',  ( 83.34567255814403097, 52.40788958926237484, 14.85282737495174565 ) ) ;
#55189=LINE ( 'NONE', #62287, #1357 ) ;
#55192=CARTESIAN_POINT ( 'NONE',  ( 73.60674897234599712, 55.48729869333283204, 16.10905085971090145 ) ) ;
#55195=CARTESIAN_POINT ( 'NONE',  ( 28.91364825607195144, 28.64441083166262203, -10.00000000000000533 ) ) ;
#55198=AXIS2_PLACEMENT_3D ( 'NONE', #38576, #15775, #69483 ) ;
#55208=CARTESIAN_POINT ( 'NONE',  ( 81.62374368218520715, 41.76230689378203209, 5.959470817902195350 ) ) ;
#55210=CYLINDRICAL_SURFACE ( 'NONE', #18410, 16.60714546451156792 ) ;
#55211=CARTESIAN_POINT ( 'NONE',  ( 32.62753302031853053, 27.03677371833804344, 10.00000000000000533 ) ) ;
#55212=CARTESIAN_POINT ( 'NONE',  ( 86.04792660047165498, 42.90958022930985294, -0.1400070824457408381 ) ) ;
#55214=CARTESIAN_POINT ( 'NONE',  ( 81.37941775519415444, 56.13859199581248305, 16.08349135110547579 ) ) ;
#55215=CARTESIAN_POINT ( 'NONE',  ( 87.06060708477828314, 46.38825358833559420, -8.733779054531098041 ) ) ;
#55219=CARTESIAN_POINT ( 'NONE',  ( 73.62564376992710891, 66.16305478508047599, -12.64589907936473701 ) ) ;
#55229=CARTESIAN_POINT ( 'NONE',  ( 19.86428432551159418, 29.65586893147756342, -7.433330006724137462 ) ) ;
#55234=CARTESIAN_POINT ( 'NONE',  ( 14.00658445089738180, 13.80170272979924917, 7.433330006724137462 ) ) ;
#55238=CARTESIAN_POINT ( 'NONE',  ( 78.70532132115687318, 57.84908500555658861, -16.23223772817032895 ) ) ;
#55239=CARTESIAN_POINT ( 'NONE',  ( 71.56491451745446852, 72.38511813685279606, -1.315970478074329764 ) ) ;
#55244=DIRECTION ( 'NONE',  ( 0.4924038765061026779, -0.8528685319524446085, -0.1736481776669273058 ) ) ;
#55245=ORIENTED_EDGE ( 'NONE', *, *, #12679, .F. ) ;
#55248=CARTESIAN_POINT ( 'NONE',  ( 85.10720402821901587, 42.81679804039411152, -3.423875221259823132 ) ) ;
#55251=CARTESIAN_POINT ( 'NONE',  ( 72.01443008256866563, 72.40752555085421704, -2.913864408233449943 ) ) ;
#55252=CARTESIAN_POINT ( 'NONE',  ( 80.08571567400755953, 57.73203133054578018, 16.60244124437337732 ) ) ;
#55253=CARTESIAN_POINT ( 'NONE',  ( 2.922271288615635232, 25.18528772668515714, -1.583844403245363130 ) ) ;
#55257=VERTEX_POINT ( 'NONE', #97451 ) ;
#55261=CARTESIAN_POINT ( 'NONE',  ( 23.56475526289127842, 35.64646525600391413, -2.839279412974133887 ) ) ;
#55263=CARTESIAN_POINT ( 'NONE',  ( 78.36395837149908061, 47.99321896167455748, -14.02406508485639591 ) ) ;
#55267=CARTESIAN_POINT ( 'NONE',  ( 74.28707621773548908, 68.55768173149772338, 11.60544092197708643 ) ) ;
#55271=VECTOR ( 'NONE', #40165, 1000.000000000000000 ) ;
#55273=CARTESIAN_POINT ( 'NONE',  ( 87.05908908046527017, 46.44005007060783186, 8.820244186435306943 ) ) ;
#55286=CARTESIAN_POINT ( 'NONE',  ( 67.68928581972274117, 66.81561979556911979, 8.564295838791961657 ) ) ;
#55287=CARTESIAN_POINT ( 'NONE',  ( 72.10195331805068975, 65.17544479578212702, -12.67587372250991073 ) ) ;
#55292=CARTESIAN_POINT ( 'NONE',  ( 84.68093819348166562, 42.16537887657799644, 0.2499978311480390847 ) ) ;
#55293=EDGE_CURVE ( 'NONE', #23145, #68627, #52837, .T. ) ;
#55297=LINE ( 'NONE', #94359, #7806 ) ;
#55298=FACE_OUTER_BOUND ( 'NONE', #75230, .T. ) ;
#55311=CARTESIAN_POINT ( 'NONE',  ( 85.45699573997251264, 48.32332763657781527, -12.23527099237751692 ) ) ;
#55313=CARTESIAN_POINT ( 'NONE',  ( 71.38293444274448518, 64.54152340162306700, 12.82260361281191052 ) ) ;
#55314=CARTESIAN_POINT ( 'NONE',  ( 88.05520221916579260, 44.74357708579884019, -4.473609059958596035 ) ) ;
#55317=CARTESIAN_POINT ( 'NONE',  ( 70.35757334106033056, 70.80882110823974074, -3.685191203022120110 ) ) ;
#55319=CARTESIAN_POINT ( 'NONE',  ( 82.25840028038837204, 41.50685769110872769, -5.875242208777979869 ) ) ;
#55326=ORIENTED_EDGE ( 'NONE', *, *, #59547, .T. ) ;
#55331=CARTESIAN_POINT ( 'NONE',  ( 12.72979851930235107, 19.30066082961420548, -10.00000000000000533 ) ) ;
#55334=CARTESIAN_POINT ( 'NONE',  ( 72.08669722957829151, 72.05604182950044390, 2.885689024754199306 ) ) ;
#55335=ADVANCED_FACE ( 'NONE', ( #95618 ), #98340, .T. ) ;
#55336=CARTESIAN_POINT ( 'NONE',  ( 4.150881819241740267, 21.13478043621385538, 8.090169943749478065 ) ) ;
#55347=CARTESIAN_POINT ( 'NONE',  ( 33.29248241878940462, 22.14754757982091604, -5.678558825948276656 ) ) ;
#55352=CARTESIAN_POINT ( 'NONE',  ( 66.05783656691208705, 68.59385915743264661, 1.875286379491093447 ) ) ;
#55357=CARTESIAN_POINT ( 'NONE',  ( 2.780145572064765425, 23.64646525600387506, -2.839279412974133887 ) ) ;
#55359=CARTESIAN_POINT ( 'NONE',  ( 14.76917458061509514, 17.03085787977761711, 9.188101187500006262 ) ) ;
#55365=CARTESIAN_POINT ( 'NONE',  ( 87.89296955652562815, 44.95200477618787716, 6.297572492595286953 ) ) ;
#55370=CARTESIAN_POINT ( 'NONE',  ( 72.85632693199180210, 70.83663663905541341, 7.234987929808680995 ) ) ;
#55373=DIRECTION ( 'NONE',  ( 0.000000000000000000, 0.000000000000000000, -1.000000000000000000 ) ) ;
#55376=CARTESIAN_POINT ( 'NONE',  ( 85.04793144752864009, 49.76842598555754194, 13.42690168825989439 ) ) ;
#55377=CARTESIAN_POINT ( 'NONE',  ( 11.41020553640983692, 28.36126292948894800, 6.180339887498949913 ) ) ;
#55383=CARTESIAN_POINT ( 'NONE',  ( 39.48888774545857672, 24.92755873383629250, 6.180339887498953466 ) ) ;
#55385=VERTEX_POINT ( 'NONE', #47201 ) ;
#55388=CARTESIAN_POINT ( 'NONE',  ( 73.70413300610479723, 62.75607992594843410, 14.52880401046331649 ) ) ;
#55390=DIRECTION ( 'NONE',  ( 0.4493970231495826861, -0.7783784768652872721, -0.4383711467890751834 ) ) ;
#55391=EDGE_LOOP ( 'NONE', ( #49950, #64362, #33877, #37255 ) ) ;
#55392=CARTESIAN_POINT ( 'NONE',  ( 82.39459624707119190, 46.56163555380788210, 11.63221967415142011 ) ) ;
#55393=CARTESIAN_POINT ( 'NONE',  ( 88.74573251350186354, 44.01220097505220963, 0.000000000000000000 ) ) ;
#55397=DIRECTION ( 'NONE',  ( 0.5000000000000013323, -0.8660254037844378194, 0.000000000000000000 ) ) ;
#55400=CARTESIAN_POINT ( 'NONE',  ( 18.36860284018464995, 32.64646525600389992, -2.839279412974133887 ) ) ;
#55408=EDGE_CURVE ( 'NONE', #45021, #11459, #52799, .T. ) ;
#55420=CARTESIAN_POINT ( 'NONE',  ( 10.05514423959709625, 21.50829794293879260, -10.00000000000000355 ) ) ;
#55430=CARTESIAN_POINT ( 'NONE',  ( 68.04221563692973973, 69.62749528806014609, 2.672723919121051228 ) ) ;
#55431=CARTESIAN_POINT ( 'NONE',  ( 31.15975419450677819, 23.15404122711134960, 8.090169943749479842 ) ) ;
#55434=CARTESIAN_POINT ( 'NONE',  ( 74.18796447308154995, 68.76651203251665834, -11.36463150814737766 ) ) ;
#55435=EDGE_CURVE ( 'NONE', #48842, #98408, #86268, .T. ) ;
#55440=DIRECTION ( 'NONE',  ( -0.8660254037844379305, -0.5000000000000014433, -0.000000000000000000 ) ) ;
#55451=EDGE_CURVE ( 'NONE', #63738, #11479, #9186, .T. ) ;
#55453=CARTESIAN_POINT ( 'NONE',  ( 72.95338987351841809, 67.58086510047205309, 11.78688422015949477 ) ) ;
#55459=CARTESIAN_POINT ( 'NONE',  ( 74.57284120713386244, 59.58620412426768809, 16.13232198448460863 ) ) ;
#55462=CARTESIAN_POINT ( 'NONE',  ( 18.45335787429653607, 11.44966523072493558, -2.296566073217252530E-15 ) ) ;
#55465=AXIS2_PLACEMENT_3D ( 'NONE', #82494, #91555, #59608 ) ;
#55468=B_SPLINE_CURVE_WITH_KNOTS ( 'NONE', 3,
 ( #55121, #32832, #86107, #1948, #2458, #16634, #63742, #78458, #1457, #55616, #48547, #94676, #25234, #79487, #97177, #65235, #58613, #89112, #81973, #18655, #64752, #2975, #27744, #18148, #19661, #12550, #58130, #66240, #11059, #65722, #96679 ),
 .UNSPECIFIED., .F., .F.,
 ( 4, 3, 3, 3, 3, 3, 3, 3, 3, 3, 4 ),
 ( 0.000000000000000000, 0.1333490885032316831, 0.3007194338854232707, 0.4699862290244899432, 0.5844252810809152932, 0.6686540514502595789, 0.7354980260655316071, 0.8028463152565562533, 0.8633854507756971719, 0.9437142632666813968, 1.000000000000000000 ),
 .UNSPECIFIED. ) ;
#55474=CARTESIAN_POINT ( 'NONE',  ( 65.88310562893973099, 69.02589174555536999, 1.996831191813060347 ) ) ;
#55475=ORIENTED_EDGE ( 'NONE', *, *, #52182, .T. ) ;
#55479=ORIENTED_EDGE ( 'NONE', *, *, #93249, .T. ) ;
#55480=CARTESIAN_POINT ( 'NONE',  ( 75.86452061248199641, 65.14283366293828692, -14.47928019947265277 ) ) ;
#55487=CARTESIAN_POINT ( 'NONE',  ( 34.84170590957603508, 35.51421378149921537, -9.188101187500004485 ) ) ;
#55493=CARTESIAN_POINT ( 'NONE',  ( 84.07632125876401119, 43.96420502296712840, -8.427032882940022063 ) ) ;
#55495=CARTESIAN_POINT ( 'NONE',  ( 86.20597319207941212, 46.97128461232403396, -10.07072581233441610 ) ) ;
#55496=LINE ( 'NONE', #10429, #11980 ) ;
#55499=DIRECTION ( 'NONE',  ( 0.5000000000000014433, -0.8660254037844378194, 0.000000000000000000 ) ) ;
#55501=VERTEX_POINT ( 'NONE', #41090 ) ;
#55505=FACE_OUTER_BOUND ( 'NONE', #72847, .T. ) ;
#55506=ORIENTED_EDGE ( 'NONE', *, *, #57133, .T. ) ;
#55508=CARTESIAN_POINT ( 'NONE',  ( 78.31895580137157253, 49.37400206353071752, 14.66798886358647813 ) ) ;
#55509=EDGE_LOOP ( 'NONE', ( #66993, #76826, #9545, #33750 ) ) ;
#55514=CARTESIAN_POINT ( 'NONE',  ( 66.90909321525143127, 68.17756947874360662, -6.600776075497400974 ) ) ;
#55515=DIRECTION ( 'NONE',  ( -0.8660254037844378194, -0.5000000000000014433, -0.000000000000000000 ) ) ;
#55521=CARTESIAN_POINT ( 'NONE',  ( 38.02916716989017942, 40.14336893147758900, 7.433330006724141015 ) ) ;
#55525=VERTEX_POINT ( 'NONE', #27900 ) ;
#55530=CARTESIAN_POINT ( 'NONE',  ( 72.76527857391883458, 64.58864651986012007, 13.32453080016684588 ) ) ;
#55533=CARTESIAN_POINT ( 'NONE',  ( 78.96239046496309300, 54.80267053941222599, 16.44022611344569285 ) ) ;
#55551=ORIENTED_EDGE ( 'NONE', *, *, #99606, .T. ) ;
#55558=CARTESIAN_POINT ( 'NONE',  ( 74.39896838111268096, 68.39356553035000275, 11.80479640254015195 ) ) ;
#55566=DIRECTION ( 'NONE',  ( -0.4330127018922173554, -0.2499999999999980016, 0.8660254037844402619 ) ) ;
#55567=CARTESIAN_POINT ( 'NONE',  ( 72.04834849415195208, 72.28436413801230742, -0.8995985284803106330 ) ) ;
#55570=DIRECTION ( 'NONE',  ( 0.4145187862775202015, -0.7179675985244525771, -0.5591929034707450175 ) ) ;
#55572=CARTESIAN_POINT ( 'NONE',  ( 76.22210074466102014, 51.34659161545482675, 15.62784121295812767 ) ) ;
#55583=CARTESIAN_POINT ( 'NONE',  ( 88.17984709959166878, 44.08761100535731714, 0.5351384936683012405 ) ) ;
#55589=CARTESIAN_POINT ( 'NONE',  ( 26.89353023359722883, 24.03085787977764198, 9.188101187500006262 ) ) ;
#55591=CARTESIAN_POINT ( 'NONE',  ( 80.73658319580380294, 47.53320970514121768, -13.02157490326441902 ) ) ;
#55592=CARTESIAN_POINT ( 'NONE',  ( 15.22926075146606273, 30.83396525600389637, -2.839279412974133887 ) ) ;
#55594=DIRECTION ( 'NONE',  ( -0.5000000000000013323, 0.8660254037844379305, 0.000000000000000000 ) ) ;
#55605=CARTESIAN_POINT ( 'NONE',  ( 77.69869663927875081, 49.40449606496737545, 15.31866489331840420 ) ) ;
#55610=B_SPLINE_CURVE_WITH_KNOTS ( 'NONE', 3,
 ( #29821, #61209, #13633, #59712, #75436, #91653, #30824, #91156, #90678, #67828, #15102, #98750, #60695, #29330, #22219, #13144 ),
 .UNSPECIFIED., .F., .F.,
 ( 4, 1, 2, 2, 2, 1, 2, 2, 4 ),
 ( 0.000000000000000000, 0.1249999999999974465, 0.1874999999999963918, 0.2499999999999953371, 0.4999999999999977796, 0.6249999999999976685, 0.6874999999999975575, 0.7499999999999975575, 1.000000000000000000 ),
 .UNSPECIFIED. ) ;
#55616=CARTESIAN_POINT ( 'NONE',  ( 72.40589440182066028, 71.76200285602328677, 5.709577571112511407 ) ) ;
#55620=CARTESIAN_POINT ( 'NONE',  ( 22.20737081713590655, 33.79752408145593279, -5.678558825948271327 ) ) ;
#55621=CARTESIAN_POINT ( 'NONE',  ( 79.78566621355244592, 44.75865846334889397, 11.33384506647717416 ) ) ;
#55622=CARTESIAN_POINT ( 'NONE',  ( 75.21677898156802655, 66.43306031420556224, -13.15226642884186070 ) ) ;
#55623=LINE ( 'NONE', #86606, #39679 ) ;
#55625=DIRECTION ( 'NONE',  ( -0.5840252505817139506, 0.000000000000000000, -0.8117354905897402606 ) ) ;
#55640=CARTESIAN_POINT ( 'NONE',  ( 78.10947740687990404, 61.47724562959768946, -16.15800848020992930 ) ) ;
#55659=CARTESIAN_POINT ( 'NONE',  ( 28.71959338928917305, 24.78052372038641593, -10.00000000000000355 ) ) ;
#55662=CARTESIAN_POINT ( 'NONE',  ( 88.27143343078938642, 44.36575123808635368, 4.213746458969101383 ) ) ;
#55663=ORIENTED_EDGE ( 'NONE', *, *, #8783, .T. ) ;
#55664=CARTESIAN_POINT ( 'NONE',  ( 85.82643298209987393, 43.85229891390187618, -5.345846949436618090 ) ) ;
#55665=LINE ( 'NONE', #63289, #6072 ) ;
#55669=CARTESIAN_POINT ( 'NONE',  ( 72.58249898592296745, 70.72798385450705894, 7.152797386299237559 ) ) ;
#55674=CARTESIAN_POINT ( 'NONE',  ( 86.31701533123542447, 45.73308513344992576, 8.415584269618911151 ) ) ;
#55676=CARTESIAN_POINT ( 'NONE',  ( 83.55704177478077099, 51.98730140788478593, 15.00998877770038042 ) ) ;
#55681=CARTESIAN_POINT ( 'NONE',  ( 72.91325260937172459, 64.33234797326966259, -13.52415029394816770 ) ) ;
#55683=CARTESIAN_POINT ( 'NONE',  ( 73.80042137613033049, 55.16559329544060120, 16.59890288620815824 ) ) ;
#55685=CARTESIAN_POINT ( 'NONE',  ( 26.33642183074453058, 30.90829794293881960, 10.00000000000000355 ) ) ;
#55695=CARTESIAN_POINT ( 'NONE',  ( 82.07978327023018039, 41.81623142779876900, 5.466382998867931775 ) ) ;
#55699=CARTESIAN_POINT ( 'NONE',  ( 37.92328063009087202, 22.86426979415092475, -3.090169943749474069 ) ) ;
#55704=CARTESIAN_POINT ( 'NONE',  ( 83.44503355366286712, 51.91352208420826031, 15.00625484349790106 ) ) ;
#55707=CARTESIAN_POINT ( 'NONE',  ( 69.94880244668077296, 66.76424936624940187, -10.23932032170969997 ) ) ;
#55714=B_SPLINE_CURVE_WITH_KNOTS ( 'NONE', 3,
 ( #56310, #100071, #48740, #52951, #37736, #6850, #84887, #62526, #69643, #30658, #10234, #14936, #91488, #22051, #87306, #53924, #15427, #84390, #60535, #99566, #46847, #46325, #743, #17839, #83901, #45345, #30149, #79672, #15944, #41103, #77250 ),
 .UNSPECIFIED., .F., .F.,
 ( 4, 3, 3, 3, 3, 3, 3, 3, 3, 3, 4 ),
 ( 0.000000000000000000, 0.1333490885032278528, 0.3007194338854267679, 0.4699862290245069296, 0.5844252810809245080, 0.6686540514502667953, 0.7354980260655522573, 0.8028463152565803451, 0.8633854507757331431, 0.9437142632667367970, 1.000000000000000000 ),
 .UNSPECIFIED. ) ;
#55722=CARTESIAN_POINT ( 'NONE',  ( 21.45803809350889679, 35.49540643055188127, 3.479690158560446702E-15 ) ) ;
#55726=ORIENTED_EDGE ( 'NONE', *, *, #38803, .T. ) ;
#55727=CARTESIAN_POINT ( 'NONE',  ( 4.137530017820133743, 25.49540643055185285, 3.479690158560446702E-15 ) ) ;
#55729=CARTESIAN_POINT ( 'NONE',  ( 77.85254210321063795, 58.20651666130322610, -16.18224212962651265 ) ) ;
#55730=CARTESIAN_POINT ( 'NONE',  ( 71.49023828022640714, 72.34911387847559183, -1.236132173619994168 ) ) ;
#55734=DIRECTION ( 'NONE',  ( -0.8660254037844379305, -0.5000000000000014433, -0.000000000000000000 ) ) ;
#55738=ORIENTED_EDGE ( 'NONE', *, *, #68616, .T. ) ;
#55742=CARTESIAN_POINT ( 'NONE',  ( 34.78335331324970525, 43.58029201028044497, 1.583844403245397769 ) ) ;
#55744=CARTESIAN_POINT ( 'NONE',  ( 72.71379711463576712, 57.17174861646414996, -15.88508012487434939 ) ) ;
#55745=CARTESIAN_POINT ( 'NONE',  ( 77.33081447068806824, 63.24619402228064047, 15.57729104808880294 ) ) ;
#55754=CARTESIAN_POINT ( 'NONE',  ( 30.72569264534336142, 26.24335787977765122, -9.188101187500008038 ) ) ;
#55757=CARTESIAN_POINT ( 'NONE',  ( 78.39811245026406539, 48.00393270933970058, -14.01973118892057357 ) ) ;
#55759=CARTESIAN_POINT ( 'NONE',  ( 74.41008358870023187, 68.25813196090381041, 11.42500230979621634 ) ) ;
#55765=CARTESIAN_POINT ( 'NONE',  ( 72.02976470237955198, 59.30830629416842470, -15.33705471575644808 ) ) ;
#55767=CARTESIAN_POINT ( 'NONE',  ( 78.86219776201926379, 59.55369065033505649, 16.50996775951927020 ) ) ;
#55768=ORIENTED_EDGE ( 'NONE', *, *, #17831, .F. ) ;
#55770=CARTESIAN_POINT ( 'NONE',  ( 69.94473186773970497, 69.73739167999330846, -5.878840642600716038 ) ) ;
#55777=CARTESIAN_POINT ( 'NONE',  ( 86.87502629904909668, 43.20941739936903758, -2.818466721968422739 ) ) ;
#55780=CARTESIAN_POINT ( 'NONE',  ( 75.48012123268173923, 53.33211347945791658, 16.49774674168797972 ) ) ;
#55782=ORIENTED_EDGE ( 'NONE', *, *, #33686, .F. ) ;
#55784=CARTESIAN_POINT ( 'NONE',  ( 83.32494336655207690, 41.48408949819171454, -1.461985904981788487 ) ) ;
#55787=CARTESIAN_POINT ( 'NONE',  ( 83.90615881913062424, 51.69600214455904563, -14.41633884075334393 ) ) ;
#55790=CARTESIAN_POINT ( 'NONE',  ( 80.64870151538644905, 57.33808369813028349, -16.23392458231729307 ) ) ;
#55799=DIRECTION ( 'NONE',  ( 0.4755282581475757664, -0.8236391035463335175, -0.3090169943749448977 ) ) ;
#55801=CARTESIAN_POINT ( 'NONE',  ( 78.92023586790456591, 59.45316570216661489, -16.52216786098995982 ) ) ;
#55803=CARTESIAN_POINT ( 'NONE',  ( 70.93180422968134735, 70.94319162518513622, -4.401341846138759450 ) ) ;
#55805=CARTESIAN_POINT ( 'NONE',  ( 82.30224259366366368, 41.51585266683629527, -5.837696018721792335 ) ) ;
#55812=CARTESIAN_POINT ( 'NONE',  ( 76.26004098100119677, 53.26552314622699669, -15.96572022850413219 ) ) ;
#55813=VERTEX_POINT ( 'NONE', #91228 ) ;
#55816=CARTESIAN_POINT ( 'NONE',  ( 87.92709505194216035, 44.79768224621495420, 4.873456775040940769 ) ) ;
#55819=CARTESIAN_POINT ( 'NONE',  ( 10.22618198766610575, 28.83705186507752671, 3.090169943749475401 ) ) ;
#55822=CARTESIAN_POINT ( 'NONE',  ( 74.08065690531799419, 54.82731643721707826, -16.13522336645903721 ) ) ;
#55828=CARTESIAN_POINT ( 'NONE',  ( 66.36217872752992264, 68.78091108627523909, -4.321716179073264996 ) ) ;
#55829=ORIENTED_EDGE ( 'NONE', *, *, #95552, .T. ) ;
#55834=CARTESIAN_POINT ( 'NONE',  ( 39.23796756512304995, 23.44966523072497822, -2.296566073217252530E-15 ) ) ;
#55837=EDGE_CURVE ( 'NONE', #42053, #46017, #72650, .T. ) ;
#55839=CARTESIAN_POINT ( 'NONE',  ( 25.38519627463738715, 32.84336893147757053, -7.433330006724137462 ) ) ;
#55842=CARTESIAN_POINT ( 'NONE',  ( 66.25952267273640928, 69.15726288014950285, 2.537017490915350670 ) ) ;
#55847=CARTESIAN_POINT ( 'NONE',  ( 8.859747497914600700, 17.06628583063839599, -9.188101187500006262 ) ) ;
#55849=VECTOR ( 'NONE', #44075, 1000.000000000000114 ) ;
#55850=CARTESIAN_POINT ( 'NONE',  ( 84.81351086726648703, 50.35522970061591508, -13.86072692636569670 ) ) ;
#55852=ADVANCED_FACE ( 'NONE', ( #4208 ), #56411, .T. ) ;
#55855=AXIS2_PLACEMENT_3D ( 'NONE', #18083, #17060, #87550 ) ;
#55857=CARTESIAN_POINT ( 'NONE',  ( 87.88245627177123254, 44.92329797532170943, 6.249457923817309357 ) ) ;
#55862=CARTESIAN_POINT ( 'NONE',  ( 86.72740319991413571, 46.97082492543196963, 10.28929863393111610 ) ) ;
#55867=CARTESIAN_POINT ( 'NONE',  ( 84.55218960391981398, 48.55517814912271746, -12.33429493815133782 ) ) ;
#55868=CARTESIAN_POINT ( 'NONE',  ( 20.78273902371470072, 14.12755873383625804, -6.180339887498949025 ) ) ;
#55880=ORIENTED_EDGE ( 'NONE', *, *, #72773, .F. ) ;
#55882=CARTESIAN_POINT ( 'NONE',  ( 73.73726724665601751, 62.90511275149663106, 14.47564044095566160 ) ) ;
#55886=ORIENTED_EDGE ( 'NONE', *, *, #3580, .T. ) ;
#55887=EDGE_CURVE ( 'NONE', #14510, #57901, #12326, .T. ) ;
#55889=CARTESIAN_POINT ( 'NONE',  ( 71.26320768968655273, 69.07654504452045785, 8.407160263220744056 ) ) ;
#55891=CARTESIAN_POINT ( 'NONE',  ( 82.51639823017981712, 53.47659673923356394, -15.74004163755323482 ) ) ;
#55892=EDGE_CURVE ( 'NONE', #40803, #54888, #85357, .T. ) ;
#55896=CARTESIAN_POINT ( 'NONE',  ( 20.38389956778225809, 29.95586893147755703, 7.433330006724141015 ) ) ;
#55902=CARTESIAN_POINT ( 'NONE',  ( 81.49499594866964003, 59.57084509763894431, -0.08682408883347023099 ) ) ;
#55904=EDGE_CURVE ( 'NONE', #53182, #26719, #81772, .T. ) ;
#55912=CARTESIAN_POINT ( 'NONE',  ( 74.94692089407371327, 66.84572622250871632, -13.20830831734917687 ) ) ;
#55917=CARTESIAN_POINT ( 'NONE',  ( 82.29815274954648885, 40.89485058540869034, -1.228882935992447578 ) ) ;
#55927=CARTESIAN_POINT ( 'NONE',  ( 87.94702792923476409, 43.95278803585774341, 0.4997626018594838460 ) ) ;
#55929=CARTESIAN_POINT ( 'NONE',  ( 83.58440307966948524, 42.98227934588280874, 6.232988767175322131 ) ) ;
#55932=LINE ( 'NONE', #9886, #98478 ) ;
#55937=CARTESIAN_POINT ( 'NONE',  ( 84.19046594057184052, 47.86424601814110247, 11.90803564236390422 ) ) ;
#55939=EDGE_CURVE ( 'NONE', #92701, #50903, #90204, .T. ) ;
#55940=CARTESIAN_POINT ( 'NONE',  ( 31.34407949807308569, 36.83478043621390441, -8.090169943749479842 ) ) ;
#55941=CARTESIAN_POINT ( 'NONE',  ( 68.88995186411204941, 64.71362435216896358, -12.21736274004632783 ) ) ;
#55947=CARTESIAN_POINT ( 'NONE',  ( 67.72512177463541150, 68.26770340457413511, -7.327815147115877004 ) ) ;
#55956=CARTESIAN_POINT ( 'NONE',  ( 18.38602693954342371, 22.56628583063840310, 9.188101187500006262 ) ) ;
#55957=CARTESIAN_POINT ( 'NONE',  ( 74.66874582000750138, 67.11449834074296916, 12.47724195657757029 ) ) ;
#55959=CARTESIAN_POINT ( 'NONE',  ( 82.44310520575160695, 54.28011738120408580, -15.96781897959229113 ) ) ;
#55973=VERTEX_POINT ( 'NONE', #39071 ) ;
#55974=CARTESIAN_POINT ( 'NONE',  ( 72.11864215578678738, 72.30468452837580173, 1.217881537791027702 ) ) ;
#55982=CARTESIAN_POINT ( 'NONE',  ( 32.59967566254915994, 39.79752408145595410, -5.678558825948271327 ) ) ;
#55989=CARTESIAN_POINT ( 'NONE',  ( 86.29029894244921195, 46.98537786981302844, -10.03429304951027490 ) ) ;
#55995=CARTESIAN_POINT ( 'NONE',  ( 45.29353982640898835, 28.01110640527296525, 2.839279412974134775 ) ) ;
#55998=EDGE_LOOP ( 'NONE', ( #94804, #25938, #95001, #28154 ) ) ;
#56004=CARTESIAN_POINT ( 'NONE',  ( 77.14924902310487198, 49.32506698715211257, -14.89041676429049232 ) ) ;
#56017=EDGE_CURVE ( 'NONE', #9204, #66666, #34533, .T. ) ;
#56020=CARTESIAN_POINT ( 'NONE',  ( 75.65485643130637072, 54.67754446188314432, 16.11849813384655050 ) ) ;
#56023=PLANE ( 'NONE',  #29882 ) ;
#56024=VERTEX_POINT ( 'NONE', #34982 ) ;
#56030=CARTESIAN_POINT ( 'NONE',  ( 71.12465364093185372, 72.19127489105424900, 0.5914781838053912999 ) ) ;
#56031=CARTESIAN_POINT ( 'NONE',  ( 80.81823777232595774, 43.03079984276644154, 9.681521901304016353 ) ) ;
#56044=DIRECTION ( 'NONE',  ( -0.4851478631379979034, 0.8403007481384877631, 0.2419218955996582654 ) ) ;
#56058=CARTESIAN_POINT ( 'NONE',  ( 69.88429420325151398, 70.97642176483110177, -1.039711900314023829 ) ) ;
#56061=CARTESIAN_POINT ( 'NONE',  ( 67.59152061837809811, 66.69868789956184685, 8.645681936733796036 ) ) ;
#56062=CARTESIAN_POINT ( 'NONE',  ( 88.03469742524457331, 44.28626028149027860, -4.397723919905312862 ) ) ;
#56067=CARTESIAN_POINT ( 'NONE',  ( 84.87428755225029420, 50.22423732196602941, -13.34510061061973829 ) ) ;
#56069=CARTESIAN_POINT ( 'NONE',  ( 77.59444824636439364, 61.81028894563407050, 15.66474382954858413 ) ) ;
#56078=CARTESIAN_POINT ( 'NONE',  ( 80.01979875032591849, 57.54866692369600401, 16.59896302490741604 ) ) ;
#56079=CARTESIAN_POINT ( 'NONE',  ( 73.43248428410468875, 69.89844921070914552, 9.717079046730820124 ) ) ;
#56081=CARTESIAN_POINT ( 'NONE',  ( 76.83812372118222811, 63.31165668814058023, -15.46182035231785079 ) ) ;
#56084=CARTESIAN_POINT ( 'NONE',  ( 88.36916805580219147, 44.19665079577453071, 0.1927284833306444622 ) ) ;
#56085=EDGE_CURVE ( 'NONE', #45306, #61384, #41073, .T. ) ;
#56090=CARTESIAN_POINT ( 'NONE',  ( 25.79477067763620468, 36.93396525600391556, 2.839279412974139660 ) ) ;
#56094=ORIENTED_EDGE ( 'NONE', *, *, #35429, .T. ) ;
#56095=CARTESIAN_POINT ( 'NONE',  ( 13.67041502465407277, 29.93396525600389424, 2.839279412974139660 ) ) ;
#56097=CARTESIAN_POINT ( 'NONE',  ( 76.57610849078304227, 63.76548037954881920, 14.87549170960290645 ) ) ;
#56099=VECTOR ( 'NONE', #2124, 1000.000000000000000 ) ;
#56111=EDGE_LOOP ( 'NONE', ( #7816, #63510 ) ) ;
#56116=CARTESIAN_POINT ( 'NONE',  ( 73.24164692391426001, 68.69381212440423212, -10.32746940148697234 ) ) ;
#56124=CARTESIAN_POINT ( 'NONE',  ( 23.32838594064934767, 31.65586893147757408, -7.433330006724137462 ) ) ;
#56125=CARTESIAN_POINT ( 'NONE',  ( 84.73244144816675316, 50.45694327749722419, -13.52220349883642569 ) ) ;
#56130=ORIENTED_EDGE ( 'NONE', *, *, #10976, .T. ) ;
#56133=CARTESIAN_POINT ( 'NONE',  ( 67.69820113011998330, 65.71482418403419956, 10.68697367106847196 ) ) ;
#56135=CARTESIAN_POINT ( 'NONE',  ( 81.78067039160912088, 55.44360204288782512, -15.94198801934737908 ) ) ;
#56140=CARTESIAN_POINT ( 'NONE',  ( 76.43459130371124388, 61.29278126438280339, -15.98275306604615054 ) ) ;
#56146=VECTOR ( 'NONE', #76162, 1000.000000000000114 ) ;
#56150=ORIENTED_EDGE ( 'NONE', *, *, #47729, .F. ) ;
#56151=CARTESIAN_POINT ( 'NONE',  ( 79.99398376985880077, 44.81349857560560679, -11.27244585305868085 ) ) ;
#56152=ADVANCED_FACE ( 'NONE', ( #5587 ), #43584, .T. ) ;
#56156=CARTESIAN_POINT ( 'NONE',  ( 83.37551210837683868, 41.64352063595823239, -2.325603929493660793 ) ) ;
#56157=CARTESIAN_POINT ( 'NONE',  ( 84.30219332075782290, 47.40784315339518429, -11.50221644715631442 ) ) ;
#56160=B_SPLINE_CURVE_WITH_KNOTS ( 'NONE', 3,
 ( #63402, #63898, #26907, #64909, #57786, #2621, #18811, #95368, #25921, #79648, #41079, #49695, #56793, #87779, #94340, #19335, #49215, #11716, #17297, #80147, #71524, #80649, #88762, #41589, #24895, #55770, #50197, #34022, #86763, #73025, #81149, #42577, #73510, #48200, #79147, #9729, #40583, #59779, #13698, #27410, #58289, #28902, #44071, #82654, #5591, #59264 ),
 .UNSPECIFIED., .F., .F.,
 ( 4, 1, 1, 1, 2, 2, 1, 1, 1, 2, 2, 1, 1, 2, 2, 1, 1, 2, 2, 1, 1, 2, 2, 1, 2, 2, 1, 2, 2, 4 ),
 ( 0.000000000000000000, 0.06249999999997057909, 0.09374999999995715927, 0.1093749999999491240, 0.1171874999999468620, 0.1249999999999445999, 0.1874999999999323874, 0.2187499999999275579, 0.2343749999999261702, 0.2421874999999250877, 0.2499999999999240052, 0.3124999999999299449, 0.3437499999999344968, 0.3593749999999367728, 0.3749999999999391043, 0.4374999999999454880, 0.4687499999999472089, 0.4843749999999496514, 0.4999999999999521494, 0.5624999999999568123, 0.5937499999999590328, 0.6093749999999601430, 0.6249999999999612532, 0.6874999999999653610, 0.7187499999999689138, 0.7499999999999725775, 0.8124999999999800160, 0.8437499999999837907, 0.8749999999999876765, 1.000000000000000000 ),
 .UNSPECIFIED. ) ;
#56161=ORIENTED_EDGE ( 'NONE', *, *, #23778, .T. ) ;
#56172=CARTESIAN_POINT ( 'NONE',  ( 80.94948737998437593, 46.40359012725748755, 12.14654003525263271 ) ) ;
#56175=CARTESIAN_POINT ( 'NONE',  ( 71.71174882302005926, 58.93038559421764688, -15.88944412480316259 ) ) ;
#56186=CARTESIAN_POINT ( 'NONE',  ( 83.48272809759448876, 51.94771123612188291, 15.01134753452855186 ) ) ;
#56190=ORIENTED_EDGE ( 'NONE', *, *, #35314, .F. ) ;
#56194=CARTESIAN_POINT ( 'NONE',  ( 74.31898897143159388, 55.32162592116677047, 16.60231691840947477 ) ) ;
#56196=CARTESIAN_POINT ( 'NONE',  ( 31.59046986846508887, 19.20801979619930222, -3.090169943749474069 ) ) ;
#56204=B_SPLINE_CURVE_WITH_KNOTS ( 'NONE', 3,
 ( #82683, #91257, #60299, #91755, #30419, #20850, #21330, #13250, #52706, #52214, #83160, #82181, #98848, #75046, #99341, #22318 ),
 .UNSPECIFIED., .F., .F.,
 ( 4, 1, 2, 2, 2, 1, 2, 2, 4 ),
 ( 0.000000000000000000, 0.1249999999999995004, 0.1874999999999981126, 0.2499999999999967248, 0.4999999999999920619, 0.6249999999999913403, 0.6874999999999925615, 0.7499999999999938938, 1.000000000000000000 ),
 .UNSPECIFIED. ) ;
#56206=ORIENTED_EDGE ( 'NONE', *, *, #11368, .T. ) ;
#56208=DIRECTION ( 'NONE',  ( 0.4330127018922168558, -0.7499999999999987788, 0.5000000000000039968 ) ) ;
#56209=CARTESIAN_POINT ( 'NONE',  ( 82.10624035338234705, 41.84472205286013491, 5.498941269084485661 ) ) ;
#56211=CARTESIAN_POINT ( 'NONE',  ( 32.88524308553003550, 19.39040679176984838, -6.890680421881970419E-14 ) ) ;
#56212=CARTESIAN_POINT ( 'NONE',  ( 39.55573625059402332, 31.03677371833804699, 10.00000000000000533 ) ) ;
#56217=CARTESIAN_POINT ( 'NONE',  ( 4.698709606056801213, 26.21091486745858390, -1.111400068045478839E-16 ) ) ;
#56220=EDGE_CURVE ( 'NONE', #99079, #96205, #40623, .T. ) ;
#56221=B_SPLINE_CURVE_WITH_KNOTS ( 'NONE', 3,
 ( #35628, #66033, #58417, #89393, #66527, #50819, #81768, #97455, #28023, #58898, #17952, #79783, #72155, #99930, #36609, #44206, #60895, #7206, #83252, #13819, #76148, #44700, #14810, #51835, #98446, #75631, #29037, #20953, #90375, #6722, #21914, #43713, #82776, #99434, #45209, #29523, #59908, #90878, #30514, #21427, #6217, #52314, #30011, #91859, #52803, #98941 ),
 .UNSPECIFIED., .F., .F.,
 ( 4, 1, 2, 2, 1, 2, 2, 1, 1, 2, 2, 1, 1, 2, 2, 1, 1, 2, 2, 1, 1, 1, 2, 2, 1, 1, 1, 2, 2, 4 ),
 ( 0.000000000000000000, 0.06249999999999610034, 0.09374999999999414357, 0.1249999999999922007, 0.1874999999999881484, 0.2187499999999878986, 0.2499999999999876765, 0.3124999999999863998, 0.3437499999999856781, 0.3593749999999852340, 0.3749999999999847899, 0.4374999999999796274, 0.4687499999999789613, 0.4843749999999789613, 0.4999999999999789058, 0.5624999999999704681, 0.5937499999999658051, 0.6093749999999658051, 0.6249999999999656941, 0.6874999999999559241, 0.7187499999999531486, 0.7343749999999520384, 0.7421874999999514833, 0.7499999999999509281, 0.8124999999999613642, 0.8437499999999666933, 0.8593749999999676925, 0.8671874999999703570, 0.8749999999999729106, 1.000000000000000000 ),
 .UNSPECIFIED. ) ;
#56225=CARTESIAN_POINT ( 'NONE',  ( 69.16499752431022330, 66.81492530410388042, -9.669340448346357419 ) ) ;
#56228=EDGE_CURVE ( 'NONE', #7719, #66239, #69044, .T. ) ;
#56230=CARTESIAN_POINT ( 'NONE',  ( 67.24564144887035866, 66.53705660361565322, -8.596795619140232603 ) ) ;
#56233=CARTESIAN_POINT ( 'NONE',  ( 77.36734184492237887, 49.76646884952617711, -14.99839566343147190 ) ) ;
#56235=ORIENTED_EDGE ( 'NONE', *, *, #33705, .T. ) ;
#56241=CARTESIAN_POINT ( 'NONE',  ( 26.72152145096863762, 27.37878583063842086, 9.188101187500006262 ) ) ;
#56247=CARTESIAN_POINT ( 'NONE',  ( 6.965323710529800927, 24.99752408145590010, 5.678558825948276656 ) ) ;
#56248=LINE ( 'NONE', #30954, #72770 ) ;
#56251=CARTESIAN_POINT ( 'NONE',  ( 72.29163330765324247, 71.12640426941348437, -6.047334876408406501 ) ) ;
#56256=EDGE_LOOP ( 'NONE', ( #72241, #70714, #55829, #36160 ) ) ;
#56262=FACE_OUTER_BOUND ( 'NONE', #91584, .T. ) ;
#56264=CARTESIAN_POINT ( 'NONE',  ( 72.77552873970981295, 57.60274552232836243, -16.30610872563569913 ) ) ;
#56265=CYLINDRICAL_SURFACE ( 'NONE', #74291, 10.00000000000001066 ) ;
#56272=CARTESIAN_POINT ( 'NONE',  ( 28.60632300232807879, 31.91421378149921040, 9.188101187500008038 ) ) ;
#56274=CARTESIAN_POINT ( 'NONE',  ( 69.68250337734514233, 70.54332952169561111, -4.835715172394301042 ) ) ;
#56276=CARTESIAN_POINT ( 'NONE',  ( 73.78595477147815984, 68.43622263357737268, 10.95456581244436123 ) ) ;
#56281=CARTESIAN_POINT ( 'NONE',  ( 78.05001017509421501, 57.38512016837487550, -16.19126229228278646 ) ) ;
#56283=CARTESIAN_POINT ( 'NONE',  ( 78.77431960351366058, 58.56495644472522599, 16.58374741466410285 ) ) ;
#56291=AXIS2_PLACEMENT_3D ( 'NONE', #7179, #53766, #45183 ) ;
#56295=CARTESIAN_POINT ( 'NONE',  ( 75.94688732371197659, 65.57317746828351801, 13.88815714291336967 ) ) ;
#56305=CARTESIAN_POINT ( 'NONE',  ( 83.78311978599397492, 51.75050911116664309, -14.85521894841905599 ) ) ;
#56308=CARTESIAN_POINT ( 'NONE',  ( 80.65713072601933220, 57.38499450659126921, -16.23539640514130866 ) ) ;
#56310=CARTESIAN_POINT ( 'NONE',  ( 72.97386446981147401, 70.68132344495337804, 8.316175787459499702 ) ) ;
#56311=CARTESIAN_POINT ( 'NONE',  ( 72.06633338339661066, 71.38138388103391208, 5.132520212388754111 ) ) ;
#56322=CARTESIAN_POINT ( 'NONE',  ( 87.97560163977048830, 44.53565211440820804, -3.995394561512739973 ) ) ;
#56331=CARTESIAN_POINT ( 'NONE',  ( 78.96647079090445231, 52.43242654007526227, -15.54601558169038356 ) ) ;
#56334=CARTESIAN_POINT ( 'NONE',  ( 87.77191196787447325, 44.75263600343390635, 5.004501849949501313 ) ) ;
#56336=CARTESIAN_POINT ( 'NONE',  ( 20.52402715336229377, 23.80066082961421969, 10.00000000000000533 ) ) ;
#56337=CARTESIAN_POINT ( 'NONE',  ( 88.17148522932362198, 43.68169873549415883, 0.1729226289268755989 ) ) ;
#56340=CARTESIAN_POINT ( 'NONE',  ( 73.99515186944866230, 54.97541550364575613, -16.60506967706033521 ) ) ;
#56354=CARTESIAN_POINT ( 'NONE',  ( 37.59133656659163591, 37.10171378149920685, 9.188101187500008038 ) ) ;
#56359=CARTESIAN_POINT ( 'NONE',  ( 26.18025557360336464, 27.06628583063842797, -9.188101187500006262 ) ) ;
#56360=CARTESIAN_POINT ( 'NONE',  ( 23.96727898247415212, 22.03677371833801857, 10.00000000000000533 ) ) ;
#56361=CARTESIAN_POINT ( 'NONE',  ( 87.99973427719299934, 43.78392399561506210, 2.406698522940700080 ) ) ;
#56363=CARTESIAN_POINT ( 'NONE',  ( 66.34034349336292280, 68.67733634918475616, 2.360395268154211301 ) ) ;
#56369=CARTESIAN_POINT ( 'NONE',  ( 15.84867609773810138, 11.01110640527290840, 2.839279412974134775 ) ) ;
#56371=CARTESIAN_POINT ( 'NONE',  ( 21.91745948943429312, 13.44966523072494269, -2.296566073217252530E-15 ) ) ;
#56373=CARTESIAN_POINT ( 'NONE',  ( 84.74798064930895691, 49.97902072749974423, -13.66263633214625806 ) ) ;
#56379=CARTESIAN_POINT ( 'NONE',  ( 87.47635513963552967, 45.03054629282574695, 6.933452704933705135 ) ) ;
#56383=( BOUNDED_CURVE ( )  B_SPLINE_CURVE ( 2, ( #49808, #3726, #27019, #71635, #2230, #94950, #25514, #56404, #87398, #17927, #48825, #79758, #41191 ),
 .UNSPECIFIED., .F., .T. ) 
 B_SPLINE_CURVE_WITH_KNOTS ( ( 3, 2, 2, 2, 2, 2, 3 ),
 ( 0.8875000000000000666, 0.8900000000000000133, 0.8950000000000000178, 0.9000000000000000222, 0.9050000000000000266, 0.9100000000000000311, 0.9125000000000000888 ),
 .UNSPECIFIED. ) 
 CURVE ( )  GEOMETRIC_REPRESENTATION_ITEM ( )  RATIONAL_B_SPLINE_CURVE ( ( 0.9755282581475767101, 0.9755282581475772652, 1.000000000000000000, 0.9510565162951535312, 1.000000000000000000, 0.9510565162951535312, 1.000000000000000000, 0.9510565162951535312, 1.000000000000000000, 0.9510565162951535312, 1.000000000000000000, 0.9755282581475761550, 0.9755282581475767101 ) ) 
 REPRESENTATION_ITEM ( '' )  );
#56386=CARTESIAN_POINT ( 'NONE',  ( 86.47877272607206578, 47.40146553843635502, 10.34156286556493853 ) ) ;
#56388=CARTESIAN_POINT ( 'NONE',  ( 76.84822201109516016, 53.05882888382841855, 15.89418035136032969 ) ) ;
#56391=CARTESIAN_POINT ( 'NONE',  ( 78.39917873861809028, 61.30051739111549836, -15.87534687166327885 ) ) ;
#56393=B_SPLINE_CURVE_WITH_KNOTS ( 'NONE', 3,
 ( #16584, #77399, #1898, #15566, #9501, #31278, #69285, #56061, #39362, #8985 ),
 .UNSPECIFIED., .F., .F.,
 ( 4, 2, 2, 2, 4 ),
 ( 0.000000000000000000, 0.2500000000000000000, 0.5000000000000000000, 0.7500000000000000000, 1.000000000000000000 ),
 .UNSPECIFIED. ) ;
#56404=CARTESIAN_POINT ( 'NONE',  ( 36.03590635313023682, 36.50829794293883168, -10.00000000000000355 ) ) ;
#56411=PLANE ( 'NONE',  #78770 ) ;
#56414=CARTESIAN_POINT ( 'NONE',  ( 70.84700895556564149, 68.24011015210355424, 9.176700790939991137 ) ) ;
#56416=CARTESIAN_POINT ( 'NONE',  ( 82.51292938203759775, 53.28734884524191528, -15.32281082862661670 ) ) ;
#56419=DIRECTION ( 'NONE',  ( 0.4330127018922146354, 0.2500000000000017208, -0.8660254037844404840 ) ) ;
#56420=CARTESIAN_POINT ( 'NONE',  ( 18.21401815691482895, 25.91421378149918198, 9.188101187500008038 ) ) ;
#56421=EDGE_CURVE ( 'NONE', #35964, #79592, #35793, .T. ) ;
#56424=CARTESIAN_POINT ( 'NONE',  ( 75.15191903148871688, 52.97183600646508239, -16.48001256418180915 ) ) ;
#56436=CARTESIAN_POINT ( 'NONE',  ( 5.452216952852307230, 26.08080186712590631, -3.090169943749475845 ) ) ;
#56442=CARTESIAN_POINT ( 'NONE',  ( 82.23777015025109449, 40.85740305880240442, -1.202640854400347736 ) ) ;
#56453=CARTESIAN_POINT ( 'NONE',  ( 80.74610282667754291, 46.90596778374671061, -12.61250437584052264 ) ) ;
#56454=DIRECTION ( 'NONE',  ( 0.3297783986044514615, 0.8484238185761762141, 0.4140328874455545538 ) ) ;
#56458=CARTESIAN_POINT ( 'NONE',  ( 69.13686587061594935, 64.31895405193962745, 11.99662287724232357 ) ) ;
#56459=CARTESIAN_POINT ( 'NONE',  ( 74.41721759878494424, 68.37665257406605690, -11.33153079197290580 ) ) ;
#56462=ORIENTED_EDGE ( 'NONE', *, *, #41371, .F. ) ;
#56463=CARTESIAN_POINT ( 'NONE',  ( 81.74963128441575577, 42.78295644149261534, 7.706177857118651886 ) ) ;
#56468=CARTESIAN_POINT ( 'NONE',  ( 68.91022223095966126, 64.71151235103670274, -12.22836756602027464 ) ) ;
#56473=CARTESIAN_POINT ( 'NONE',  ( 70.21263088009048658, 68.31033697602117627, -9.405330560664618034 ) ) ;
#56481=CARTESIAN_POINT ( 'NONE',  ( 20.65814732634927609, 20.43085787977763346, -9.188101187500008038 ) ) ;
#56482=CARTESIAN_POINT ( 'NONE',  ( 75.06873900396388422, 67.14982071245070472, 12.61085099019435951 ) ) ;
#56494=CARTESIAN_POINT ( 'NONE',  ( 81.72556729995484659, 55.26675154459383066, -15.91896077131915455 ) ) ;
#56500=CARTESIAN_POINT ( 'NONE',  ( 83.80743799779062897, 52.10092053580531513, -14.60766023568177197 ) ) ;
#56501=CARTESIAN_POINT ( 'NONE',  ( 72.32516777325903945, 71.91622842696713747, -5.210293257461823480 ) ) ;
#56505=CARTESIAN_POINT ( 'NONE',  ( 32.94608582406294772, 39.99752408145594984, 5.678558825948277544 ) ) ;
#56508=CARTESIAN_POINT ( 'NONE',  ( 77.75702407734982557, 61.66006977308100545, 16.07490810555906791 ) ) ;
#56513=CARTESIAN_POINT ( 'NONE',  ( 78.99750231315303495, 60.09927444898351467, 16.11767558604333317 ) ) ;
#56515=CARTESIAN_POINT ( 'NONE',  ( 88.39405946958876825, 44.08409158760228053, -2.802556091636618341 ) ) ;
#56517=CARTESIAN_POINT ( 'NONE',  ( 77.90281930814079203, 52.05526166391488374, -15.59995652318183978 ) ) ;
#56518=CARTESIAN_POINT ( 'NONE',  ( 80.55420448732139960, 44.52191585150384157, 11.40672976540375672 ) ) ;
#56521=ORIENTED_EDGE ( 'NONE', *, *, #25154, .F. ) ;
#56522=ORIENTED_EDGE ( 'NONE', *, *, #68695, .T. ) ;
#56524=ORIENTED_EDGE ( 'NONE', *, *, #54186, .F. ) ;
#56525=CARTESIAN_POINT ( 'NONE',  ( 77.29488782935133884, 49.16221438579500358, -14.80191796116666048 ) ) ;
#56527=CARTESIAN_POINT ( 'NONE',  ( 74.51129208461142639, 56.54966615295543164, 16.08098109482861204 ) ) ;
#56530=VERTEX_POINT ( 'NONE', #82889 ) ;
#56539=CARTESIAN_POINT ( 'NONE',  ( 70.98683038387876820, 61.11472152276905945, -14.49225651734631271 ) ) ;
#56540=CARTESIAN_POINT ( 'NONE',  ( 3.154811933878272523, 22.79752408145590081, -5.678558825948271327 ) ) ;
#56558=CARTESIAN_POINT ( 'NONE',  ( 65.74195682738610458, 69.08314406761469684, -0.1047288108484802499 ) ) ;
#56559=VERTEX_POINT ( 'NONE', #23511 ) ;
#56570=CARTESIAN_POINT ( 'NONE',  ( 70.21442515943250839, 62.76251953271914630, -13.45827767252464824 ) ) ;
#56573=CARTESIAN_POINT ( 'NONE',  ( 70.94226914272195472, 66.08589450064482662, -11.46747304436338410 ) ) ;
#56576=CARTESIAN_POINT ( 'NONE',  ( 73.93840856004327122, 68.59252082510937498, 11.39217114877860659 ) ) ;
#56577=CARTESIAN_POINT ( 'NONE',  ( 80.79374179619712493, 43.01268775703235292, -9.676513497087860571 ) ) ;
#56578=CARTESIAN_POINT ( 'NONE',  ( 70.17798417058853033, 71.11987868467312524, -1.451298496092467971 ) ) ;
#56583=AXIS2_PLACEMENT_3D ( 'NONE', #4340, #89021, #96590 ) ;
#56589=CARTESIAN_POINT ( 'NONE',  ( 76.61245916897973984, 51.33784933831625352, 16.06823738657550038 ) ) ;
#56593=CARTESIAN_POINT ( 'NONE',  ( 78.30173519175639285, 54.99922236594399294, -16.08531814199762877 ) ) ;
#56594=CARTESIAN_POINT ( 'NONE',  ( 81.75863700535872169, 59.11420539249230899, 0.4987820251299123764 ) ) ;
#56595=CARTESIAN_POINT ( 'NONE',  ( 73.40253668476441362, 69.84345263918817182, 9.170520863686014934 ) ) ;
#56606=CARTESIAN_POINT ( 'NONE',  ( 87.42943499906034788, 43.57385683440216440, -3.059512906073269978 ) ) ;
#56608=VECTOR ( 'NONE', #81462, 1000.000000000000114 ) ;
#56610=CARTESIAN_POINT ( 'NONE',  ( 25.31423016981892715, 26.56628583063841731, 9.188101187500006262 ) ) ;
#56612=CARTESIAN_POINT ( 'NONE',  ( 79.64551941974546878, 47.76551340485320196, -13.52520812116594762 ) ) ;
#56614=CARTESIAN_POINT ( 'NONE',  ( 19.81074232005190794, 13.29860640527291693, -2.839279412974138328 ) ) ;
#56616=CARTESIAN_POINT ( 'NONE',  ( 76.63523979702124223, 63.50111620409151669, 15.35509843086873438 ) ) ;
#56622=CARTESIAN_POINT ( 'NONE',  ( 86.22850481619846619, 47.19188645326008924, 10.82438011396962096 ) ) ;
#56626=CARTESIAN_POINT ( 'NONE',  ( 74.80005638580958305, 53.39398799171427612, 16.06185578139195869 ) ) ;
#56628=CARTESIAN_POINT ( 'NONE',  ( 82.07265110639774264, 53.99302234254209054, 15.59308437138326831 ) ) ;
#56632=CARTESIAN_POINT ( 'NONE',  ( 78.99848661620950452, 60.24637179098724005, -16.44349368446546222 ) ) ;
#56633=ORIENTED_EDGE ( 'NONE', *, *, #74094, .F. ) ;
#56635=ORIENTED_EDGE ( 'NONE', *, *, #33849, .T. ) ;
#56640=CARTESIAN_POINT ( 'NONE',  ( 29.48198420892519067, 37.99752408145594273, 5.678558825948276656 ) ) ;
#56641=CARTESIAN_POINT ( 'NONE',  ( 80.03260168065229152, 44.35101574960664550, 11.52491460830935921 ) ) ;
#56642=CARTESIAN_POINT ( 'NONE',  ( 84.81351086726648703, 50.35522970061591508, -13.86072692636569670 ) ) ;
#56643=CARTESIAN_POINT ( 'NONE',  ( 83.29144881691568969, 48.30668213657163079, -12.61020633307858141 ) ) ;
#56646=ORIENTED_EDGE ( 'NONE', *, *, #19714, .F. ) ;
#56649=CARTESIAN_POINT ( 'NONE',  ( 68.15538884038467415, 65.80901214634647545, 10.85944937509076880 ) ) ;
#56651=CARTESIAN_POINT ( 'NONE',  ( 81.62233317761165097, 55.86806713927244772, -16.01587696651938941 ) ) ;
#56663=CARTESIAN_POINT ( 'NONE',  ( 77.79976927246816842, 61.42068562798239384, -16.13251659512815550 ) ) ;
#56667=CARTESIAN_POINT ( 'NONE',  ( 80.24153816591007171, 44.93970165375741033, -11.25787842664069593 ) ) ;
#56668=DIRECTION ( 'NONE',  ( -0.2503889871761755259, -0.9681453171404016400, 0.000000000000000000 ) ) ;
#56680=CARTESIAN_POINT ( 'NONE',  ( 75.89038410296754478, 65.15355031958958421, -14.48133090960389069 ) ) ;
#56682=CARTESIAN_POINT ( 'NONE',  ( 87.45985321408362267, 44.85427673109838764, -6.610136163016259836 ) ) ;
#56683=CARTESIAN_POINT ( 'NONE',  ( 77.38344707992528981, 49.10671604805792612, -15.27628165681131200 ) ) ;
#56684=CARTESIAN_POINT ( 'NONE',  ( 87.69233101511819939, 44.71197863951398688, 5.019790285073527869 ) ) ;
#56685=VERTEX_POINT ( 'NONE', #72668 ) ;
#56689=CARTESIAN_POINT ( 'NONE',  ( 81.02345755814515371, 43.60871490852765930, 9.417864885350642368 ) ) ;
#56693=CARTESIAN_POINT ( 'NONE',  ( 76.27763170702772300, 51.65450477961197606, -16.17713714789237045 ) ) ;
#56694=EDGE_CURVE ( 'NONE', #55385, #92377, #84105, .T. ) ;
#56696=VERTEX_POINT ( 'NONE', #27045 ) ;
#56699=CARTESIAN_POINT ( 'NONE',  ( 85.81778828754448796, 44.78275566574458111, 7.330141423013616375 ) ) ;
#56701=CARTESIAN_POINT ( 'NONE',  ( 77.92825354283080230, 61.79113456967466789, 16.06764011202815823 ) ) ;
#56702=CARTESIAN_POINT ( 'NONE',  ( 79.14312167556931854, 57.64441083166269664, 0.000000000000000000 ) ) ;
#56706=CARTESIAN_POINT ( 'NONE',  ( 36.19122982252199705, 21.86426979415092120, -3.090169943749474069 ) ) ;
#56710=CARTESIAN_POINT ( 'NONE',  ( 37.75683693788968753, 23.92755873383628895, 6.180339887498953466 ) ) ;
#56714=CARTESIAN_POINT ( 'NONE',  ( 84.89389514258827774, 43.37484338261454297, -5.486889282241953048 ) ) ;
#56718=CARTESIAN_POINT ( 'NONE',  ( 81.43924684539796033, 45.70540712647618875, 11.36428502046352307 ) ) ;
#56720=CARTESIAN_POINT ( 'NONE',  ( 86.55741050250372837, 46.28210205434145053, 9.003020896430676601 ) ) ;
#56723=CARTESIAN_POINT ( 'NONE',  ( 82.34816354767144730, 41.40331793722689468, 5.506344658241145495 ) ) ;
#56726=CARTESIAN_POINT ( 'NONE',  ( 43.11943305279750405, 25.86426979415093186, -3.090169943749474069 ) ) ;
#56731=EDGE_CURVE ( 'NONE', #54308, #81557, #56221, .T. ) ;
#56736=CARTESIAN_POINT ( 'NONE',  ( 70.77885289983220218, 66.68069319803313988, -10.82095828200581344 ) ) ;
#56737=CARTESIAN_POINT ( 'NONE',  ( 28.99180842189336005, 40.23654200823203553, 1.583844403245397769 ) ) ;
#56749=CARTESIAN_POINT ( 'NONE',  ( 23.84800118292001159, 31.95586893147756058, 7.433330006724141015 ) ) ;
#56753=VERTEX_POINT ( 'NONE', #89867 ) ;
#56754=CARTESIAN_POINT ( 'NONE',  ( 11.61360469066603507, 28.74646525600389069, 2.839279412974139660 ) ) ;
#56756=CARTESIAN_POINT ( 'NONE',  ( 71.92697733641804803, 72.63665773354594535, -0.7151800694983956319 ) ) ;
#56757=ORIENTED_EDGE ( 'NONE', *, *, #20110, .T. ) ;
#56769=CARTESIAN_POINT ( 'NONE',  ( 72.05747908138206981, 72.41062208079183904, -3.017343731799825512 ) ) ;
#56770=CARTESIAN_POINT ( 'NONE',  ( 72.99661548417863344, 57.62305516421401563, -16.32377903997647550 ) ) ;
#56771=CARTESIAN_POINT ( 'NONE',  ( 78.28473355307382064, 61.06446511097402663, -15.91087495820213427 ) ) ;
#56779=CARTESIAN_POINT ( 'NONE',  ( 33.80247542503471436, 34.91421378149921395, 9.188101187500008038 ) ) ;
#56781=CARTESIAN_POINT ( 'NONE',  ( 78.38442356856859305, 47.88785470443450976, -14.51451505513508877 ) ) ;
#56783=CARTESIAN_POINT ( 'NONE',  ( 73.89028189157257032, 68.56231543382321547, 10.89439152759356944 ) ) ;
#56788=CARTESIAN_POINT ( 'NONE',  ( 77.76107068773923459, 57.49243831483684630, -16.18103606519603588 ) ) ;
#56793=CARTESIAN_POINT ( 'NONE',  ( 68.18719692898707763, 69.37638032551880940, -4.036890616949536437 ) ) ;
#56796=EDGE_CURVE ( 'NONE', #82804, #15274, #1891, .T. ) ;
#56800=CARTESIAN_POINT ( 'NONE',  ( 75.63519723909450931, 65.56940250126960734, 13.79863107474653106 ) ) ;
#56805=CARTESIAN_POINT ( 'NONE',  ( 85.46896714245875160, 44.18043371586173151, -6.563648887624578876 ) ) ;
#56808=EDGE_CURVE ( 'NONE', #19318, #58918, #79161, .T. ) ;
#56812=AXIS2_PLACEMENT_3D ( 'NONE', #13070, #15021, #5452 ) ;
#56813=CARTESIAN_POINT ( 'NONE',  ( 76.08933885469296854, 51.45880163392949669, -15.66904507028006321 ) ) ;
#56815=CARTESIAN_POINT ( 'NONE',  ( 80.65100716643621581, 57.48104863357441729, -16.23842874147667104 ) ) ;
#56822=CARTESIAN_POINT ( 'NONE',  ( 67.72909538816377051, 68.47758282218532599, 5.729597447110076125 ) ) ;
#56831=EDGE_CURVE ( 'NONE', #67005, #52194, #32198, .T. ) ;
#56833=FACE_OUTER_BOUND ( 'NONE', #17564, .T. ) ;
#56838=CARTESIAN_POINT ( 'NONE',  ( 19.65800174957785629, 23.30066082961421969, -10.00000000000000533 ) ) ;
#56839=CARTESIAN_POINT ( 'NONE',  ( 68.34576586436469370, 65.68917945663493185, -10.35820680181607401 ) ) ;
#56840=CARTESIAN_POINT ( 'NONE',  ( 70.62955678152277983, 60.80479719363770386, -15.06269029744276899 ) ) ;
#56854=CARTESIAN_POINT ( 'NONE',  ( 40.42214693012152793, 25.19860640527295104, 2.839279412974134775 ) ) ;
#56856=CARTESIAN_POINT ( 'NONE',  ( 79.14312167556931854, 57.64441083166269664, 0.000000000000000000 ) ) ;
#56857=CARTESIAN_POINT ( 'NONE',  ( 38.69009612255265296, 24.19860640527295104, 2.839279412974134775 ) ) ;
#56864=EDGE_CURVE ( 'NONE', #77944, #24489, #47206, .T. ) ;
#56865=CARTESIAN_POINT ( 'NONE',  ( 8.350964356584899662, 25.79752408145590792, -5.678558825948271327 ) ) ;
#56867=CARTESIAN_POINT ( 'NONE',  ( 11.93836421708519779, 28.93396525600389069, 2.839279412974139660 ) ) ;
#56870=CARTESIAN_POINT ( 'NONE',  ( 84.58308955143566266, 49.89698236725671165, -13.67050406800346707 ) ) ;
#56876=CARTESIAN_POINT ( 'NONE',  ( 87.20396902780147741, 45.40285486062717979, 7.109937478028163227 ) ) ;
#56882=CARTESIAN_POINT ( 'NONE',  ( 86.16320141619598871, 47.68791953076239309, 10.83576430555930514 ) ) ;
#56884=CARTESIAN_POINT ( 'NONE',  ( 78.14700529810005492, 60.07939060848261192, 16.01736686316025171 ) ) ;
#56887=CARTESIAN_POINT ( 'NONE',  ( 78.17184439828042741, 61.78404217785180919, -15.73488545980961106 ) ) ;
#56888=CARTESIAN_POINT ( 'NONE',  ( 83.70979198902698215, 48.81106761220289769, -12.83638129120513582 ) ) ;
#56889=CARTESIAN_POINT ( 'NONE',  ( 80.73218360117679993, 43.11930967842982199, 9.845968670453535410 ) ) ;
#56894=B_SPLINE_CURVE_WITH_KNOTS ( 'NONE', 3,
 ( #37411, #68317, #21241, #12145, #74462, #52118, #8039, #45998, #47517, #77939, #54600, #68814, #93155, #77441, #8529, #16619, #22732, #30827, #70830, #76917, #1441, #15606, #61214, #84568, #94164, #69816, #9024, #39401, #78444, #7515, #70315, #15106, #23211, #63222, #930, #85059, #32321, #428, #16125, #38409, #31315, #76443, #61713, #24716, #93664, #62204 ),
 .UNSPECIFIED., .F., .F.,
 ( 4, 1, 1, 1, 2, 2, 1, 1, 1, 2, 2, 1, 1, 2, 2, 1, 1, 2, 2, 1, 1, 2, 2, 1, 2, 2, 1, 2, 2, 4 ),
 ( 0.000000000000000000, 0.06249999999999045208, 0.09374999999998595568, 0.1093749999999837630, 0.1171874999999826666, 0.1249999999999815703, 0.1874999999999715505, 0.2187499999999681921, 0.2343749999999664990, 0.2421874999999656386, 0.2499999999999647504, 0.3124999999999691358, 0.3437499999999713562, 0.3593749999999705236, 0.3749999999999696909, 0.4374999999999719114, 0.4687499999999726885, 0.4843749999999730771, 0.4999999999999734657, 0.5624999999999801270, 0.5937499999999854561, 0.6093749999999880096, 0.6249999999999906741, 0.6874999999999933387, 0.7187499999999946709, 0.7499999999999960032, 0.8124999999999956701, 0.8437499999999957812, 0.8749999999999958922, 1.000000000000000000 ),
 .UNSPECIFIED. ) ;
#56902=CARTESIAN_POINT ( 'NONE',  ( 66.31795133325435643, 69.20145725284447735, 2.477662600225434719 ) ) ;
#56904=CARTESIAN_POINT ( 'NONE',  ( 83.59128512182542181, 50.22172742876573182, -14.18173862977107902 ) ) ;
#56907=CARTESIAN_POINT ( 'NONE',  ( 69.52914236679859528, 65.28759244955678298, 11.39865997334715253 ) ) ;
#56913=CARTESIAN_POINT ( 'NONE',  ( 20.98529944902502820, 27.51421378149918695, -9.188101187500004485 ) ) ;
#56921=CARTESIAN_POINT ( 'NONE',  ( 15.56473500984127512, 9.390406791769814632, -7.779800476318352071E-15 ) ) ;
#56936=CARTESIAN_POINT ( 'NONE',  ( 82.71170519429942658, 40.59673265032024148, -1.400181599122515497 ) ) ;
#56938=CARTESIAN_POINT ( 'NONE',  ( 19.36651902841724038, 19.38052372038640669, 10.00000000000000533 ) ) ;
#56943=ORIENTED_EDGE ( 'NONE', *, *, #43490, .F. ) ;
#56944=CARTESIAN_POINT ( 'NONE',  ( 74.37117806044521728, 68.42743621588296321, -11.25900170040250003 ) ) ;
#56946=CARTESIAN_POINT ( 'NONE',  ( 83.41573487747820081, 42.76472624850124760, 5.963828435803965711 ) ) ;
#56954=CARTESIAN_POINT ( 'NONE',  ( 82.41745805622035448, 43.86099032315292590, 8.743768202596600148 ) ) ;
#56967=( BOUNDED_CURVE ( )  B_SPLINE_CURVE ( 2, ( #90862, #4730, #97438, #11836, #44191, #58885, #28008, #66018, #88892, #43193, #42695, #73626, #21414 ),
 .UNSPECIFIED., .F., .T. ) 
 B_SPLINE_CURVE_WITH_KNOTS ( ( 3, 2, 2, 2, 2, 2, 3 ),
 ( 0.2374999999999999889, 0.2399999999999999911, 0.2449999999999999956, 0.2500000000000000000, 0.2550000000000000044, 0.2600000000000000089, 0.2625000000000000111 ),
 .UNSPECIFIED. ) 
 CURVE ( )  GEOMETRIC_REPRESENTATION_ITEM ( )  RATIONAL_B_SPLINE_CURVE ( ( 0.9755282581475768211, 0.9755282581475768211, 1.000000000000000000, 0.9510565162951535312, 1.000000000000000000, 0.9510565162951535312, 1.000000000000000000, 0.9510565162951535312, 1.000000000000000000, 0.9510565162951535312, 1.000000000000000000, 0.9755282581475768211, 0.9755282581475768211 ) ) 
 REPRESENTATION_ITEM ( '' )  );
#56971=CARTESIAN_POINT ( 'NONE',  ( 27.11361191214091804, 16.44966523072495335, -2.296566073217252530E-15 ) ) ;
#56972=CARTESIAN_POINT ( 'NONE',  ( 75.24247008381291835, 66.93257772500234637, 12.82047627203052009 ) ) ;
#56981=CARTESIAN_POINT ( 'NONE',  ( 82.35643665848068906, 41.29992738147394959, -3.430024729213354107 ) ) ;
#56982=CARTESIAN_POINT ( 'NONE',  ( 32.88524308553003550, 19.39040679176984838, -6.890680421881970419E-14 ) ) ;
#56983=CARTESIAN_POINT ( 'NONE',  ( 81.77662633183955165, 55.53141904912255455, -15.95577929170707066 ) ) ;
#56986=VECTOR ( 'NONE', #42052, 1000.000000000000000 ) ;
#56989=CARTESIAN_POINT ( 'NONE',  ( 71.92106615665200309, 72.60175000959986846, 1.189886861346824753 ) ) ;
#56993=LINE ( 'NONE', #72229, #9706 ) ;
#56997=CARTESIAN_POINT ( 'NONE',  ( 8.323093432028223049, 20.50829794293878905, -10.00000000000000355 ) ) ;
#57009=DIRECTION ( 'NONE',  ( 0.06958655048003267729, -0.1205274409548735270, -0.9902680687415703620 ) ) ;
#57010=CARTESIAN_POINT ( 'NONE',  ( 81.95257519206566599, 50.72568879219577553, -14.43282536261877524 ) ) ;
#57011=CARTESIAN_POINT ( 'NONE',  ( 73.27328646083023500, 70.16270934360544231, -9.274526489422589393 ) ) ;
#57018=LINE ( 'NONE', #35226, #35270 ) ;
#57020=CARTESIAN_POINT ( 'NONE',  ( 88.33249819345715537, 44.18347584668511985, -0.1457987645956864697 ) ) ;
#57021=CARTESIAN_POINT ( 'NONE',  ( 79.20956237034324943, 53.22039654841660195, 15.72328171560790189 ) ) ;
#57023=CARTESIAN_POINT ( 'NONE',  ( 82.33552489548483777, 41.24829604067362254, 3.267574154620816795 ) ) ;
#57028=CARTESIAN_POINT ( 'NONE',  ( 77.71695824120644147, 49.45779813244274692, 15.33409790704233799 ) ) ;
#57031=CARTESIAN_POINT ( 'NONE',  ( 70.73063444094617580, 61.07312936796083847, -14.44582943987787260 ) ) ;
#57032=CARTESIAN_POINT ( 'NONE',  ( 45.41683807177152232, 29.14754757982093736, -5.678558825948276656 ) ) ;
#57033=ORIENTED_EDGE ( 'NONE', *, *, #33961, .T. ) ;
#57040=DIRECTION ( 'NONE',  ( -0.1710100716628374096, 0.2961981327260301833, 0.9396926207859057634 ) ) ;
#57049=CARTESIAN_POINT ( 'NONE',  ( 36.94473716931751284, 21.73415679381824361, -6.890680421881970419E-14 ) ) ;
#57050=CARTESIAN_POINT ( 'NONE',  ( 66.22544434996629548, 69.36168404795429865, 0.1681498104656474202 ) ) ;
#57059=CARTESIAN_POINT ( 'NONE',  ( 87.99156517466562377, 44.25173956186072388, 2.816193757564026789 ) ) ;
#57063=CARTESIAN_POINT ( 'NONE',  ( 74.05886703568846485, 66.92701276778755926, 12.81588082616969970 ) ) ;
#57068=CARTESIAN_POINT ( 'NONE',  ( 80.69702293635484125, 43.52605551489090630, -9.543807321698503543 ) ) ;
#57074=CARTESIAN_POINT ( 'NONE',  ( 88.15573124791052351, 44.39703741701313078, -4.524867680024764915 ) ) ;
#57085=CARTESIAN_POINT ( 'NONE',  ( 74.41491511734228936, 56.32654587899735077, -16.10167882689214025 ) ) ;
#57086=CARTESIAN_POINT ( 'NONE',  ( 83.53204454370724363, 52.39401912150450613, -15.17729711222452416 ) ) ;
#57087=CARTESIAN_POINT ( 'NONE',  ( 73.30631488696991482, 69.89686749726290316, 9.630897265116471928 ) ) ;
#57093=CARTESIAN_POINT ( 'NONE',  ( 84.13355168651825977, 43.02656781755162996, -6.806181843193294334 ) ) ;
#57096=ADVANCED_FACE ( 'NONE', ( #79663 ), #26920, .T. ) ;
#57097=CARTESIAN_POINT ( 'NONE',  ( 78.58115897284257301, 49.46449540821208757, -15.15569606598211116 ) ) ;
#57098=CARTESIAN_POINT ( 'NONE',  ( 76.15623579681398780, 64.25551128800826461, 14.96979677531604480 ) ) ;
#57100=CARTESIAN_POINT ( 'NONE',  ( 18.92609651878039756, 19.43085787977762280, -9.188101187500008038 ) ) ;
#57108=CARTESIAN_POINT ( 'NONE',  ( 70.34454795187326681, 61.29844696719631969, 14.78467410917921043 ) ) ;
#57119=CARTESIAN_POINT ( 'NONE',  ( 72.67454777811306599, 57.54427597285661022, -16.30613687664699896 ) ) ;
#57120=CARTESIAN_POINT ( 'NONE',  ( 77.26942776676457925, 63.03888086361324383, -15.26992705839576381 ) ) ;
#57127=CARTESIAN_POINT ( 'NONE',  ( 41.30863684418880410, 35.80066082961425167, 10.00000000000000533 ) ) ;
#57128=CARTESIAN_POINT ( 'NONE',  ( 36.43182450750799006, 23.96004757982092315, -5.678558825948275768 ) ) ;
#57129=CARTESIAN_POINT ( 'NONE',  ( 79.76833976871120058, 44.78188551475517443, 11.36349263846995328 ) ) ;
#57130=CARTESIAN_POINT ( 'NONE',  ( 84.29414043670328738, 48.06250324931478701, -12.02348180207343020 ) ) ;
#57133=EDGE_CURVE ( 'NONE', #86000, #92701, #98424, .T. ) ;
#57136=VERTEX_POINT ( 'NONE', #21799 ) ;
#57147=DIRECTION ( 'NONE',  ( 0.06958655048003267729, -0.1205274409548735270, -0.9902680687415703620 ) ) ;
#57152=ORIENTED_EDGE ( 'NONE', *, *, #39324, .T. ) ;
#57154=EDGE_CURVE ( 'NONE', #16006, #31346, #91258, .T. ) ;
#57155=CARTESIAN_POINT ( 'NONE',  ( 80.32594557099248789, 44.72898953253431387, -11.70945978744232363 ) ) ;
#57167=EDGE_CURVE ( 'NONE', #16883, #35964, #55665, .T. ) ;
#57173=CARTESIAN_POINT ( 'NONE',  ( 87.93413682123004094, 44.35120838780621000, 4.768703809423659123 ) ) ;
#57174=EDGE_LOOP ( 'NONE', ( #16778, #35943, #193, #5311, #79168, #58306, #73469, #61757, #9819, #81629, #40177, #95563, #94218, #28601, #99621, #16169, #67371, #54437, #83726, #95351, #19100, #43855, #7403, #97930, #17986, #50456, #40787, #63227, #48291, #9085, #62468, #88989, #99052, #25889 ) ) ;
#57176=EDGE_CURVE ( 'NONE', #59093, #53284, #33924, .T. ) ;
#57180=CARTESIAN_POINT ( 'NONE',  ( 80.72100776821309864, 43.43651575216833294, 9.420844811674243147 ) ) ;
#57183=CARTESIAN_POINT ( 'NONE',  ( 77.58957552442460326, 61.75793702469097468, 15.67560070342385892 ) ) ;
#57186=CARTESIAN_POINT ( 'NONE',  ( 86.40663024008399873, 45.92652238299617551, 8.627225980297390961 ) ) ;
#57187=CARTESIAN_POINT ( 'NONE',  ( 16.27523747222386774, 28.13478043621388025, 8.090169943749478065 ) ) ;
#57188=CARTESIAN_POINT ( 'NONE',  ( 83.24496396852070745, 52.35953078789503934, 14.85683903734107147 ) ) ;
#57191=CARTESIAN_POINT ( 'NONE',  ( 27.78891098193510345, 37.81751292744058190, -6.180339887498951690 ) ) ;
#57193=CARTESIAN_POINT ( 'NONE',  ( 73.88036207731340710, 64.05502917650269978, -13.99130931570255143 ) ) ;
#57195=CARTESIAN_POINT ( 'NONE',  ( 74.19373413002220730, 55.14634173073913814, 16.60422751163261879 ) ) ;
#57197=CARTESIAN_POINT ( 'NONE',  ( 29.87413333957346140, 40.18080186712595747, 3.090169943749475401 ) ) ;
#57202=CARTESIAN_POINT ( 'NONE',  ( 84.10129132598619606, 43.29379949965990448, -6.284272029605274312 ) ) ;
#57206=CARTESIAN_POINT ( 'NONE',  ( 82.79565879694258967, 50.14544268168955199, 13.93210848370866373 ) ) ;
#57209=CARTESIAN_POINT ( 'NONE',  ( 87.13721241349922764, 46.29175778497492644, 8.541777034186077699 ) ) ;
#57211=CARTESIAN_POINT ( 'NONE',  ( 71.92697733641804803, 72.63665773354594535, -0.7151800694983956319 ) ) ;
#57214=CARTESIAN_POINT ( 'NONE',  ( 87.15721324309708962, 46.06501070407752252, 8.877681887861816890 ) ) ;
#57216=CARTESIAN_POINT ( 'NONE',  ( 32.98506340464173547, 40.81751292744058901, -6.180339887498951690 ) ) ;
#57234=CARTESIAN_POINT ( 'NONE',  ( 67.03286369130589151, 67.01141394008774910, -8.665391638908033656 ) ) ;
#57239=CARTESIAN_POINT ( 'NONE',  ( 33.71705561599726053, 20.26216523072496045, -2.296566073217252530E-15 ) ) ;
#57243=VERTEX_POINT ( 'NONE', #58182 ) ;
#57244=CARTESIAN_POINT ( 'NONE',  ( 10.42942532566755354, 26.99752408145591076, 5.678558825948276656 ) ) ;
#57248=EDGE_CURVE ( 'NONE', #86732, #4961, #85161, .T. ) ;
#57250=CARTESIAN_POINT ( 'NONE',  ( 72.13998692144450331, 71.54377819717346654, -5.860361805407116265 ) ) ;
#57254=CARTESIAN_POINT ( 'NONE',  ( 73.09674767720407829, 64.62968492494913164, -13.92540306414895745 ) ) ;
#57255=EDGE_LOOP ( 'NONE', ( #45443, #40436, #37355, #93997 ) ) ;
#57260=VERTEX_POINT ( 'NONE', #82032 ) ;
#57261=CARTESIAN_POINT ( 'NONE',  ( 65.92723761077292011, 68.94945291078158789, -2.624861927977415021 ) ) ;
#57263=CARTESIAN_POINT ( 'NONE',  ( 71.08765421117847438, 71.69956734233102225, -3.661842409509368235 ) ) ;
#57264=CARTESIAN_POINT ( 'NONE',  ( 78.18520617608054124, 61.02381034122267067, -15.90742658069108728 ) ) ;
#57272=VERTEX_POINT ( 'NONE', #12608 ) ;
#57273=CARTESIAN_POINT ( 'NONE',  ( 38.53854167689037524, 24.11110640527295246, -2.839279412974138328 ) ) ;
#57275=CARTESIAN_POINT ( 'NONE',  ( 78.51822142034139063, 47.92457381461660049, -14.49495123615230519 ) ) ;
#57277=CARTESIAN_POINT ( 'NONE',  ( 73.77070425341645432, 68.39923094797843817, 11.48015304846416029 ) ) ;
#57282=ORIENTED_EDGE ( 'NONE', *, *, #35314, .T. ) ;
#57285=CARTESIAN_POINT ( 'NONE',  ( 80.00759052209035360, 56.61424376545486581, -16.17082543645087256 ) ) ;
#57293=VECTOR ( 'NONE', #92766, 1000.000000000000114 ) ;
#57301=EDGE_CURVE ( 'NONE', #2820, #53182, #40434, .T. ) ;
#57303=ORIENTED_EDGE ( 'NONE', *, *, #60320, .F. ) ;
#57304=CARTESIAN_POINT ( 'NONE',  ( 82.35638529324310753, 44.23013856389444953, -9.288241028977028080 ) ) ;
#57305=CARTESIAN_POINT ( 'NONE',  ( 84.91096221446015591, 42.98959058816011947, 4.352075159545532479 ) ) ;
#57312=CARTESIAN_POINT ( 'NONE',  ( 80.46835216585913031, 57.85139773374410055, -16.60023610630909019 ) ) ;
#57319=CARTESIAN_POINT ( 'NONE',  ( 68.61230155682829945, 69.51726337545549939, 4.400640945930509140 ) ) ;
#57323=CARTESIAN_POINT ( 'NONE',  ( 18.52134341065869805, 22.64441083166260427, -10.00000000000000533 ) ) ;
#57330=CARTESIAN_POINT ( 'NONE',  ( 83.49981249572846309, 50.92614816156454083, -14.12294194579210682 ) ) ;
#57333=CARTESIAN_POINT ( 'NONE',  ( 66.57729162794665001, 67.76982667965772578, -7.017260695426948303 ) ) ;
#57338=CARTESIAN_POINT ( 'NONE',  ( 23.89366908878298190, 14.76426979415089846, 3.090169943749476733 ) ) ;
#57341=CARTESIAN_POINT ( 'NONE',  ( 72.22168947570742148, 72.04854175159199769, -3.193460859968826782 ) ) ;
#57343=CARTESIAN_POINT ( 'NONE',  ( 74.07743547874019896, 55.48756474711195352, -16.11625136640599365 ) ) ;
#57354=CARTESIAN_POINT ( 'NONE',  ( 42.32740281844729680, 26.29860640527295601, -2.839279412974138328 ) ) ;
#57357=CARTESIAN_POINT ( 'NONE',  ( 29.25887229277395463, 38.93396525600392266, 2.839279412974139660 ) ) ;
#57364=( NAMED_UNIT ( * ) SI_UNIT ( $, .STERADIAN. ) SOLID_ANGLE_UNIT ( ) );
#57365=CARTESIAN_POINT ( 'NONE',  ( 12.55777956335723644, 9.111106405272902720, -2.839279412974138328 ) ) ;
#57367=CARTESIAN_POINT ( 'NONE',  ( 19.08966579672462416, 13.94754757982089011, 5.678558825948272215 ) ) ;
#57379=CARTESIAN_POINT ( 'NONE',  ( 87.43576499144317893, 45.00137247461035628, 6.922634181320205471 ) ) ;
#57381=ORIENTED_EDGE ( 'NONE', *, *, #36249, .T. ) ;
#57384=CARTESIAN_POINT ( 'NONE',  ( 86.41183189003805865, 47.25727891775800771, 10.78350007392548271 ) ) ;
#57386=CARTESIAN_POINT ( 'NONE',  ( 77.07529298142445384, 54.05291532172810776, 16.01725459708226751 ) ) ;
#57390=CARTESIAN_POINT ( 'NONE',  ( 88.52345208173723279, 43.89072024811925843, -0.4439432684152969100 ) ) ;
#57391=CARTESIAN_POINT ( 'NONE',  ( 81.74377432616384453, 48.00429482119757552, -13.52050817838834895 ) ) ;
#57392=CARTESIAN_POINT ( 'NONE',  ( 80.55884490112875085, 43.45966037107459812, 9.562419172017994740 ) ) ;
#57393=ORIENTED_EDGE ( 'NONE', *, *, #71624, .T. ) ;
#57397=ORIENTED_EDGE ( 'NONE', *, *, #93120, .T. ) ;
#57403=ORIENTED_EDGE ( 'NONE', *, *, #98727, .T. ) ;
#57413=CARTESIAN_POINT ( 'NONE',  ( 24.98947064339976265, 26.37878583063841731, 9.188101187500006262 ) ) ;
#57416=CARTESIAN_POINT ( 'NONE',  ( 85.46847960764181096, 42.12007198895852156, -0.3052117524058582942 ) ) ;
#57422=CARTESIAN_POINT ( 'NONE',  ( 44.43605786102924782, 27.78380873178790722, -6.180339887498949025 ) ) ;
#57430=CARTESIAN_POINT ( 'NONE',  ( 81.65310433048475147, 42.64019311979919280, 7.560891536010023728 ) ) ;
#57444=CARTESIAN_POINT ( 'NONE',  ( 80.89292881529833323, 46.87624008130001840, -12.53476188675516134 ) ) ;
#57447=EDGE_CURVE ( 'NONE', #42575, #43244, #23519, .T. ) ;
#57450=CARTESIAN_POINT ( 'NONE',  ( 74.14322651144246379, 67.86457474202013884, -11.65196598083728041 ) ) ;
#57454=CARTESIAN_POINT ( 'NONE',  ( 83.24352937575713440, 45.45189662214414028, 10.11960700973886951 ) ) ;
#57457=CARTESIAN_POINT ( 'NONE',  ( 68.49429924950833026, 64.43582602095906964, -12.25658928467158049 ) ) ;
#57467=B_SPLINE_CURVE_WITH_KNOTS ( 'NONE', 3,
 ( #40115, #70024, #69534, #85280, #55314, #92866, #63930, #46212, #71054, #15826, #1656, #33030, #38624, #94869, #71554, #56322, #32541, #87316, #94373, #46729, #24928, #31519, #77657, #77131 ),
 .UNSPECIFIED., .F., .F.,
 ( 4, 2, 2, 2, 2, 2, 2, 2, 2, 2, 2, 4 ),
 ( 0.000000000000000000, 0.1249999999999977240, 0.2499999999999954481, 0.3749999999999931721, 0.4374999999999883427, 0.4999999999999834577, 0.5624999999999785727, 0.6249999999999736877, 0.6874999999999686917, 0.7499999999999638067, 0.8749999999999820144, 1.000000000000000000 ),
 .UNSPECIFIED. ) ;
#57468=CARTESIAN_POINT ( 'NONE',  ( 84.27717094892697958, 45.26462376842967217, 9.982582507191876786 ) ) ;
#57470=CARTESIAN_POINT ( 'NONE',  ( 21.91745948943428601, 13.44966523072494269, -2.296566073217252530E-15 ) ) ;
#57471=CARTESIAN_POINT ( 'NONE',  ( 74.89568429962641005, 67.14399892254596125, 12.98700472788359406 ) ) ;
#57473=CARTESIAN_POINT ( 'NONE',  ( 81.78504375891562006, 41.48292696562020865, -5.073134180756075473 ) ) ;
#57482=CARTESIAN_POINT ( 'NONE',  ( 74.31929878905869202, 64.95657537261109837, -14.11942355924862014 ) ) ;
#57483=CARTESIAN_POINT ( 'NONE',  ( 25.79892497710874366, 15.86426979415090166, -3.090169943749474069 ) ) ;
#57485=CARTESIAN_POINT ( 'NONE',  ( 71.90360357134964886, 72.59530952775406831, 1.145984468326242789 ) ) ;
#57487=CARTESIAN_POINT ( 'NONE',  ( 77.71695824127769470, 49.45779813231933986, 15.33409790721217369 ) ) ;
#57492=CARTESIAN_POINT ( 'NONE',  ( 71.99762221142530905, 71.50039512193581004, -5.770478025556951884 ) ) ;
#57497=CARTESIAN_POINT ( 'NONE',  ( 42.15722797529793553, 32.84335787977767041, 9.188101187500006262 ) ) ;
#57500=B_SPLINE_CURVE_WITH_KNOTS ( 'NONE', 3,
 ( #57473, #19522, #51889, #28081, #82830, #88456, #75200, #19015, #11908, #66089 ),
 .UNSPECIFIED., .F., .F.,
 ( 4, 2, 2, 2, 4 ),
 ( 0.000000000000000000, 0.2500000000000000000, 0.5000000000000000000, 0.7500000000000000000, 1.000000000000000000 ),
 .UNSPECIFIED. ) ;
#57512=CARTESIAN_POINT ( 'NONE',  ( 78.74619901529338506, 51.78797505174686933, -15.41928803356502264 ) ) ;
#57513=CARTESIAN_POINT ( 'NONE',  ( 84.49829320381432751, 49.81850184317473662, -13.23518311421627125 ) ) ;
#57521=CARTESIAN_POINT ( 'NONE',  ( 74.75863154782773279, 57.63597024813910252, 16.00019208182263597 ) ) ;
#57525=CARTESIAN_POINT ( 'NONE',  ( 81.90913890621609994, 41.07391263979702245, 3.568215028523603394 ) ) ;
#57529=DIRECTION ( 'NONE',  ( -0.4145187862775162602, 0.7179675985244458047, -0.5591929034707565638 ) ) ;
#57531=CARTESIAN_POINT ( 'NONE',  ( 72.73940707191790978, 68.18235160057777478, -10.56708786553003065 ) ) ;
#57533=CARTESIAN_POINT ( 'NONE',  ( 70.82864487769981565, 61.11463513126617642, -14.45246479568451825 ) ) ;
#57536=CARTESIAN_POINT ( 'NONE',  ( 85.33699565288863198, 48.33901173460944278, -12.30238903177781395 ) ) ;
#57540=CARTESIAN_POINT ( 'NONE',  ( 76.18525949220615701, 64.77142460697901072, -14.35656184529598711 ) ) ;
#57546=CARTESIAN_POINT ( 'NONE',  ( 83.68679791621119080, 41.62673357145322228, 0.2031610672272064766 ) ) ;
#57547=CARTESIAN_POINT ( 'NONE',  ( 88.15760586300541490, 44.17367696878018535, -1.747427669005709117 ) ) ;
#57551=CARTESIAN_POINT ( 'NONE',  ( 66.25373396628860689, 68.82734845049694172, 0.1167526145283954014 ) ) ;
#57560=CARTESIAN_POINT ( 'NONE',  ( 88.24872265415196182, 44.28890599193383792, 2.074108197446814739 ) ) ;
#57568=LINE ( 'NONE', #88542, #66300 ) ;
#57569=( BOUNDED_CURVE ( )  B_SPLINE_CURVE ( 2, ( #93772, #529, #72454, #3060, #19256, #49619, #42992, #80572, #50122, #88685, #97255, #88187, #11150 ),
 .UNSPECIFIED., .F., .T. ) 
 B_SPLINE_CURVE_WITH_KNOTS ( ( 3, 2, 2, 2, 2, 2, 3 ),
 ( 0.3125000000000000000, 0.3150000000000000022, 0.3200000000000000067, 0.3250000000000000111, 0.3300000000000000155, 0.3350000000000000200, 0.3375000000000000222 ),
 .UNSPECIFIED. ) 
 CURVE ( )  GEOMETRIC_REPRESENTATION_ITEM ( )  RATIONAL_B_SPLINE_CURVE ( ( 0.9755282581475768211, 0.9755282581475768211, 1.000000000000000000, 0.9510565162951535312, 1.000000000000000000, 0.9510565162951535312, 1.000000000000000000, 0.9510565162951535312, 1.000000000000000000, 0.9510565162951535312, 1.000000000000000000, 0.9755282581475768211, 0.9755282581475768211 ) ) 
 REPRESENTATION_ITEM ( '' )  );
#57576=CARTESIAN_POINT ( 'NONE',  ( 88.19119485691749105, 44.51220553762047416, -4.804906155116626110 ) ) ;
#57578=EDGE_CURVE ( 'NONE', #62365, #71177, #17481, .T. ) ;
#57580=CARTESIAN_POINT ( 'NONE',  ( 76.92873890057782660, 49.89429371730488327, 15.13083596839045519 ) ) ;
#57585=CARTESIAN_POINT ( 'NONE',  ( 76.93595106450065657, 55.49016027357946257, -16.15734999971556007 ) ) ;
#57591=CARTESIAN_POINT ( 'NONE',  ( 73.05674748647940930, 57.23263728894347935, 15.90451911058029744 ) ) ;
#57595=CARTESIAN_POINT ( 'NONE',  ( 75.62238463899576857, 65.35737373615053514, 14.30258955018443601 ) ) ;
#57598=CARTESIAN_POINT ( 'NONE',  ( 27.72828276626169952, 36.98502408145593989, -5.678558825948271327 ) ) ;
#57600=CARTESIAN_POINT ( 'NONE',  ( 84.33507765194615047, 46.83375941775653217, -10.92698133767611779 ) ) ;
#57602=CARTESIAN_POINT ( 'NONE',  ( 19.52749640002317122, 16.98920272979925628, 7.433330006724137462 ) ) ;
#57609=CARTESIAN_POINT ( 'NONE',  ( 86.18930939419189485, 47.16029689842823558, 10.81535065263619622 ) ) ;
#57614=CARTESIAN_POINT ( 'NONE',  ( 85.35443477132466228, 48.30880629543902671, -11.80360700664790663 ) ) ;
#57623=CARTESIAN_POINT ( 'NONE',  ( 76.95433588952691650, 62.91899607007382400, -15.24877360450729036 ) ) ;
#57630=CARTESIAN_POINT ( 'NONE',  ( 25.29680607046014984, 36.64646525600391413, -2.839279412974133887 ) ) ;
#57641=CARTESIAN_POINT ( 'NONE',  ( 85.76547152072677704, 48.63404149359708128, -11.87225177386112485 ) ) ;
#57649=EDGE_LOOP ( 'NONE', ( #1751, #51688, #48439, #25366 ) ) ;
#57651=DIRECTION ( 'NONE',  ( -0.8660254037844377084, -0.5000000000000014433, -0.000000000000000000 ) ) ;
#57653=ORIENTED_EDGE ( 'NONE', *, *, #88378, .F. ) ;
#57655=CARTESIAN_POINT ( 'NONE',  ( 86.90364953904725098, 45.87765456670206277, -8.164248709133197224 ) ) ;
#57656=CARTESIAN_POINT ( 'NONE',  ( 71.40026156493414078, 59.28187485775010401, 15.24249285347964289 ) ) ;
#57665=EDGE_LOOP ( 'NONE', ( #39552, #37309, #14642, #62749, #51149, #35450 ) ) ;
#57666=CARTESIAN_POINT ( 'NONE',  ( 75.95690509902382814, 65.20561023377018728, -14.47468716891346219 ) ) ;
#57675=ORIENTED_EDGE ( 'NONE', *, *, #15902, .F. ) ;
#57676=CARTESIAN_POINT ( 'NONE',  ( 86.04035583496818163, 43.88013096475103225, -5.118424826341424705 ) ) ;
#57686=CARTESIAN_POINT ( 'NONE',  ( 79.29854305342225018, 47.63708018034404290, 13.57368722073299239 ) ) ;
#57687=CARTESIAN_POINT ( 'NONE',  ( 70.36141869169587437, 70.50703831449676784, -4.583400824472941615 ) ) ;
#57689=CARTESIAN_POINT ( 'NONE',  ( 78.07729254143889364, 61.93885312825283052, 15.69741212657180540 ) ) ;
#57694=CARTESIAN_POINT ( 'NONE',  ( 71.00220796100531118, 64.77528057016907326, -12.50717593332708866 ) ) ;
#57697=CARTESIAN_POINT ( 'NONE',  ( 31.86369474034375671, 37.13478043621390157, 8.090169943749478065 ) ) ;
#57698=CARTESIAN_POINT ( 'NONE',  ( 77.93902080370800434, 47.95641163770635274, 14.13009455829524796 ) ) ;
#57701=AXIS2_PLACEMENT_3D ( 'NONE', #28254, #57651, #58640 ) ;
#57702=CARTESIAN_POINT ( 'NONE',  ( 83.66935810104509130, 43.26081338140035371, -6.695904667356427531 ) ) ;
#57706=CARTESIAN_POINT ( 'NONE',  ( 86.89976093607516816, 45.97909969559822940, 8.962991326411129833 ) ) ;
#57708=CARTESIAN_POINT ( 'NONE',  ( 82.19706587503785045, 41.28416451854318581, 5.427054723112330059 ) ) ;
#57712=CARTESIAN_POINT ( 'NONE',  ( 34.30168821287347924, 42.73705186507756792, -3.090169943749475845 ) ) ;
#57720=CARTESIAN_POINT ( 'NONE',  ( 83.70690788325238429, 51.99575818335755883, 14.97781791391902750 ) ) ;
#57722=CARTESIAN_POINT ( 'NONE',  ( 75.48012123268173923, 53.33211347945791658, 16.49774674168797617 ) ) ;
#57728=CARTESIAN_POINT ( 'NONE',  ( 67.11837730215745523, 67.11470315592687541, -8.588528573970526381 ) ) ;
#57729=EDGE_CURVE ( 'NONE', #66666, #11364, #80327, .T. ) ;
#57734=CARTESIAN_POINT ( 'NONE',  ( 30.72569264534336142, 26.24335787977765122, -9.188101187500008038 ) ) ;
#57736=CARTESIAN_POINT ( 'NONE',  ( 86.53129273504272589, 47.24044952787517104, -10.15552464530777854 ) ) ;
#57741=CARTESIAN_POINT ( 'NONE',  ( 12.86511499041763074, 19.37878583063839244, 9.188101187500006262 ) ) ;
#57748=CARTESIAN_POINT ( 'NONE',  ( 72.32024965620544776, 71.13684411087814397, -6.061350040765782765 ) ) ;
#57761=CARTESIAN_POINT ( 'NONE',  ( 72.80719422333380919, 57.61781679197407868, -16.30664549720600931 ) ) ;
#57762=CARTESIAN_POINT ( 'NONE',  ( 78.37369994444134136, 61.17973184547403775, -15.89768920957586751 ) ) ;
#57772=CARTESIAN_POINT ( 'NONE',  ( 37.04286019156342746, 27.10170272979929607, -7.433330006724141015 ) ) ;
#57774=CARTESIAN_POINT ( 'NONE',  ( 75.24181145021050554, 66.45540672401639881, -13.14705475788992040 ) ) ;
#57785=LINE ( 'NONE', #96338, #69030 ) ;
#57786=CARTESIAN_POINT ( 'NONE',  ( 67.27025623861466386, 69.09150813649328882, -3.041265173945424838 ) ) ;
#57789=CARTESIAN_POINT ( 'NONE',  ( 80.09487356998278074, 52.84115226274354171, 15.95029973925667832 ) ) ;
#57791=EDGE_CURVE ( 'NONE', #72450, #36817, #93592, .T. ) ;
#57798=CARTESIAN_POINT ( 'NONE',  ( 84.55722348921307230, 44.16439880798394313, -7.444406649127180309 ) ) ;
#57803=CARTESIAN_POINT ( 'NONE',  ( 75.21950657921868810, 63.51667331280388851, 14.62111120148422394 ) ) ;
#57812=EDGE_CURVE ( 'NONE', #61768, #84261, #620, .T. ) ;
#57820=CARTESIAN_POINT ( 'NONE',  ( 21.28706459136418871, 17.45404122711133255, -8.090169943749478065 ) ) ;
#57828=CARTESIAN_POINT ( 'NONE',  ( 76.56471838561475352, 53.17383487477179926, -15.93209607857030008 ) ) ;
#57829=ORIENTED_EDGE ( 'NONE', *, *, #21052, .T. ) ;
#57835=CARTESIAN_POINT ( 'NONE',  ( 25.62571989635185332, 15.76426979415090202, 3.090169943749476733 ) ) ;
#57839=CARTESIAN_POINT ( 'NONE',  ( 72.01037534753049840, 72.25474680761037405, -3.568257732133948590 ) ) ;
#57841=CARTESIAN_POINT ( 'NONE',  ( 73.92320082988518948, 55.40069282120870042, -16.11615024270321328 ) ) ;
#57844=CARTESIAN_POINT ( 'NONE',  ( 76.01760950601774880, 55.66421313266628346, 16.60722370189778019 ) ) ;
#57845=CARTESIAN_POINT ( 'NONE',  ( 23.79565599918673158, 37.23654200823203553, 1.583844403245397769 ) ) ;
#57850=LINE ( 'NONE', #42639, #27998 ) ;
#57854=CARTESIAN_POINT ( 'NONE',  ( 33.90715327291019321, 42.68290643055189548, 3.479690158560446702E-15 ) ) ;
#57857=CARTESIAN_POINT ( 'NONE',  ( 33.43441462842632461, 34.70171378149921537, -9.188101187500004485 ) ) ;
#57862=CARTESIAN_POINT ( 'NONE',  ( 41.47628181354097165, 29.11029122506297995, -8.090169943749478065 ) ) ;
#57865=CARTESIAN_POINT ( 'NONE',  ( 12.18311320154372801, 9.960047579820882291, -5.678558825948276656 ) ) ;
#57866=CARTESIAN_POINT ( 'NONE',  ( 71.90400658755810070, 72.53437165389429708, 1.750395423964758557 ) ) ;
#57867=CARTESIAN_POINT ( 'NONE',  ( 16.80672687576512203, 25.10171378149917842, 9.188101187500008038 ) ) ;
#57879=CARTESIAN_POINT ( 'NONE',  ( 66.27858692599893686, 68.56926275514072699, 4.816128439524981708 ) ) ;
#57886=VERTEX_POINT ( 'NONE', #29745 ) ;
#57891=ORIENTED_EDGE ( 'NONE', *, *, #57578, .T. ) ;
#57893=CARTESIAN_POINT ( 'NONE',  ( 77.74234477000247523, 50.56326866554580590, -15.20697261137338074 ) ) ;
#57895=CARTESIAN_POINT ( 'NONE',  ( 81.28922747573520269, 43.24881869083999675, 9.615907131230160942 ) ) ;
#57899=AXIS2_PLACEMENT_3D ( 'NONE', #18046, #26635, #79878 ) ;
#57901=VERTEX_POINT ( 'NONE', #23121 ) ;
#57919=LINE ( 'NONE', #10836, #60923 ) ;
#57920=CARTESIAN_POINT ( 'NONE',  ( 22.11595037535113661, 30.95586893147756413, 7.433330006724141015 ) ) ;
#57929=B_SPLINE_CURVE_WITH_KNOTS ( 'NONE', 3,
 ( #29977, #71991, #55745, #1084, #39052, #78089, #93309, #25374, #48691, #77596, #69964, #41055, #79626, #17791, #31962, #54758, #92808, #86235, #93822, #32482, #87258, #86737, #71497, #2596, #8183, #23866, #579, #10189, #31463, #85744, #9701 ),
 .UNSPECIFIED., .F., .F.,
 ( 4, 3, 3, 3, 3, 3, 3, 3, 3, 3, 4 ),
 ( 0.000000000000000000, 0.1333490885032357909, 0.3007194338854210502, 0.4699862290245036545, 0.5844252810809178467, 0.6686540514502550270, 0.7354980260655467061, 0.8028463152565693539, 0.8633854507757410257, 0.9437142632667440134, 1.000000000000000000 ),
 .UNSPECIFIED. ) ;
#57931=DIRECTION ( 'NONE',  ( -0.4755282581475737680, 0.8236391035463299648, -0.3090169943749573878 ) ) ;
#57942=CARTESIAN_POINT ( 'NONE',  ( 12.26669281485430929, 30.58029201028040944, 1.583844403245363353 ) ) ;
#57955=PLANE ( 'NONE',  #90407 ) ;
#57960=CARTESIAN_POINT ( 'NONE',  ( 79.32558605478153879, 59.69129752972263248, -16.52184683405510768 ) ) ;
#57966=CARTESIAN_POINT ( 'NONE',  ( 72.73269248836916745, 71.16345857084107251, -7.307540741686426422 ) ) ;
#57971=CARTESIAN_POINT ( 'NONE',  ( 74.17788031095660983, 67.68212350510704312, -12.30096152613073279 ) ) ;
#57973=CARTESIAN_POINT ( 'NONE',  ( 68.93032405664872897, 67.85419375520189078, 8.166185397134730906 ) ) ;
#57975=VERTEX_POINT ( 'NONE', #69231 ) ;
#57981=CARTESIAN_POINT ( 'NONE',  ( 20.11807774711229868, 23.56628583063840665, 9.188101187500006262 ) ) ;
#57982=CARTESIAN_POINT ( 'NONE',  ( 75.25170673533752108, 66.73598490943447814, 12.94887977284632363 ) ) ;
#57994=CARTESIAN_POINT ( 'NONE',  ( 81.59924320624311633, 55.92250459863397083, -16.38315390958105766 ) ) ;
#57995=VERTEX_POINT ( 'NONE', #40316 ) ;
#57997=CARTESIAN_POINT ( 'NONE',  ( 80.56131375285130503, 46.02381187782341243, 12.65584631694679274 ) ) ;
#57998=EDGE_CURVE ( 'NONE', #91452, #184, #96081, .T. ) ;
#57999=CARTESIAN_POINT ( 'NONE',  ( 84.27505121841375058, 43.30459200202938064, 6.061470481410601074 ) ) ;
#58002=CARTESIAN_POINT ( 'NONE',  ( 72.01497877597556396, 71.50364303677275757, -5.786257741033058011 ) ) ;
#58007=CARTESIAN_POINT ( 'NONE',  ( 10.72711477659875534, 18.14441083166259361, 10.00000000000000533 ) ) ;
#58017=CARTESIAN_POINT ( 'NONE',  ( 74.99511382823338579, 53.05528727595338978, -16.49829891682232486 ) ) ;
#58022=CARTESIAN_POINT ( 'NONE',  ( 79.94457760174631744, 51.39983459170911573, -15.10834372778664658 ) ) ;
#58028=ORIENTED_EDGE ( 'NONE', *, *, #6422, .F. ) ;
#58031=CARTESIAN_POINT ( 'NONE',  ( 75.56522282763701526, 61.49378516209786483, 15.36079468230518685 ) ) ;
#58035=LINE ( 'NONE', #48947, #88654 ) ;
#58036=CARTESIAN_POINT ( 'NONE',  ( 80.73992981690828685, 43.57577410340355328, -9.572596457172796391 ) ) ;
#58039=EDGE_CURVE ( 'NONE', #40944, #76398, #58035, .T. ) ;
#58044=CARTESIAN_POINT ( 'NONE',  ( 70.52664859635549988, 61.35291825783819064, -14.80704222503500844 ) ) ;
#58045=CARTESIAN_POINT ( 'NONE',  ( 8.350964356584899662, 25.79752408145590792, -5.678558825948271327 ) ) ;
#58046=VECTOR ( 'NONE', #38214, 1000.000000000000114 ) ;
#58049=CARTESIAN_POINT ( 'NONE',  ( 85.48848937474792820, 48.32878387211594884, -12.22513733614603559 ) ) ;
#58052=CARTESIAN_POINT ( 'NONE',  ( 78.23198182499388054, 47.91966744817526092, -14.02533881450480813 ) ) ;
#58058=CARTESIAN_POINT ( 'NONE',  ( 88.09265120180700137, 44.13139543698701317, -1.715510155970429995 ) ) ;
#58062=CARTESIAN_POINT ( 'NONE',  ( 66.45864018013874386, 68.94716056944170646, 0.01924691867824903160 ) ) ;
#58070=CARTESIAN_POINT ( 'NONE',  ( 88.13736778048858866, 44.32197654044805546, 2.735995528162057155 ) ) ;
#58075=CARTESIAN_POINT ( 'NONE',  ( 77.75329651808065989, 60.51879551299917637, -15.90944513805293425 ) ) ;
#58077=ADVANCED_FACE ( 'NONE', ( #4853 ), #11746, .T. ) ;
#58078=CARTESIAN_POINT ( 'NONE',  ( 70.80625596290352064, 66.10710362255882444, -11.37769121604388367 ) ) ;
#58081=CARTESIAN_POINT ( 'NONE',  ( 80.61734525203304713, 43.35833479104773147, -9.401381521366195315 ) ) ;
#58086=CARTESIAN_POINT ( 'NONE',  ( 87.63170318219839316, 44.36446170533410793, -4.079950490519348882 ) ) ;
#58088=LINE ( 'NONE', #41886, #94969 ) ;
#58092=CARTESIAN_POINT ( 'NONE',  ( 84.40121558736829854, 50.67993577924135451, 13.77038979431789123 ) ) ;
#58093=CARTESIAN_POINT ( 'NONE',  ( 79.23610557255210551, 54.64639511583943232, -15.99020243353516868 ) ) ;
#58095=EDGE_CURVE ( 'NONE', #46807, #39534, #76721, .T. ) ;
#58106=CARTESIAN_POINT ( 'NONE',  ( 27.52682148520507965, 37.93396525600392266, 2.839279412974139660 ) ) ;
#58107=CARTESIAN_POINT ( 'NONE',  ( 80.55977923466276991, 44.53388773495298381, 11.41474457630165062 ) ) ;
#58108=CARTESIAN_POINT ( 'NONE',  ( 75.82019069382886300, 62.35695433681328126, 15.58349134701113670 ) ) ;
#58110=CARTESIAN_POINT ( 'NONE',  ( 19.41443888993109823, 32.18502408145592852, 5.678558825948277544 ) ) ;
#58115=CARTESIAN_POINT ( 'NONE',  ( 86.17334730086119521, 47.14257514812162952, 10.80675504988608715 ) ) ;
#58116=CARTESIAN_POINT ( 'NONE',  ( 74.42628153207887465, 62.65944167963375122, 15.19835750912931971 ) ) ;
#58121=CARTESIAN_POINT ( 'NONE',  ( 25.25549177415142310, 22.78052372038641238, -10.00000000000000355 ) ) ;
#58122=VERTEX_POINT ( 'NONE', #28129 ) ;
#58124=EDGE_LOOP ( 'NONE', ( #17574, #5575, #89898, #40330 ) ) ;
#58126=CARTESIAN_POINT ( 'NONE',  ( 81.53115339410010165, 41.92267797703283350, -7.515177224638171616 ) ) ;
#58127=EDGE_LOOP ( 'NONE', ( #4980, #86018, #87491, #64763 ) ) ;
#58128=CARTESIAN_POINT ( 'NONE',  ( 85.47913374364790684, 42.62622548008751266, 0.2499991700750583967 ) ) ;
#58130=CARTESIAN_POINT ( 'NONE',  ( 71.99267133948018227, 71.58944556433895912, 5.550980660130552913 ) ) ;
#58133=CARTESIAN_POINT ( 'NONE',  ( 88.09812594050896450, 44.33653194584124435, -4.440584375772045789 ) ) ;
#58137=CARTESIAN_POINT ( 'NONE',  ( 27.91350267930052809, 31.51421378149921182, -9.188101187500004485 ) ) ;
#58138=CARTESIAN_POINT ( 'NONE',  ( 72.40300161649089716, 60.75817645194375416, -14.95975737059987409 ) ) ;
#58142=ORIENTED_EDGE ( 'NONE', *, *, #9427, .T. ) ;
#58144=CARTESIAN_POINT ( 'NONE',  ( 68.28786865650171478, 65.57955037385437436, 10.43542532682454649 ) ) ;
#58146=CARTESIAN_POINT ( 'NONE',  ( 85.46201571263348740, 48.63304775035897620, 12.47391791266364791 ) ) ;
#58160=CARTESIAN_POINT ( 'NONE',  ( 87.04446681553140763, 45.94690404971670716, -8.147129491944053115 ) ) ;
#58161=CARTESIAN_POINT ( 'NONE',  ( 71.71749174456839171, 59.03106295208012710, 15.36370853995013697 ) ) ;
#58166=VERTEX_POINT ( 'NONE', #60502 ) ;
#58173=CARTESIAN_POINT ( 'NONE',  ( 29.97214642916971883, 17.70852965304480264, 1.583844403245330712 ) ) ;
#58174=CARTESIAN_POINT ( 'NONE',  ( 70.49515160751757037, 69.39311819046854168, -7.234649680376111114 ) ) ;
#58180=EDGE_LOOP ( 'NONE', ( #19026, #75134, #47728, #94220, #17915, #80592, #45763, #16664, #51273, #62543, #21187, #64369, #16171, #64790, #29854, #14763, #47304, #30392, #75867, #89754, #71964, #98594, #43946, #88487, #98854, #1842, #15390, #63630, #40235, #56190, #90373, #26278, #95084, #40716, #24127, #96761, #77655, #8217, #22285, #3659, #5543, #8083, #98543, #93240 ) ) ;
#58182=CARTESIAN_POINT ( 'NONE',  ( 82.29734961797252879, 53.60383310410945512, 15.81226994477779790 ) ) ;
#58183=CARTESIAN_POINT ( 'NONE',  ( 82.19743676121389342, 40.60779097105204727, -3.273795677556531114 ) ) ;
#58186=ADVANCED_FACE ( 'NONE', ( #22019 ), #98553, .T. ) ;
#58192=CARTESIAN_POINT ( 'NONE',  ( 80.38896062813260812, 51.85953464289088544, 15.18891967833937962 ) ) ;
#58194=EDGE_CURVE ( 'NONE', #82635, #23145, #51429, .T. ) ;
#58196=CARTESIAN_POINT ( 'NONE',  ( 78.13090640523601849, 61.76054338150410672, 16.10053832301867871 ) ) ;
#58199=EDGE_CURVE ( 'NONE', #90841, #27648, #46336, .T. ) ;
#58201=CARTESIAN_POINT ( 'NONE',  ( 80.13399453211208368, 44.22126075786002275, -11.35348423903955783 ) ) ;
#58203=CARTESIAN_POINT ( 'NONE',  ( 10.72711477659875534, 18.14441083166259361, 10.00000000000000533 ) ) ;
#58205=CARTESIAN_POINT ( 'NONE',  ( 38.41907791167486153, 30.38052372038643867, 10.00000000000000533 ) ) ;
#58209=CARTESIAN_POINT ( 'NONE',  ( 86.54608540568763431, 43.64951324792490084, -3.608069729097785672 ) ) ;
#58213=CARTESIAN_POINT ( 'NONE',  ( 86.94335770270596697, 46.00923847012510493, 8.969699243401572986 ) ) ;
#58215=CARTESIAN_POINT ( 'NONE',  ( 71.72615628857761294, 72.05106317348395351, -1.629725736277438441 ) ) ;
#58219=CARTESIAN_POINT ( 'NONE',  ( 40.62554608437772430, 25.58380873178790083, 6.180339887498953466 ) ) ;
#58228=CARTESIAN_POINT ( 'NONE',  ( 34.38043361391329711, 31.80066082961424812, 10.00000000000000533 ) ) ;
#58235=CARTESIAN_POINT ( 'NONE',  ( 67.41728548999284953, 66.73849313723850685, -8.451184109718100856 ) ) ;
#58239=CARTESIAN_POINT ( 'NONE',  ( 72.11270410251323426, 62.11537045185059469, 14.87459164730639571 ) ) ;
#58240=CARTESIAN_POINT ( 'NONE',  ( 34.69977369993912220, 22.96004757982091959, -5.678558825948276656 ) ) ;
#58242=CARTESIAN_POINT ( 'NONE',  ( 86.30036054584773808, 46.98594781855085500, -10.02878425733469037 ) ) ;
#58243=EDGE_CURVE ( 'NONE', #74723, #27875, #39684, .T. ) ;
#58246=CARTESIAN_POINT ( 'NONE',  ( 11.44039960990914651, 28.64646525600389282, -2.839279412974133887 ) ) ;
#58250=ORIENTED_EDGE ( 'NONE', *, *, #81125, .T. ) ;
#58251=CARTESIAN_POINT ( 'NONE',  ( 77.50334873148125325, 59.55703387409915450, 16.42230352199692689 ) ) ;
#58256=ORIENTED_EDGE ( 'NONE', *, *, #35572, .T. ) ;
#58261=CARTESIAN_POINT ( 'NONE',  ( 66.07636532461724244, 68.52392620069937834, -2.382434824416819641 ) ) ;
#58263=LINE ( 'NONE', #13672, #24050 ) ;
#58264=CARTESIAN_POINT ( 'NONE',  ( 78.39570488777410162, 61.38734676664308409, -15.85619035535652799 ) ) ;
#58265=ADVANCED_FACE ( 'NONE', ( #61512 ), #7825, .T. ) ;
#58275=CARTESIAN_POINT ( 'NONE',  ( 32.50825522076439000, 36.95586893147758190, 7.433330006724141015 ) ) ;
#58284=CARTESIAN_POINT ( 'NONE',  ( 71.24387660651150611, 63.97505982078597953, -13.10960455195070473 ) ) ;
#58285=CARTESIAN_POINT ( 'NONE',  ( 88.28592015977814356, 44.16006502160688996, -0.2344584660017056954 ) ) ;
#58286=CARTESIAN_POINT ( 'NONE',  ( 66.16089386745949241, 68.65346719215108351, -4.358124916883920008 ) ) ;
#58289=CARTESIAN_POINT ( 'NONE',  ( 72.36856322112618045, 69.84542717626317199, -8.279172892043805021 ) ) ;
#58292=CARTESIAN_POINT ( 'NONE',  ( 79.84223750413882215, 51.63136904638950853, 15.66302827892303995 ) ) ;
#58294=DIRECTION ( 'NONE',  ( 0.9669094993746140121, -0.2551196190400366048, 0.000000000000000000 ) ) ;
#58299=CARTESIAN_POINT ( 'NONE',  ( 85.35694830404344202, 44.17699873431174495, -6.675819990932985171 ) ) ;
#58306=ORIENTED_EDGE ( 'NONE', *, *, #30455, .T. ) ;
#58307=CARTESIAN_POINT ( 'NONE',  ( 76.93992332084131647, 56.94179084800790491, 16.18160332842839466 ) ) ;
#58318=CARTESIAN_POINT ( 'NONE',  ( 21.79139015901366960, 20.78052372038640883, -10.00000000000000355 ) ) ;
#58333=CARTESIAN_POINT ( 'NONE',  ( 18.81282613181931040, 26.56454794089041727, 10.00000000000000355 ) ) ;
#58334=CARTESIAN_POINT ( 'NONE',  ( 88.12195951149128348, 43.65269896049575493, 0.1370767085644954975 ) ) ;
#58336=CARTESIAN_POINT ( 'NONE',  ( 72.03933155393818311, 72.41131128147422658, -2.965003495713515402 ) ) ;
#58338=CARTESIAN_POINT ( 'NONE',  ( 74.15479259495415931, 55.62765001672816823, -16.59030973361144845 ) ) ;
#58341=CARTESIAN_POINT ( 'NONE',  ( 75.17267702473046143, 67.05865199424735579, 12.71180004614658365 ) ) ;
#58349=CARTESIAN_POINT ( 'NONE',  ( 79.43361010913639575, 59.55165593117043699, 16.18183685357123736 ) ) ;
#58350=CARTESIAN_POINT ( 'NONE',  ( 38.86330120330953974, 24.29860640527295246, -2.839279412974138328 ) ) ;
#58351=CARTESIAN_POINT ( 'NONE',  ( 17.74301629803562363, 32.01751292744056343, 6.180339887498949913 ) ) ;
#58357=CARTESIAN_POINT ( 'NONE',  ( 14.28983037092611319, 10.11110640527290627, -2.839279412974138328 ) ) ;
#58359=CARTESIAN_POINT ( 'NONE',  ( 21.77916244986271366, 18.28920272979926764, -7.433330006724141015 ) ) ;
#58361=ADVANCED_FACE ( 'NONE', ( #49435 ), #15822, .T. ) ;
#58365=CARTESIAN_POINT ( 'NONE',  ( 75.13576154535616070, 53.51470238525797640, -16.05299128471374814 ) ) ;
#58370=CARTESIAN_POINT ( 'NONE',  ( 82.34753025084647504, 40.38730442864357428, 1.410118989783748278 ) ) ;
#58371=CARTESIAN_POINT ( 'NONE',  ( 66.15678826669763168, 68.52882108677162876, 4.729996398140529301 ) ) ;
#58372=CARTESIAN_POINT ( 'NONE',  ( 87.37622458635497935, 44.94434973981048387, 6.879737256407628010 ) ) ;
#58374=ORIENTED_EDGE ( 'NONE', *, *, #49148, .T. ) ;
#58379=CARTESIAN_POINT ( 'NONE',  ( 80.47734257382147405, 57.78184453145892263, -16.59809864164601478 ) ) ;
#58385=CARTESIAN_POINT ( 'NONE',  ( 81.05763270389508079, 43.67158023151815627, 9.470390458390101074 ) ) ;
#58396=ORIENTED_EDGE ( 'NONE', *, *, #82939, .T. ) ;
#58409=CARTESIAN_POINT ( 'NONE',  ( 73.22055517253131995, 58.28100772285806386, -15.76052744220302770 ) ) ;
#58412=CARTESIAN_POINT ( 'NONE',  ( 85.23385146218150510, 41.99429442906141929, -0.6099763831586285656 ) ) ;
#58417=CARTESIAN_POINT ( 'NONE',  ( 83.08655343033629492, 51.67706410362837488, -14.60604715524620367 ) ) ;
#58429=CARTESIAN_POINT ( 'NONE',  ( 82.74024154138081144, 40.61182045439817756, -1.385978721574811834 ) ) ;
#58438=CARTESIAN_POINT ( 'NONE',  ( 71.94643353573427191, 71.53214566342799685, 5.625104812542565114 ) ) ;
#58441=ADVANCED_FACE ( 'NONE', ( #31475 ), #20678, .T. ) ;
#58444=DIRECTION ( 'NONE',  ( -0.4330127018922203530, 0.7500000000000046629, 0.4999999999999919509 ) ) ;
#58455=CARTESIAN_POINT ( 'NONE',  ( 79.20094478699866158, 45.83966577849356838, -12.45917745233390406 ) ) ;
#58459=CARTESIAN_POINT ( 'NONE',  ( 71.31959007138432582, 71.35434536779762027, 3.842738600495782197 ) ) ;
#58461=( BOUNDED_CURVE ( )  B_SPLINE_CURVE ( 2, ( #69450, #76091, #60831, #14261, #7145, #84208, #69941, #54228, #39032, #7652, #53735, #22851, #83196 ),
 .UNSPECIFIED., .F., .T. ) 
 B_SPLINE_CURVE_WITH_KNOTS ( ( 3, 2, 2, 2, 2, 2, 3 ),
 ( 0.08750000000000000833, 0.08999999999999999667, 0.09500000000000000111, 0.1000000000000000056, 0.1049999999999999961, 0.1100000000000000006, 0.1125000000000000028 ),
 .UNSPECIFIED. ) 
 CURVE ( )  GEOMETRIC_REPRESENTATION_ITEM ( )  RATIONAL_B_SPLINE_CURVE ( ( 0.9755282581475768211, 0.9755282581475768211, 1.000000000000000000, 0.9510565162951535312, 1.000000000000000000, 0.9510565162951535312, 1.000000000000000000, 0.9510565162951535312, 1.000000000000000000, 0.9510565162951535312, 1.000000000000000000, 0.9755282581475768211, 0.9755282581475768211 ) ) 
 REPRESENTATION_ITEM ( '' )  );
#58465=CARTESIAN_POINT ( 'NONE',  ( 84.53133730985203442, 45.87904168161020380, 10.50013902873333471 ) ) ;
#58467=CARTESIAN_POINT ( 'NONE',  ( 22.87854050506884462, 34.18502408145592852, 5.678558825948277544 ) ) ;
#58471=CARTESIAN_POINT ( 'NONE',  ( 75.15246256102729205, 67.05878861674010238, 13.14576163508979434 ) ) ;
#58472=CARTESIAN_POINT ( 'NONE',  ( 11.62691283633230377, 30.21091486745859811, -1.111400068045478839E-16 ) ) ;
#58480=CARTESIAN_POINT ( 'NONE',  ( 70.00968539685798930, 68.79935913217504151, 7.688938106457000821 ) ) ;
#58482=CARTESIAN_POINT ( 'NONE',  ( 71.66539077729500207, 72.47145342129385881, 0.9585255015204302564 ) ) ;
#58483=CARTESIAN_POINT ( 'NONE',  ( 77.55198886215855225, 49.72190584956302217, 14.94683709150641349 ) ) ;
#58485=B_SPLINE_CURVE_WITH_KNOTS ( 'NONE', 3,
 ( #6858, #8365, #69150, #83910, #39232, #70140, #15436, #752, #46334, #24054, #7867, #258, #16451, #70652, #61042, #100079, #30668, #93999, #31636, #39723, #77258, #92493, #23039, #38746, #69651, #31140, #62536, #93496, #54949, #47349, #14473, #79314, #57444, #86925, #80302, #56453, #96498, #48366, #9882, #2278, #10370, #49854, #34651, #94493, #71684, #42242 ),
 .UNSPECIFIED., .F., .F.,
 ( 4, 1, 2, 2, 1, 2, 2, 1, 1, 2, 2, 1, 1, 2, 2, 1, 1, 2, 2, 1, 1, 1, 2, 2, 1, 1, 1, 2, 2, 4 ),
 ( 0.000000000000000000, 0.06250000000000428824, 0.09375000000000484335, 0.1250000000000054123, 0.1875000000000069111, 0.2187500000000092426, 0.2500000000000115463, 0.3125000000000164868, 0.3437500000000191513, 0.3593750000000205946, 0.3750000000000220379, 0.4375000000000278666, 0.4687500000000291989, 0.4843750000000298095, 0.5000000000000303091, 0.5625000000000234257, 0.5937500000000196509, 0.6093750000000160982, 0.6250000000000124345, 0.6875000000000081046, 0.7187500000000074385, 0.7343750000000071054, 0.7421875000000066613, 0.7500000000000061062, 0.8124999999999911182, 0.8437499999999836797, 0.8593749999999802380, 0.8671874999999783507, 0.8749999999999764633, 1.000000000000000000 ),
 .UNSPECIFIED. ) ;
#58487=DIRECTION ( 'NONE',  ( -0.1039558454088829048, 0.1800568059919617214, 0.9781476007338041345 ) ) ;
#58491=CARTESIAN_POINT ( 'NONE',  ( 12.43831579814173693, 15.38052372038639248, 10.00000000000000533 ) ) ;
#58492=CARTESIAN_POINT ( 'NONE',  ( 81.75404519488073163, 42.76199632323480415, 8.646050847852000842 ) ) ;
#58499=CARTESIAN_POINT ( 'NONE',  ( 78.91446233654380649, 59.71533271261715470, 16.49719907270642238 ) ) ;
#58500=DIRECTION ( 'NONE',  ( -0.8660254037844377084, -0.5000000000000014433, -0.000000000000000000 ) ) ;
#58506=CARTESIAN_POINT ( 'NONE',  ( 84.48836950856804151, 49.89909654526366722, -13.70430404532020319 ) ) ;
#58510=VERTEX_POINT ( 'NONE', #58764 ) ;
#58517=LINE ( 'NONE', #89489, #28350 ) ;
#58520=CARTESIAN_POINT ( 'NONE',  ( 82.19410048901978882, 40.72072028018710199, 3.734475190160377434 ) ) ;
#58528=CARTESIAN_POINT ( 'NONE',  ( 76.00843876396085363, 56.26865137601856048, 16.15028453724080393 ) ) ;
#58529=CARTESIAN_POINT ( 'NONE',  ( 5.233272902960924178, 23.99752408145590010, 5.678558825948277544 ) ) ;
#58536=CARTESIAN_POINT ( 'NONE',  ( 76.27092524855413558, 64.92237886744916864, -14.30682806216622360 ) ) ;
#58540=CARTESIAN_POINT ( 'NONE',  ( 86.03189311092296521, 43.36316420155662144, 3.487833995403543774 ) ) ;
#58541=CARTESIAN_POINT ( 'NONE',  ( 88.41107184461979784, 44.00353577411875960, -2.298891457252526749 ) ) ;
#58542=ORIENTED_EDGE ( 'NONE', *, *, #67322, .F. ) ;
#58545=CARTESIAN_POINT ( 'NONE',  ( 65.77405155218870902, 69.10179338945289373, 0.09299488885824654105 ) ) ;
#58560=CARTESIAN_POINT ( 'NONE',  ( 72.27428605645289394, 62.29733430174115227, -14.32261433990752941 ) ) ;
#58562=CARTESIAN_POINT ( 'NONE',  ( 80.19866971488238505, 58.11932589254354298, 16.26542142913219635 ) ) ;
#58564=FACE_OUTER_BOUND ( 'NONE', #46803, .T. ) ;
#58566=CARTESIAN_POINT ( 'NONE',  ( 80.72225415553992889, 43.55209726595803943, -9.557057607487440265 ) ) ;
#58572=AXIS2_PLACEMENT_3D ( 'NONE', #35471, #94944, #43567 ) ;
#58576=CARTESIAN_POINT ( 'NONE',  ( 84.51504024060453446, 50.21520769139153373, 13.87897165174792846 ) ) ;
#58578=CARTESIAN_POINT ( 'NONE',  ( 79.36263291408793918, 45.67866562566761957, -12.88899626193393821 ) ) ;
#58585=CARTESIAN_POINT ( 'NONE',  ( 86.02614724684285363, 42.97974342575955120, -1.241900217485796931 ) ) ;
#58586=CARTESIAN_POINT ( 'NONE',  ( 75.59035046094346910, 65.27760725598233194, 14.33377162271303185 ) ) ;
#58588=CARTESIAN_POINT ( 'NONE',  ( 30.66313333631612892, 33.10171378149921395, 9.188101187500008038 ) ) ;
#58592=CARTESIAN_POINT ( 'NONE',  ( 26.36427918851389407, 18.14754757982090894, -5.678558825948276656 ) ) ;
#58593=CARTESIAN_POINT ( 'NONE',  ( 11.86377311551791358, 18.80066082961420548, 10.00000000000000533 ) ) ;
#58597=CARTESIAN_POINT ( 'NONE',  ( 70.40814973419489320, 60.99421022303731377, 14.40290003289568510 ) ) ;
#58599=CARTESIAN_POINT ( 'NONE',  ( 72.30023906772009923, 71.55035954458072922, 5.049600667910633334 ) ) ;
#58602=CARTESIAN_POINT ( 'NONE',  ( 74.77656783286164455, 53.42788812744306881, 16.06606871515787205 ) ) ;
#58603=EDGE_LOOP ( 'NONE', ( #93346, #27162, #12579, #80920 ) ) ;
#58604=CARTESIAN_POINT ( 'NONE',  ( 80.01176385998078899, 46.97566021387115143, -13.51455718187173716 ) ) ;
#58608=CARTESIAN_POINT ( 'NONE',  ( 85.52743691353181532, 43.19076203672399572, 3.962637686270520376 ) ) ;
#58610=CARTESIAN_POINT ( 'NONE',  ( 85.97353089263540937, 42.92677418585991234, 0.9306074700887760898 ) ) ;
#58612=EDGE_CURVE ( 'NONE', #31579, #2203, #33087, .T. ) ;
#58613=CARTESIAN_POINT ( 'NONE',  ( 72.21801880702699350, 71.73430858976985292, 5.514776891874389797 ) ) ;
#58615=DIRECTION ( 'NONE',  ( -0.8660254037844378194, -0.5000000000000014433, -0.000000000000000000 ) ) ;
#58616=CARTESIAN_POINT ( 'NONE',  ( 87.93946558867349950, 44.22841546557597781, -4.388681702043145449 ) ) ;
#58617=CARTESIAN_POINT ( 'NONE',  ( 83.80885942164384517, 50.03953058205711102, 14.02354566334989094 ) ) ;
#58619=CARTESIAN_POINT ( 'NONE',  ( 27.31210279805776509, 33.95586893147756768, 7.433330006724141015 ) ) ;
#58620=CARTESIAN_POINT ( 'NONE',  ( 71.85117389033869983, 60.90190494782929420, -14.78537330145037032 ) ) ;
#58622=EDGE_CURVE ( 'NONE', #31579, #50345, #76492, .T. ) ;
#58623=CARTESIAN_POINT ( 'NONE',  ( 87.21028088194235295, 45.40991956565691368, 7.116430392365408863 ) ) ;
#58627=CARTESIAN_POINT ( 'NONE',  ( 81.13146525994932290, 42.42342676164043525, 7.700666981504315167 ) ) ;
#58628=CARTESIAN_POINT ( 'NONE',  ( 84.41999685182091184, 50.11946239824889915, 13.85565564441014708 ) ) ;
#58631=CARTESIAN_POINT ( 'NONE',  ( 85.77117071415351290, 48.61266522586591776, 12.32040783412941920 ) ) ;
#58634=CYLINDRICAL_SURFACE ( 'NONE', #3196, 16.60714546451156792 ) ;
#58637=CARTESIAN_POINT ( 'NONE',  ( 78.98760635313000478, 59.78900401997537273, 16.49402793498109077 ) ) ;
#58640=DIRECTION ( 'NONE',  ( 0.5000000000000013323, -0.8660254037844378194, 0.000000000000000000 ) ) ;
#58642=ORIENTED_EDGE ( 'NONE', *, *, #87242, .T. ) ;
#58645=VERTEX_POINT ( 'NONE', #63272 ) ;
#58646=CARTESIAN_POINT ( 'NONE',  ( 87.19094985451131663, 46.20751697815333614, -8.392937380860479024 ) ) ;
#58649=B_SPLINE_SURFACE_WITH_KNOTS ( 'NONE', 3, 1, ( 
 ( #34679, #57982 ),
 ( #95032, #9906 ),
 ( #95550, #26098 ),
 ( #86952, #11416 ),
 ( #17485, #56972 ),
 ( #2307, #87470 ),
 ( #79832, #25596 ),
 ( #49887, #87957 ),
 ( #33188, #18005 ),
 ( #80333, #56482 ),
 ( #10902, #25077 ),
 ( #10399, #41777 ),
 ( #72723, #3314 ),
 ( #41268, #34194 ),
 ( #65085, #26597 ),
 ( #57471, #88454 ),
 ( #50379, #80846 ),
 ( #42270, #48393 ),
 ( #88965, #73203 ),
 ( #65581, #19519 ),
 ( #96529, #81332 ),
 ( #42761, #73693 ),
 ( #4277, #35177 ),
 ( #66087, #55957 ),
 ( #79336, #46718 ),
 ( #1648, #8231 ),
 ( #23916, #39598 ),
 ( #93870, #77646 ),
 ( #94365, #33532 ),
 ( #64429, #86283 ),
 ( #39099, #78644 ) ),
 .UNSPECIFIED., .F., .F., .F.,
 ( 4, 3, 3, 3, 3, 3, 3, 3, 3, 3, 4 ),
 ( 2, 2 ),
 ( 0.000000000000000000, 0.1333490885032276307, 0.3007194338854349835, 0.4699862290245034879, 0.5844252810809318355, 0.6686540514502756771, 0.7354980260655390456, 0.8028463152565503691, 0.8633854507757023899, 0.9437142632666907227, 1.000000000000000000 ),
 ( 0.000000000000000000, 1.000000000000000000 ),
 .UNSPECIFIED. ) ;
#58661=CARTESIAN_POINT ( 'NONE',  ( 82.20451920363863962, 44.49317834911897052, 9.706292511583995974 ) ) ;
#58663=CARTESIAN_POINT ( 'NONE',  ( 69.77715862259884716, 62.22749446745734758, -13.61937327518938723 ) ) ;
#58665=ORIENTED_EDGE ( 'NONE', *, *, #55084, .F. ) ;
#58667=CARTESIAN_POINT ( 'NONE',  ( 71.59914813136816747, 63.10835605410795779, 13.72820954599041166 ) ) ;
#58668=CARTESIAN_POINT ( 'NONE',  ( 81.98951371156157109, 41.06142891364449099, -3.326342120204745623 ) ) ;
#58672=CARTESIAN_POINT ( 'NONE',  ( 76.03251232036760143, 51.31991947663375697, -16.13754705453489180 ) ) ;
#58675=CARTESIAN_POINT ( 'NONE',  ( 79.34578826044543121, 47.78602306556283708, 13.64286931921999368 ) ) ;
#58677=CARTESIAN_POINT ( 'NONE',  ( 24.82038151633537026, 14.73415679381822230, 1.333680081654574804E-15 ) ) ;
#58678=CARTESIAN_POINT ( 'NONE',  ( 77.75702407734982557, 61.66006977308100545, 16.07490810555907146 ) ) ;
#58682=CARTESIAN_POINT ( 'NONE',  ( 69.00782751094600087, 70.34284141419077230, -1.981107559596647860 ) ) ;
#58683=DIRECTION ( 'NONE',  ( 0.8660254037844377084, 0.5000000000000015543, 0.000000000000000000 ) ) ;
#58685=CARTESIAN_POINT ( 'NONE',  ( 36.37119629183458613, 23.12755873383628114, -6.180339887498949025 ) ) ;
#58686=CARTESIAN_POINT ( 'NONE',  ( 75.66122109319597655, 57.70107486379740180, -16.51614346280108947 ) ) ;
#58689=CARTESIAN_POINT ( 'NONE',  ( 82.69282291038285848, 43.21275928182573267, -7.572188776693871581 ) ) ;
#58692=CARTESIAN_POINT ( 'NONE',  ( 69.04267406240978744, 70.00324579014528581, 5.266832899270860402 ) ) ;
#58694=B_SPLINE_CURVE_WITH_KNOTS ( 'NONE', 3,
 ( #68011, #75625, #6212, #76142 ),
 .UNSPECIFIED., .F., .F.,
 ( 4, 4 ),
 ( 0.000000000000000000, 0.1555655374897298437 ),
 .UNSPECIFIED. ) ;
#58695=CARTESIAN_POINT ( 'NONE',  ( 86.86399242946149002, 45.94634269538593685, 8.946615921987719489 ) ) ;
#58697=CARTESIAN_POINT ( 'NONE',  ( 72.10465435074424079, 72.28376592976228210, -1.461586084520088091 ) ) ;
#58700=CARTESIAN_POINT ( 'NONE',  ( 86.80989918712758424, 45.87808919071956382, 8.896275332294523608 ) ) ;
#58703=CARTESIAN_POINT ( 'NONE',  ( 7.127696690345725727, 16.06628583063839244, -9.188101187500006262 ) ) ;
#58713=CARTESIAN_POINT ( 'NONE',  ( 81.90189478934432543, 58.86607563204950822, -0.3830222215594885626 ) ) ;
#58720=CARTESIAN_POINT ( 'NONE',  ( 67.44257088933083821, 67.25355904253446226, -8.657396272464442433 ) ) ;
#58726=CARTESIAN_POINT ( 'NONE',  ( 29.48198420892518357, 37.99752408145594273, 5.678558825948277544 ) ) ;
#58731=CARTESIAN_POINT ( 'NONE',  ( 68.49108285301745980, 64.31732535079238744, 12.34849984288629976 ) ) ;
#58735=CARTESIAN_POINT ( 'NONE',  ( 77.68610095332765297, 61.14218577032889357, 16.17973444202652189 ) ) ;
#58746=ORIENTED_EDGE ( 'NONE', *, *, #3463, .T. ) ;
#58747=CARTESIAN_POINT ( 'NONE',  ( 66.50139985668020870, 68.79878299985570322, -2.191674848154488764 ) ) ;
#58748=EDGE_CURVE ( 'NONE', #42933, #34456, #4486, .T. ) ;
#58751=CARTESIAN_POINT ( 'NONE',  ( 78.14988184308933228, 61.89697373328141339, -16.07278474554906467 ) ) ;
#58752=ADVANCED_FACE ( 'NONE', ( #25269 ), #71894, .T. ) ;
#58757=ORIENTED_EDGE ( 'NONE', *, *, #48139, .F. ) ;
#58762=CARTESIAN_POINT ( 'NONE',  ( 75.30635741883537548, 66.56121636111578255, -13.10152444272999617 ) ) ;
#58764=CARTESIAN_POINT ( 'NONE',  ( 28.28448313147312021, 16.73415679381822585, 1.333680081654574804E-15 ) ) ;
#58765=CARTESIAN_POINT ( 'NONE',  ( 81.90070505019525626, 55.28399500932853528, 16.25061773925407493 ) ) ;
#58769=CARTESIAN_POINT ( 'NONE',  ( 69.32120137048818265, 64.30962851660092383, -12.08911290385783488 ) ) ;
#58782=EDGE_LOOP ( 'NONE', ( #11346, #42264, #4820, #29376, #99246, #24031 ) ) ;
#58783=CARTESIAN_POINT ( 'NONE',  ( 82.57684337742131220, 44.21772893957315631, -9.119279311071077032 ) ) ;
#58784=CARTESIAN_POINT ( 'NONE',  ( 85.77746269900303844, 44.00077978609508023, 5.766797212797135863 ) ) ;
#58786=CARTESIAN_POINT ( 'NONE',  ( 79.36123937160471087, 59.78439649202068296, -16.16115984811566264 ) ) ;
#58787=CARTESIAN_POINT ( 'NONE',  ( 75.44622636097695079, 64.91049876765895021, 14.07243495672977929 ) ) ;
#58790=CARTESIAN_POINT ( 'NONE',  ( 77.17013742012716193, 58.35697113532116731, 16.12913492606394428 ) ) ;
#58792=AXIS2_PLACEMENT_3D ( 'NONE', #5906, #83442, #36796 ) ;
#58793=CARTESIAN_POINT ( 'NONE',  ( 72.63051688559265529, 71.46180251613422740, -5.713833537422692288 ) ) ;
#58804=CARTESIAN_POINT ( 'NONE',  ( 24.66226663818958187, 15.20801979619928979, -3.090169943749474069 ) ) ;
#58809=CARTESIAN_POINT ( 'NONE',  ( 72.18990340680744566, 72.03918383723207342, -3.149060597287207219 ) ) ;
#58819=CARTESIAN_POINT ( 'NONE',  ( 23.98812876850004727, 25.80066082961422325, 10.00000000000000533 ) ) ;
#58820=CARTESIAN_POINT ( 'NONE',  ( 85.56715572150820037, 48.66046822832736041, 12.44852408270450184 ) ) ;
#58822=CARTESIAN_POINT ( 'NONE',  ( 72.09461912472968947, 72.35512880999853280, -3.358616764072534178 ) ) ;
#58823=CARTESIAN_POINT ( 'NONE',  ( 74.04272560325144070, 55.47781366761107336, -16.11579405751482241 ) ) ;
#58832=CARTESIAN_POINT ( 'NONE',  ( 72.84354978475252551, 71.10232518220604447, -7.524857974791624216 ) ) ;
#58833=CARTESIAN_POINT ( 'NONE',  ( 78.96537477373632896, 60.10141448056572955, 16.11562121875446252 ) ) ;
#58834=CARTESIAN_POINT ( 'NONE',  ( 39.87427548755113804, 25.94754757982092741, 5.678558825948272215 ) ) ;
#58837=CARTESIAN_POINT ( 'NONE',  ( 80.88635954517316407, 43.32100077011654804, -9.977154956976749034 ) ) ;
#58838=DIRECTION ( 'NONE',  ( -0.8660254037844377084, -0.5000000000000014433, -0.000000000000000000 ) ) ;
#58839=CARTESIAN_POINT ( 'NONE',  ( 13.73114039420206645, 19.87878583063839955, -9.188101187500006262 ) ) ;
#58844=CARTESIAN_POINT ( 'NONE',  ( 78.55537653917157570, 48.00561504237174404, -13.97647359956260082 ) ) ;
#58845=EDGE_LOOP ( 'NONE', ( #96473, #55782, #39793, #24078 ) ) ;
#58846=CARTESIAN_POINT ( 'NONE',  ( 75.16744714750042533, 53.52973880860442080, -16.05274081456337143 ) ) ;
#58851=CARTESIAN_POINT ( 'NONE',  ( 66.74649031818020717, 68.37427386808708718, 4.497794777592671878 ) ) ;
#58860=CARTESIAN_POINT ( 'NONE',  ( 88.01315147845571119, 43.76068472133272280, -2.215761827693341957 ) ) ;
#58861=CARTESIAN_POINT ( 'NONE',  ( 80.71776722511965829, 57.44908488972237137, 16.57971273854668226 ) ) ;
#58864=CARTESIAN_POINT ( 'NONE',  ( 87.53583079710631409, 45.45925790797146249, -6.823327534849023657 ) ) ;
#58865=EDGE_CURVE ( 'NONE', #39534, #76006, #29499, .T. ) ;
#58872=CARTESIAN_POINT ( 'NONE',  ( 73.86319654356421438, 60.42244647389022560, 15.35035339019570877 ) ) ;
#58873=B_SPLINE_SURFACE_WITH_KNOTS ( 'NONE', 3, 1, ( 
 ( #12896, #10014 ),
 ( #13381, #43253 ),
 ( #49011, #63703 ),
 ( #94640, #43752 ),
 ( #74696, #25195 ),
 ( #79945, #2422 ),
 ( #64201, #36154 ),
 ( #5275, #10508 ),
 ( #33823, #81812 ),
 ( #72331, #2934 ),
 ( #17604, #67058 ),
 ( #56079, #97981 ),
 ( #28558, #48513 ),
 ( #95150, #56595 ),
 ( #95661, #26210 ),
 ( #57087, #88068 ),
 ( #18617, #50861 ),
 ( #74198, #4787 ),
 ( #35667, #21957 ),
 ( #15843, #90916 ),
 ( #7247, #31046 ),
 ( #21465, #14850 ),
 ( #60943, #68056 ),
 ( #5760, #6762 ),
 ( #14366, #46752 ),
 ( #15334, #98979 ),
 ( #69047, #29563 ),
 ( #38129, #99976 ),
 ( #61445, #60437 ),
 ( #61933, #92885 ),
 ( #38648, #98489 ) ),
 .UNSPECIFIED., .F., .F., .F.,
 ( 4, 3, 3, 3, 3, 3, 3, 3, 3, 3, 4 ),
 ( 2, 2 ),
 ( 0.000000000000000000, 0.1333490885032317663, 0.3007194338854262683, 0.4699862290245025997, 0.5844252810809391629, 0.6686540514502795629, 0.7354980260655534785, 0.8028463152565619154, 0.8633854507757232621, 0.9437142632667340214, 1.000000000000000000 ),
 ( 0.000000000000000000, 1.000000000000000000 ),
 .UNSPECIFIED. ) ;
#58878=CARTESIAN_POINT ( 'NONE',  ( 31.31925169811195175, 41.58029201028044497, 1.583844403245397769 ) ) ;
#58885=CARTESIAN_POINT ( 'NONE',  ( 16.59523773630703758, 17.78052372038640172, -10.00000000000000355 ) ) ;
#58887=CARTESIAN_POINT ( 'NONE',  ( 87.78081971166569986, 44.10618430004836910, 2.676874261813567468 ) ) ;
#58889=ORIENTED_EDGE ( 'NONE', *, *, #42188, .T. ) ;
#58890=CARTESIAN_POINT ( 'NONE',  ( 80.11389927631944374, 55.76916087316497084, -16.10389376604875977 ) ) ;
#58898=CARTESIAN_POINT ( 'NONE',  ( 81.56337590313989949, 52.27981926771280285, -15.13415753732220281 ) ) ;
#58905=CARTESIAN_POINT ( 'NONE',  ( 82.56870460112591559, 41.65958751012770733, 5.823109254649875055 ) ) ;
#58911=CARTESIAN_POINT ( 'NONE',  ( 82.79584117221035910, 40.63928722116583714, -1.337132909417009907 ) ) ;
#58918=VERTEX_POINT ( 'NONE', #20677 ) ;
#58935=CARTESIAN_POINT ( 'NONE',  ( 71.61432594831697429, 58.98614140521502236, -15.36087278562343705 ) ) ;
#58936=CARTESIAN_POINT ( 'NONE',  ( 71.80545688294488116, 72.09185741349443788, -1.683858184180939466 ) ) ;
#58939=CARTESIAN_POINT ( 'NONE',  ( 72.51713095402790543, 57.34819825014498917, 15.84120035366163748 ) ) ;
#58940=CARTESIAN_POINT ( 'NONE',  ( 71.68417880216854599, 71.76513893551050671, 3.129347443225863667 ) ) ;
#58945=LINE ( 'NONE', #28569, #4512 ) ;
#58947=CARTESIAN_POINT ( 'NONE',  ( 31.56043161122053320, 21.14754757982091249, -5.678558825948276656 ) ) ;
#58950=CYLINDRICAL_SURFACE ( 'NONE', #27113, 16.60714546451156792 ) ;
#58952=CARTESIAN_POINT ( 'NONE',  ( 74.81608510805732237, 67.12708246140779522, 12.96692076351790313 ) ) ;
#58953=CARTESIAN_POINT ( 'NONE',  ( 68.54233294502577678, 64.36627527950462024, 11.68987016893086661 ) ) ;
#58954=EDGE_LOOP ( 'NONE', ( #26156, #747, #69244, #97412 ) ) ;
#58962=CARTESIAN_POINT ( 'NONE',  ( 82.42550552036020406, 41.22741995948170057, -4.950294589197148376 ) ) ;
#58965=CARTESIAN_POINT ( 'NONE',  ( 71.85326037870230209, 72.57223462184859386, 1.067429543862054020 ) ) ;
#58966=CARTESIAN_POINT ( 'NONE',  ( 85.61868005752367594, 45.39050660362939027, 8.416507326733476901 ) ) ;
#58969=CARTESIAN_POINT ( 'NONE',  ( 69.52235898866341302, 70.68104077638899696, 1.790919661406474628 ) ) ;
#58973=CARTESIAN_POINT ( 'NONE',  ( 43.45144817956826699, 30.80170272979930601, 7.433330006724137462 ) ) ;
#58977=CARTESIAN_POINT ( 'NONE',  ( 86.19539083654223077, 46.94244887560866886, -10.58787169974291409 ) ) ;
#58994=CARTESIAN_POINT ( 'NONE',  ( 88.40016726344319409, 43.81338102853380434, 0.1423130075416289830 ) ) ;
#59007=CARTESIAN_POINT ( 'NONE',  ( 74.05623475345210238, 67.87786276047000911, -11.59565021290446651 ) ) ;
#59011=CARTESIAN_POINT ( 'NONE',  ( 3.501222095392049649, 22.99752408145588944, 5.678558825948277544 ) ) ;
#59020=CARTESIAN_POINT ( 'NONE',  ( 85.49318370521093868, 48.99722645306706426, -12.73116331006621316 ) ) ;
#59022=CARTESIAN_POINT ( 'NONE',  ( 85.47549930518324857, 42.86882085676075604, 2.634943531499700509 ) ) ;
#59023=CARTESIAN_POINT ( 'NONE',  ( 88.22236200735214595, 44.33456397151151407, -2.449239693650651972 ) ) ;
#59027=CARTESIAN_POINT ( 'NONE',  ( 66.07564871127969752, 68.72588067980983340, 0.03328844042743933640 ) ) ;
#59034=DIRECTION ( 'NONE',  ( -0.8660254037844377084, -0.5000000000000014433, -0.000000000000000000 ) ) ;
#59035=CARTESIAN_POINT ( 'NONE',  ( 88.11819866784119881, 43.86870363832047559, 2.501606352371065878 ) ) ;
#59043=ADVANCED_FACE ( 'NONE', ( #29761 ), #60634, .T. ) ;
#59050=CARTESIAN_POINT ( 'NONE',  ( 87.79556561918005286, 44.17086485108952587, -4.468589225908882412 ) ) ;
#59053=CARTESIAN_POINT ( 'NONE',  ( 78.10701254639744207, 51.83640423345583059, 15.50559604832989002 ) ) ;
#59054=CARTESIAN_POINT ( 'NONE',  ( 75.84078283921671471, 51.59066639860267145, 15.72938320682324154 ) ) ;
#59058=EDGE_CURVE ( 'NONE', #71177, #39764, #14570, .T. ) ;
#59059=CARTESIAN_POINT ( 'NONE',  ( 84.81065254960435595, 50.29073443720920977, 13.39702072830814394 ) ) ;
#59066=DIRECTION ( 'NONE',  ( -0.8660254037844379305, -0.5000000000000014433, -0.000000000000000000 ) ) ;
#59074=CARTESIAN_POINT ( 'NONE',  ( 75.69465226566293836, 65.43705427022661070, 14.28313312794709233 ) ) ;
#59076=CARTESIAN_POINT ( 'NONE',  ( 40.03666203415436797, 35.06628583063844928, -9.188101187500006262 ) ) ;
#59080=CARTESIAN_POINT ( 'NONE',  ( 18.45699304436188015, 28.84336893147756342, -7.433330006724137462 ) ) ;
#59081=CARTESIAN_POINT ( 'NONE',  ( 10.15257209397493199, 21.56454794089039950, 10.00000000000000355 ) ) ;
#59086=CARTESIAN_POINT ( 'NONE',  ( 70.42963173116773135, 60.96378554420563489, 14.42110835124151080 ) ) ;
#59087=CARTESIAN_POINT ( 'NONE',  ( 75.88031102442633369, 65.78928292664191702, -14.15509851726639390 ) ) ;
#59093=VERTEX_POINT ( 'NONE', #47936 ) ;
#59097=CARTESIAN_POINT ( 'NONE',  ( 86.98912267288208966, 45.08269913945084539, 6.733204870563289646 ) ) ;
#59101=CARTESIAN_POINT ( 'NONE',  ( 88.42017002704760387, 43.92753743058676008, 1.721442031696316599 ) ) ;
#59109=CARTESIAN_POINT ( 'NONE',  ( 40.64525884627276042, 24.26216523072497466, -2.296566073217252530E-15 ) ) ;
#59112=CARTESIAN_POINT ( 'NONE',  ( 87.32503761238780271, 45.47676291781615276, 7.117495199483119706 ) ) ;
#59114=EDGE_LOOP ( 'NONE', ( #19490, #32698, #99271, #82093 ) ) ;
#59118=CARTESIAN_POINT ( 'NONE',  ( 85.37538261767947745, 48.57005942898851458, 12.46403972397472337 ) ) ;
#59119=CARTESIAN_POINT ( 'NONE',  ( 66.25468035962502711, 68.66496212375022878, -2.132244879849610975 ) ) ;
#59121=CARTESIAN_POINT ( 'NONE',  ( 82.39721099679231031, 40.42262220688863295, 1.474573639680701431 ) ) ;
#59126=ORIENTED_EDGE ( 'NONE', *, *, #62355, .F. ) ;
#59133=CARTESIAN_POINT ( 'NONE',  ( 87.08635211577573898, 45.98159987514826241, -8.162078895322940397 ) ) ;
#59140=ORIENTED_EDGE ( 'NONE', *, *, #39324, .F. ) ;
#59142=ORIENTED_EDGE ( 'NONE', *, *, #51901, .T. ) ;
#59146=CARTESIAN_POINT ( 'NONE',  ( 84.05646506986525424, 49.99712786259807729, 13.48608966145228649 ) ) ;
#59148=CARTESIAN_POINT ( 'NONE',  ( 69.42588139327764907, 62.69554889617239013, -13.80398409906540280 ) ) ;
#59153=CARTESIAN_POINT ( 'NONE',  ( 82.12032703770964304, 50.14001162089422081, 14.08521554294405931 ) ) ;
#59154=CARTESIAN_POINT ( 'NONE',  ( 82.05174726562462695, 41.11851925668477747, -3.408449855420926156 ) ) ;
#59157=CARTESIAN_POINT ( 'NONE',  ( 72.12859001842100781, 72.20979474176914437, 3.988024951247647110 ) ) ;
#59158=CARTESIAN_POINT ( 'NONE',  ( 82.16472207147782569, 40.63388750005248085, -3.462830440365086027 ) ) ;
#59170=CARTESIAN_POINT ( 'NONE',  ( 72.02976470237955198, 59.30830629416842470, -15.33705471575644808 ) ) ;
#59172=CARTESIAN_POINT ( 'NONE',  ( 40.17197850526964942, 35.14441083166263979, 10.00000000000000533 ) ) ;
#59175=CARTESIAN_POINT ( 'NONE',  ( 82.48682597242610370, 54.22050469884690216, 15.58985929802052617 ) ) ;
#59177=DIRECTION ( 'NONE',  ( -0.8660254037844378194, -0.5000000000000014433, -0.000000000000000000 ) ) ;
#59180=CARTESIAN_POINT ( 'NONE',  ( 70.45698661661860740, 71.51623517888778281, 2.879531975083107653 ) ) ;
#59191=CARTESIAN_POINT ( 'NONE',  ( 36.79557518129325899, 43.01751292744061317, 6.180339887498949913 ) ) ;
#59196=CARTESIAN_POINT ( 'NONE',  ( 72.97333888298118154, 62.81283549581255699, 14.28620849118072833 ) ) ;
#59197=CARTESIAN_POINT ( 'NONE',  ( 75.06695094285400671, 67.05599132900850634, -12.66018568268392208 ) ) ;
#59206=VERTEX_POINT ( 'NONE', #50942 ) ;
#59214=CARTESIAN_POINT ( 'NONE',  ( 71.63103492117564031, 72.07843208848032646, 3.395715836721231895 ) ) ;
#59215=CARTESIAN_POINT ( 'NONE',  ( 28.76090768559789979, 38.64646525600391413, -2.839279412974133887 ) ) ;
#59220=CARTESIAN_POINT ( 'NONE',  ( 23.79748941506785798, 22.24335787977763346, -9.188101187500008038 ) ) ;
#59225=ORIENTED_EDGE ( 'NONE', *, *, #38751, .F. ) ;
#59244=AXIS2_PLACEMENT_3D ( 'NONE', #81778, #95994, #66042 ) ;
#59254=CARTESIAN_POINT ( 'NONE',  ( 81.68759648889933089, 55.58869686435339474, 15.96161034574012838 ) ) ;
#59259=EDGE_CURVE ( 'NONE', #72252, #50208, #41310, .T. ) ;
#59260=CARTESIAN_POINT ( 'NONE',  ( 71.31394413970843971, 63.96069529197309578, -13.14444410564831500 ) ) ;
#59262=CARTESIAN_POINT ( 'NONE',  ( 87.87434464428623926, 43.89907206790573468, 3.349129858248744540 ) ) ;
#59263=ORIENTED_EDGE ( 'NONE', *, *, #78367, .T. ) ;
#59264=CARTESIAN_POINT ( 'NONE',  ( 73.51948839908328637, 69.73627507762921596, -9.361350578256052657 ) ) ;
#59266=CARTESIAN_POINT ( 'NONE',  ( 76.08252525470864214, 51.16590352028240574, -16.09814970804995582 ) ) ;
#59271=ORIENTED_EDGE ( 'NONE', *, *, #56085, .F. ) ;
#59277=CARTESIAN_POINT ( 'NONE',  ( 67.94904719768317136, 67.86889835017325368, -8.208080553877501018 ) ) ;
#59284=CARTESIAN_POINT ( 'NONE',  ( 76.46051236311743082, 54.44209003778230738, 16.09620867652457576 ) ) ;
#59286=CARTESIAN_POINT ( 'NONE',  ( 72.48631355412707933, 71.22806908010377924, -6.072071567456138297 ) ) ;
#59294=CARTESIAN_POINT ( 'NONE',  ( 16.60635795911645829, 31.36126292948894445, 6.180339887498949913 ) ) ;
#59296=CARTESIAN_POINT ( 'NONE',  ( 82.06776773193392671, 41.79991662876560099, 5.443441096911677768 ) ) ;
#59312=CARTESIAN_POINT ( 'NONE',  ( 23.82048379914786906, 32.49103043416550207, -8.090169943749479842 ) ) ;
#59313=CARTESIAN_POINT ( 'NONE',  ( 85.11013511109823071, 48.98411268001765251, 12.43910323488882241 ) ) ;
#59315=CARTESIAN_POINT ( 'NONE',  ( 71.89533859728123844, 71.71086590489794332, -3.843102063196407681 ) ) ;
#59316=CARTESIAN_POINT ( 'NONE',  ( 73.82984320377984488, 55.19439280614383847, -16.12229116386306771 ) ) ;
#59319=CARTESIAN_POINT ( 'NONE',  ( 75.73386563160880769, 54.39615213926118287, 16.57551599053614311 ) ) ;
#59323=EDGE_CURVE ( 'NONE', #21672, #13779, #44234, .T. ) ;
#59326=CARTESIAN_POINT ( 'NONE',  ( 72.84756190538608678, 70.91156448913383770, -7.844936087786376966 ) ) ;
#59328=CARTESIAN_POINT ( 'NONE',  ( 43.33837710268888799, 27.94754757982092741, 5.678558825948272215 ) ) ;
#59335=CARTESIAN_POINT ( 'NONE',  ( 14.74991654177707723, 23.91421378149918198, 9.188101187500008038 ) ) ;
#59336=CARTESIAN_POINT ( 'NONE',  ( 71.96242732416024523, 72.61395932958828325, 1.324942441655010628 ) ) ;
#59341=VERTEX_POINT ( 'NONE', #56921 ) ;
#59349=CARTESIAN_POINT ( 'NONE',  ( 82.53995181069322484, 40.45689495123288282, 0.8907401359745065195 ) ) ;
#59351=CARTESIAN_POINT ( 'NONE',  ( 66.18541256665433536, 68.53576410546624231, 4.757783260268557690 ) ) ;
#59353=VERTEX_POINT ( 'NONE', #11369 ) ;
#59360=CARTESIAN_POINT ( 'NONE',  ( 80.31556117237309422, 57.81632953744806258, 16.60139635717628082 ) ) ;
#59363=CARTESIAN_POINT ( 'NONE',  ( 79.14312167556931854, 57.64441083166269664, 0.000000000000000000 ) ) ;
#59365=CARTESIAN_POINT ( 'NONE',  ( 81.01203187699685770, 43.60516739924280216, 9.421401130122879053 ) ) ;
#59368=CARTESIAN_POINT ( 'NONE',  ( 74.14512716957341354, 61.63656387330870956, 15.03512766998534467 ) ) ;
#59372=ORIENTED_EDGE ( 'NONE', *, *, #63866, .T. ) ;
#59378=CARTESIAN_POINT ( 'NONE',  ( 73.52359277784351832, 69.81900013914946612, 9.283661257273005063 ) ) ;
#59386=ORIENTED_EDGE ( 'NONE', *, *, #75121, .T. ) ;
#59387=CARTESIAN_POINT ( 'NONE',  ( 73.13914032746497185, 58.30547864447190420, -15.74582499144751679 ) ) ;
#59389=CARTESIAN_POINT ( 'NONE',  ( 32.48073783699224748, 37.49103043416551628, -8.090169943749479842 ) ) ;
#59392=CARTESIAN_POINT ( 'NONE',  ( 67.08913548327878118, 66.86964105702345762, 8.907371351497101131 ) ) ;
#59399=CARTESIAN_POINT ( 'NONE',  ( 71.78685388442551130, 69.08504693158637622, 8.871386085792403620 ) ) ;
#59401=CARTESIAN_POINT ( 'NONE',  ( 79.19103031000082638, 46.13451125956017052, 12.66280935556781095 ) ) ;
#59422=CARTESIAN_POINT ( 'NONE',  ( 69.74575514227493045, 70.90735852889230273, 0.2747676320513545156 ) ) ;
#59424=CARTESIAN_POINT ( 'NONE',  ( 13.50812563192542548, 9.927558733836244542, 6.180339887498953466 ) ) ;
#59436=CARTESIAN_POINT ( 'NONE',  ( 10.11087252192314345, 14.03677371833799548, 10.00000000000000533 ) ) ;
#59437=CARTESIAN_POINT ( 'NONE',  ( 80.06754722118087386, 49.20904160353000378, 14.67962688378318958 ) ) ;
#59438=CARTESIAN_POINT ( 'NONE',  ( 71.46737963517870185, 59.24065988555543782, -15.76538128299026909 ) ) ;
#59448=DIRECTION ( 'NONE',  ( -0.2033683215378938036, 0.3522442655536374700, -0.9135454576426059736 ) ) ;
#59451=CARTESIAN_POINT ( 'NONE',  ( 28.18775043786755319, 21.98920272979927759, 7.433330006724137462 ) ) ;
#59454=CARTESIAN_POINT ( 'NONE',  ( 75.03531058944138010, 53.45646444308351874, -16.05297267460561628 ) ) ;
#59455=LINE ( 'NONE', #66586, #77564 ) ;
#59457=CARTESIAN_POINT ( 'NONE',  ( 68.99476962784538614, 64.41967618265260853, 12.49304100067268486 ) ) ;
#59465=CARTESIAN_POINT ( 'NONE',  ( 69.88579529611078556, 68.58817071522582864, 7.900203795979792609 ) ) ;
#59468=CARTESIAN_POINT ( 'NONE',  ( 71.96958093079467744, 72.27199135482793224, 0.6334255257473564438 ) ) ;
#59473=CARTESIAN_POINT ( 'NONE',  ( 67.07226750202337939, 68.19592289027032450, 5.518172639132539636 ) ) ;
#59474=CYLINDRICAL_SURFACE ( 'NONE', #30646, 10.00000000000001066 ) ;
#59477=CARTESIAN_POINT ( 'NONE',  ( 14.19121639173650706, 20.14441083166259716, 10.00000000000000533 ) ) ;
#59480=CARTESIAN_POINT ( 'NONE',  ( 73.83109025078562127, 55.13289435005326311, 16.60030462077566327 ) ) ;
#59481=CARTESIAN_POINT ( 'NONE',  ( 86.48326989762649930, 47.07371192975631402, -10.55119608217690441 ) ) ;
#59495=CARTESIAN_POINT ( 'NONE',  ( 73.11394343355392778, 69.60018041412448042, -9.852821959973875110 ) ) ;
#59497=CARTESIAN_POINT ( 'NONE',  ( 81.38913804857537571, 41.97458054521010951, -7.739545251740827858 ) ) ;
#59506=VERTEX_POINT ( 'NONE', #42709 ) ;
#59512=CARTESIAN_POINT ( 'NONE',  ( 71.26654922642217116, 68.38198715351988710, -9.349859695236091284 ) ) ;
#59515=CARTESIAN_POINT ( 'NONE',  ( 76.83134550358633419, 60.61061650515956956, 15.77294948966528132 ) ) ;
#59516=CARTESIAN_POINT ( 'NONE',  ( 2.405479210251257438, 24.49540643055184930, 3.479690158560446702E-15 ) ) ;
#59524=CARTESIAN_POINT ( 'NONE',  ( 80.50527454617468948, 50.48295520238254142, -15.12725957157805823 ) ) ;
#59527=CARTESIAN_POINT ( 'NONE',  ( 88.32926345284593594, 43.93619003093853337, -2.170256470903187740 ) ) ;
#59530=CARTESIAN_POINT ( 'NONE',  ( 74.97996761797446652, 67.38724533294661967, -12.85106452774880204 ) ) ;
#59540=CARTESIAN_POINT ( 'NONE',  ( 76.12511762330939291, 65.41126435427986507, 14.01861623752280650 ) ) ;
#59542=ORIENTED_EDGE ( 'NONE', *, *, #94384, .F. ) ;
#59547=EDGE_CURVE ( 'NONE', #36835, #47529, #19646, .T. ) ;
#59548=CARTESIAN_POINT ( 'NONE',  ( 67.77468730211444381, 66.37560510333101149, -9.226434066144044266 ) ) ;
#59552=CARTESIAN_POINT ( 'NONE',  ( 84.68381221926802027, 47.49403502698439894, 11.40130350688633420 ) ) ;
#59558=CARTESIAN_POINT ( 'NONE',  ( 77.84078212536968522, 50.78282023170922344, 15.24705710655046786 ) ) ;
#59562=CARTESIAN_POINT ( 'NONE',  ( 81.98204644731730184, 41.14170830008083612, -5.380964918418895238 ) ) ;
#59567=CARTESIAN_POINT ( 'NONE',  ( 84.59313982267055110, 50.24721290632345472, 13.87151924479132425 ) ) ;
#59575=CARTESIAN_POINT ( 'NONE',  ( 6.332637391379750014, 21.84336893147753855, -7.433330006724137462 ) ) ;
#59584=CARTESIAN_POINT ( 'NONE',  ( 39.32338737416051089, 38.10171378149922106, 9.188101187500008038 ) ) ;
#59586=FACE_BOUND ( 'NONE', #65533, .T. ) ;
#59588=CARTESIAN_POINT ( 'NONE',  ( 28.09632999608277615, 19.14754757982091604, -5.678558825948276656 ) ) ;
#59593=CARTESIAN_POINT ( 'NONE',  ( 70.94178428196880759, 60.98283367154441947, 14.53595739235115936 ) ) ;
#59603=CARTESIAN_POINT ( 'NONE',  ( 85.26196194431867070, 42.92904878948160530, 3.532607271268957572 ) ) ;
#59608=DIRECTION ( 'NONE',  ( 0.000000000000000000, -0.3470917258701586294, -0.9378311862123559495 ) ) ;
#59611=CARTESIAN_POINT ( 'NONE',  ( 88.13402233310422673, 44.37312773088997631, -4.489783613381807648 ) ) ;
#59616=CARTESIAN_POINT ( 'NONE',  ( 43.73469409959700016, 27.11110640527295956, -2.839279412974138328 ) ) ;
#59617=CARTESIAN_POINT ( 'NONE',  ( 75.75053192129530544, 59.74695923988007706, -15.79163679635876427 ) ) ;
#59632=CARTESIAN_POINT ( 'NONE',  ( 82.18773400532718654, 40.81893033463614984, 1.092004392742265795 ) ) ;
#59640=B_SPLINE_CURVE_WITH_KNOTS ( 'NONE', 3,
 ( #3635, #12228, #58787, #81166, #65415, #27430, #4110, #80164, #57803, #73042, #65905, #20327, #96358, #42108, #66413, #72548, #5117, #87794, #43086, #74539, #74029, #64421, #19829, #12737, #97339, #88782, #50213, #4617, #42595, #81654, #82162, #34038, #89280, #19352, #27907, #50700, #34516, #95384, #41605, #35510, #18336, #49230, #26924, #96862, #43602, #73529 ),
 .UNSPECIFIED., .F., .F.,
 ( 4, 1, 2, 2, 1, 2, 2, 1, 1, 2, 2, 1, 1, 2, 2, 1, 1, 2, 2, 1, 1, 1, 2, 2, 1, 1, 1, 2, 2, 4 ),
 ( 0.000000000000000000, 0.06249999999998762101, 0.09374999999998372135, 0.1249999999999798217, 0.1874999999999718003, 0.2187499999999678035, 0.2499999999999638067, 0.3124999999999550915, 0.3437499999999526490, 0.3593749999999524825, 0.3749999999999522604, 0.4374999999999585887, 0.4687499999999626965, 0.4843749999999644174, 0.4999999999999661382, 0.5624999999999762412, 0.5937499999999804601, 0.6093749999999825695, 0.6249999999999846789, 0.6874999999999930056, 0.7187499999999977796, 0.7343750000000009992, 0.7421875000000016653, 0.7500000000000023315, 0.8125000000000105471, 0.8437500000000147660, 0.8593750000000154321, 0.8671875000000148770, 0.8750000000000143219, 1.000000000000000000 ),
 .UNSPECIFIED. ) ;
#59646=CARTESIAN_POINT ( 'NONE',  ( 87.24292777721575476, 46.11748857515735267, -8.882011181227387198 ) ) ;
#59652=EDGE_CURVE ( 'NONE', #31643, #7307, #87347, .T. ) ;
#59656=VERTEX_POINT ( 'NONE', #70003 ) ;
#59659=CARTESIAN_POINT ( 'NONE',  ( 83.83418024175072958, 48.96564077411333926, 12.89930316525782850 ) ) ;
#59661=CARTESIAN_POINT ( 'NONE',  ( 69.63548731322468655, 62.62411233422432133, -13.34129631502566227 ) ) ;
#59667=CARTESIAN_POINT ( 'NONE',  ( 82.47313821142903123, 40.87591070147813355, -3.712110524942620948 ) ) ;
#59670=CARTESIAN_POINT ( 'NONE',  ( 71.88653196722606253, 72.25570330380722339, 3.269911192557279911 ) ) ;
#59671=CARTESIAN_POINT ( 'NONE',  ( 82.69055213595072473, 42.56357957931876967, 6.360044358398685205 ) ) ;
#59674=CARTESIAN_POINT ( 'NONE',  ( 80.74302285234506371, 53.94966248920944452, 15.73036127202275658 ) ) ;
#59679=CARTESIAN_POINT ( 'NONE',  ( 77.58957552442460326, 61.75793702469097468, 15.67560070342386602 ) ) ;
#59681=AXIS2_PLACEMENT_3D ( 'NONE', #89904, #72711, #3301 ) ;
#59682=CARTESIAN_POINT ( 'NONE',  ( 66.44743792946236738, 67.95054874496071307, 6.521299778128105018 ) ) ;
#59689=CARTESIAN_POINT ( 'NONE',  ( 73.45606387015448036, 70.03420106287664737, -9.568701002945239509 ) ) ;
#59697=CARTESIAN_POINT ( 'NONE',  ( 72.11463582380375215, 72.32045887020245800, 3.546959094384888100 ) ) ;
#59704=CARTESIAN_POINT ( 'NONE',  ( 71.54037008220826976, 72.37285432226113358, -1.295160433098011543 ) ) ;
#59707=CARTESIAN_POINT ( 'NONE',  ( 22.44070990177030112, 31.14336893147756413, 7.433330006724141015 ) ) ;
#59710=CARTESIAN_POINT ( 'NONE',  ( 41.30863684418880410, 35.80066082961425167, 10.00000000000000533 ) ) ;
#59712=CARTESIAN_POINT ( 'NONE',  ( 76.42791049025993289, 61.90737760121017885, 15.82173950495353232 ) ) ;
#59713=ORIENTED_EDGE ( 'NONE', *, *, #23778, .F. ) ;
#59714=CARTESIAN_POINT ( 'NONE',  ( 73.42682404930152984, 64.53156016964122443, 13.57139978262335234 ) ) ;
#59715=CARTESIAN_POINT ( 'NONE',  ( 70.84057020560329931, 67.84468212244721030, -9.645047131074784730 ) ) ;
#59727=CARTESIAN_POINT ( 'NONE',  ( 82.63281508726200286, 40.94328431233920895, -3.617117793111275681 ) ) ;
#59730=CARTESIAN_POINT ( 'NONE',  ( 79.07447601446385477, 46.01053808348076046, -12.62649058706214511 ) ) ;
#59732=CARTESIAN_POINT ( 'NONE',  ( 72.96265021447784704, 70.35314760898533848, -8.120586438831022491 ) ) ;
#59736=CARTESIAN_POINT ( 'NONE',  ( 25.69310950058095955, 17.76004757982089899, 5.678558825948272215 ) ) ;
#59737=CARTESIAN_POINT ( 'NONE',  ( 26.58620497985335973, 27.30066082961423035, -10.00000000000000533 ) ) ;
#59739=CARTESIAN_POINT ( 'NONE',  ( 75.22859809181653645, 66.95660471994222007, -12.79880029611497427 ) ) ;
#59748=CARTESIAN_POINT ( 'NONE',  ( 66.23237210115183871, 68.64930917983895142, -2.151527110974545298 ) ) ;
#59750=LINE ( 'NONE', #21276, #11133 ) ;
#59757=FACE_OUTER_BOUND ( 'NONE', #63144, .T. ) ;
#59765=CARTESIAN_POINT ( 'NONE',  ( 75.32358509735726670, 66.62760184127506591, -13.06371402686526473 ) ) ;
#59769=CARTESIAN_POINT ( 'NONE',  ( 81.89559477234445239, 55.33976261442212774, 16.26127046582525892 ) ) ;
#59771=CARTESIAN_POINT ( 'NONE',  ( 72.38282305304500142, 69.07686135063536881, 9.305092211891095033 ) ) ;
#59774=AXIS2_PLACEMENT_3D ( 'NONE', #74302, #59034, #41867 ) ;
#59775=CARTESIAN_POINT ( 'NONE',  ( 73.64227373014415434, 63.39856954260761057, -14.21043620611602698 ) ) ;
#59778=VERTEX_POINT ( 'NONE', #66779 ) ;
#59779=CARTESIAN_POINT ( 'NONE',  ( 71.70884033504357546, 69.86088245213113623, -7.641946344699698024 ) ) ;
#59780=CARTESIAN_POINT ( 'NONE',  ( 76.04814661432739342, 51.39648587280629499, -16.15155320745066803 ) ) ;
#59782=B_SPLINE_CURVE_WITH_KNOTS ( 'NONE', 3,
 ( #16642, #88111, #71869, #78466, #87122, #94188, #9567, #79990, #94683, #47537, #33347, #2981, #18662, #70855, #39920, #40921, #78981, #64246, #24741, #41943, #17140, #72878, #95707, #9050, #72374, #79494, #48037, #2467, #3470, #34347, #96188, #33873, #56643, #1464, #40429, #10056, #26255, #57130, #32840, #26748, #32344, #95196, #10558, #25768, #87626, #49541 ),
 .UNSPECIFIED., .F., .F.,
 ( 4, 1, 1, 1, 2, 2, 1, 1, 1, 2, 2, 1, 1, 2, 2, 1, 1, 2, 2, 1, 1, 2, 2, 1, 2, 2, 1, 2, 2, 4 ),
 ( 0.000000000000000000, 0.06249999999996047606, 0.09374999999994101940, 0.1093749999999315409, 0.1171874999999289180, 0.1249999999999263089, 0.1874999999998932521, 0.2187499999998767930, 0.2343749999998704092, 0.2421874999998690769, 0.2499999999998677724, 0.3124999999998596123, 0.3437499999998554490, 0.3593749999998534506, 0.3749999999998514522, 0.4374999999998536726, 0.4687499999998547828, 0.4843749999998554490, 0.4999999999998561151, 0.5624999999998625544, 0.5937499999998642197, 0.6093749999998666622, 0.6249999999998691047, 0.6874999999998885336, 0.7187499999998983036, 0.7499999999999080735, 0.8124999999999311662, 0.8437499999999426015, 0.8749999999999540368, 1.000000000000000000 ),
 .UNSPECIFIED. ) ;
#59792=FACE_OUTER_BOUND ( 'NONE', #10328, .T. ) ;
#59795=CARTESIAN_POINT ( 'NONE',  ( 76.16668535934209672, 53.10184382116266022, 15.96041101260095907 ) ) ;
#59799=CARTESIAN_POINT ( 'NONE',  ( 79.67161915667092842, 46.83867530445827043, 12.95308866772764311 ) ) ;
#59800=CARTESIAN_POINT ( 'NONE',  ( 73.66290725793270155, 69.32596597699954089, -9.966140398900341424 ) ) ;
#59801=ADVANCED_FACE ( 'NONE', ( #20692 ), #19846, .T. ) ;
#59809=CARTESIAN_POINT ( 'NONE',  ( 17.99199860517156324, 32.16126292948895582, -6.180339887498951690 ) ) ;
#59818=VERTEX_POINT ( 'NONE', #84025 ) ;
#59820=CARTESIAN_POINT ( 'NONE',  ( 66.83424962952723547, 68.16180659050830570, -6.545639671669595927 ) ) ;
#59821=CARTESIAN_POINT ( 'NONE',  ( 73.08532603445986808, 70.49974493736067416, -7.999444584973850247 ) ) ;
#59826=CARTESIAN_POINT ( 'NONE',  ( 30.82187231905848535, 18.76426979415091267, 3.090169943749476733 ) ) ;
#59827=CARTESIAN_POINT ( 'NONE',  ( 85.59998877908455484, 48.66343243370425142, 12.43629469118824638 ) ) ;
#59844=CARTESIAN_POINT ( 'NONE',  ( 45.61829935282815995, 28.19860640527296525, 2.839279412974134775 ) ) ;
#59850=CARTESIAN_POINT ( 'NONE',  ( 17.37926562425035826, 12.96004757982088762, -5.678558825948276656 ) ) ;
#59854=CARTESIAN_POINT ( 'NONE',  ( 71.41016749218992743, 59.45273978182969188, 15.19346469599747174 ) ) ;
#59859=CARTESIAN_POINT ( 'NONE',  ( 81.14314822843688546, 42.42749270467351153, 7.695795501257847171 ) ) ;
#59860=ORIENTED_EDGE ( 'NONE', *, *, #32475, .F. ) ;
#59863=CARTESIAN_POINT ( 'NONE',  ( 76.70949559664001072, 63.86342103896397759, 14.86793590975532631 ) ) ;
#59866=ORIENTED_EDGE ( 'NONE', *, *, #91965, .T. ) ;
#59867=DIRECTION ( 'NONE',  ( 0.4924038765061026779, -0.8528685319524446085, -0.1736481776669273058 ) ) ;
#59872=CARTESIAN_POINT ( 'NONE',  ( 80.25077290097513583, 58.18867766503439043, -16.60702595570231566 ) ) ;
#59875=CARTESIAN_POINT ( 'NONE',  ( 78.04299808706751662, 61.03337783168321096, -15.88841590149242222 ) ) ;
#59876=ADVANCED_FACE ( 'NONE', ( #19098 ), #82177, .T. ) ;
#59877=CARTESIAN_POINT ( 'NONE',  ( 81.08217831220640903, 43.07020448918126476, 9.543463939025171427 ) ) ;
#59887=DIRECTION ( 'NONE',  ( -0.8660254037844378194, -0.5000000000000013323, -0.000000000000000000 ) ) ;
#59890=EDGE_CURVE ( 'NONE', #76483, #89630, #6086, .T. ) ;
#59896=VECTOR ( 'NONE', #67210, 1000.000000000000114 ) ;
#59900=CARTESIAN_POINT ( 'NONE',  ( 74.38854607822595710, 57.91757908437448776, -15.94610812356584262 ) ) ;
#59908=CARTESIAN_POINT ( 'NONE',  ( 76.40818250836743175, 54.09807576519859396, -16.06719028116590309 ) ) ;
#59910=CARTESIAN_POINT ( 'NONE',  ( 79.49157516048417449, 46.35107416014648152, 12.69267528992099869 ) ) ;
#59912=CARTESIAN_POINT ( 'NONE',  ( 76.20052385246813742, 55.90692255230084129, -16.60794131075797608 ) ) ;
#59916=CARTESIAN_POINT ( 'NONE',  ( 83.34650525046124869, 42.68055930881851623, 6.999721904327397937 ) ) ;
#59931=CARTESIAN_POINT ( 'NONE',  ( 81.85611950375817969, 41.21271484795168760, -5.731628893815098102 ) ) ;
#59934=DIRECTION ( 'NONE',  ( 0.000000000000000000, -1.000000000000000000, 1.060575238724906175E-16 ) ) ;
#59937=CARTESIAN_POINT ( 'NONE',  ( 79.26974131400612578, 59.52036692680489693, -16.53359576550785803 ) ) ;
#59939=CARTESIAN_POINT ( 'NONE',  ( 80.18492040316456837, 47.57055350794450987, -13.79677460666521149 ) ) ;
#59940=ADVANCED_FACE ( 'NONE', ( #92009 ), #66761, .T. ) ;
#59942=CARTESIAN_POINT ( 'NONE',  ( 66.18968672761215544, 68.49487770601442094, -4.881532527435783919 ) ) ;
#59950=CARTESIAN_POINT ( 'NONE',  ( 70.58107171170311744, 70.42171057263509226, 5.244054101350007713 ) ) ;
#59951=CARTESIAN_POINT ( 'NONE',  ( 66.41207382487917243, 68.05599230888550721, -4.871615717380384680 ) ) ;
#59957=CARTESIAN_POINT ( 'NONE',  ( 24.17276070933917609, 32.14336893147756768, 7.433330006724141015 ) ) ;
#59959=CARTESIAN_POINT ( 'NONE',  ( 85.33699565288863198, 48.33901173460944278, -12.30238903177781395 ) ) ;
#59961=CARTESIAN_POINT ( 'NONE',  ( 88.21274111123641148, 43.92339361237885953, 2.502205135834638217 ) ) ;
#59963=CARTESIAN_POINT ( 'NONE',  ( 68.83067416445564390, 64.29043214222643599, 12.51914382770813461 ) ) ;
#59973=CARTESIAN_POINT ( 'NONE',  ( 71.64147408072075507, 72.45736481867632506, 0.9627058344235318588 ) ) ;
#59974=DIRECTION ( 'NONE',  ( -0.4972609476841356457, 0.8612812260087758798, 0.1045284632676436315 ) ) ;
#59977=CARTESIAN_POINT ( 'NONE',  ( 68.57078111580027269, 69.83554316562776876, 3.250710778096809417 ) ) ;
#59982=CARTESIAN_POINT ( 'NONE',  ( 19.88154021482007749, 11.28848085856230377, 1.475505719884397138E-15 ) ) ;
#59983=CARTESIAN_POINT ( 'NONE',  ( 84.09923392499968031, 48.62025565107681047, 13.03358251092844000 ) ) ;
#59984=EDGE_LOOP ( 'NONE', ( #49457, #37432, #56757, #17016 ) ) ;
#59986=CARTESIAN_POINT ( 'NONE',  ( 86.15665200708443194, 46.94614013873178493, -10.61509939557872073 ) ) ;
#59987=CARTESIAN_POINT ( 'NONE',  ( 84.69910869649594076, 45.11611167524748822, -8.770891836413943210 ) ) ;
#59990=CARTESIAN_POINT ( 'NONE',  ( 79.42275183545125117, 59.70681295713441727, -16.17365378312262436 ) ) ;
#59992=CARTESIAN_POINT ( 'NONE',  ( 87.34642337659644795, 43.20430561321286689, -4.696387144280492735E-07 ) ) ;
#59993=CARTESIAN_POINT ( 'NONE',  ( 69.35253854973147725, 63.01665765329197910, 13.58811665792164014 ) ) ;
#59997=CARTESIAN_POINT ( 'NONE',  ( 68.62032050481585088, 70.74532250035436221, 0.7225376792652218327 ) ) ;
#59998=CARTESIAN_POINT ( 'NONE',  ( 81.60031397647219364, 42.64669660525676420, -7.620194330344577160 ) ) ;
#60004=CARTESIAN_POINT ( 'NONE',  ( 81.56554115986412512, 50.74390853957432057, 14.52805404999391214 ) ) ;
#60009=ORIENTED_EDGE ( 'NONE', *, *, #58199, .T. ) ;
#60011=EDGE_CURVE ( 'NONE', #62487, #36092, #86914, .T. ) ;
#60015=CARTESIAN_POINT ( 'NONE',  ( 82.81701024667485456, 53.37631690731208778, -15.29776186725079334 ) ) ;
#60018=CARTESIAN_POINT ( 'NONE',  ( 76.68531899032339538, 59.74883463824316010, 15.90439264542311726 ) ) ;
#60019=CARTESIAN_POINT ( 'NONE',  ( 7.668962567711002265, 16.37878583063838533, 9.188101187500006262 ) ) ;
#60029=CARTESIAN_POINT ( 'NONE',  ( 85.73939067079162157, 43.09395395977590226, 3.031127533106598548 ) ) ;
#60041=CARTESIAN_POINT ( 'NONE',  ( 33.32252067603396029, 20.20801979619930577, -3.090169943749474069 ) ) ;
#60051=CARTESIAN_POINT ( 'NONE',  ( 84.82223274050802786, 47.96708222389427334, 11.74877015797738622 ) ) ;
#60056=CARTESIAN_POINT ( 'NONE',  ( 87.84668905185571930, 44.44462267732798466, -3.943169391390685341 ) ) ;
#60058=CARTESIAN_POINT ( 'NONE',  ( 79.27428326626197475, 58.12688789515522103, 16.22428513376493342 ) ) ;
#60061=CARTESIAN_POINT ( 'NONE',  ( 78.47336120520917291, 54.13984261423279776, -15.94495912723520625 ) ) ;
#60072=EDGE_CURVE ( 'NONE', #37857, #55385, #20901, .T. ) ;
#60074=CARTESIAN_POINT ( 'NONE',  ( 9.573022157908470220, 14.03085787977760646, 9.188101187500006262 ) ) ;
#60082=CARTESIAN_POINT ( 'NONE',  ( 42.15419773769040290, 26.19860640527295814, 2.839279412974134775 ) ) ;
#60084=FACE_BOUND ( 'NONE', #11035, .T. ) ;
#60085=ORIENTED_EDGE ( 'NONE', *, *, #26577, .F. ) ;
#60086=CARTESIAN_POINT ( 'NONE',  ( 23.51121325743158508, 19.28920272979927120, -7.433330006724141015 ) ) ;
#60091=VERTEX_POINT ( 'NONE', #23359 ) ;
#60092=CARTESIAN_POINT ( 'NONE',  ( 70.80219251493628008, 60.87566219113961807, 14.54675205938061744 ) ) ;
#60098=CARTESIAN_POINT ( 'NONE',  ( 70.27693386828532596, 63.84783520667136258, 13.41007760784634151 ) ) ;
#60101=CARTESIAN_POINT ( 'NONE',  ( 82.87596643829704135, 41.15858874971023340, 0.1873015203630768732 ) ) ;
#60105=CARTESIAN_POINT ( 'NONE',  ( 86.43879872498249028, 47.50144577818752367, -11.01113278173270693 ) ) ;
#60111=CARTESIAN_POINT ( 'NONE',  ( 35.31444455405989657, 43.49540643055190969, 3.479690158560446702E-15 ) ) ;
#60112=PLANE ( 'NONE',  #42944 ) ;
#60126=CARTESIAN_POINT ( 'NONE',  ( 82.48576119632784298, 40.42786996717531167, 0.9267432163235941323 ) ) ;
#60128=EDGE_CURVE ( 'NONE', #12155, #14695, #75338, .T. ) ;
#60129=CARTESIAN_POINT ( 'NONE',  ( 77.31442247797616574, 63.22349627092265223, -15.21530826047764862 ) ) ;
#60133=ORIENTED_EDGE ( 'NONE', *, *, #50506, .T. ) ;
#60135=CARTESIAN_POINT ( 'NONE',  ( 27.20206195878591870, 37.74646525600392266, 2.839279412974139660 ) ) ;
#60139=CARTESIAN_POINT ( 'NONE',  ( 74.18796447308154995, 68.76651203251665834, -11.36463150814737766 ) ) ;
#60142=CARTESIAN_POINT ( 'NONE',  ( 31.58830253577720626, 26.43677371833803136, -10.00000000000000355 ) ) ;
#60143=CARTESIAN_POINT ( 'NONE',  ( 15.16022976130349065, 27.49103043416548431, -8.090169943749479842 ) ) ;
#60146=ORIENTED_EDGE ( 'NONE', *, *, #69288, .T. ) ;
#60152=CARTESIAN_POINT ( 'NONE',  ( 83.76918405636864406, 48.70819753632389393, 12.74357695574461147 ) ) ;
#60153=PLANE ( 'NONE',  #4772 ) ;
#60154=CARTESIAN_POINT ( 'NONE',  ( 69.82388864200702017, 62.78505363333596279, -13.30987185219257718 ) ) ;
#60158=CARTESIAN_POINT ( 'NONE',  ( 82.14295211724746082, 50.23227492270505223, 14.12545005886346772 ) ) ;
#60159=CARTESIAN_POINT ( 'NONE',  ( 82.10416747357091083, 41.15855318747237135, -3.445724401907877432 ) ) ;
#60162=DIRECTION ( 'NONE',  ( 0.5000000000000014433, -0.8660254037844378194, 0.000000000000000000 ) ) ;
#60166=CARTESIAN_POINT ( 'NONE',  ( 72.06082664650362801, 70.73905283940008815, -6.476476296684364975 ) ) ;
#60172=EDGE_CURVE ( 'NONE', #60539, #12691, #8181, .T. ) ;
#60177=ADVANCED_FACE ( 'NONE', ( #84228 ), #84714, .T. ) ;
#60178=CARTESIAN_POINT ( 'NONE',  ( 37.05984716305037807, 40.13478043621391578, 8.090169943749478065 ) ) ;
#60180=CARTESIAN_POINT ( 'NONE',  ( 82.78345634833958400, 53.69061190982763776, 15.38144188222361386 ) ) ;
#60181=CARTESIAN_POINT ( 'NONE',  ( 71.72870690310715247, 72.16142621409359492, 3.283488654313290844 ) ) ;
#60186=CARTESIAN_POINT ( 'NONE',  ( 43.71265818875933462, 33.43677371833805267, -10.00000000000000355 ) ) ;
#60188=CARTESIAN_POINT ( 'NONE',  ( 71.70482085610929346, 72.04085231235103493, -1.605959201768876410 ) ) ;
#60190=CARTESIAN_POINT ( 'NONE',  ( 21.14648969749996965, 33.18502408145592142, 5.678558825948276656 ) ) ;
#60193=CARTESIAN_POINT ( 'NONE',  ( 44.08964769951546714, 27.58380873178791148, 6.180339887498953466 ) ) ;
#60198=CARTESIAN_POINT ( 'NONE',  ( 73.54743893589137826, 64.98868938413073693, 13.35376214375427217 ) ) ;
#60199=CARTESIAN_POINT ( 'NONE',  ( 70.04496804106824470, 67.88492258065853946, -9.012774590751471138 ) ) ;
#60215=CARTESIAN_POINT ( 'NONE',  ( 79.21691572551614513, 45.75049196499858084, -12.99762880459370784 ) ) ;
#60217=CARTESIAN_POINT ( 'NONE',  ( 73.10684881258417533, 70.60603909402131251, -7.845798253817742207 ) ) ;
#60220=VECTOR ( 'NONE', #34692, 1000.000000000000114 ) ;
#60222=CARTESIAN_POINT ( 'NONE',  ( 20.65934362447757167, 23.87878583063841376, -9.188101187500006262 ) ) ;
#60223=CARTESIAN_POINT ( 'NONE',  ( 75.61128893809926410, 57.78454237761125256, 16.06483355829618986 ) ) ;
#60224=CARTESIAN_POINT ( 'NONE',  ( 67.76226342272079251, 69.50789913810500309, -2.504574930950261624 ) ) ;
#60226=ADVANCED_FACE ( 'NONE', ( #83216 ), #577, .T. ) ;
#60228=ORIENTED_EDGE ( 'NONE', *, *, #73902, .F. ) ;
#60234=DIRECTION ( 'NONE',  ( 0.9646071681523454844, -0.2636911283094535152, 0.000000000000000000 ) ) ;
#60238=CARTESIAN_POINT ( 'NONE',  ( 81.53661897590532703, 55.80016554358400072, 16.37044094275388417 ) ) ;
#60253=CARTESIAN_POINT ( 'NONE',  ( 66.62639878018896411, 67.83600655791506995, 6.946500236981309584 ) ) ;
#60256=B_SPLINE_CURVE_WITH_KNOTS ( 'NONE', 3,
 ( #18555, #43321, #27652, #74267, #42323, #26146, #58036, #33758, #73744, #97083 ),
 .UNSPECIFIED., .F., .F.,
 ( 4, 2, 2, 2, 4 ),
 ( 0.000000000000000000, 0.2500000000000000000, 0.5000000000000000000, 0.7500000000000000000, 1.000000000000000000 ),
 .UNSPECIFIED. ) ;
#60258=CARTESIAN_POINT ( 'NONE',  ( 81.46866702687000839, 55.81909161095428829, 16.37896761046575378 ) ) ;
#60260=CARTESIAN_POINT ( 'NONE',  ( 71.11923220532735002, 65.88429979018354743, 11.70261362563623386 ) ) ;
#60267=CARTESIAN_POINT ( 'NONE',  ( 76.12238913165759868, 51.10370791208713115, -15.58940357410317468 ) ) ;
#60275=CARTESIAN_POINT ( 'NONE',  ( 80.09120749856197108, 44.41673742825524585, -10.86461196121644157 ) ) ;
#60278=CARTESIAN_POINT ( 'NONE',  ( 73.06696598015496136, 70.66213948254207367, 7.705144097525488789 ) ) ;
#60279=CARTESIAN_POINT ( 'NONE',  ( 73.78116818605872140, 66.73777287303562389, -12.34320005290799394 ) ) ;
#60281=CARTESIAN_POINT ( 'NONE',  ( 77.51198627597376856, 60.98384281500086956, 15.82258133188943106 ) ) ;
#60285=CARTESIAN_POINT ( 'NONE',  ( 81.13117295687578689, 52.04838968429105250, 15.10467803161753331 ) ) ;
#60295=B_SPLINE_SURFACE_WITH_KNOTS ( 'NONE', 3, 1, ( 
 ( #38931, #69836 ),
 ( #448, #62223 ),
 ( #23727, #16144 ),
 ( #6048, #67855 ),
 ( #98776, #94185 ),
 ( #71361, #93685 ),
 ( #17655, #71867 ),
 ( #78463, #57129 ),
 ( #950, #55621 ),
 ( #56641, #39917 ),
 ( #8550, #18153 ),
 ( #2465, #24738 ),
 ( #63748, #64244 ),
 ( #49052, #79988 ),
 ( #41432, #38312 ),
 ( #60606, #69221 ),
 ( #61612, #77331 ),
 ( #38813, #325 ),
 ( #62101, #29245 ),
 ( #52039, #13553 ),
 ( #78340, #78846 ),
 ( #94066, #95073 ),
 ( #70211, #40304 ),
 ( #71747, #63621 ),
 ( #48932, #24125 ),
 ( #1837, #54497 ),
 ( #79871, #25114 ),
 ( #25636, #41305 ),
 ( #56518, #87506 ),
 ( #72248, #85476 ),
 ( #3831, #35719 ) ),
 .UNSPECIFIED., .F., .F., .F.,
 ( 4, 3, 3, 3, 3, 3, 3, 3, 3, 3, 4 ),
 ( 2, 2 ),
 ( 0.000000000000000000, 0.1122669598086740300, 0.2243161639709581601, 0.3396355846219040742, 0.4553962076585059138, 0.5677860799922319623, 0.6749047109689451096, 0.7773884377078192909, 0.8775581155834162317, 0.9782364162377708006, 1.000000000000000000 ),
 ( 0.000000000000000000, 1.000000000000000000 ),
 .UNSPECIFIED. ) ;
#60296=CARTESIAN_POINT ( 'NONE',  ( 26.29472225869274382, 23.38052372038642091, 10.00000000000000533 ) ) ;
#60297=DIRECTION ( 'NONE',  ( -0.4999999999999982792, 0.8660254037844398178, 0.000000000000000000 ) ) ;
#60299=CARTESIAN_POINT ( 'NONE',  ( 67.28775127781241849, 69.02525132645125439, -5.181563858835234626 ) ) ;
#60306=VECTOR ( 'NONE', #30221, 1000.000000000000114 ) ;
#60307=CARTESIAN_POINT ( 'NONE',  ( 66.49880604618508073, 67.93642891560753583, -6.609368650527830624 ) ) ;
#60308=CARTESIAN_POINT ( 'NONE',  ( 72.45751905151222161, 70.67373443742414452, -7.865264308201653343 ) ) ;
#60311=CARTESIAN_POINT ( 'NONE',  ( 30.57965140047823738, 19.78380873178787880, -6.180339887498949025 ) ) ;
#60312=CARTESIAN_POINT ( 'NONE',  ( 85.51397903554266122, 48.65227260402726017, 12.46570927396283146 ) ) ;
#60314=CARTESIAN_POINT ( 'NONE',  ( 71.87910863004675832, 71.70566666627038899, -3.826659594235088946 ) ) ;
#60315=CARTESIAN_POINT ( 'NONE',  ( 78.14015596324891533, 47.79605781560269406, 14.53813849190288465 ) ) ;
#60317=DIRECTION ( 'NONE',  ( 0.8660254037844399289, 0.4999999999999977240, -0.000000000000000000 ) ) ;
#60320=EDGE_CURVE ( 'NONE', #10093, #60091, #76330, .T. ) ;
#60323=FACE_OUTER_BOUND ( 'NONE', #46950, .T. ) ;
#60328=CARTESIAN_POINT ( 'NONE',  ( 44.05945362601616466, 27.29860640527295956, -2.839279412974138328 ) ) ;
#60335=CARTESIAN_POINT ( 'NONE',  ( 20.93478768117288524, 17.80170272979926338, 7.433330006724137462 ) ) ;
#60337=CARTESIAN_POINT ( 'NONE',  ( 71.84836080304555139, 59.06364556286701628, 15.37505501383178519 ) ) ;
#60339=EDGE_LOOP ( 'NONE', ( #96005, #59713, #21532, #57403 ) ) ;
#60340=CARTESIAN_POINT ( 'NONE',  ( 86.19897734768302655, 45.52340696477872939, -8.150747010710539087 ) ) ;
#60341=CARTESIAN_POINT ( 'NONE',  ( 85.27924949840783597, 45.45504446614027927, -9.497384621978497421 ) ) ;
#60342=CARTESIAN_POINT ( 'NONE',  ( 75.10336920942704353, 53.49933058092891258, -16.05324734149355237 ) ) ;
#60343=CARTESIAN_POINT ( 'NONE',  ( 88.25515730755107313, 44.35562341810459941, 2.525333633695516333 ) ) ;
#60344=EDGE_LOOP ( 'NONE', ( #68961, #7664, #31148, #77141 ) ) ;
#60346=CARTESIAN_POINT ( 'NONE',  ( 82.39721099668476256, 40.42262220707492304, 1.474573639734337860 ) ) ;
#60347=CARTESIAN_POINT ( 'NONE',  ( 76.88576290890495102, 63.85744880123300504, 14.90658078946527354 ) ) ;
#60354=ORIENTED_EDGE ( 'NONE', *, *, #99606, .F. ) ;
#60357=CARTESIAN_POINT ( 'NONE',  ( 80.29069729260778843, 58.15026982914754683, -16.60659103188077879 ) ) ;
#60362=AXIS2_PLACEMENT_3D ( 'NONE', #60583, #5419, #27725 ) ;
#60363=ORIENTED_EDGE ( 'NONE', *, *, #34989, .F. ) ;
#60371=ORIENTED_EDGE ( 'NONE', *, *, #1243, .T. ) ;
#60378=CARTESIAN_POINT ( 'NONE',  ( 73.41164147859498712, 69.84296063560688594, 9.177452858377941780 ) ) ;
#60379=CARTESIAN_POINT ( 'NONE',  ( 82.80579214661656806, 42.74001471116365991, -6.585052516728319816 ) ) ;
#60389=CARTESIAN_POINT ( 'NONE',  ( 79.36418056962840240, 56.08893731827392770, -16.16201821102233183 ) ) ;
#60393=CARTESIAN_POINT ( 'NONE',  ( 78.29855726973434571, 47.75006341431981127, 13.92167056375030043 ) ) ;
#60396=CARTESIAN_POINT ( 'NONE',  ( 72.48280754011685190, 70.60311863597817705, 7.264376673680498442 ) ) ;
#60398=CARTESIAN_POINT ( 'NONE',  ( 79.39828970323148383, 45.77552746013876828, 12.94240580742716240 ) ) ;
#60405=CARTESIAN_POINT ( 'NONE',  ( 71.99267133948018227, 71.58944556433895912, 5.550980660130568900 ) ) ;
#60410=FACE_OUTER_BOUND ( 'NONE', #58127, .T. ) ;
#60411=LINE ( 'NONE', #28037, #90714 ) ;
#60423=DIRECTION ( 'NONE',  ( 0.4851478631379963491, -0.8403007481384849875, 0.2419218955996714493 ) ) ;
#60427=ORIENTED_EDGE ( 'NONE', *, *, #7646, .F. ) ;
#60434=CARTESIAN_POINT ( 'NONE',  ( 14.64478397084458550, 10.58380873178785642, 6.180339887498953466 ) ) ;
#60436=CARTESIAN_POINT ( 'NONE',  ( 71.61759974305658716, 58.94635126778479872, -15.37279249342744336 ) ) ;
#60437=CARTESIAN_POINT ( 'NONE',  ( 73.07265265467388815, 69.63838777454593298, 9.188147135407486843 ) ) ;
#60441=CARTESIAN_POINT ( 'NONE',  ( 73.11778380043915604, 57.33886984688226818, 15.89460713103382439 ) ) ;
#60443=CARTESIAN_POINT ( 'NONE',  ( 64.77737111682257876, 68.52662068827326891, 0.000000000000000000 ) ) ;
#60444=CARTESIAN_POINT ( 'NONE',  ( 66.40824058694533960, 68.21386763270049869, -4.392278699897152805 ) ) ;
#60452=CARTESIAN_POINT ( 'NONE',  ( 22.33066906249845118, 34.93396525600390845, 2.839279412974139660 ) ) ;
#60454=CARTESIAN_POINT ( 'NONE',  ( 83.58592293191674116, 51.62412561587523641, -14.84978998814507989 ) ) ;
#60456=CARTESIAN_POINT ( 'NONE',  ( 84.50387165700357173, 41.56312468464896170, -0.5288249497319834624 ) ) ;
#60458=CARTESIAN_POINT ( 'NONE',  ( 68.96547873374085214, 64.13046873611052945, 12.06460432375195957 ) ) ;
#60460=CARTESIAN_POINT ( 'NONE',  ( 81.50039046230392614, 52.51855974082073431, 15.62894985664426528 ) ) ;
#60461=CARTESIAN_POINT ( 'NONE',  ( 73.03232164105139645, 66.66734575193103751, -12.55698212435192929 ) ) ;
#60470=CARTESIAN_POINT ( 'NONE',  ( 71.98264401366868981, 72.39816763649429276, -2.869464145551841039 ) ) ;
#60471=CARTESIAN_POINT ( 'NONE',  ( 67.94301448590864823, 69.19482911460316643, 4.205308713653838737 ) ) ;
#60475=CARTESIAN_POINT ( 'NONE',  ( 11.07908504951724282, 25.13478043621386959, 8.090169943749478065 ) ) ;
#60476=CARTESIAN_POINT ( 'NONE',  ( 81.38228331512368641, 42.18052851754683275, 8.075145019496556387 ) ) ;
#60477=ORIENTED_EDGE ( 'NONE', *, *, #78944, .T. ) ;
#60479=CARTESIAN_POINT ( 'NONE',  ( 86.37020013017546205, 47.54260244662367541, -11.08968936411752715 ) ) ;
#60483=FACE_OUTER_BOUND ( 'NONE', #78652, .T. ) ;
#60485=CARTESIAN_POINT ( 'NONE',  ( 70.02414138031360835, 62.78214778883172187, 13.38063900663788708 ) ) ;
#60489=CARTESIAN_POINT ( 'NONE',  ( 73.05863210132505969, 69.60576123971951290, -9.808587366596233537 ) ) ;
#60491=CARTESIAN_POINT ( 'NONE',  ( 81.20776596464571639, 42.33569611896157880, -7.485437602881505725 ) ) ;
#60493=ADVANCED_FACE ( 'NONE', ( #67357 ), #91198, .T. ) ;
#60496=CARTESIAN_POINT ( 'NONE',  ( 82.02196949114711799, 53.52097756913676818, 15.46628681541728056 ) ) ;
#60498=CARTESIAN_POINT ( 'NONE',  ( 68.27542981431423641, 68.50580704656320563, 6.393928382725774462 ) ) ;
#60500=VERTEX_POINT ( 'NONE', #68353 ) ;
#60502=CARTESIAN_POINT ( 'NONE',  ( 66.18968672761215544, 68.49487770601442094, -4.881532527435783919 ) ) ;
#60505=CARTESIAN_POINT ( 'NONE',  ( 82.84342636331510334, 53.76751615666388062, -15.40379040879673056 ) ) ;
#60508=CARTESIAN_POINT ( 'NONE',  ( 76.97307773550161869, 61.50313384435956010, 15.60575781086138747 ) ) ;
#60509=CARTESIAN_POINT ( 'NONE',  ( 13.01786573420820226, 22.91421378149917842, 9.188101187500008038 ) ) ;
#60512=CARTESIAN_POINT ( 'NONE',  ( 85.67692334825835587, 48.86287692480856748, 12.08569265371076185 ) ) ;
#60514=ORIENTED_EDGE ( 'NONE', *, *, #92264, .T. ) ;
#60535=CARTESIAN_POINT ( 'NONE',  ( 72.62753967730402849, 70.91775434214520146, 7.625672695449470240 ) ) ;
#60537=CARTESIAN_POINT ( 'NONE',  ( 76.04770329001843265, 65.50818618912236957, 13.94958420308868341 ) ) ;
#60539=VERTEX_POINT ( 'NONE', #78476 ) ;
#60544=CARTESIAN_POINT ( 'NONE',  ( 86.39222172200696548, 43.37934728214441549, 2.793685208327149283 ) ) ;
#60546=CARTESIAN_POINT ( 'NONE',  ( 83.55683262847328763, 44.73071775418808471, 9.087976461446411136 ) ) ;
#60550=FACE_OUTER_BOUND ( 'NONE', #85763, .T. ) ;
#60554=CARTESIAN_POINT ( 'NONE',  ( 81.28829938836423707, 53.14541240262165900, -15.42935213604580014 ) ) ;
#60560=EDGE_CURVE ( 'NONE', #8880, #59093, #13207, .T. ) ;
#60564=EDGE_CURVE ( 'NONE', #65477, #10093, #26798, .T. ) ;
#60569=CARTESIAN_POINT ( 'NONE',  ( 4.462289544239296468, 25.68290643055184574, 3.479690158560446702E-15 ) ) ;
#60570=B_SPLINE_CURVE_WITH_KNOTS ( 'NONE', 3,
 ( #88149, #48598, #72917, #33908, #18697, #19214, #88648, #27292, #81521, #71904, #2504, #34869, #73397, #3508, #72416, #49092, #50084, #58174, #33386, #94722, #25281, #87163, #81041, #3020, #17695, #80531, #11111, #11604, #65283, #3983, #89159, #40472, #71404, #64288, #25806, #90631, #91116, #37361, #83017, #20690, #53068, #83516, #52073, #90116, #74898, #12090 ),
 .UNSPECIFIED., .F., .F.,
 ( 4, 1, 2, 2, 1, 2, 2, 1, 1, 2, 2, 1, 1, 2, 2, 1, 1, 2, 2, 1, 1, 1, 2, 2, 1, 1, 1, 2, 2, 4 ),
 ( 0.000000000000000000, 0.06250000000000308087, 0.09375000000000487110, 0.1250000000000066613, 0.1875000000000102418, 0.2187500000000134059, 0.2500000000000165423, 0.3125000000000192624, 0.3437500000000203726, 0.3593750000000210387, 0.3750000000000217049, 0.4375000000000275890, 0.4687500000000319189, 0.4843750000000340838, 0.5000000000000363043, 0.5625000000000544009, 0.5937500000000636158, 0.6093750000000668354, 0.6250000000000700551, 0.6875000000000744960, 0.7187500000000768274, 0.7343750000000780487, 0.7421875000000773825, 0.7500000000000766054, 0.8125000000000563993, 0.8437500000000449640, 0.8593750000000376366, 0.8671875000000351941, 0.8750000000000327516, 1.000000000000000000 ),
 .UNSPECIFIED. ) ;
#60571=CARTESIAN_POINT ( 'NONE',  ( 67.97445910463009966, 65.68506835540814848, 10.87894195494597405 ) ) ;
#60574=CARTESIAN_POINT ( 'NONE',  ( 83.53981050848499024, 42.15194584004071032, -4.113498934485630087 ) ) ;
#60576=LINE ( 'NONE', #77299, #95711 ) ;
#60578=CARTESIAN_POINT ( 'NONE',  ( 35.16646543599519248, 35.70171378149922248, -9.188101187500004485 ) ) ;
#60582=CARTESIAN_POINT ( 'NONE',  ( 22.87854050506884462, 34.18502408145592852, 5.678558825948277544 ) ) ;
#60583=CARTESIAN_POINT ( 'NONE',  ( 80.87517248313827167, 58.64441083166272506, 0.000000000000000000 ) ) ;
#60587=CARTESIAN_POINT ( 'NONE',  ( 70.62030545033579187, 60.85430430480430886, 14.51265376387380357 ) ) ;
#60589=AXIS2_PLACEMENT_3D ( 'NONE', #56424, #40205, #46828 ) ;
#60593=ORIENTED_EDGE ( 'NONE', *, *, #53101, .T. ) ;
#60596=CARTESIAN_POINT ( 'NONE',  ( 78.34913526621272695, 61.55915279984171917, 16.16953766326405173 ) ) ;
#60597=CARTESIAN_POINT ( 'NONE',  ( 87.56426860159915293, 44.18524048238309376, 3.435755015769986542 ) ) ;
#60603=PLANE ( 'NONE',  #15360 ) ;
#60605=CARTESIAN_POINT ( 'NONE',  ( 38.25529575686164208, 27.80170272979929535, 7.433330006724137462 ) ) ;
#60606=CARTESIAN_POINT ( 'NONE',  ( 80.21439583186709399, 44.30090529131236110, 11.38393923939230312 ) ) ;
#60607=CARTESIAN_POINT ( 'NONE',  ( 81.32801083308449108, 55.42016325551186640, -16.33050219934855107 ) ) ;
#60610=CARTESIAN_POINT ( 'NONE',  ( 87.41510241510319190, 45.50646524919893920, 7.075312488460167692 ) ) ;
#60612=ORIENTED_EDGE ( 'NONE', *, *, #36373, .F. ) ;
#60619=CARTESIAN_POINT ( 'NONE',  ( 77.01186407997560934, 60.03506380231930706, -15.92001384120855434 ) ) ;
#60620=CARTESIAN_POINT ( 'NONE',  ( 82.33327191752177043, 40.37251757887272419, 1.340760960699656001 ) ) ;
#60622=CARTESIAN_POINT ( 'NONE',  ( 77.25443146841556086, 63.45523539686509196, -15.12022256747658133 ) ) ;
#60628=CARTESIAN_POINT ( 'NONE',  ( 44.74566838383860556, 28.76004757982093807, 5.678558825948272215 ) ) ;
#60633=CARTESIAN_POINT ( 'NONE',  ( 86.85107213257295200, 45.77346519082802700, -8.718545132792499430 ) ) ;
#60634=PLANE ( 'NONE',  #22104 ) ;
#60647=CARTESIAN_POINT ( 'NONE',  ( 82.65084931856372918, 45.44814966469950690, 10.48390544538666802 ) ) ;
#60651=ORIENTED_EDGE ( 'NONE', *, *, #2847, .F. ) ;
#60653=CARTESIAN_POINT ( 'NONE',  ( 71.49811913338204761, 62.77384012672010272, 13.87084472012334047 ) ) ;
#60659=CARTESIAN_POINT ( 'NONE',  ( 84.63953139824421612, 45.77662167243946101, 9.618633832723032739 ) ) ;
#60662=CARTESIAN_POINT ( 'NONE',  ( 82.69964235597838353, 53.57960405717556540, -15.73923566368025817 ) ) ;
#60670=CARTESIAN_POINT ( 'NONE',  ( 67.61660396824018449, 69.64692688607806303, -0.1948645553118400486 ) ) ;
#60671=CARTESIAN_POINT ( 'NONE',  ( 73.47631802762754205, 69.90797475050369769, -9.735925655486411756 ) ) ;
#60672=DIRECTION ( 'NONE',  ( -0.8660254037844379305, -0.5000000000000014433, -0.000000000000000000 ) ) ;
#60674=DIRECTION ( 'NONE',  ( -0.8660254037844378194, -0.5000000000000014433, -0.000000000000000000 ) ) ;
#60675=CARTESIAN_POINT ( 'NONE',  ( 80.07812099633126479, 57.44764983040322193, -16.59488970948941500 ) ) ;
#60676=CARTESIAN_POINT ( 'NONE',  ( 82.41572850117692894, 54.24742443672926839, 15.60867231807350386 ) ) ;
#60678=CARTESIAN_POINT ( 'NONE',  ( 72.19644594898640833, 72.08809165107794570, 3.016574430004901775 ) ) ;
#60684=B_SPLINE_CURVE_WITH_KNOTS ( 'NONE', 3,
 ( #19453, #12839, #20428, #11835, #43699, #97925, #50309, #81262, #28500, #35107, #42694, #44190, #21413, #75129, #5704, #90861, #36595, #67499, #83236, #44683, #73625, #4210, #75615, #6204, #91840, #7191, #53296, #61878, #68495, #84249, #76605 ),
 .UNSPECIFIED., .F., .F.,
 ( 4, 3, 3, 3, 3, 3, 3, 3, 3, 3, 4 ),
 ( 0.000000000000000000, 0.1333490885032384554, 0.3007194338854541904, 0.4699862290245523377, 0.5844252810809684728, 0.6686540514502963273, 0.7354980260655706870, 0.8028463152565942229, 0.8633854507757449115, 0.9437142632667596676, 1.000000000000000000 ),
 .UNSPECIFIED. ) ;
#60689=CARTESIAN_POINT ( 'NONE',  ( 20.11807774711229868, 23.56628583063840665, 9.188101187500006262 ) ) ;
#60692=CARTESIAN_POINT ( 'NONE',  ( 35.61831302110521591, 44.65659080271453263, -1.878358725466461243E-16 ) ) ;
#60695=CARTESIAN_POINT ( 'NONE',  ( 75.45705218706063988, 56.32278965122512204, 16.59324974296169941 ) ) ;
#60697=CARTESIAN_POINT ( 'NONE',  ( 82.51842583923367158, 41.01935388997881660, -1.203081695168224607 ) ) ;
#60711=CARTESIAN_POINT ( 'NONE',  ( 79.26634259771995517, 46.14609980727534122, -13.24417246943884585 ) ) ;
#60713=CARTESIAN_POINT ( 'NONE',  ( 73.05865758147265865, 70.45434667956401142, -8.047668221016442303 ) ) ;
#60716=CARTESIAN_POINT ( 'NONE',  ( 26.03951966209473312, 17.96004757982090538, -5.678558825948275768 ) ) ;
#60717=CARTESIAN_POINT ( 'NONE',  ( 75.46625377326144246, 57.04332640536068055, 16.11435909797048538 ) ) ;
#60725=ORIENTED_EDGE ( 'NONE', *, *, #62312, .T. ) ;
#60726=CARTESIAN_POINT ( 'NONE',  ( 80.68086640182862368, 49.71203738446756404, -14.26703970971597357 ) ) ;
#60744=ORIENTED_EDGE ( 'NONE', *, *, #410, .T. ) ;
#60747=CARTESIAN_POINT ( 'NONE',  ( 66.94215247483215592, 67.56144765985021650, 6.663993637373098800 ) ) ;
#60753=CARTESIAN_POINT ( 'NONE',  ( 87.49951909536234496, 45.04593868083598807, 6.937257679092508234 ) ) ;
#60754=ORIENTED_EDGE ( 'NONE', *, *, #97908, .T. ) ;
#60760=CARTESIAN_POINT ( 'NONE',  ( 76.10854616902780378, 51.47353040525071322, -15.66966529414775344 ) ) ;
#60761=CARTESIAN_POINT ( 'NONE',  ( 76.01570425163725986, 65.59347775405139203, -14.29814048726880316 ) ) ;
#60772=CARTESIAN_POINT ( 'NONE',  ( 72.96752522106987726, 70.88037482455226268, 8.005050465142900862 ) ) ;
#60777=DIRECTION ( 'NONE',  ( -0.5295078238379101743, -0.5024823063052971106, 0.6834712842135728383 ) ) ;
#60778=CARTESIAN_POINT ( 'NONE',  ( 79.78458617808020392, 47.16083178010686794, 13.11770283550262128 ) ) ;
#60789=CARTESIAN_POINT ( 'NONE',  ( 26.22111236500157361, 16.10801979619929369, 3.090169943749476733 ) ) ;
#60801=CARTESIAN_POINT ( 'NONE',  ( 66.67858973989486060, 68.09147666472189542, -6.506024203352879454 ) ) ;
#60802=CARTESIAN_POINT ( 'NONE',  ( 72.81549581358450496, 70.27905260404436660, -8.103349982428230902 ) ) ;
#60807=CARTESIAN_POINT ( 'NONE',  ( 20.61848683307935914, 34.83705186507754803, 3.090169943749475401 ) ) ;
#60808=CARTESIAN_POINT ( 'NONE',  ( 85.63218110832043806, 48.66108713908771932, 12.42024371201311972 ) ) ;
#60810=CARTESIAN_POINT ( 'NONE',  ( 72.08668889666979851, 71.79979336344656815, -3.927014794161233890 ) ) ;
#60819=CARTESIAN_POINT ( 'NONE',  ( 72.67106054446416863, 70.72958228892086652, -7.972900045040105077 ) ) ;
#60821=CARTESIAN_POINT ( 'NONE',  ( 77.36600796148924530, 49.13692148722834929, -14.77749963168140113 ) ) ;
#60830=CARTESIAN_POINT ( 'NONE',  ( 16.40018271037384068, 27.65586893147755987, -7.433330006724137462 ) ) ;
#60831=CARTESIAN_POINT ( 'NONE',  ( 15.40662013169548672, 9.864269794150882120, -3.090169943749474069 ) ) ;
#60832=CARTESIAN_POINT ( 'NONE',  ( 71.41401697283629346, 59.26550905095592725, 15.24935196003983329 ) ) ;
#60837=VECTOR ( 'NONE', #23531, 1000.000000000000000 ) ;
#60840=FACE_OUTER_BOUND ( 'NONE', #46896, .T. ) ;
#60842=PLANE ( 'NONE',  #52207 ) ;
#60843=CARTESIAN_POINT ( 'NONE',  ( 71.99578165902696014, 71.45753870159522592, -4.731601630015590310 ) ) ;
#60844=CARTESIAN_POINT ( 'NONE',  ( 77.23262995875991521, 63.36386537804837360, 15.13973818951359007 ) ) ;
#60860=ORIENTED_EDGE ( 'NONE', *, *, #58748, .T. ) ;
#60863=CARTESIAN_POINT ( 'NONE',  ( 75.25170673533752108, 66.73598490943447814, 12.94887977284632896 ) ) ;
#60871=CARTESIAN_POINT ( 'NONE',  ( 78.22627483185729602, 47.75561434913958436, -14.49489253473961092 ) ) ;
#60872=CARTESIAN_POINT ( 'NONE',  ( 83.83559978620640152, 51.92718615610179711, 14.52128790932804137 ) ) ;
#60876=CARTESIAN_POINT ( 'NONE',  ( 80.86872469022158327, 51.16822586326628652, -15.30852264838738108 ) ) ;
#60884=B_SPLINE_CURVE_WITH_KNOTS ( 'NONE', 3,
 ( #95624, #50455, #97584, #35758, #89997, #20573, #51451, #82420, #26173, #10985, #41857, #72802, #38218, #84880, #30651, #91996, #75271, #53918, #99069, #61535, #68637, #74784, #21559, #51959, #5364, #90997, #92478, #52441, #22547, #14929, #5856, #45337, #75769, #36741, #36245, #13955, #43845, #76269, #68141, #82899, #6357, #6842, #67647, #29162, #37243, #90510 ),
 .UNSPECIFIED., .F., .F.,
 ( 4, 1, 2, 2, 1, 2, 2, 1, 1, 2, 2, 1, 1, 2, 2, 1, 1, 2, 2, 1, 1, 1, 2, 2, 1, 1, 1, 2, 2, 4 ),
 ( 0.000000000000000000, 0.06249999999998620548, 0.09374999999997919720, 0.1249999999999721889, 0.1874999999999613365, 0.2187499999999554523, 0.2499999999999495959, 0.3124999999999385492, 0.3437499999999330536, 0.3593749999999300004, 0.3749999999999269473, 0.4374999999999178990, 0.4687499999999141798, 0.4843749999999123479, 0.4999999999999105160, 0.5624999999999169553, 0.5937499999999182876, 0.6093749999999193978, 0.6249999999999203970, 0.6874999999999228395, 0.7187499999999235056, 0.7343749999999257261, 0.7421874999999290567, 0.7499999999999322764, 0.8124999999999713562, 0.8437499999999910072, 0.8593750000000005551, 0.8671875000000035527, 0.8750000000000065503, 1.000000000000000000 ),
 .UNSPECIFIED. ) ;
#60887=CARTESIAN_POINT ( 'NONE',  ( 70.25033766539972646, 68.19075070162745078, 8.808644737539518488 ) ) ;
#60889=CARTESIAN_POINT ( 'NONE',  ( 67.12762392158883529, 66.70947246983655532, 8.261873050784338091 ) ) ;
#60891=CARTESIAN_POINT ( 'NONE',  ( 78.37377739669621235, 47.42489695864805554, 14.28740524439509230 ) ) ;
#60895=CARTESIAN_POINT ( 'NONE',  ( 80.28604642359979948, 52.75975974871795415, -15.47868605385456497 ) ) ;
#60898=CARTESIAN_POINT ( 'NONE',  ( 79.11953551025055731, 46.13320601581522595, 12.69056890641700086 ) ) ;
#60902=CARTESIAN_POINT ( 'NONE',  ( 69.26382730489497419, 65.05794468884164417, -11.47466192821767805 ) ) ;
#60906=CARTESIAN_POINT ( 'NONE',  ( 72.16868224958085420, 71.71251872039211150, 5.498261171115592205 ) ) ;
#60910=DIRECTION ( 'NONE',  ( -0.8660254037844377084, -0.5000000000000014433, -0.000000000000000000 ) ) ;
#60923=VECTOR ( 'NONE', #56419, 1000.000000000000114 ) ;
#60925=CARTESIAN_POINT ( 'NONE',  ( 81.93485011922251715, 41.32099105351304758, -5.877334436009162388 ) ) ;
#60926=CARTESIAN_POINT ( 'NONE',  ( 76.45572749640669485, 51.64231386250387601, -16.15369532800221108 ) ) ;
#60927=CARTESIAN_POINT ( 'NONE',  ( 68.68909986782581711, 64.16576715805911135, -12.55144644517788421 ) ) ;
#60930=DIRECTION ( 'NONE',  ( 0.7691052716734813055, 0.08748735329024863450, 0.6331058711608413825 ) ) ;
#60933=EDGE_CURVE ( 'NONE', #24489, #69981, #65289, .T. ) ;
#60939=CARTESIAN_POINT ( 'NONE',  ( 7.004301291108590455, 25.81751292744054282, -6.180339887498951690 ) ) ;
#60943=CARTESIAN_POINT ( 'NONE',  ( 73.13555747811004437, 69.81939941050913490, 9.605153593488003239 ) ) ;
#60948=CARTESIAN_POINT ( 'NONE',  ( 72.58511477355777686, 57.25044146139839540, 15.86244954290823017 ) ) ;
#60956=CARTESIAN_POINT ( 'NONE',  ( 35.39919958817179690, 22.29860640527294535, -2.839279412974138328 ) ) ;
#60959=CARTESIAN_POINT ( 'NONE',  ( 75.12085108667970701, 52.90659536716842126, -15.99877795348665011 ) ) ;
#60967=LINE ( 'NONE', #62452, #79058 ) ;
#60968=CARTESIAN_POINT ( 'NONE',  ( 12.16146256644911716, 9.947547579820875896, 5.678558825948272215 ) ) ;
#60979=CARTESIAN_POINT ( 'NONE',  ( 10.55946980724658069, 24.83478043621386888, -8.090169943749479842 ) ) ;
#60980=CARTESIAN_POINT ( 'NONE',  ( 86.70911053808110580, 46.89117940024963360, 10.21290512048939014 ) ) ;
#60983=CARTESIAN_POINT ( 'NONE',  ( 86.54659259230355417, 47.35344409918261732, -10.80230753912617914 ) ) ;
#60985=EDGE_LOOP ( 'NONE', ( #67582, #27977, #9602, #49299 ) ) ;
#60990=CARTESIAN_POINT ( 'NONE',  ( 69.94772996192264713, 62.88149894362739190, 13.87021638775245336 ) ) ;
#60994=CARTESIAN_POINT ( 'NONE',  ( 81.22534965261213813, 42.38499988906294647, -7.548277495761163358 ) ) ;
#60998=CARTESIAN_POINT ( 'NONE',  ( 81.90811180363191113, 52.66149361526625938, 15.20919891352879993 ) ) ;
#61000=CARTESIAN_POINT ( 'NONE',  ( 68.31157111924099468, 68.55647029866582898, 6.335902121074872717 ) ) ;
#61007=CARTESIAN_POINT ( 'NONE',  ( 82.86418038935372010, 53.70170152444392642, -15.38246542855200261 ) ) ;
#61008=CARTESIAN_POINT ( 'NONE',  ( 75.28641870618297105, 56.93067274799551569, -16.55615621114917957 ) ) ;
#61009=CARTESIAN_POINT ( 'NONE',  ( 16.25825050073692069, 15.10170272979925876, -7.433330006724141015 ) ) ;
#61018=CARTESIAN_POINT ( 'NONE',  ( 80.00173192732594885, 44.68233805328101482, 11.15140268308046601 ) ) ;
#61026=CARTESIAN_POINT ( 'NONE',  ( 75.03771487841180488, 67.29470115673238695, -12.93936238812017336 ) ) ;
#61029=B_SPLINE_CURVE_WITH_KNOTS ( 'NONE', 3,
 ( #47691, #17305, #70501, #31993, #94843, #41088, #62903, #16804, #48209, #40086, #25404, #56295, #92841, #77629, #1632, #17823, #10220, #31001, #61890, #56800, #26913, #95861, #88269, #87785 ),
 .UNSPECIFIED., .F., .F.,
 ( 4, 2, 2, 2, 2, 2, 2, 2, 2, 2, 2, 4 ),
 ( 0.000000000000000000, 0.1250000000000054123, 0.2500000000000108247, 0.3750000000000162093, 0.4375000000000207057, 0.5000000000000252021, 0.5625000000000296430, 0.6250000000000341949, 0.6875000000000386358, 0.7500000000000431877, 0.8750000000000215383, 1.000000000000000000 ),
 .UNSPECIFIED. ) ;
#61033=CARTESIAN_POINT ( 'NONE',  ( 86.19940314562042261, 44.63913117227356508, -6.631687147223989776 ) ) ;
#61036=CARTESIAN_POINT ( 'NONE',  ( 24.34666095796415419, 37.55466486950700755, 7.012934429366973338E-14 ) ) ;
#61042=CARTESIAN_POINT ( 'NONE',  ( 84.15081258030213007, 46.26608709097053662, -10.48838324873663019 ) ) ;
#61057=CARTESIAN_POINT ( 'NONE',  ( 77.86314341856081001, 54.34344560458549012, -16.01061743008826355 ) ) ;
#61066=CARTESIAN_POINT ( 'NONE',  ( 68.71908087017774847, 68.45513031344326293, 6.959568858202175967 ) ) ;
#61075=DIRECTION ( 'NONE',  ( -0.2702110370271911810, -0.9515975153008192633, -0.1464519181915933110 ) ) ;
#61082=CARTESIAN_POINT ( 'NONE',  ( 41.95273645663377948, 27.14754757982093381, -5.678558825948275768 ) ) ;
#61086=CARTESIAN_POINT ( 'NONE',  ( 28.77833178495667710, 28.56628583063842441, 9.188101187500006262 ) ) ;
#61088=CARTESIAN_POINT ( 'NONE',  ( 70.81027263193901433, 64.39395113940368276, -13.25098958810220395 ) ) ;
#61091=CARTESIAN_POINT ( 'NONE',  ( 84.81216594078708226, 50.08139507223255293, -13.70157583983569971 ) ) ;
#61092=CARTESIAN_POINT ( 'NONE',  ( 76.01947567912945658, 65.31078134063972129, -14.44091581795174051 ) ) ;
#61099=CARTESIAN_POINT ( 'NONE',  ( 28.93411276635479368, 38.74646525600392266, 2.839279412974139660 ) ) ;
#61105=CARTESIAN_POINT ( 'NONE',  ( 86.52685127962818967, 47.39493317473652212, -10.85533565734824890 ) ) ;
#61110=CARTESIAN_POINT ( 'NONE',  ( 35.97235683590213284, 38.95586893147758190, 7.433330006724141015 ) ) ;
#61111=FACE_OUTER_BOUND ( 'NONE', #90220, .T. ) ;
#61119=CARTESIAN_POINT ( 'NONE',  ( 86.86990765421666083, 45.77415147683691288, -8.704208088459520098 ) ) ;
#61120=CARTESIAN_POINT ( 'NONE',  ( 79.74434664762874547, 56.88260642345687756, 16.21928422613826370 ) ) ;
#61121=PLANE ( 'NONE',  #56812 ) ;
#61125=CARTESIAN_POINT ( 'NONE',  ( 74.80133982707299367, 60.85566197117798026, -15.41540466998751846 ) ) ;
#61127=VECTOR ( 'NONE', #50376, 1000.000000000000114 ) ;
#61129=CARTESIAN_POINT ( 'NONE',  ( 76.82578666445662918, 64.07401149769333415, -15.18382690731647600 ) ) ;
#61135=CARTESIAN_POINT ( 'NONE',  ( 38.30580752471379213, 37.51421378149922958, -9.188101187500004485 ) ) ;
#61140=CARTESIAN_POINT ( 'NONE',  ( 73.97927654802940367, 68.30869415006648637, -11.66811813765111516 ) ) ;
#61146=EDGE_LOOP ( 'NONE', ( #92489, #53049, #45241, #73246 ) ) ;
#61155=AXIS2_PLACEMENT_3D ( 'NONE', #61863, #61373, #31468 ) ;
#61163=ORIENTED_EDGE ( 'NONE', *, *, #74763, .F. ) ;
#61166=CARTESIAN_POINT ( 'NONE',  ( 72.77247963031311428, 66.86076665135031760, 11.73453098109765058 ) ) ;
#61167=CARTESIAN_POINT ( 'NONE',  ( 82.31724296769202454, 41.27996126847105529, -3.439593570527449629 ) ) ;
#61175=VECTOR ( 'NONE', #48238, 1000.000000000000114 ) ;
#61177=CARTESIAN_POINT ( 'NONE',  ( 82.54140815357128247, 53.47864718817667296, -15.73643156343348259 ) ) ;
#61182=CARTESIAN_POINT ( 'NONE',  ( 66.45995819386082815, 67.97305414892089459, 6.490190279896535408 ) ) ;
#61185=CARTESIAN_POINT ( 'NONE',  ( 73.42123007364070020, 69.75766128465485849, -9.876216450746401421 ) ) ;
#61186=CARTESIAN_POINT ( 'NONE',  ( 76.41050813019120369, 51.44656437704933438, 15.62581973270596514 ) ) ;
#61188=CARTESIAN_POINT ( 'NONE',  ( 45.27367124825920541, 27.10801979619933277, 3.090169943749476733 ) ) ;
#61191=CARTESIAN_POINT ( 'NONE',  ( 72.14978007694548978, 72.25075206688683238, 3.885827817524740713 ) ) ;
#61196=CARTESIAN_POINT ( 'NONE',  ( 81.64670023727850889, 42.65128533460878657, -7.584980231169042852 ) ) ;
#61198=CARTESIAN_POINT ( 'NONE',  ( 80.02673061647857367, 50.59600265380255024, -14.77882822326097845 ) ) ;
#61203=CARTESIAN_POINT ( 'NONE',  ( 23.51121325743158508, 19.28920272979927120, -7.433330006724141015 ) ) ;
#61206=CARTESIAN_POINT ( 'NONE',  ( 14.61458989734527947, 10.29860640527290805, -2.839279412974138328 ) ) ;
#61208=CARTESIAN_POINT ( 'NONE',  ( 77.27782791576461818, 63.42193016440150899, 15.51014190020122641 ) ) ;
#61209=CARTESIAN_POINT ( 'NONE',  ( 76.57849375015202043, 63.06061772104433771, 15.49930747022867195 ) ) ;
#61212=CARTESIAN_POINT ( 'NONE',  ( 72.67360971685785387, 61.67685437178258212, 14.68373298776349856 ) ) ;
#61214=CARTESIAN_POINT ( 'NONE',  ( 77.35066759761136268, 56.08440499094516696, -16.16557419915228166 ) ) ;
#61215=VECTOR ( 'NONE', #86502, 1000.000000000000000 ) ;
#61216=CARTESIAN_POINT ( 'NONE',  ( 87.77948443791279942, 45.22530890134208903, -6.970560438077714416 ) ) ;
#61221=CARTESIAN_POINT ( 'NONE',  ( 76.92172728274191229, 49.74558783373824156, 15.08244268300244784 ) ) ;
#61227=CARTESIAN_POINT ( 'NONE',  ( 79.09449567167088446, 45.94901772720934474, -12.57695653887258480 ) ) ;
#61232=CARTESIAN_POINT ( 'NONE',  ( 15.27916758686040311, 29.79752408145592568, -5.678558825948271327 ) ) ;
#61233=CARTESIAN_POINT ( 'NONE',  ( 75.19925724589786853, 55.75564056399659307, 16.15125504434804782 ) ) ;
#61242=CARTESIAN_POINT ( 'NONE',  ( 68.13485488127290068, 65.64062842649776996, -10.28058960440808534 ) ) ;
#61259=CARTESIAN_POINT ( 'NONE',  ( 67.08790609839790875, 67.65794649167050068, 6.640929181028614181 ) ) ;
#61262=CARTESIAN_POINT ( 'NONE',  ( 81.18434463996317163, 55.62183548715842107, 16.37412944077603782 ) ) ;
#61265=CARTESIAN_POINT ( 'NONE',  ( 70.57311072637669724, 64.37600167932460238, 12.58562827297202347 ) ) ;
#61268=EDGE_CURVE ( 'NONE', #32407, #38046, #2587, .T. ) ;
#61272=CARTESIAN_POINT ( 'NONE',  ( 76.09263634981390112, 51.44000213080718709, -15.66469206649365198 ) ) ;
#61273=EDGE_CURVE ( 'NONE', #94177, #52768, #4839, .T. ) ;
#61275=B_SPLINE_CURVE_WITH_KNOTS ( 'NONE', 3,
 ( #3794, #11413, #65082, #89437, #43262, #74707, #58465, #57468, #13392, #19992, #80843, #19010, #81821, #4797, #12396, #88451 ),
 .UNSPECIFIED., .F., .F.,
 ( 4, 1, 2, 2, 2, 1, 2, 2, 4 ),
 ( 0.000000000000000000, 0.1250000000000012768, 0.1875000000000005829, 0.2499999999999998890, 0.4999999999999976685, 0.6249999999999978906, 0.6874999999999987788, 0.7499999999999996669, 1.000000000000000000 ),
 .UNSPECIFIED. ) ;
#61277=CARTESIAN_POINT ( 'NONE',  ( 75.80192922086310148, 65.84738460970490337, -14.09986028324621898 ) ) ;
#61283=VECTOR ( 'NONE', #21759, 1000.000000000000114 ) ;
#61285=CARTESIAN_POINT ( 'NONE',  ( 87.73298548431468191, 44.18903561216112763, 4.633618514853090176 ) ) ;
#61287=CARTESIAN_POINT ( 'NONE',  ( 88.07576543976308869, 43.78748546321877910, -2.154750241475199335 ) ) ;
#61289=CARTESIAN_POINT ( 'NONE',  ( 79.51501685758188387, 59.30344737611886075, -16.21767406144808987 ) ) ;
#61290=CARTESIAN_POINT ( 'NONE',  ( 72.78409883976615902, 66.98531790838794109, -11.66862470457359002 ) ) ;
#61295=CARTESIAN_POINT ( 'NONE',  ( 82.11473172643496810, 40.78303678057567083, 1.182234453112787298 ) ) ;
#61296=CARTESIAN_POINT ( 'NONE',  ( 79.56975053609437509, 46.55862065107593395, 12.80488734779169846 ) ) ;
#61297=CARTESIAN_POINT ( 'NONE',  ( 83.29275869314055569, 52.39031112279613467, 14.85814565312617397 ) ) ;
#61305=CARTESIAN_POINT ( 'NONE',  ( 81.74119788692269140, 59.14441083166271795, 0.000000000000000000 ) ) ;
#61306=CARTESIAN_POINT ( 'NONE',  ( 26.39431744575845684, 16.20801979619929156, -3.090169943749474069 ) ) ;
#61313=ORIENTED_EDGE ( 'NONE', *, *, #53586, .F. ) ;
#61314=DIRECTION ( 'NONE',  ( 0.8660254037844379305, 0.5000000000000014433, 0.000000000000000000 ) ) ;
#61315=CARTESIAN_POINT ( 'NONE',  ( 72.62340041749850172, 70.70648146094342223, -7.965908336710425530 ) ) ;
#61316=CARTESIAN_POINT ( 'NONE',  ( 81.85549098805211088, 41.30720913978863962, 5.950207739220628511 ) ) ;
#61320=CARTESIAN_POINT ( 'NONE',  ( 33.69734285410222441, 21.58380873178789017, 6.180339887498953466 ) ) ;
#61327=CARTESIAN_POINT ( 'NONE',  ( 82.31762945370437023, 41.36718402847516529, 5.460911063167284141 ) ) ;
#61331=CARTESIAN_POINT ( 'NONE',  ( 72.49337063691619676, 70.67504402769608873, -7.896386945446496775 ) ) ;
#61334=CARTESIAN_POINT ( 'NONE',  ( 42.70206918026080700, 25.44966523072497822, -2.296566073217252530E-15 ) ) ;
#61342=CARTESIAN_POINT ( 'NONE',  ( 14.90450122504689823, 30.64646525600389637, -2.839279412974133887 ) ) ;
#61344=CARTESIAN_POINT ( 'NONE',  ( 72.03620616349491002, 59.26415205210582826, 15.35034427320005079 ) ) ;
#61348=CARTESIAN_POINT ( 'NONE',  ( 43.71482552144721723, 26.20801979619932354, -3.090169943749474069 ) ) ;
#61351=CARTESIAN_POINT ( 'NONE',  ( 75.34249057394406179, 53.53749946893489664, -16.04535326226222480 ) ) ;
#61353=CARTESIAN_POINT ( 'NONE',  ( 81.52647152047666168, 42.51558550804076475, 7.474308617801350252 ) ) ;
#61354=ORIENTED_EDGE ( 'NONE', *, *, #80820, .F. ) ;
#61356=CARTESIAN_POINT ( 'NONE',  ( 72.63327417104410699, 71.45201850668806287, -5.742053798226967487 ) ) ;
#61364=ORIENTED_EDGE ( 'NONE', *, *, #40977, .T. ) ;
#61373=DIRECTION ( 'NONE',  ( -0.8660254037844379305, -0.5000000000000014433, -0.000000000000000000 ) ) ;
#61378=CARTESIAN_POINT ( 'NONE',  ( 78.13699514187493378, 47.68854696100831347, -13.93943695986319931 ) ) ;
#61383=CARTESIAN_POINT ( 'NONE',  ( 83.21184101803882527, 52.33542056097268613, 14.85481608591265967 ) ) ;
#61384=VERTEX_POINT ( 'NONE', #73477 ) ;
#61385=ORIENTED_EDGE ( 'NONE', *, *, #87882, .F. ) ;
#61397=CARTESIAN_POINT ( 'NONE',  ( 71.77039740172594406, 70.92856646297812517, 5.774134966689192794 ) ) ;
#61398=CARTESIAN_POINT ( 'NONE',  ( 67.09442320589272413, 69.80147035112786114, 1.451480095758326039 ) ) ;
#61399=CARTESIAN_POINT ( 'NONE',  ( 67.15803325889245912, 66.63036032015114074, 8.397731182079862577 ) ) ;
#61401=CARTESIAN_POINT ( 'NONE',  ( 78.64589612872744340, 47.50488844158302015, 14.24760414073640646 ) ) ;
#61406=CARTESIAN_POINT ( 'NONE',  ( 79.41534452234611763, 46.24203507740502772, 12.64746779647137487 ) ) ;
#61407=CARTESIAN_POINT ( 'NONE',  ( 81.84288204769163144, 58.96828869888589253, -0.4567727288213002668 ) ) ;
#61408=CARTESIAN_POINT ( 'NONE',  ( 72.84093999290328725, 56.97456911652175648, -16.40692799624908815 ) ) ;
#61409=CARTESIAN_POINT ( 'NONE',  ( 68.10039974585599509, 65.18542567973287305, -10.72853162865224519 ) ) ;
#61413=CARTESIAN_POINT ( 'NONE',  ( 72.49520321802694411, 71.62171839754151392, 6.144630347475415810 ) ) ;
#61418=CARTESIAN_POINT ( 'NONE',  ( 66.85822330536446145, 67.61959507708256467, -6.456617525293864013 ) ) ;
#61423=CARTESIAN_POINT ( 'NONE',  ( 85.68664465223866955, 48.45350732935998650, -12.23334744974732402 ) ) ;
#61439=AXIS2_PLACEMENT_3D ( 'NONE', #63102, #31196, #24102 ) ;
#61442=CARTESIAN_POINT ( 'NONE',  ( 13.25914332478948410, 9.783808731787853930, -6.180339887498949025 ) ) ;
#61445=CARTESIAN_POINT ( 'NONE',  ( 73.03785937943386841, 69.69865149502336976, 9.683281169778272357 ) ) ;
#61450=CARTESIAN_POINT ( 'NONE',  ( 72.53392300481422694, 57.31226291295279651, 15.84842549994240990 ) ) ;
#61452=CARTESIAN_POINT ( 'NONE',  ( 8.758203689844268780, 28.55466486950697913, -1.111400068045478839E-16 ) ) ;
#61453=ORIENTED_EDGE ( 'NONE', *, *, #81668, .T. ) ;
#61458=CARTESIAN_POINT ( 'NONE',  ( 34.51455378690028652, 28.43085787977765477, -9.188101187500008038 ) ) ;
#61462=CARTESIAN_POINT ( 'NONE',  ( 74.94213196210210981, 53.20634399479197896, -16.03712342241558275 ) ) ;
#61463=CARTESIAN_POINT ( 'NONE',  ( 70.32223144932660830, 70.48993496229302025, 5.907123158273768659 ) ) ;
#61465=CARTESIAN_POINT ( 'NONE',  ( 68.55596672819507376, 64.28337496226291137, 12.40357123185196819 ) ) ;
#61469=CARTESIAN_POINT ( 'NONE',  ( 6.802937163926562114, 15.87878583063839066, -9.188101187500006262 ) ) ;
#61471=CARTESIAN_POINT ( 'NONE',  ( 7.290083236948965428, 25.18502408145589655, 5.678558825948276656 ) ) ;
#61475=CARTESIAN_POINT ( 'NONE',  ( 69.53667171941721392, 62.56887577352630814, 13.34165820888200216 ) ) ;
#61484=CARTESIAN_POINT ( 'NONE',  ( 72.48280754011685190, 70.60311863597817705, 7.264376673680498442 ) ) ;
#61488=CARTESIAN_POINT ( 'NONE',  ( 81.59902824993105241, 45.46755018456938302, -11.06827361697009060 ) ) ;
#61494=CARTESIAN_POINT ( 'NONE',  ( 69.33571648121584019, 62.94790354691227918, 13.62394890031374572 ) ) ;
#61501=ORIENTED_EDGE ( 'NONE', *, *, #82054, .F. ) ;
#61505=CARTESIAN_POINT ( 'NONE',  ( 73.99038332904399340, 64.06192407381385578, 14.02288482052439456 ) ) ;
#61512=FACE_OUTER_BOUND ( 'NONE', #26495, .T. ) ;
#61516=CARTESIAN_POINT ( 'NONE',  ( 82.56047309644807797, 54.07683023134061528, -15.52634518316282097 ) ) ;
#61518=CARTESIAN_POINT ( 'NONE',  ( 74.04864439501488960, 57.31504094317030251, -16.45781754585126677 ) ) ;
#61519=CARTESIAN_POINT ( 'NONE',  ( 10.08301516415377641, 26.79752408145591147, -5.678558825948271327 ) ) ;
#61521=CARTESIAN_POINT ( 'NONE',  ( 80.12283971196008281, 57.76720862780120314, 16.60271659255639065 ) ) ;
#61522=FACE_OUTER_BOUND ( 'NONE', #62971, .T. ) ;
#61530=CARTESIAN_POINT ( 'NONE',  ( 67.95331009947700807, 66.07265274243333408, -10.46626145091951621 ) ) ;
#61535=CARTESIAN_POINT ( 'NONE',  ( 73.89769204157855143, 62.62724885997820934, -14.63212924024895933 ) ) ;
#61543=CARTESIAN_POINT ( 'NONE',  ( 87.79103858326931231, 44.11529954957103428, 2.696194862051933150 ) ) ;
#61549=CARTESIAN_POINT ( 'NONE',  ( 84.68093819348166562, 42.16537887657799644, 0.2499978311480390847 ) ) ;
#61551=CARTESIAN_POINT ( 'NONE',  ( 82.68581151109542304, 43.22490338220254102, 7.598561826035989064 ) ) ;
#61559=CARTESIAN_POINT ( 'NONE',  ( 76.38284716662768403, 54.82274627456094152, -16.11362980023774227 ) ) ;
#61560=CARTESIAN_POINT ( 'NONE',  ( 80.57046890446221710, 57.17601910317578984, -16.22952344167990901 ) ) ;
#61567=CARTESIAN_POINT ( 'NONE',  ( 68.74125309881081591, 68.48789582852654689, 6.924389039908457555 ) ) ;
#61574=CARTESIAN_POINT ( 'NONE',  ( 13.03712377304622194, 16.03085787977761356, 9.188101187500006262 ) ) ;
#61575=CARTESIAN_POINT ( 'NONE',  ( 74.83655476910676896, 53.51806293180212037, 16.54630480343736920 ) ) ;
#61584=DIRECTION ( 'NONE',  ( 0.9532659690011938691, -0.2314883312386622760, 0.1941575258509293800 ) ) ;
#61585=CARTESIAN_POINT ( 'NONE',  ( 86.33473264480980447, 47.64805230391016977, 10.69327747295855247 ) ) ;
#61587=CARTESIAN_POINT ( 'NONE',  ( 33.49394369984602804, 21.19860640527294038, 2.839279412974134775 ) ) ;
#61593=EDGE_CURVE ( 'NONE', #87380, #45306, #79870, .T. ) ;
#61594=CARTESIAN_POINT ( 'NONE',  ( 84.48836950856804151, 49.89909654526366722, -13.70430404532020319 ) ) ;
#61595=CARTESIAN_POINT ( 'NONE',  ( 78.72343666810984075, 48.48097556600880864, 14.16619407085236837 ) ) ;
#61600=CARTESIAN_POINT ( 'NONE',  ( 73.64088816139484095, 69.63733386616164012, 10.15931356738738423 ) ) ;
#61601=CARTESIAN_POINT ( 'NONE',  ( 27.02885687802902837, 37.64646525600391413, -2.839279412974133887 ) ) ;
#61603=CARTESIAN_POINT ( 'NONE',  ( 84.37825102736907468, 49.99960613749294680, 13.80049582259581520 ) ) ;
#61606=CARTESIAN_POINT ( 'NONE',  ( 86.53913842531343903, 47.33648749047813453, -10.24973804167819935 ) ) ;
#61608=CARTESIAN_POINT ( 'NONE',  ( 84.56695678370634539, 50.23807730109928826, 13.87492620287773804 ) ) ;
#61611=CARTESIAN_POINT ( 'NONE',  ( 86.26411663623493098, 44.87056880271241255, -7.873569013553530560 ) ) ;
#61612=CARTESIAN_POINT ( 'NONE',  ( 80.24827019267925721, 44.30331806697298447, 11.36816880119114437 ) ) ;
#61613=CARTESIAN_POINT ( 'NONE',  ( 79.14312167556931854, 57.64441083166269664, 0.000000000000000000 ) ) ;
#61627=CARTESIAN_POINT ( 'NONE',  ( 78.90549422596571105, 46.47045305960070039, 12.99985401326298984 ) ) ;
#61629=CARTESIAN_POINT ( 'NONE',  ( 76.69634485559663517, 63.33187278031594758, -15.42689205524521157 ) ) ;
#61634=CARTESIAN_POINT ( 'NONE',  ( 70.73253466316766946, 60.52854348683570151, -14.67665510802405748 ) ) ;
#61637=ORIENTED_EDGE ( 'NONE', *, *, #99957, .F. ) ;
#61641=CARTESIAN_POINT ( 'NONE',  ( 73.88216889899386786, 63.33152347620602285, -14.31039344191799323 ) ) ;
#61645=CARTESIAN_POINT ( 'NONE',  ( 73.60132943463672461, 67.75729915613128185, 11.45358097554368904 ) ) ;
#61647=CARTESIAN_POINT ( 'NONE',  ( 73.92365886092795790, 54.91122253338699011, -16.13237890612813885 ) ) ;
#61659=CARTESIAN_POINT ( 'NONE',  ( 81.50391902668040700, 43.19956922895749329, 8.559400874430535211 ) ) ;
#61661=CARTESIAN_POINT ( 'NONE',  ( 69.81582973446273854, 63.14295414325376044, -13.67321376832284230 ) ) ;
#61670=CARTESIAN_POINT ( 'NONE',  ( 83.20126876621219481, 43.26424907438605771, 7.146979139294720618 ) ) ;
#61672=CARTESIAN_POINT ( 'NONE',  ( 11.39698775767666916, 6.984156793818252495, 0.000000000000000000 ) ) ;
#61673=CARTESIAN_POINT ( 'NONE',  ( 72.88043634756726874, 66.05899410211006284, -12.94925710025703758 ) ) ;
#61682=DIRECTION ( 'NONE',  ( -0.8660254037844377084, -0.5000000000000015543, -0.000000000000000000 ) ) ;
#61683=CARTESIAN_POINT ( 'NONE',  ( 73.47333430897622009, 69.87645613598228067, -9.771583980831868743 ) ) ;
#61684=CARTESIAN_POINT ( 'NONE',  ( 76.51704343084249160, 51.19216947614988555, 16.04754391915694001 ) ) ;
#61692=CARTESIAN_POINT ( 'NONE',  ( 88.03872450704908204, 44.00635692270125787, 0.5520354079413645199 ) ) ;
#61694=CARTESIAN_POINT ( 'NONE',  ( 79.43825615163621023, 50.76615999754224617, -14.96098264411816103 ) ) ;
#61698=CARTESIAN_POINT ( 'NONE',  ( 18.69336236660381090, 32.83396525600390703, -2.839279412974133887 ) ) ;
#61701=CARTESIAN_POINT ( 'NONE',  ( 11.45782370926791849, 18.56628583063839244, 9.188101187500006262 ) ) ;
#61713=CARTESIAN_POINT ( 'NONE',  ( 81.39852127369077550, 54.56569132021830626, -15.77998593897333635 ) ) ;
#61718=FACE_OUTER_BOUND ( 'NONE', #47066, .T. ) ;
#61723=CARTESIAN_POINT ( 'NONE',  ( 69.52010333882432747, 68.86091139190541810, -7.091978748607149718 ) ) ;
#61726=CARTESIAN_POINT ( 'NONE',  ( 79.23755946070403411, 46.33870301756119403, -12.78202225028572236 ) ) ;
#61730=CARTESIAN_POINT ( 'NONE',  ( 24.98947064339976265, 26.37878583063841731, 9.188101187500006262 ) ) ;
#61731=CARTESIAN_POINT ( 'NONE',  ( 74.73487060833782891, 53.69418506457893869, 16.08953207461605928 ) ) ;
#61733=CARTESIAN_POINT ( 'NONE',  ( 75.26246398335119636, 66.91264289108335106, -12.84364210877655132 ) ) ;
#61741=CARTESIAN_POINT ( 'NONE',  ( 71.63504328546106592, 65.51313058377321852, 12.81449884532781702 ) ) ;
#61742=CARTESIAN_POINT ( 'NONE',  ( 68.10299200362963745, 65.62433957351714753, -10.27834201520733615 ) ) ;
#61755=ORIENTED_EDGE ( 'NONE', *, *, #36832, .T. ) ;
#61757=ORIENTED_EDGE ( 'NONE', *, *, #63923, .F. ) ;
#61759=CARTESIAN_POINT ( 'NONE',  ( 66.67403404533332889, 67.50885822679623516, 6.470379398463248499 ) ) ;
#61766=CARTESIAN_POINT ( 'NONE',  ( 72.01025194461936962, 68.18098373561990400, 10.06619654333739611 ) ) ;
#61768=VERTEX_POINT ( 'NONE', #91079 ) ;
#61770=CARTESIAN_POINT ( 'NONE',  ( 18.71539827744147644, 26.50829794293879971, -10.00000000000000355 ) ) ;
#61772=EDGE_LOOP ( 'NONE', ( #56462, #85660, #15537, #34800 ) ) ;
#61773=CARTESIAN_POINT ( 'NONE',  ( 15.24912932961584744, 31.73705186507753950, -3.090169943749475845 ) ) ;
#61775=CARTESIAN_POINT ( 'NONE',  ( 75.75493378409400691, 65.86437009324527025, -14.07593894684413449 ) ) ;
#61781=CARTESIAN_POINT ( 'NONE',  ( 83.93224464401249918, 43.69151124717017609, -7.184054031788095429 ) ) ;
#61782=CARTESIAN_POINT ( 'NONE',  ( 32.74284248606149106, 41.83705186507756224, 3.090169943749475401 ) ) ;
#61785=CARTESIAN_POINT ( 'NONE',  ( 79.37421766178685800, 59.09322915855462099, -16.22839383466721230 ) ) ;
#61786=CARTESIAN_POINT ( 'NONE',  ( 71.77304829242562789, 67.17973620888965058, -10.95076504957269314 ) ) ;
#61792=CARTESIAN_POINT ( 'NONE',  ( 83.43509040966195300, 52.41314640276721804, 14.83374206111990468 ) ) ;
#61799=CARTESIAN_POINT ( 'NONE',  ( 74.02712935233476799, 55.22068333997034983, 16.12340877065539502 ) ) ;
#61800=CARTESIAN_POINT ( 'NONE',  ( 21.98544502579644799, 24.64441083166261137, -10.00000000000000533 ) ) ;
#61808=CARTESIAN_POINT ( 'NONE',  ( 66.92722021384717834, 67.66083605152657299, -6.453759971695879116 ) ) ;
#61809=CARTESIAN_POINT ( 'NONE',  ( 72.67106054446415442, 70.72958228892088073, -7.972900045040099748 ) ) ;
#61812=CARTESIAN_POINT ( 'NONE',  ( 75.37455147550954848, 53.49333803353913197, 16.03970701519320841 ) ) ;
#61813=CARTESIAN_POINT ( 'NONE',  ( 36.60665582185911404, 20.94473085651394584, 1.475505719884397138E-15 ) ) ;
#61814=CARTESIAN_POINT ( 'NONE',  ( 77.91581387522141711, 57.42368465423609791, 16.60724471479637998 ) ) ;
#61816=CARTESIAN_POINT ( 'NONE',  ( 82.61787247804464585, 43.35655690195848422, 8.757983355685475146 ) ) ;
#61821=CARTESIAN_POINT ( 'NONE',  ( 82.35975313173908319, 41.41624149291902057, 5.521678208619409389 ) ) ;
#61827=CARTESIAN_POINT ( 'NONE',  ( 27.76637506322961002, 39.52903772873361277, -1.583844403245329602 ) ) ;
#61829=B_SPLINE_CURVE_WITH_KNOTS ( 'NONE', 3,
 ( #42184, #98902, #59872, #60357, #99398, #6685, #52277, #75595, #5683, #58379, #20913, #51275, #89355, #45173, #68470, #51800, #90337, #97414, #52762, #37561, #27982, #29484, #76111, #5194, #13782, #74109, #44169, #36572, #83724, #89830, #19908 ),
 .UNSPECIFIED., .F., .F.,
 ( 4, 3, 3, 3, 3, 3, 3, 3, 3, 3, 4 ),
 ( 0.000000000000000000, 0.1333490885032447282, 0.3007194338854389248, 0.4699862290245251373, 0.5844252810809574816, 0.6686540514502947730, 0.7354980260655736846, 0.8028463152565851191, 0.8633854507757401375, 0.9437142632667373521, 1.000000000000000000 ),
 .UNSPECIFIED. ) ;
#61833=FACE_OUTER_BOUND ( 'NONE', #76984, .T. ) ;
#61835=B_SPLINE_CURVE_WITH_KNOTS ( 'NONE', 3,
 ( #84150, #36495, #68390, #22798, #75514, #36995, #14696, #13706, #30393, #98824, #76029, #67398, #6099, #35993, #51720, #5113, #29405, #28915, #98323, #76507, #37479, #91731, #99808, #91231, #92248, #52682, #22295, #53677, #7088, #83644, #61285 ),
 .UNSPECIFIED., .F., .F.,
 ( 4, 3, 3, 3, 3, 3, 3, 3, 3, 3, 4 ),
 ( 0.000000000000000000, 0.1333490885032314888, 0.3007194338854323190, 0.4699862290245113150, 0.5844252810809227316, 0.6686540514502676835, 0.7354980260655422653, 0.8028463152565505911, 0.8633854507757149355, 0.9437142632667404607, 1.000000000000000000 ),
 .UNSPECIFIED. ) ;
#61837=CARTESIAN_POINT ( 'NONE',  ( 15.27916758686040488, 29.79752408145592568, -5.678558825948271327 ) ) ;
#61839=CARTESIAN_POINT ( 'NONE',  ( 71.55582279638187515, 59.08747183676958770, 15.32285513291258283 ) ) ;
#61843=FACE_OUTER_BOUND ( 'NONE', #969, .T. ) ;
#61845=CARTESIAN_POINT ( 'NONE',  ( 81.80089866349948124, 42.11013410072107632, 7.569077868460975189 ) ) ;
#61848=CARTESIAN_POINT ( 'NONE',  ( 72.57160893180984829, 71.52012305816319326, -5.479963803933916466 ) ) ;
#61852=ORIENTED_EDGE ( 'NONE', *, *, #22167, .F. ) ;
#61854=CARTESIAN_POINT ( 'NONE',  ( 85.96141273360541391, 43.06913367483099364, -2.383719173196181540 ) ) ;
#61855=EDGE_LOOP ( 'NONE', ( #46759, #88374, #3713, #20025 ) ) ;
#61857=CARTESIAN_POINT ( 'NONE',  ( 31.41726478770819853, 19.10801979619930435, 3.090169943749476733 ) ) ;
#61858=FACE_OUTER_BOUND ( 'NONE', #98759, .T. ) ;
#61862=EDGE_LOOP ( 'NONE', ( #50423, #73000, #76241, #51833 ) ) ;
#61863=CARTESIAN_POINT ( 'NONE',  ( 81.77599116216271113, 59.08414711118528118, -0.4951340343707851255 ) ) ;
#61865=ORIENTED_EDGE ( 'NONE', *, *, #86171, .T. ) ;
#61866=CARTESIAN_POINT ( 'NONE',  ( 24.28583178621855865, 34.99752408145591431, 5.678558825948277544 ) ) ;
#61868=CARTESIAN_POINT ( 'NONE',  ( 78.14698338385944965, 47.61700244333332677, -13.90103454460489019 ) ) ;
#61873=CARTESIAN_POINT ( 'NONE',  ( 39.22461576370143632, 27.81029122506297568, 8.090169943749479842 ) ) ;
#61878=CARTESIAN_POINT ( 'NONE',  ( 82.31027433114240921, 53.67166805628564674, 15.82896004337745133 ) ) ;
#61885=EDGE_CURVE ( 'NONE', #47421, #90587, #52011, .T. ) ;
#61887=CARTESIAN_POINT ( 'NONE',  ( 69.47271657258438893, 66.54530737956719122, 10.18805627866735009 ) ) ;
#61890=CARTESIAN_POINT ( 'NONE',  ( 75.70701541337017204, 65.59976764996046938, 13.80433314997810967 ) ) ;
#61891=CARTESIAN_POINT ( 'NONE',  ( 70.72212250024647062, 65.42481974022895486, -11.87866371874642724 ) ) ;
#61892=CARTESIAN_POINT ( 'NONE',  ( 78.11787979767646561, 47.76729556080021410, 13.98403596371365687 ) ) ;
#61896=CARTESIAN_POINT ( 'NONE',  ( 84.25586279892151254, 41.93059359979653777, -0.3096221969905373905 ) ) ;
#61905=CARTESIAN_POINT ( 'NONE',  ( 72.50757856258960032, 71.58588072324644713, 5.252804842291221021 ) ) ;
#61915=CARTESIAN_POINT ( 'NONE',  ( 85.73738684536749588, 48.47886545727438801, -11.76341085017970656 ) ) ;
#61917=CARTESIAN_POINT ( 'NONE',  ( 71.54181076156694985, 65.04745795580406309, 12.54713244084793722 ) ) ;
#61919=FACE_OUTER_BOUND ( 'NONE', #9710, .T. ) ;
#61921=CARTESIAN_POINT ( 'NONE',  ( 81.93905738806562056, 41.80096582289180418, -5.620942555805415353 ) ) ;
#61925=CARTESIAN_POINT ( 'NONE',  ( 15.13540196134234606, 32.23654200823202132, 1.583844403245363353 ) ) ;
#61930=CARTESIAN_POINT ( 'NONE',  ( 8.751641773298651117, 23.79103043416547081, 8.090169943749478065 ) ) ;
#61933=CARTESIAN_POINT ( 'NONE',  ( 73.03023235113748513, 69.68176590430279305, 9.698330045464274463 ) ) ;
#61937=CARTESIAN_POINT ( 'NONE',  ( 73.12850034369863295, 57.37224303518116386, 15.89072477728744381 ) ) ;
#61939=CARTESIAN_POINT ( 'NONE',  ( 8.162811221194553823, 28.21091486745858745, -1.111400068045478839E-16 ) ) ;
#61945=CARTESIAN_POINT ( 'NONE',  ( 29.46033357383057449, 37.98502408145594700, -5.678558825948271327 ) ) ;
#61950=CARTESIAN_POINT ( 'NONE',  ( 88.47364309043327069, 44.01569472767099711, 2.145854971186520466 ) ) ;
#61951=CARTESIAN_POINT ( 'NONE',  ( 66.12980561864134188, 68.57555640412795128, 2.249234565191243540 ) ) ;
#61957=CARTESIAN_POINT ( 'NONE',  ( 17.90548643172614263, 12.19860640527291373, 2.839279412974134775 ) ) ;
#61970=CARTESIAN_POINT ( 'NONE',  ( 71.38434165879655779, 70.64309506879222056, 6.834342629426365612 ) ) ;
#61971=CARTESIAN_POINT ( 'NONE',  ( 85.74237854190519670, 45.04157437062109182, -7.829273241313135401 ) ) ;
#61974=CARTESIAN_POINT ( 'NONE',  ( 79.50784967658378832, 59.51503684596524124, -16.19812362877713596 ) ) ;
#61977=CARTESIAN_POINT ( 'NONE',  ( 69.87354030794955406, 62.76892477261478120, 13.90980553379283968 ) ) ;
#61978=ORIENTED_EDGE ( 'NONE', *, *, #68316, .T. ) ;
#61982=B_SPLINE_SURFACE_WITH_KNOTS ( 'NONE', 3, 1, ( 
 ( #60980, #91945 ),
 ( #22496, #17389 ),
 ( #55862, #56386 ),
 ( #80239, #26506 ),
 ( #48809, #48301 ),
 ( #64499, #47773 ),
 ( #73118, #2213 ),
 ( #33603, #88358 ),
 ( #95459, #71617 ),
 ( #96437, #32595 ),
 ( #2716, #26011 ),
 ( #34110, #24984 ),
 ( #18917, #72624 ),
 ( #63493, #63990 ),
 ( #57384, #56882 ),
 ( #79742, #86354 ),
 ( #3225, #49302 ),
 ( #49790, #87865 ),
 ( #33094, #79246 ),
 ( #94431, #9818 ),
 ( #18411, #40679 ),
 ( #86857, #78711 ),
 ( #65002, #10304 ),
 ( #94932, #27001 ),
 ( #95945, #80753 ),
 ( #10806, #72112 ),
 ( #11324, #87382 ),
 ( #42182, #40173 ),
 ( #1713, #25493 ),
 ( #41679, #17911 ),
 ( #41176, #3709 ) ),
 .UNSPECIFIED., .F., .F., .F.,
 ( 4, 3, 3, 3, 3, 3, 3, 3, 3, 3, 4 ),
 ( 2, 2 ),
 ( 0.000000000000000000, 0.1333490885032306283, 0.3007194338854234927, 0.4699862290244963270, 0.5844252810809187348, 0.6686540514502645749, 0.7354980260655307189, 0.8028463152565288308, 0.8633854507756889562, 0.9437142632666959408, 1.000000000000000000 ),
 ( 0.000000000000000000, 1.000000000000000000 ),
 .UNSPECIFIED. ) ;
#61984=ORIENTED_EDGE ( 'NONE', *, *, #77782, .F. ) ;
#61988=CARTESIAN_POINT ( 'NONE',  ( 70.71203917888955459, 71.32383586654306384, 2.333515263935871609 ) ) ;
#61992=CARTESIAN_POINT ( 'NONE',  ( 81.93576472774982733, 45.45616636752174600, 10.86207910360908180 ) ) ;
#61996=CARTESIAN_POINT ( 'NONE',  ( 69.46089132522230614, 68.43734353126103542, -7.767842414235587079 ) ) ;
#62000=CARTESIAN_POINT ( 'NONE',  ( 19.20273687360401027, 16.80170272979925628, 7.433330006724137462 ) ) ;
#62010=CARTESIAN_POINT ( 'NONE',  ( 83.58300336379315354, 45.77414047968564148, -10.26591261625669738 ) ) ;
#62016=CARTESIAN_POINT ( 'NONE',  ( 75.07571136114333399, 67.05229642490533593, -13.12030194816077611 ) ) ;
#62024=CARTESIAN_POINT ( 'NONE',  ( 11.39698775767667982, 6.984156793818257825, 1.224646799147354243E-15 ) ) ;
#62026=CARTESIAN_POINT ( 'NONE',  ( 75.91719666336339856, 65.48793379249461566, 14.32281418338181211 ) ) ;
#62032=CARTESIAN_POINT ( 'NONE',  ( 67.13635405088328412, 67.13670889057797808, -8.571836668080649702 ) ) ;
#62035=FACE_OUTER_BOUND ( 'NONE', #49741, .T. ) ;
#62043=CARTESIAN_POINT ( 'NONE',  ( 66.47763888060634940, 67.99612994687967671, 6.463816603905427449 ) ) ;
#62044=CARTESIAN_POINT ( 'NONE',  ( 80.61729146147543190, 57.24021084763496248, -16.23099362249694266 ) ) ;
#62047=CARTESIAN_POINT ( 'NONE',  ( 83.32573152649015924, 51.37405908170996582, 14.80978086562886631 ) ) ;
#62054=CARTESIAN_POINT ( 'NONE',  ( 68.60781884079298720, 68.28949036833112984, 7.135800403798556957 ) ) ;
#62063=CARTESIAN_POINT ( 'NONE',  ( 16.17343562415726765, 11.19860640527290840, 2.839279412974134775 ) ) ;
#62066=CARTESIAN_POINT ( 'NONE',  ( 75.97421294056728414, 58.33098411539324957, -16.47611980641094931 ) ) ;
#62074=CARTESIAN_POINT ( 'NONE',  ( 86.20356499834056763, 47.68669917282567638, 10.81083910437671669 ) ) ;
#62077=CARTESIAN_POINT ( 'NONE',  ( 34.67812306484450602, 22.94754757982092030, 5.678558825948272215 ) ) ;
#62078=LINE ( 'NONE', #92539, #81482 ) ;
#62083=ORIENTED_EDGE ( 'NONE', *, *, #94051, .T. ) ;
#62085=CARTESIAN_POINT ( 'NONE',  ( 79.16403909620731838, 50.00558055149382852, 14.72677174306799230 ) ) ;
#62087=LINE ( 'NONE', #93032, #64660 ) ;
#62090=CARTESIAN_POINT ( 'NONE',  ( 73.49483902118549850, 69.87589544865461733, 9.786909576851130055 ) ) ;
#62091=CARTESIAN_POINT ( 'NONE',  ( 39.38594668318775405, 31.24335787977766188, -9.188101187500008038 ) ) ;
#62096=CARTESIAN_POINT ( 'NONE',  ( 86.13921288864840164, 46.97634557790220811, -10.11631737044880808 ) ) ;
#62099=CARTESIAN_POINT ( 'NONE',  ( 82.26287869091245852, 44.55745556623967474, -10.46805190375325445 ) ) ;
#62100=CARTESIAN_POINT ( 'NONE',  ( 45.09207854535236493, 28.96004757982094446, -5.678558825948275768 ) ) ;
#62101=CARTESIAN_POINT ( 'NONE',  ( 80.31877406852532886, 44.32323502835605211, 11.34894536411993471 ) ) ;
#62102=CARTESIAN_POINT ( 'NONE',  ( 84.87268683136555580, 50.02192652042950982, -13.22765022071786944 ) ) ;
#62103=CARTESIAN_POINT ( 'NONE',  ( 81.22979812886450190, 55.45288652294036069, -16.34461090620092349 ) ) ;
#62106=ORIENTED_EDGE ( 'NONE', *, *, #49617, .F. ) ;
#62107=CARTESIAN_POINT ( 'NONE',  ( 77.26467096630975107, 49.18305258566515903, -14.81582409400270350 ) ) ;
#62108=AXIS2_PLACEMENT_3D ( 'NONE', #66366, #97298, #60234 ) ;
#62110=CARTESIAN_POINT ( 'NONE',  ( 87.04951863019347513, 45.82536234993809643, -8.629913247614998895 ) ) ;
#62111=ORIENTED_EDGE ( 'NONE', *, *, #31753, .T. ) ;
#62121=CARTESIAN_POINT ( 'NONE',  ( 70.57165604962446537, 60.75797888666558322, -14.54259087274441953 ) ) ;
#62122=CARTESIAN_POINT ( 'NONE',  ( 33.95706010830453181, 41.64646525600393545, -2.839279412974133887 ) ) ;
#62128=APPLICATION_CONTEXT ( 'automotive_design' ) ;
#62132=CARTESIAN_POINT ( 'NONE',  ( 72.72789744706139459, 64.44696951616786862, 13.39283383340056588 ) ) ;
#62153=CARTESIAN_POINT ( 'NONE',  ( 73.09495692854210347, 67.84340929558865696, 11.06288556080568597 ) ) ;
#62161=CARTESIAN_POINT ( 'NONE',  ( 22.93021583062070690, 14.20801979619928623, -3.090169943749474069 ) ) ;
#62164=CARTESIAN_POINT ( 'NONE',  ( 70.02394384298496277, 66.60507294567733538, -11.13771036556853744 ) ) ;
#62171=CARTESIAN_POINT ( 'NONE',  ( 84.88661097013314816, 50.13767530291475794, -13.29087463649034007 ) ) ;
#62172=CARTESIAN_POINT ( 'NONE',  ( 80.44215978124604760, 58.39441083166273216, 0.000000000000000000 ) ) ;
#62173=CARTESIAN_POINT ( 'NONE',  ( 73.40082382908687464, 69.73317320774677341, -9.891058063621702701 ) ) ;
#62174=CARTESIAN_POINT ( 'NONE',  ( 76.13141603458973350, 51.16231187342496867, 16.09112476300021655 ) ) ;
#62186=CARTESIAN_POINT ( 'NONE',  ( 88.52345208173723279, 43.89072024811925843, -0.4439432684152972430 ) ) ;
#62190=CARTESIAN_POINT ( 'NONE',  ( 67.39295136396972907, 69.98592323009434324, -1.247867760768429646 ) ) ;
#62192=CARTESIAN_POINT ( 'NONE',  ( 26.50621139815082472, 30.70171378149920471, -9.188101187500004485 ) ) ;
#62194=CARTESIAN_POINT ( 'NONE',  ( 82.80780985081015899, 47.11681503041204877, -11.90565482037006539 ) ) ;
#62195=CARTESIAN_POINT ( 'NONE',  ( 16.34664070491415444, 11.29860640527290983, -2.839279412974138328 ) ) ;
#62197=CARTESIAN_POINT ( 'NONE',  ( 77.21750963125948886, 63.47318699979658163, 15.10190582221587263 ) ) ;
#62198=LINE ( 'NONE', #15600, #41365 ) ;
#62199=EDGE_CURVE ( 'NONE', #81391, #35343, #12004, .T. ) ;
#62204=CARTESIAN_POINT ( 'NONE',  ( 82.56047309644807797, 54.07683023134062239, -15.52634518316282630 ) ) ;
#62210=CARTESIAN_POINT ( 'NONE',  ( 82.35193903712398367, 53.76144841737797719, 15.84691369965403318 ) ) ;
#62215=ORIENTED_EDGE ( 'NONE', *, *, #73533, .T. ) ;
#62218=CARTESIAN_POINT ( 'NONE',  ( 66.29454943693275482, 69.24199052626691753, -2.144636311159408226 ) ) ;
#62220=CARTESIAN_POINT ( 'NONE',  ( 82.16322555321710297, 45.01969389507814157, 10.99933557872955525 ) ) ;
#62222=CARTESIAN_POINT ( 'NONE',  ( 28.38260615371904905, 22.10170272979928185, -7.433330006724141015 ) ) ;
#62223=CARTESIAN_POINT ( 'NONE',  ( 79.75048646024721677, 44.95318393210929742, 11.52289528432964438 ) ) ;
#62225=CARTESIAN_POINT ( 'NONE',  ( 75.31212634066369560, 66.58130303916082937, -13.09031499722823710 ) ) ;
#62231=CARTESIAN_POINT ( 'NONE',  ( 67.77717145076422867, 65.67792780390388430, 10.77137413574873825 ) ) ;
#62232=CARTESIAN_POINT ( 'NONE',  ( 67.99201013372248781, 65.53178319986331246, -10.30868045286246115 ) ) ;
#62243=CARTESIAN_POINT ( 'NONE',  ( 74.58922631747108767, 66.95469429158355013, 12.55546573254311937 ) ) ;
#62244=CARTESIAN_POINT ( 'NONE',  ( 78.18406947592188772, 61.66846224198985027, -16.12704840749690050 ) ) ;
#62247=ORIENTED_EDGE ( 'NONE', *, *, #75734, .T. ) ;
#62249=CARTESIAN_POINT ( 'NONE',  ( 80.05820879288631886, 44.42019321735476467, -10.88558367697336848 ) ) ;
#62253=CARTESIAN_POINT ( 'NONE',  ( 79.81928979513558886, 48.51125504466014604, -13.89558333913432087 ) ) ;
#62260=CARTESIAN_POINT ( 'NONE',  ( 24.06687416953986514, 14.86426979415089633, -3.090169943749474069 ) ) ;
#62263=CARTESIAN_POINT ( 'NONE',  ( 76.16798847255994076, 65.32953285235316798, -14.06901634343885021 ) ) ;
#62268=CARTESIAN_POINT ( 'NONE',  ( 83.81371460731152467, 43.68598234505141420, -7.289791965750151981 ) ) ;
#62269=CARTESIAN_POINT ( 'NONE',  ( 32.45591003703110999, 42.23654200823204974, 1.583844403245397769 ) ) ;
#62273=B_SPLINE_CURVE_WITH_KNOTS ( 'NONE', 3,
 ( #44853, #28668, #68161, #37750, #51978, #60051, #13003, #59552, #21578, #90529, #43863, #7355, #75793, #44362, #52463, #45837, #5382, #6379, #76289, #82917, #6861, #99087, #29669, #13492, #60546, #91503, #75295, #52963, #14476, #24058, #84898, #86929, #69154, #93498, #7873, #15439, #61551, #23042, #46338, #78778, #23540, #8858, #1779, #92497, #30671, #69653 ),
 .UNSPECIFIED., .F., .F.,
 ( 4, 1, 2, 2, 1, 2, 2, 1, 1, 2, 2, 1, 1, 2, 2, 1, 1, 2, 2, 1, 1, 1, 2, 2, 1, 1, 1, 2, 2, 4 ),
 ( 0.000000000000000000, 0.06249999999999282518, 0.09374999999998952227, 0.1249999999999862332, 0.1874999999999796274, 0.2187499999999759637, 0.2499999999999722999, 0.3124999999999658051, 0.3437499999999626965, 0.3593749999999617528, 0.3749999999999607536, 0.4374999999999629741, 0.4687499999999648614, 0.4843749999999655831, 0.4999999999999663602, 0.5624999999999700240, 0.5937499999999719114, 0.6093749999999720224, 0.6249999999999721334, 0.6874999999999705791, 0.7187499999999698019, 0.7343749999999689138, 0.7421874999999691358, 0.7499999999999692468, 0.8124999999999721334, 0.8437499999999744649, 0.8593749999999756861, 0.8671874999999771294, 0.8749999999999785727, 1.000000000000000000 ),
 .UNSPECIFIED. ) ;
#62274=CARTESIAN_POINT ( 'NONE',  ( 72.49654942766741783, 70.83148394934322312, 7.643478247317299967 ) ) ;
#62276=CARTESIAN_POINT ( 'NONE',  ( 70.75328031780846061, 67.31962847426909491, -10.19312708527341371 ) ) ;
#62281=CARTESIAN_POINT ( 'NONE',  ( 12.22230530498202050, 30.55466486950698624, -1.111400068045478839E-16 ) ) ;
#62283=CARTESIAN_POINT ( 'NONE',  ( 83.70690788325238429, 51.99575818335755173, 14.97781791391902928 ) ) ;
#62285=ORIENTED_EDGE ( 'NONE', *, *, #87657, .F. ) ;
#62287=CARTESIAN_POINT ( 'NONE',  ( 84.14312167556933275, 48.98415679381830756, 0.000000000000000000 ) ) ;
#62291=CARTESIAN_POINT ( 'NONE',  ( 73.63433810907314125, 55.41313869502708656, 16.11241297416459872 ) ) ;
#62293=CARTESIAN_POINT ( 'NONE',  ( 35.05457148360284236, 21.20801979619930933, -3.090169943749474069 ) ) ;
#62304=CARTESIAN_POINT ( 'NONE',  ( 35.21268636174862365, 20.73415679381824006, 1.333680081654574804E-15 ) ) ;
#62308=CARTESIAN_POINT ( 'NONE',  ( 27.80420065655628648, 34.79103043416550634, 8.090169943749478065 ) ) ;
#62309=CARTESIAN_POINT ( 'NONE',  ( 85.03485922901262484, 42.43661927826852320, -1.488589828080878252 ) ) ;
#62311=CARTESIAN_POINT ( 'NONE',  ( 81.60179630412660856, 55.93049734755844327, 16.03035934503441240 ) ) ;
#62312=EDGE_CURVE ( 'NONE', #26530, #13530, #97772, .T. ) ;
#62313=CARTESIAN_POINT ( 'NONE',  ( 84.74131058565687624, 48.42447779055156332, 12.64580013056608898 ) ) ;
#62318=DIRECTION ( 'NONE',  ( 0.000000000000000000, 0.7457702847286216130, -0.6662031840330625565 ) ) ;
#62321=CARTESIAN_POINT ( 'NONE',  ( 67.43464856002299257, 69.65467215062919593, -3.403559293901139871 ) ) ;
#62323=CARTESIAN_POINT ( 'NONE',  ( 29.61202869050421427, 35.83478043621390441, -8.090169943749479842 ) ) ;
#62331=B_SPLINE_CURVE_WITH_KNOTS ( 'NONE', 3,
 ( #77560, #30442, #56, #46119, #53725, #54217, #8645, #84684, #15224, #54725 ),
 .UNSPECIFIED., .F., .F.,
 ( 4, 2, 2, 2, 4 ),
 ( 0.000000000000000000, 0.0002622400424272925377, 0.0005244800848545850755, 0.0007867201272818776132, 0.001048960169709170151 ),
 .UNSPECIFIED. ) ;
#62333=CARTESIAN_POINT ( 'NONE',  ( 23.32475077058400004, 14.26216523072494446, -2.296566073217252530E-15 ) ) ;
#62335=CARTESIAN_POINT ( 'NONE',  ( 71.66445348058819320, 59.04578686578420132, 15.85137124283286170 ) ) ;
#62338=CARTESIAN_POINT ( 'NONE',  ( 8.149503075528279794, 26.74646525600388358, 2.839279412974139660 ) ) ;
#62339=CARTESIAN_POINT ( 'NONE',  ( 78.42229082697367915, 57.96928826923493716, -16.21819880184166252 ) ) ;
#62340=CARTESIAN_POINT ( 'NONE',  ( 88.19071408691713998, 44.34108068381398482, 2.666398900887132939 ) ) ;
#62343=CARTESIAN_POINT ( 'NONE',  ( 70.02460195589141279, 70.89239522396498216, -2.258892735534246743 ) ) ;
#62346=ADVANCED_FACE ( 'NONE', ( #71570 ), #74886, .T. ) ;
#62353=CARTESIAN_POINT ( 'NONE',  ( 72.70498915057306988, 57.04919252086779835, -16.38563882821832607 ) ) ;
#62354=DIRECTION ( 'NONE',  ( -0.8660254037844378194, -0.5000000000000014433, -0.000000000000000000 ) ) ;
#62355=EDGE_CURVE ( 'NONE', #48577, #13530, #74571, .T. ) ;
#62362=CARTESIAN_POINT ( 'NONE',  ( 35.07444006175263240, 22.11110640527294535, -2.839279412974138328 ) ) ;
#62364=CARTESIAN_POINT ( 'NONE',  ( 78.24241764518251330, 47.43171081316724980, -14.32955934271819665 ) ) ;
#62365=VERTEX_POINT ( 'NONE', #44121 ) ;
#62367=CARTESIAN_POINT ( 'NONE',  ( 24.34666095796415419, 37.55466486950700755, 7.012934429366973338E-14 ) ) ;
#62370=CARTESIAN_POINT ( 'NONE',  ( 34.40128339993918871, 35.56454794089043503, 10.00000000000000355 ) ) ;
#62374=CARTESIAN_POINT ( 'NONE',  ( 82.59969462453734934, 42.72094940597061452, -6.768182983292747146 ) ) ;
#62379=CARTESIAN_POINT ( 'NONE',  ( 90.04477061917849312, 44.76220097505219542, 0.000000000000000000 ) ) ;
#62383=CARTESIAN_POINT ( 'NONE',  ( 68.85038956537171373, 65.11612515096180687, 11.21264051096888004 ) ) ;
#62386=CARTESIAN_POINT ( 'NONE',  ( 71.82406175789866154, 65.23099472832208789, -12.52007583028708559 ) ) ;
#62387=CARTESIAN_POINT ( 'NONE',  ( 78.73346053687757262, 47.61223242048821191, 14.27696141479210468 ) ) ;
#62391=CARTESIAN_POINT ( 'NONE',  ( 83.45882455891384666, 41.54361669290386772, -1.301328012872986717 ) ) ;
#62392=CARTESIAN_POINT ( 'NONE',  ( 87.35668359673078953, 44.84080960044052944, -6.701380392922970053 ) ) ;
#62398=CARTESIAN_POINT ( 'NONE',  ( 83.89856196509347797, 51.66380357613086005, -14.40442690555789618 ) ) ;
#62400=EDGE_LOOP ( 'NONE', ( #56150, #81378, #30350, #27665 ) ) ;
#62402=CARTESIAN_POINT ( 'NONE',  ( 72.59841233342120859, 71.52691570274980393, 5.510137056446514414 ) ) ;
#62410=CARTESIAN_POINT ( 'NONE',  ( 85.74775437209392237, 48.65322352004045570, -12.36257617231559891 ) ) ;
#62412=CARTESIAN_POINT ( 'NONE',  ( 87.74907107289484998, 44.16117455547062320, -4.521424286948808380 ) ) ;
#62416=CARTESIAN_POINT ( 'NONE',  ( 82.22868350776323609, 41.49786495964391264, -5.893870365715465631 ) ) ;
#62421=PLANE ( 'NONE',  #62868 ) ;
#62427=CARTESIAN_POINT ( 'NONE',  ( 17.13867093926436169, 10.86426979415088567, -3.090169943749474069 ) ) ;
#62429=CARTESIAN_POINT ( 'NONE',  ( 73.95758533133535195, 54.98678301060776619, -16.60461700056748313 ) ) ;
#62430=FACE_OUTER_BOUND ( 'NONE', #12151, .T. ) ;
#62433=CARTESIAN_POINT ( 'NONE',  ( 73.16563970766678437, 57.31928544487961830, 16.38500887864065803 ) ) ;
#62434=CARTESIAN_POINT ( 'NONE',  ( 72.46511837996447980, 71.56249752072032777, 6.234640293157904800 ) ) ;
#62435=CARTESIAN_POINT ( 'NONE',  ( 66.67307728759789143, 68.37645106841958409, -4.361463599803915514 ) ) ;
#62441=CARTESIAN_POINT ( 'NONE',  ( 29.64435718874111458, 29.06628583063843152, -9.188101187500006262 ) ) ;
#62446=CARTESIAN_POINT ( 'NONE',  ( 66.24548473545846150, 68.62659743099872856, 2.338129593227180614 ) ) ;
#62450=EDGE_CURVE ( 'NONE', #46528, #66065, #28857, .T. ) ;
#62452=CARTESIAN_POINT ( 'NONE',  ( 66.97748580466556234, 68.05911003901715617, 6.908000617270676713 ) ) ;
#62453=CARTESIAN_POINT ( 'NONE',  ( 13.11890841201833169, 13.28920272979925166, -7.433330006724141015 ) ) ;
#62464=ORIENTED_EDGE ( 'NONE', *, *, #67698, .T. ) ;
#62465=VERTEX_POINT ( 'NONE', #39502 ) ;
#62468=ORIENTED_EDGE ( 'NONE', *, *, #58622, .F. ) ;
#62469=CARTESIAN_POINT ( 'NONE',  ( 26.55243232390424879, 15.73415679381822585, 1.333680081654574804E-15 ) ) ;
#62477=CARTESIAN_POINT ( 'NONE',  ( 69.42765538681520354, 62.69932690130006137, 13.22847919835291997 ) ) ;
#62478=ORIENTED_EDGE ( 'NONE', *, *, #1243, .F. ) ;
#62482=DIRECTION ( 'NONE',  ( -0.8660254037844378194, -0.5000000000000014433, -0.000000000000000000 ) ) ;
#62483=ORIENTED_EDGE ( 'NONE', *, *, #66634, .T. ) ;
#62486=CARTESIAN_POINT ( 'NONE',  ( 72.49386282319785835, 57.57572440859879492, 15.80166580940835885 ) ) ;
#62487=VERTEX_POINT ( 'NONE', #7124 ) ;
#62491=CARTESIAN_POINT ( 'NONE',  ( 83.77234465117980733, 51.52744445023363795, 14.35368014269928771 ) ) ;
#62494=CARTESIAN_POINT ( 'NONE',  ( 82.39556149134112673, 53.49063599510539291, -15.76428462505608330 ) ) ;
#62496=CARTESIAN_POINT ( 'NONE',  ( 78.91703011957858394, 55.68952724942787569, -16.53731823143577628 ) ) ;
#62497=CARTESIAN_POINT ( 'NONE',  ( 18.92729281690869314, 22.87878583063841020, -9.188101187500006262 ) ) ;
#62500=B_SPLINE_CURVE_WITH_KNOTS ( 'NONE', 3,
 ( #60821, #68934, #99860, #69441, #62834, #46121, #1564, #56233, #31931, #86204 ),
 .UNSPECIFIED., .F., .F.,
 ( 4, 2, 2, 2, 4 ),
 ( 0.000000000000000000, 0.2500000000000000000, 0.5000000000000000000, 0.7500000000000000000, 1.000000000000000000 ),
 .UNSPECIFIED. ) ;
#62501=CARTESIAN_POINT ( 'NONE',  ( 80.71776722511965829, 57.44908488972237848, 16.57971273854667515 ) ) ;
#62509=EDGE_CURVE ( 'NONE', #34846, #24668, #65099, .T. ) ;
#62511=CARTESIAN_POINT ( 'NONE',  ( 82.74931449563905517, 45.88034904727371099, -10.83867196349580375 ) ) ;
#62514=CARTESIAN_POINT ( 'NONE',  ( 71.81026643095458439, 59.04125517816913771, 15.87515779228373525 ) ) ;
#62517=CARTESIAN_POINT ( 'NONE',  ( 74.96814850772597083, 66.86370092720996183, -13.20453066047568846 ) ) ;
#62522=CARTESIAN_POINT ( 'NONE',  ( 82.35750029267607886, 40.37841760621454057, -1.251208198262858229 ) ) ;
#62523=B_SPLINE_CURVE_WITH_KNOTS ( 'NONE', 3,
 ( #718, #30125, #61518, #53905, #31606, #61008, #8329, #1230, #15405, #62496, #70109, #46299, #91980, #24018, #77746, #22530 ),
 .UNSPECIFIED., .F., .F.,
 ( 4, 1, 2, 2, 2, 1, 2, 2, 4 ),
 ( 0.000000000000000000, 0.1250000000000004996, 0.1874999999999985290, 0.2499999999999965583, 0.4999999999999943379, 0.6249999999999932276, 0.6874999999999927836, 0.7499999999999922284, 1.000000000000000000 ),
 .UNSPECIFIED. ) ;
#62526=CARTESIAN_POINT ( 'NONE',  ( 72.94747830045673709, 70.90780099059745112, 7.943658523256111437 ) ) ;
#62528=CARTESIAN_POINT ( 'NONE',  ( 75.51640727855378543, 65.37558461351387962, 13.86249185021059738 ) ) ;
#62536=CARTESIAN_POINT ( 'NONE',  ( 82.03968029452317978, 46.65024194024377380, -11.88741162480429381 ) ) ;
#62540=CARTESIAN_POINT ( 'NONE',  ( 74.13858531873714242, 68.40778981217252408, -11.66187469989377767 ) ) ;
#62543=ORIENTED_EDGE ( 'NONE', *, *, #60560, .F. ) ;
#62562=CARTESIAN_POINT ( 'NONE',  ( 10.75418485208671981, 27.18502408145590010, 5.678558825948277544 ) ) ;
#62574=CARTESIAN_POINT ( 'NONE',  ( 86.06077315872715872, 47.66653318574839204, 10.87392282977397784 ) ) ;
#62582=B_SPLINE_SURFACE_WITH_KNOTS ( 'NONE', 3, 1, ( 
 ( #13230, #51723 ),
 ( #90763, #44085 ),
 ( #29409, #92253 ),
 ( #52192, #60278 ),
 ( #84636, #14207 ),
 ( #37483, #68394 ),
 ( #60772, #21313 ),
 ( #45584, #76033 ),
 ( #6610, #13 ),
 ( #53199, #98326 ),
 ( #83648, #99814 ),
 ( #99319, #82666 ),
 ( #29899, #91736 ),
 ( #68887, #75027 ),
 ( #5607, #28919 ),
 ( #22299, #76511 ),
 ( #7094, #30397 ),
 ( #15176, #76989 ),
 ( #7596, #38483 ),
 ( #69397, #30897 ),
 ( #92731, #54171 ),
 ( #70392, #17706 ),
 ( #85140, #15687 ),
 ( #63294, #55669 ),
 ( #62274, #93229 ),
 ( #23283, #54674 ),
 ( #46580, #16696 ),
 ( #77517, #24303 ),
 ( #8108, #38983 ),
 ( #500, #69888 ),
 ( #87172, #1003 ) ),
 .UNSPECIFIED., .F., .F., .F.,
 ( 4, 3, 3, 3, 3, 3, 3, 3, 3, 3, 4 ),
 ( 2, 2 ),
 ( 0.000000000000000000, 0.1333490885032278528, 0.3007194338854267679, 0.4699862290245069296, 0.5844252810809245080, 0.6686540514502667953, 0.7354980260655522573, 0.8028463152565803451, 0.8633854507757331431, 0.9437142632667367970, 1.000000000000000000 ),
 ( 0.000000000000000000, 1.000000000000000000 ),
 .UNSPECIFIED. ) ;
#62583=CARTESIAN_POINT ( 'NONE',  ( 75.89038410296754478, 65.15355031958958421, -14.48133090960389069 ) ) ;
#62586=CARTESIAN_POINT ( 'NONE',  ( 72.39511741677974044, 71.78066914166659274, -5.650358525013035482 ) ) ;
#62590=VERTEX_POINT ( 'NONE', #27828 ) ;
#62591=CARTESIAN_POINT ( 'NONE',  ( 73.22997076551303053, 69.87431308930813145, 9.604659174840600500 ) ) ;
#62593=CARTESIAN_POINT ( 'NONE',  ( 33.72069078606260462, 37.65586893147758474, -7.433330006724137462 ) ) ;
#62598=CARTESIAN_POINT ( 'NONE',  ( 81.68695031315317578, 44.07415216466816332, -10.32458475606733650 ) ) ;
#62600=CARTESIAN_POINT ( 'NONE',  ( 86.48326989762649930, 47.07371192975631402, -10.55119608217691507 ) ) ;
#62603=CARTESIAN_POINT ( 'NONE',  ( 27.95316317257044858, 17.10801979619929725, 3.090169943749476733 ) ) ;
#62604=CARTESIAN_POINT ( 'NONE',  ( 42.85004829832549689, 33.24335787977766898, -9.188101187500008038 ) ) ;
#62611=CARTESIAN_POINT ( 'NONE',  ( 77.18140344432271149, 49.55420220550890065, -15.47549763322615668 ) ) ;
#62616=FACE_BOUND ( 'NONE', #99193, .T. ) ;
#62620=CARTESIAN_POINT ( 'NONE',  ( 82.39843561648048365, 40.93538189525752813, 1.011552965053796438 ) ) ;
#62626=CARTESIAN_POINT ( 'NONE',  ( 41.28156676870083430, 26.76004757982093452, 5.678558825948272215 ) ) ;
#62628=CARTESIAN_POINT ( 'NONE',  ( 27.43138059761190206, 24.03677371833803278, 10.00000000000000533 ) ) ;
#62633=CARTESIAN_POINT ( 'NONE',  ( 69.93330931759959412, 71.50341667604121199, 8.155205941333377477E-06 ) ) ;
#62636=CARTESIAN_POINT ( 'NONE',  ( 79.23761817010250752, 56.43779631686524567, 16.57197305649037844 ) ) ;
#62659=CARTESIAN_POINT ( 'NONE',  ( 72.63364946472314898, 61.52540385496723019, 15.23333689719127548 ) ) ;
#62664=CARTESIAN_POINT ( 'NONE',  ( 74.41008358870023187, 68.25813196090381041, 11.92500230979621634 ) ) ;
#62666=CARTESIAN_POINT ( 'NONE',  ( 74.19679258280018530, 68.60443047759615354, 11.01698511858023721 ) ) ;
#62667=CARTESIAN_POINT ( 'NONE',  ( 68.77417503162503465, 70.33503179494164215, 0.5183767665663540081 ) ) ;
#62675=CARTESIAN_POINT ( 'NONE',  ( 84.88336942958184750, 50.06956966849930524, -13.25211461007744695 ) ) ;
#62678=CARTESIAN_POINT ( 'NONE',  ( 73.36513840663161545, 69.69468182635826281, -9.911920066630193205 ) ) ;
#62679=CARTESIAN_POINT ( 'NONE',  ( 76.29262445978407925, 51.36595510716406920, 15.62292352366308634 ) ) ;
#62689=DIRECTION ( 'NONE',  ( 0.5778974349098237040, 0.4186690413702433000, -0.7005360722495078685 ) ) ;
#62690=CARTESIAN_POINT ( 'NONE',  ( 88.33576385398527009, 44.18506255568602370, -0.1374804814267040487 ) ) ;
#62691=CARTESIAN_POINT ( 'NONE',  ( 85.51062282364698319, 48.96702101389664108, -12.23238128493630583 ) ) ;
#62693=CARTESIAN_POINT ( 'NONE',  ( 71.64316818921393804, 72.05741665177616539, -3.509880912999890690 ) ) ;
#62696=CARTESIAN_POINT ( 'NONE',  ( 30.35763184873497877, 26.03085787977764198, 9.188101187500006262 ) ) ;
#62699=CARTESIAN_POINT ( 'NONE',  ( 8.146472837920740062, 20.10171378149916777, 9.188101187500008038 ) ) ;
#62701=CARTESIAN_POINT ( 'NONE',  ( 77.07103148522583069, 63.64506183647083759, 15.39324216548719626 ) ) ;
#62704=CARTESIAN_POINT ( 'NONE',  ( 69.81582973455007846, 63.14295414310246457, -13.67321376818635059 ) ) ;
#62711=CARTESIAN_POINT ( 'NONE',  ( 77.52094420404428377, 49.23844290216526787, 15.29553459438156793 ) ) ;
#62717=ADVANCED_FACE ( 'NONE', ( #23699 ), #67587, .T. ) ;
#62718=CARTESIAN_POINT ( 'NONE',  ( 67.67030795740730298, 68.61334932093440386, -5.327093496892230107 ) ) ;
#62722=CARTESIAN_POINT ( 'NONE',  ( 76.67567146729665239, 63.34086528488000312, -15.41964329106466103 ) ) ;
#62727=CARTESIAN_POINT ( 'NONE',  ( 29.70508255828911004, 19.01110640527293327, 2.839279412974134775 ) ) ;
#62731=ORIENTED_EDGE ( 'NONE', *, *, #76077, .F. ) ;
#62735=ORIENTED_EDGE ( 'NONE', *, *, #62509, .T. ) ;
#62738=CARTESIAN_POINT ( 'NONE',  ( 67.85199900019571828, 65.46856307543899334, 10.29293294925176738 ) ) ;
#62739=CARTESIAN_POINT ( 'NONE',  ( 67.81340710963647211, 65.98316596844472315, -10.47555129015767683 ) ) ;
#62740=CARTESIAN_POINT ( 'NONE',  ( 81.75198846930985042, 55.31526633232800094, -15.92433154267821394 ) ) ;
#62746=AXIS2_PLACEMENT_3D ( 'NONE', #2982, #34348, #55625 ) ;
#62749=ORIENTED_EDGE ( 'NONE', *, *, #62199, .T. ) ;
#62754=VERTEX_POINT ( 'NONE', #79961 ) ;
#62757=CARTESIAN_POINT ( 'NONE',  ( 80.25975942986622158, 44.70959520753981309, -11.72582774008359152 ) ) ;
#62761=CARTESIAN_POINT ( 'NONE',  ( 83.27207070336380923, 47.65589845134895342, -12.15996375230644233 ) ) ;
#62764=ORIENTED_EDGE ( 'NONE', *, *, #44773, .F. ) ;
#62765=EDGE_CURVE ( 'NONE', #52745, #9204, #2953, .T. ) ;
#62769=ORIENTED_EDGE ( 'NONE', *, *, #75270, .F. ) ;
#62770=CARTESIAN_POINT ( 'NONE',  ( 15.04662694159776670, 32.18528772668517490, -1.583844403245363575 ) ) ;
#62774=EDGE_CURVE ( 'NONE', #85165, #64642, #17626, .T. ) ;
#62777=CARTESIAN_POINT ( 'NONE',  ( 87.52536710082529225, 44.57545605528624577, 4.902363546664118665 ) ) ;
#62779=CARTESIAN_POINT ( 'NONE',  ( 82.01543408846627869, 43.66070079000877513, -8.773935687765517244 ) ) ;
#62780=ADVANCED_FACE ( 'NONE', ( #9539 ), #58950, .T. ) ;
#62781=CARTESIAN_POINT ( 'NONE',  ( 36.13333420750807079, 36.56454794089044924, 10.00000000000000355 ) ) ;
#62783=ADVANCED_FACE ( 'NONE', ( #70825 ), #71842, .T. ) ;
#62786=B_SPLINE_CURVE_WITH_KNOTS ( 'NONE', 3,
 ( #44304, #59997, #90966, #52407, #83353, #71125, #85877, #31094 ),
 .UNSPECIFIED., .F., .F.,
 ( 4, 2, 2, 4 ),
 ( 0.4503330015877973214, 0.7251665007938997709, 0.8625832503969499410, 1.000000000000000000 ),
 .UNSPECIFIED. ) ;
#62792=CARTESIAN_POINT ( 'NONE',  ( 85.10088869340128781, 43.69823583396123468, 5.977407741011665721 ) ) ;
#62795=CARTESIAN_POINT ( 'NONE',  ( 83.95452371275135306, 51.84303909528517806, 14.85259985614520062 ) ) ;
#62797=ORIENTED_EDGE ( 'NONE', *, *, #64311, .F. ) ;
#62803=FACE_BOUND ( 'NONE', #60985, .T. ) ;
#62805=CARTESIAN_POINT ( 'NONE',  ( 30.82863370761418054, 19.92755873383627119, 6.180339887498953466 ) ) ;
#62820=CARTESIAN_POINT ( 'NONE',  ( 35.76051414856368638, 25.81029122506296858, 8.090169943749479842 ) ) ;
#62821=CARTESIAN_POINT ( 'NONE',  ( 78.11027170948028697, 58.64888375189529768, 16.54994857808256015 ) ) ;
#62828=CARTESIAN_POINT ( 'NONE',  ( 68.90019008890776320, 66.82522398943339681, -9.471753670772901756 ) ) ;
#62832=CARTESIAN_POINT ( 'NONE',  ( 67.86617404580020718, 69.78291350440201768, -3.870024980962481820 ) ) ;
#62834=CARTESIAN_POINT ( 'NONE',  ( 77.11858699210218049, 49.43661330258253628, -14.93544102205281554 ) ) ;
#62839=CARTESIAN_POINT ( 'NONE',  ( 73.08094384907833785, 54.14441083166271795, 0.000000000000000000 ) ) ;
#62842=CARTESIAN_POINT ( 'NONE',  ( 16.91979795264450459, 27.95586893147755347, 7.433330006724141015 ) ) ;
#62847=CARTESIAN_POINT ( 'NONE',  ( 9.248262631489305718, 13.84335787977760823, 9.188101187500006262 ) ) ;
#62848=DIRECTION ( 'NONE',  ( -0.8660254037844378194, -0.5000000000000013323, -0.000000000000000000 ) ) ;
#62849=CARTESIAN_POINT ( 'NONE',  ( 79.25711091567707456, 57.60615597753891137, -16.24568049410854442 ) ) ;
#62850=CARTESIAN_POINT ( 'NONE',  ( 71.70445494439258027, 72.46184198916859032, -1.357087204883099751 ) ) ;
#62853=CARTESIAN_POINT ( 'NONE',  ( 72.27803260052462520, 71.63036165027699553, -5.844549976855538453 ) ) ;
#62860=CARTESIAN_POINT ( 'NONE',  ( 85.86466870016465691, 43.03755298354901981, -2.506393329082034160 ) ) ;
#62865=DIRECTION ( 'NONE',  ( 0.5000000000000014433, -0.8660254037844378194, 0.000000000000000000 ) ) ;
#62868=AXIS2_PLACEMENT_3D ( 'NONE', #30042, #60930, #22446 ) ;
#62869=VECTOR ( 'NONE', #47575, 1000.000000000000000 ) ;
#62876=CARTESIAN_POINT ( 'NONE',  ( 25.14222138719033595, 29.91421378149919974, 9.188101187500008038 ) ) ;
#62881=CARTESIAN_POINT ( 'NONE',  ( 74.32474745866193189, 68.52230083288840490, 11.65590001247777252 ) ) ;
#62888=EDGE_CURVE ( 'NONE', #79874, #7443, #30071, .T. ) ;
#62897=EDGE_CURVE ( 'NONE', #95476, #86521, #15206, .T. ) ;
#62903=CARTESIAN_POINT ( 'NONE',  ( 76.10657944533755881, 65.44108555233269442, 13.99905362479801951 ) ) ;
#62911=ADVANCED_FACE ( 'NONE', ( #76201 ), #99992, .T. ) ;
#62915=CARTESIAN_POINT ( 'NONE',  ( 68.45344762042827824, 64.57392882346940155, 12.12708197196866600 ) ) ;
#62918=CARTESIAN_POINT ( 'NONE',  ( 85.41673846469936393, 44.62557248619319950, -7.387197001228601678 ) ) ;
#62927=CARTESIAN_POINT ( 'NONE',  ( 85.53665298850141596, 48.34007191699684114, -12.21196891364053450 ) ) ;
#62929=CARTESIAN_POINT ( 'NONE',  ( 72.14622295904345606, 66.92643202321383455, 11.38291742270067530 ) ) ;
#62942=CARTESIAN_POINT ( 'NONE',  ( 20.42956747364522485, 12.76426979415089313, 3.090169943749476733 ) ) ;
#62946=CARTESIAN_POINT ( 'NONE',  ( 17.03907575219864867, 18.03677371833801502, 10.00000000000000533 ) ) ;
#62947=CARTESIAN_POINT ( 'NONE',  ( 84.03077106726578904, 48.73883679912442801, -13.14056060433543038 ) ) ;
#62949=CARTESIAN_POINT ( 'NONE',  ( 66.84345300777175680, 68.16924383811607413, -6.541651360653301772 ) ) ;
#62963=CARTESIAN_POINT ( 'NONE',  ( 32.94607225727562394, 21.94754757982091675, 5.678558825948272215 ) ) ;
#62970=CARTESIAN_POINT ( 'NONE',  ( 65.88354372152944904, 68.95778724155981365, 2.436355252633338520 ) ) ;
#62971=EDGE_LOOP ( 'NONE', ( #5799, #10608, #34163, #13091 ) ) ;
#62976=CARTESIAN_POINT ( 'NONE',  ( 8.474262601947446072, 26.93396525600388713, 2.839279412974139660 ) ) ;
#62992=CARTESIAN_POINT ( 'NONE',  ( 73.06582205585958434, 70.62793229939931905, 7.756361730470036520 ) ) ;
#62999=CARTESIAN_POINT ( 'NONE',  ( 79.33413028100275710, 59.08315638148421556, -16.22733909814880704 ) ) ;
#63001=FACE_OUTER_BOUND ( 'NONE', #63269, .T. ) ;
#63002=ORIENTED_EDGE ( 'NONE', *, *, #76521, .T. ) ;
#63006=B_SPLINE_CURVE_WITH_KNOTS ( 'NONE', 3,
 ( #32701, #49405, #80352, #41794, #56500, #3333, #71224, #32199, #1817, #63601, #94541, #72228, #34211, #9922, #79357, #11436, #40782, #71730, #95054, #10416, #87974, #2835, #79851, #33724 ),
 .UNSPECIFIED., .F., .F.,
 ( 4, 2, 2, 2, 2, 2, 2, 2, 2, 2, 2, 4 ),
 ( 0.000000000000000000, 0.1249999999999974742, 0.2499999999999949485, 0.3749999999999924505, 0.4374999999999911737, 0.4999999999999898970, 0.5624999999999886757, 0.6249999999999873435, 0.6874999999999861222, 0.7499999999999849010, 0.8749999999999924505, 1.000000000000000000 ),
 .UNSPECIFIED. ) ;
#63010=CARTESIAN_POINT ( 'NONE',  ( 73.14366643852760319, 60.29835623558181368, 15.26756996240958131 ) ) ;
#63016=DIRECTION ( 'NONE',  ( -0.8660254037844378194, -0.5000000000000013323, -0.000000000000000000 ) ) ;
#63020=CARTESIAN_POINT ( 'NONE',  ( 82.79952076536555694, 53.35385224299954388, -15.29414667009053197 ) ) ;
#63023=CARTESIAN_POINT ( 'NONE',  ( 15.62557774837418023, 29.99752408145591076, 5.678558825948277544 ) ) ;
#63028=VERTEX_POINT ( 'NONE', #32576 ) ;
#63043=CARTESIAN_POINT ( 'NONE',  ( 82.10452652000643070, 40.74900335645702398, -0.8276724821365912810 ) ) ;
#63044=B_SPLINE_CURVE_WITH_KNOTS ( 'NONE', 3,
 ( #39332, #35979, #13695, #93079, #100180, #12714, #70247, #77874, #46435, #15535 ),
 .UNSPECIFIED., .F., .F.,
 ( 4, 2, 2, 2, 4 ),
 ( 0.000000000000000000, 0.2500000000000000000, 0.5000000000000000000, 0.7500000000000000000, 1.000000000000000000 ),
 .UNSPECIFIED. ) ;
#63049=CARTESIAN_POINT ( 'NONE',  ( 75.69998711193903773, 65.59611928177264417, 13.80412242752735708 ) ) ;
#63054=LINE ( 'NONE', #63550, #79281 ) ;
#63057=DIRECTION ( 'NONE',  ( -0.8660254037844377084, -0.5000000000000014433, -0.000000000000000000 ) ) ;
#63058=CARTESIAN_POINT ( 'NONE',  ( 84.81383324307122962, 44.91740293199559630, 8.403696530403449216 ) ) ;
#63061=CARTESIAN_POINT ( 'NONE',  ( 74.46849378157413923, 68.15278936780924823, -11.56277540856588537 ) ) ;
#63064=PLANE ( 'NONE',  #46330 ) ;
#63066=DIRECTION ( 'NONE',  ( -0.4386133837897802090, -0.6599160945941812129, 0.6100238090894836152 ) ) ;
#63069=CARTESIAN_POINT ( 'NONE',  ( 68.62314303196725973, 64.18211696513540687, -12.51050211285727087 ) ) ;
#63072=CARTESIAN_POINT ( 'NONE',  ( 68.90560621877192204, 63.79076715805910425, -12.30144644517788421 ) ) ;
#63075=DIRECTION ( 'NONE',  ( -0.5000000000000014433, 0.8660254037844378194, 0.000000000000000000 ) ) ;
#63083=CARTESIAN_POINT ( 'NONE',  ( 11.39049277451480080, 29.68290643055186706, 3.479690158560446702E-15 ) ) ;
#63086=CARTESIAN_POINT ( 'NONE',  ( 71.47384123275857348, 72.35069954344788812, 1.100233114707620530 ) ) ;
#63088=CARTESIAN_POINT ( 'NONE',  ( 29.44299306155908624, 19.12755873383627403, -6.180339887498949025 ) ) ;
#63097=EDGE_LOOP ( 'NONE', ( #34722, #89012, #52712, #66525, #24401 ) ) ;
#63099=CARTESIAN_POINT ( 'NONE',  ( 82.21410988452117863, 40.73976263626466476, 3.762362152834606732 ) ) ;
#63102=CARTESIAN_POINT ( 'NONE',  ( 79.14312167556931854, 57.64441083166269664, 0.000000000000000000 ) ) ;
#63109=CARTESIAN_POINT ( 'NONE',  ( 37.97985170016632850, 33.87878583063844928, -9.188101187500006262 ) ) ;
#63112=CARTESIAN_POINT ( 'NONE',  ( 78.01910789048406514, 61.79390329888819622, 16.07883194446994324 ) ) ;
#63117=CARTESIAN_POINT ( 'NONE',  ( 86.53491854233801917, 47.25312861645894458, -10.16653990104887484 ) ) ;
#63122=FACE_OUTER_BOUND ( 'NONE', #29754, .T. ) ;
#63128=CARTESIAN_POINT ( 'NONE',  ( 77.25514995865366075, 49.69881203954133042, -14.99743653824481093 ) ) ;
#63130=CARTESIAN_POINT ( 'NONE',  ( 74.83300825804853673, 57.97047224133282128, 15.96654120040242830 ) ) ;
#63131=CARTESIAN_POINT ( 'NONE',  ( 79.13079929454947603, 52.80933996073559911, 15.63716892723882701 ) ) ;
#63136=CARTESIAN_POINT ( 'NONE',  ( 77.86555730066851311, 62.20866292688850052, -15.95979438352862090 ) ) ;
#63142=CARTESIAN_POINT ( 'NONE',  ( 70.45245543053056281, 60.92432115798627024, -14.97201685956949646 ) ) ;
#63143=CARTESIAN_POINT ( 'NONE',  ( 42.48198750171711424, 33.03085787977767041, 9.188101187500006262 ) ) ;
#63144=EDGE_LOOP ( 'NONE', ( #11714, #11897, #96209, #38150 ) ) ;
#63145=CARTESIAN_POINT ( 'NONE',  ( 85.72965280032694579, 48.53761792183082946, -12.28028246049512262 ) ) ;
#63151=CARTESIAN_POINT ( 'NONE',  ( 72.62875423623682991, 64.07121235873044895, 13.57049568789011218 ) ) ;
#63152=CARTESIAN_POINT ( 'NONE',  ( 81.29539683296886210, 43.25976067974499273, 9.624898955577574355 ) ) ;
#63153=CARTESIAN_POINT ( 'NONE',  ( 78.15243512869371045, 51.09092126905193254, 15.77939321497872172 ) ) ;
#63154=CARTESIAN_POINT ( 'NONE',  ( 36.02478613032081967, 22.92755873383628540, 6.180339887498953466 ) ) ;
#63156=VERTEX_POINT ( 'NONE', #3205 ) ;
#63157=B_SPLINE_CURVE_WITH_KNOTS ( 'NONE', 3,
 ( #70294, #31784, #79449, #904, #24206, #24696, #87072, #86074, #70810, #8019 ),
 .UNSPECIFIED., .F., .F.,
 ( 4, 2, 2, 2, 4 ),
 ( 0.000000000000000000, 0.2500000000000000000, 0.5000000000000000000, 0.7500000000000000000, 1.000000000000000000 ),
 .UNSPECIFIED. ) ;
#63159=CARTESIAN_POINT ( 'NONE',  ( 65.76755514393656199, 69.09664133051965962, -0.2187238748589619697 ) ) ;
#63161=DIRECTION ( 'NONE',  ( 0.8660254037844377084, 0.5000000000000015543, -0.000000000000000000 ) ) ;
#63166=EDGE_CURVE ( 'NONE', #59506, #52122, #44257, .T. ) ;
#63167=CARTESIAN_POINT ( 'NONE',  ( 71.23113041218663000, 71.96307377266813887, -2.934963719734108967 ) ) ;
#63171=VERTEX_POINT ( 'NONE', #89329 ) ;
#63173=CARTESIAN_POINT ( 'NONE',  ( 72.04273812837080015, 59.28583566120335746, 15.84548535902080246 ) ) ;
#63178=CARTESIAN_POINT ( 'NONE',  ( 73.77733668265750566, 68.41783923479601981, 11.46675506585084925 ) ) ;
#63181=CARTESIAN_POINT ( 'NONE',  ( 71.22043767567281236, 71.52608235244971979, -2.909787917308754857 ) ) ;
#63185=CARTESIAN_POINT ( 'NONE',  ( 87.87167583597285159, 44.45939398776243223, -3.944263742802939010 ) ) ;
#63188=CARTESIAN_POINT ( 'NONE',  ( 78.26604366595239526, 47.45132970578329434, 14.33273657485265318 ) ) ;
#63189=CARTESIAN_POINT ( 'NONE',  ( 77.96474761936472930, 54.41649311639740461, 16.03208068940686459 ) ) ;
#63190=CARTESIAN_POINT ( 'NONE',  ( 84.47860975560725194, 49.82577972120142817, -13.24615549146050952 ) ) ;
#63191=CARTESIAN_POINT ( 'NONE',  ( 77.66178915777496172, 61.94839236767001722, 15.64246823995104130 ) ) ;
#63192=CARTESIAN_POINT ( 'NONE',  ( 67.19266499973009843, 66.86638716927541282, 8.992916727549332023 ) ) ;
#63193=CARTESIAN_POINT ( 'NONE',  ( 75.97174564027631050, 51.49815502093342445, 16.18122344262006251 ) ) ;
#63195=B_SPLINE_CURVE_WITH_KNOTS ( 'NONE', 3,
 ( #52928, #46826, #15408, #92954, #62501, #91468, #6830, #23014, #93469, #83880, #14442, #45324, #45807, #46303, #54400, #37231, #30129, #38716, #39200, #24022, #7324, #61521, #77228, #100049, #29639, #38204, #70112, #68625, #85376, #15921, #77749 ),
 .UNSPECIFIED., .F., .F.,
 ( 4, 3, 3, 3, 3, 3, 3, 3, 3, 3, 4 ),
 ( 0.000000000000000000, 0.1333490885032399820, 0.3007194338854488058, 0.4699862290245400698, 0.5844252810809538179, 0.6686540514502882226, 0.7354980260655652469, 0.8028463152565959993, 0.8633854507757408037, 0.9437142632667595565, 1.000000000000000000 ),
 .UNSPECIFIED. ) ;
#63206=CARTESIAN_POINT ( 'NONE',  ( 88.50942844660002606, 43.88426665780151836, -0.4971503815960300887 ) ) ;
#63207=CARTESIAN_POINT ( 'NONE',  ( 4.698709606056801213, 26.21091486745858390, -1.111400068045478839E-16 ) ) ;
#63208=CARTESIAN_POINT ( 'NONE',  ( 86.04433559121571307, 43.25845178644564726, -4.809067209069766591 ) ) ;
#63211=CARTESIAN_POINT ( 'NONE',  ( 30.43941648770709207, 23.28920272979928541, -7.433330006724141015 ) ) ;
#63212=DIRECTION ( 'NONE',  ( 0.4755282581475757664, -0.8236391035463335175, -0.3090169943749448977 ) ) ;
#63214=CARTESIAN_POINT ( 'NONE',  ( 13.72994409607376731, 16.43085787977761569, -9.188101187500008038 ) ) ;
#63222=CARTESIAN_POINT ( 'NONE',  ( 79.42436089683208422, 55.33937033912253156, -16.05718545809815367 ) ) ;
#63223=CARTESIAN_POINT ( 'NONE',  ( 87.67135465677671391, 44.96834575157770075, -6.594061650049633627 ) ) ;
#63227=ORIENTED_EDGE ( 'NONE', *, *, #22069, .F. ) ;
#63228=CARTESIAN_POINT ( 'NONE',  ( 77.61293579238375173, 49.29402822633370818, 15.29643791220711257 ) ) ;
#63235=ORIENTED_EDGE ( 'NONE', *, *, #54384, .T. ) ;
#63238=CARTESIAN_POINT ( 'NONE',  ( 79.48743557011087546, 46.24584566380116968, -13.22586493812016961 ) ) ;
#63241=B_SPLINE_CURVE_WITH_KNOTS ( 'NONE', 3,
 ( #81641, #73027, #41082, #2623, #33512, #41591, #72533, #34024, #64912, #31737, #51183, #69753, #856, #38848, #93084, #82656 ),
 .UNSPECIFIED., .F., .F.,
 ( 4, 1, 2, 2, 2, 1, 2, 2, 4 ),
 ( 0.000000000000000000, 0.1250000000000028311, 0.1875000000000019706, 0.2500000000000011102, 0.4999999999999938938, 0.6249999999999916733, 0.6874999999999928946, 0.7499999999999941158, 1.000000000000000000 ),
 .UNSPECIFIED. ) ;
#63244=CARTESIAN_POINT ( 'NONE',  ( 20.47532000956703158, 32.79752408145593279, -5.678558825948271327 ) ) ;
#63246=CARTESIAN_POINT ( 'NONE',  ( 74.76064909570827410, 66.79516745633127073, -13.17056974000816183 ) ) ;
#63249=CYLINDRICAL_SURFACE ( 'NONE', #6128, 10.00000000000001066 ) ;
#63250=ORIENTED_EDGE ( 'NONE', *, *, #10980, .T. ) ;
#63253=FACE_OUTER_BOUND ( 'NONE', #27643, .T. ) ;
#63254=CARTESIAN_POINT ( 'NONE',  ( 68.10759289738595612, 66.09109068389082609, -10.54117928085663536 ) ) ;
#63255=CARTESIAN_POINT ( 'NONE',  ( 81.50264768554443151, 55.96797772595287057, -16.03733208502487173 ) ) ;
#63257=CARTESIAN_POINT ( 'NONE',  ( 41.58988463324670448, 24.41603393254329646, -1.583844403245396437 ) ) ;
#63261=CARTESIAN_POINT ( 'NONE',  ( 79.06677544641175359, 59.81915678714237572, 16.49560342610751107 ) ) ;
#63266=CARTESIAN_POINT ( 'NONE',  ( 77.86555730066851311, 62.20866292688850052, -15.95979438352862090 ) ) ;
#63267=ORIENTED_EDGE ( 'NONE', *, *, #58039, .F. ) ;
#63269=EDGE_LOOP ( 'NONE', ( #84244, #56524, #49812, #71642 ) ) ;
#63271=CARTESIAN_POINT ( 'NONE',  ( 80.02650856630110354, 44.34150727177379991, -11.51959576634213889 ) ) ;
#63272=CARTESIAN_POINT ( 'NONE',  ( 9.894862028763428796, 29.21091486745858745, -1.111400068045478839E-16 ) ) ;
#63273=CARTESIAN_POINT ( 'NONE',  ( 27.54669006335486614, 38.83705186507756224, 3.090169943749475401 ) ) ;
#63274=CARTESIAN_POINT ( 'NONE',  ( 80.14541552094489418, 48.42908552485922513, -13.75865811180872633 ) ) ;
#63282=CARTESIAN_POINT ( 'NONE',  ( 76.19947903059282623, 64.78545985970092147, -14.35372622111362340 ) ) ;
#63286=CARTESIAN_POINT ( 'NONE',  ( 87.97302621401057365, 44.79893962918851713, 4.797252263720211296 ) ) ;
#63288=CARTESIAN_POINT ( 'NONE',  ( 85.64888316943795132, 43.83034633356992060, -5.532248923516708494 ) ) ;
#63289=CARTESIAN_POINT ( 'NONE',  ( 78.41477381122238910, 47.32040575024741713, -14.22103711499937262 ) ) ;
#63294=CARTESIAN_POINT ( 'NONE',  ( 72.51358964696871112, 70.84733833069179809, 7.633428234268400558 ) ) ;
#63299=CARTESIAN_POINT ( 'NONE',  ( 82.41089694499171969, 41.02494636910944337, 1.928000225379814747 ) ) ;
#63301=CARTESIAN_POINT ( 'NONE',  ( 83.50089166959301679, 52.39794543819676420, 14.81166283256270688 ) ) ;
#63302=CYLINDRICAL_SURFACE ( 'NONE', #90009, 10.00000000000001066 ) ;
#63307=CARTESIAN_POINT ( 'NONE',  ( 76.03928946417400425, 63.29995371072659793, -14.91268113313668131 ) ) ;
#63309=FACE_BOUND ( 'NONE', #36867, .T. ) ;
#63310=CARTESIAN_POINT ( 'NONE',  ( 79.93310189433655921, 56.55788664210029992, 16.55897019584611840 ) ) ;
#63311=CARTESIAN_POINT ( 'NONE',  ( 30.64569906364082641, 29.64441083166262558, -10.00000000000000533 ) ) ;
#63315=CARTESIAN_POINT ( 'NONE',  ( 79.27712787825650764, 45.82676469203064329, -12.41914995154098911 ) ) ;
#63320=CARTESIAN_POINT ( 'NONE',  ( 81.76792596524467172, 46.55419044997203315, 11.93009829901677143 ) ) ;
#63328=CARTESIAN_POINT ( 'NONE',  ( 38.33870662942799612, 21.94473085651394939, 1.475505719884397138E-15 ) ) ;
#63331=CARTESIAN_POINT ( 'NONE',  ( 81.68874591563863419, 55.69259006457333783, 15.98051127425669016 ) ) ;
#63340=CARTESIAN_POINT ( 'NONE',  ( 68.67969803741280543, 66.83109073523215216, -9.305244569184894843 ) ) ;
#63347=CARTESIAN_POINT ( 'NONE',  ( 67.38141398091791245, 66.37704590880964872, -8.922811476558264232 ) ) ;
#63354=CARTESIAN_POINT ( 'NONE',  ( 27.86299091144838869, 21.80170272979927404, 7.433330006724137462 ) ) ;
#63359=CARTESIAN_POINT ( 'NONE',  ( 4.886862741447147052, 23.79752408145590081, -5.678558825948271327 ) ) ;
#63361=CARTESIAN_POINT ( 'NONE',  ( 77.07948589789764071, 58.51398417617086523, -16.11007920833352003 ) ) ;
#63362=CARTESIAN_POINT ( 'NONE',  ( 71.94004515418134815, 72.62285878051592647, -1.062404765500833070 ) ) ;
#63364=VERTEX_POINT ( 'NONE', #92779 ) ;
#63376=CARTESIAN_POINT ( 'NONE',  ( 71.64316818921395225, 72.05741665177615118, -3.509880912999884917 ) ) ;
#63377=CARTESIAN_POINT ( 'NONE',  ( 72.80497836564586578, 57.33751094343604393, -15.86650228098510773 ) ) ;
#63385=CARTESIAN_POINT ( 'NONE',  ( 24.44940106416278169, 29.51421378149920116, -9.188101187500004485 ) ) ;
#63390=CARTESIAN_POINT ( 'NONE',  ( 74.24116255903008721, 68.58322516222325760, 11.05893809163644725 ) ) ;
#63391=CARTESIAN_POINT ( 'NONE',  ( 31.49087468139936874, 26.38052372038642446, 10.00000000000000533 ) ) ;
#63396=CARTESIAN_POINT ( 'NONE',  ( 87.01921871845581791, 46.46248764730437131, 8.883936319678571891 ) ) ;
#63397=CARTESIAN_POINT ( 'NONE',  ( 84.88073312764632306, 43.04194891362699593, -4.562917901942581622 ) ) ;
#63402=CARTESIAN_POINT ( 'NONE',  ( 66.54075137518580618, 68.81555626029071959, -2.231460399992863497 ) ) ;
#63408=CARTESIAN_POINT ( 'NONE',  ( 87.60644657549313763, 43.46191668553660747, -1.868725964739645473 ) ) ;
#63409=CARTESIAN_POINT ( 'NONE',  ( 67.52176836666478721, 67.08338768382488126, 8.956287543224618730 ) ) ;
#63410=CARTESIAN_POINT ( 'NONE',  ( 75.35830705743131830, 64.29999869705460469, -14.30093840670493677 ) ) ;
#63415=CARTESIAN_POINT ( 'NONE',  ( 69.84840267283668425, 64.12174718186125233, 12.47111010752439775 ) ) ;
#63420=CARTESIAN_POINT ( 'NONE',  ( 83.86862482182540646, 51.60241004480363358, -14.38537263802609800 ) ) ;
#63421=CARTESIAN_POINT ( 'NONE',  ( 76.15170329134147664, 51.05213637843759500, -15.57434085608729468 ) ) ;
#63423=CARTESIAN_POINT ( 'NONE',  ( 80.42785451945398734, 57.51445601405281138, -16.58998511169260937 ) ) ;
#63432=CARTESIAN_POINT ( 'NONE',  ( 71.85042758235270810, 71.69843285251393183, -3.789477364735254650 ) ) ;
#63435=CARTESIAN_POINT ( 'NONE',  ( 85.37327613081673405, 48.30298695785122476, -11.79049452454833613 ) ) ;
#63439=CARTESIAN_POINT ( 'NONE',  ( 80.27865570437573695, 44.72452793390266379, -11.72932060911959518 ) ) ;
#63447=CARTESIAN_POINT ( 'NONE',  ( 82.97379378944903294, 51.10958875718078076, -14.34435646701223099 ) ) ;
#63452=CARTESIAN_POINT ( 'NONE',  ( 14.65590419365400976, 24.16454794089040448, -10.00000000000000355 ) ) ;
#63461=CARTESIAN_POINT ( 'NONE',  ( 66.39359272226485587, 68.79637079869742422, -4.330331651545298755 ) ) ;
#63468=CARTESIAN_POINT ( 'NONE',  ( 30.81771801958594281, 39.83396525600392835, -2.839279412974133887 ) ) ;
#63469=CARTESIAN_POINT ( 'NONE',  ( 80.37385980795637863, 57.92309568092906602, -16.24750533957013587 ) ) ;
#63475=FACE_OUTER_BOUND ( 'NONE', #65549, .T. ) ;
#63476=ORIENTED_EDGE ( 'NONE', *, *, #31199, .T. ) ;
#63477=DIRECTION ( 'NONE',  ( 0.7691052716734860795, 0.08748735329024150131, -0.6331058711608366085 ) ) ;
#63480=CARTESIAN_POINT ( 'NONE',  ( 5.558032429380089567, 24.18502408145589655, 5.678558825948276656 ) ) ;
#63493=CARTESIAN_POINT ( 'NONE',  ( 86.44281908042910345, 47.25702098485090374, 10.76508247627446302 ) ) ;
#63495=CARTESIAN_POINT ( 'NONE',  ( 69.40701071331325522, 66.80176887165785615, 10.58398152440570783 ) ) ;
#63498=CARTESIAN_POINT ( 'NONE',  ( 68.76720517553677325, 63.84246230342036199, -12.20210122296020216 ) ) ;
#63499=CARTESIAN_POINT ( 'NONE',  ( 84.96125173846019152, 48.42999138336367082, -12.07229602349086584 ) ) ;
#63510=ORIENTED_EDGE ( 'NONE', *, *, #218, .T. ) ;
#63512=CARTESIAN_POINT ( 'NONE',  ( 74.58922631747108767, 66.95469429158355013, 12.55546573254311937 ) ) ;
#63516=CARTESIAN_POINT ( 'NONE',  ( 83.08735981439933482, 48.59651280663791084, 12.88586852374721126 ) ) ;
#63517=CARTESIAN_POINT ( 'NONE',  ( 70.50418369191052648, 67.51709059444762318, 9.786528338479930866 ) ) ;
#63524=CARTESIAN_POINT ( 'NONE',  ( 22.39139443204644664, 24.87878583063842086, -9.188101187500006262 ) ) ;
#63541=CARTESIAN_POINT ( 'NONE',  ( 82.14352512031462084, 40.76412825037346721, -0.7169653898824394078 ) ) ;
#63545=CARTESIAN_POINT ( 'NONE',  ( 75.84977083960791333, 65.49147256048033228, 14.30114164871031335 ) ) ;
#63547=ORIENTED_EDGE ( 'NONE', *, *, #2899, .F. ) ;
#63550=CARTESIAN_POINT ( 'NONE',  ( 1.396987757676509734, 24.30466486950695071, 0.000000000000000000 ) ) ;
#63553=CARTESIAN_POINT ( 'NONE',  ( 88.22357128540845395, 44.11249832625940570, 0.5032066602140912170 ) ) ;
#63554=B_SPLINE_CURVE_WITH_KNOTS ( 'NONE', 3,
 ( #78911, #1894, #85538, #16080, #39852, #24185, #94123, #39358, #71302, #86544, #17075, #62666, #46985, #55068, #70272, #47965, #86053, #16578, #15562, #32276, #883, #47476, #87050, #31762 ),
 .UNSPECIFIED., .F., .F.,
 ( 4, 2, 2, 2, 2, 2, 2, 2, 2, 2, 2, 4 ),
 ( 0.000000000000000000, 0.1249999999999993894, 0.2499999999999987788, 0.3749999999999981681, 0.4374999999999897304, 0.4999999999999812372, 0.5624999999999726885, 0.6249999999999642508, 0.6874999999999557021, 0.7499999999999471534, 0.8749999999999735767, 1.000000000000000000 ),
 .UNSPECIFIED. ) ;
#63556=CARTESIAN_POINT ( 'NONE',  ( 33.14931559527707350, 20.10801979619930435, 3.090169943749476733 ) ) ;
#63559=CARTESIAN_POINT ( 'NONE',  ( 74.20878020607858616, 68.72316200637693839, -11.41572480156362879 ) ) ;
#63564=CARTESIAN_POINT ( 'NONE',  ( 82.68335232665059209, 44.33947160102358964, 9.174560444508216506 ) ) ;
#63582=CARTESIAN_POINT ( 'NONE',  ( 10.31635424878816742, 24.14336893147753926, 7.433330006724141015 ) ) ;
#63583=CARTESIAN_POINT ( 'NONE',  ( 73.03004930954443807, 60.83881918362380503, -15.55364876364052051 ) ) ;
#63589=CARTESIAN_POINT ( 'NONE',  ( 20.88255934282640425, 35.55466486950700045, -1.111400068045478839E-16 ) ) ;
#63591=CARTESIAN_POINT ( 'NONE',  ( 41.76871284172324295, 36.06628583063844928, -9.188101187500006262 ) ) ;
#63593=DIRECTION ( 'NONE',  ( -0.4493970231495795775, 0.7783784768652820540, -0.4383711467890876734 ) ) ;
#63600=CARTESIAN_POINT ( 'NONE',  ( 79.24255149360672590, 50.29911346356186641, 14.82443660399750485 ) ) ;
#63601=CARTESIAN_POINT ( 'NONE',  ( 83.91397729048109966, 51.84092357031820342, -14.47588020021706612 ) ) ;
#63602=FACE_OUTER_BOUND ( 'NONE', #26420, .T. ) ;
#63605=PLANE ( 'NONE',  #98987 ) ;
#63606=CARTESIAN_POINT ( 'NONE',  ( 31.85034293892215018, 41.49540643055189548, 3.479690158560446702E-15 ) ) ;
#63608=ORIENTED_EDGE ( 'NONE', *, *, #3840, .F. ) ;
#63614=CARTESIAN_POINT ( 'NONE',  ( 86.33167747996513697, 46.96304910452010262, -10.52679092302836317 ) ) ;
#63618=CARTESIAN_POINT ( 'NONE',  ( 25.96360177180014972, 20.15404122711134249, 8.090169943749479842 ) ) ;
#63619=LINE ( 'NONE', #72757, #81838 ) ;
#63621=CARTESIAN_POINT ( 'NONE',  ( 80.24672568527826400, 44.80204066275088337, 11.13114128994728524 ) ) ;
#63622=CARTESIAN_POINT ( 'NONE',  ( 84.85099494643192486, 49.96072780641430455, -13.19879633021795939 ) ) ;
#63628=CARTESIAN_POINT ( 'NONE',  ( 77.28539951127001473, 49.71994323448210196, -14.99865734462259148 ) ) ;
#63630=ORIENTED_EDGE ( 'NONE', *, *, #508, .F. ) ;
#63632=CARTESIAN_POINT ( 'NONE',  ( 78.19591265575934358, 48.92920433772970057, 14.51337752615410359 ) ) ;
#63638=CARTESIAN_POINT ( 'NONE',  ( 79.01390229250786490, 46.15383090619681639, 12.74691942439358350 ) ) ;
#63644=CARTESIAN_POINT ( 'NONE',  ( 70.70263562602700347, 60.54883119609748832, -14.66132127786565142 ) ) ;
#63645=CARTESIAN_POINT ( 'NONE',  ( 44.43411998782967487, 26.44966523072497822, -2.296566073217252530E-15 ) ) ;
#63647=CARTESIAN_POINT ( 'NONE',  ( 86.59925754919576946, 43.68706288513137537, -5.068886987635317531 ) ) ;
#63650=DIRECTION ( 'NONE',  ( -0.5000000000000014433, 0.8660254037844377084, 0.000000000000000000 ) ) ;
#63653=CARTESIAN_POINT ( 'NONE',  ( 72.38627258597001912, 63.15220171016905226, 13.97079549884010596 ) ) ;
#63656=CARTESIAN_POINT ( 'NONE',  ( 28.39959312520600676, 35.13478043621390157, 8.090169943749478065 ) ) ;
#63674=B_SPLINE_SURFACE_WITH_KNOTS ( 'NONE', 3, 1, ( 
 ( #83765, #15296 ),
 ( #45214, #13825 ),
 ( #76152, #44704 ),
 ( #37605, #86780 ),
 ( #70513, #54293 ),
 ( #32525, #32003 ),
 ( #63914, #78134 ),
 ( #16813, #8721 ),
 ( #23404, #33015 ),
 ( #31503, #85263 ),
 ( #47700, #15808 ),
 ( #33525, #79667 ),
 ( #17314, #55787 ),
 ( #86277, #62398 ),
 ( #2638, #622 ),
 ( #56305, #63420 ),
 ( #92851, #41098 ),
 ( #79166, #93353 ),
 ( #94853, #48218 ),
 ( #1642, #78638 ),
 ( #8225, #48733 ),
 ( #40098, #17834 ),
 ( #24420, #9745 ),
 ( #46713, #54810 ),
 ( #39592, #40603 ),
 ( #77641, #71539 ),
 ( #2132, #25413 ),
 ( #87301, #10229 ),
 ( #72034, #47211 ),
 ( #93864, #39094 ),
 ( #70007, #23910 ) ),
 .UNSPECIFIED., .F., .F., .F.,
 ( 4, 3, 3, 3, 3, 3, 3, 3, 3, 3, 4 ),
 ( 2, 2 ),
 ( 0.000000000000000000, 0.1333490885032327655, 0.3007194338854324855, 0.4699862290245073182, 0.5844252810809297261, 0.6686540514502762322, 0.7354980260655518132, 0.8028463152565620264, 0.8633854507757146024, 0.9437142632667205877, 1.000000000000000000 ),
 ( 0.000000000000000000, 1.000000000000000000 ),
 .UNSPECIFIED. ) ;
#63678=EDGE_CURVE ( 'NONE', #41092, #99018, #17128, .T. ) ;
#63692=CARTESIAN_POINT ( 'NONE',  ( 77.57362400355269472, 52.51412412160524923, 15.74026747803791437 ) ) ;
#63694=CARTESIAN_POINT ( 'NONE',  ( 77.93222884788742988, 62.01307363188976751, 15.66297058137760345 ) ) ;
#63697=CARTESIAN_POINT ( 'NONE',  ( 76.61699804220991439, 51.35236863086766590, 16.07092595041460470 ) ) ;
#63701=CARTESIAN_POINT ( 'NONE',  ( 75.85550969639162133, 55.85942037733559573, -16.16270098209340489 ) ) ;
#63703=CARTESIAN_POINT ( 'NONE',  ( 73.67568143663486069, 69.57707014568420334, 9.664179533016600487 ) ) ;
#63705=EDGE_CURVE ( 'NONE', #46236, #35455, #10545, .T. ) ;
#63709=PLANE ( 'NONE',  #65392 ) ;
#63711=PLANE ( 'NONE',  #11269 ) ;
#63712=CARTESIAN_POINT ( 'NONE',  ( 74.67000616351420206, 66.81477949400924388, -13.12245706047550797 ) ) ;
#63714=CARTESIAN_POINT ( 'NONE',  ( 25.62156559687931434, 36.83396525600391413, -2.839279412974133887 ) ) ;
#63718=CARTESIAN_POINT ( 'NONE',  ( 15.51250667149479590, 27.14336893147754992, 7.433330006724141015 ) ) ;
#63720=CARTESIAN_POINT ( 'NONE',  ( 76.53355563625230218, 63.67723833686833501, 14.89832570204743156 ) ) ;
#63726=CARTESIAN_POINT ( 'NONE',  ( 87.56524498856292382, 45.09937575355993999, -6.113837049084305697 ) ) ;
#63730=VERTEX_POINT ( 'NONE', #32828 ) ;
#63731=VECTOR ( 'NONE', #88063, 1000.000000000000114 ) ;
#63734=VERTEX_POINT ( 'NONE', #41930 ) ;
#63737=CARTESIAN_POINT ( 'NONE',  ( 71.86256228778262312, 72.60615528678948749, -0.5650332253008888417 ) ) ;
#63738=VERTEX_POINT ( 'NONE', #26735 ) ;
#63742=CARTESIAN_POINT ( 'NONE',  ( 72.48128350488923388, 71.72257018173657173, 5.902110541236701202 ) ) ;
#63747=CARTESIAN_POINT ( 'NONE',  ( 25.85549604718420014, 26.87878583063842797, -9.188101187500006262 ) ) ;
#63748=CARTESIAN_POINT ( 'NONE',  ( 80.11408820379499218, 44.30976117890687505, 11.44504534144087415 ) ) ;
#63749=CARTESIAN_POINT ( 'NONE',  ( 84.55537670905214043, 50.62155581810768012, -14.09136642048690646 ) ) ;
#63754=ORIENTED_EDGE ( 'NONE', *, *, #63853, .T. ) ;
#63756=CARTESIAN_POINT ( 'NONE',  ( 67.64202414628154258, 65.88146472340838500, 10.47854541773734738 ) ) ;
#63769=VERTEX_POINT ( 'NONE', #40908 ) ;
#63774=DIRECTION ( 'NONE',  ( -0.5000000000000013323, 0.8660254037844379305, 0.000000000000000000 ) ) ;
#63776=CARTESIAN_POINT ( 'NONE',  ( 81.06232478827473642, 48.19955485970237419, -13.34453326799301465 ) ) ;
#63781=ORIENTED_EDGE ( 'NONE', *, *, #64816, .T. ) ;
#63782=CARTESIAN_POINT ( 'NONE',  ( 76.15759952524373944, 64.74876932168429278, -14.35981515594801117 ) ) ;
#63801=CARTESIAN_POINT ( 'NONE',  ( 83.61997526984366402, 42.04153653030706295, 3.612101932814229865 ) ) ;
#63803=FACE_OUTER_BOUND ( 'NONE', #21030, .T. ) ;
#63813=CARTESIAN_POINT ( 'NONE',  ( 34.62385580964452458, 25.15404122711136026, 8.090169943749479842 ) ) ;
#63816=CARTESIAN_POINT ( 'NONE',  ( 85.48133813011057214, 42.12748250430919938, 0.7844986839966693326 ) ) ;
#63820=CARTESIAN_POINT ( 'NONE',  ( 85.93470712620026575, 48.23248545518190866, 11.93606436224419909 ) ) ;
#63824=CARTESIAN_POINT ( 'NONE',  ( 82.05688055765639888, 41.79543639811913636, 5.447568203553421640 ) ) ;
#63827=CARTESIAN_POINT ( 'NONE',  ( 34.73240388683179702, 38.79103043416552765, 8.090169943749478065 ) ) ;
#63833=CARTESIAN_POINT ( 'NONE',  ( 87.02632046633624441, 46.40069582530824022, -8.775412300074195926 ) ) ;
#63837=CARTESIAN_POINT ( 'NONE',  ( 70.65091078760467269, 66.69545628194936171, -10.73269157464200063 ) ) ;
#63850=CARTESIAN_POINT ( 'NONE',  ( 21.59633513308047270, 30.65586893147756697, -7.433330006724137462 ) ) ;
#63853=EDGE_CURVE ( 'NONE', #2203, #90942, #68329, .T. ) ;
#63856=CARTESIAN_POINT ( 'NONE',  ( 8.534987971495436199, 16.87878583063839599, -9.188101187500006262 ) ) ;
#63858=CARTESIAN_POINT ( 'NONE',  ( 70.80322137413752159, 60.50400129575321273, -14.70302039727343413 ) ) ;
#63861=CARTESIAN_POINT ( 'NONE',  ( 72.43677597718138372, 71.19342475292700101, -6.085942204204715544 ) ) ;
#63862=CARTESIAN_POINT ( 'NONE',  ( 85.32021429529936540, 49.09450955528861726, 12.43078529658329501 ) ) ;
#63866=EDGE_CURVE ( 'NONE', #90587, #86729, #4279, .T. ) ;
#63867=VERTEX_POINT ( 'NONE', #75848 ) ;
#63872=CARTESIAN_POINT ( 'NONE',  ( 35.07028576228009342, 43.18080186712595747, 3.090169943749475401 ) ) ;
#63873=CARTESIAN_POINT ( 'NONE',  ( 71.98986200492696241, 72.23686350399877654, -3.591898176886850980 ) ) ;
#63874=CARTESIAN_POINT ( 'NONE',  ( 72.84182891927886772, 57.62769808626433843, -16.30833842344255302 ) ) ;
#63884=CARTESIAN_POINT ( 'NONE',  ( 27.58754685475307156, 27.87878583063842797, -9.188101187500006262 ) ) ;
#63886=CARTESIAN_POINT ( 'NONE',  ( 68.84404707066741480, 70.34727783162064441, -3.881443619315931404 ) ) ;
#63888=CARTESIAN_POINT ( 'NONE',  ( 73.89028189157257032, 68.56231543382321547, 11.39439152759357832 ) ) ;
#63893=CARTESIAN_POINT ( 'NONE',  ( 77.90651215622740722, 57.43855308693908768, -16.18645963951878031 ) ) ;
#63895=CARTESIAN_POINT ( 'NONE',  ( 77.80402915230507688, 52.55141458490561490, 16.18111265596900594 ) ) ;
#63896=ORIENTED_EDGE ( 'NONE', *, *, #15269, .F. ) ;
#63898=CARTESIAN_POINT ( 'NONE',  ( 66.68553331399648698, 68.87473950154989666, -2.393764034506348004 ) ) ;
#63903=VECTOR ( 'NONE', #78200, 1000.000000000000114 ) ;
#63904=CARTESIAN_POINT ( 'NONE',  ( 83.45583532732622700, 42.49119406076365379, -6.508603157797417715 ) ) ;
#63905=CARTESIAN_POINT ( 'NONE',  ( 67.68597986140046885, 66.81033470680795006, 8.568866250934442874 ) ) ;
#63906=CARTESIAN_POINT ( 'NONE',  ( 69.41227148360343335, 65.59617998781489234, -11.06349461743358376 ) ) ;
#63907=DIRECTION ( 'NONE',  ( -0.5000000000000014433, 0.8660254037844379305, 0.000000000000000000 ) ) ;
#63911=CARTESIAN_POINT ( 'NONE',  ( 83.80819523040570118, 41.96166617173753366, 2.742002955682231846 ) ) ;
#63914=CARTESIAN_POINT ( 'NONE',  ( 83.77593207218663451, 52.15966500954240104, -15.02877900679588130 ) ) ;
#63917=CARTESIAN_POINT ( 'NONE',  ( 80.41821068662579819, 57.11076416847725312, -16.23042426913554692 ) ) ;
#63923=EDGE_CURVE ( 'NONE', #64236, #23117, #11496, .T. ) ;
#63928=CARTESIAN_POINT ( 'NONE',  ( 85.42558612123971784, 48.32295466858820987, -12.24938428992806116 ) ) ;
#63930=CARTESIAN_POINT ( 'NONE',  ( 88.07866424057203858, 44.70482641456190009, -4.324981154599603528 ) ) ;
#63931=CARTESIAN_POINT ( 'NONE',  ( 69.58738856513491555, 70.56840624901691683, -2.716338601311397483 ) ) ;
#63940=CARTESIAN_POINT ( 'NONE',  ( 80.15537031803718548, 52.05204710506983190, -15.26801063640590783 ) ) ;
#63941=ORIENTED_EDGE ( 'NONE', *, *, #55435, .F. ) ;
#63945=CARTESIAN_POINT ( 'NONE',  ( 17.05992553822454383, 21.80066082961421259, 10.00000000000000533 ) ) ;
#63946=CARTESIAN_POINT ( 'NONE',  ( 85.94199290331987129, 48.36193870280315110, 12.04004775853120357 ) ) ;
#63947=CARTESIAN_POINT ( 'NONE',  ( 85.02181358025761426, 48.43635879085736207, -12.52173728460538982 ) ) ;
#63949=CARTESIAN_POINT ( 'NONE',  ( 71.76351473723394747, 71.84897031608997509, 2.971691788643012977 ) ) ;
#63957=DIRECTION ( 'NONE',  ( 0.9634819383873026721, -0.2491829092639719911, 0.09803281150813247802 ) ) ;
#63960=CARTESIAN_POINT ( 'NONE',  ( 35.00289615805098009, 41.18502408145595695, 5.678558825948277544 ) ) ;
#63964=CARTESIAN_POINT ( 'NONE',  ( 32.94607225727562394, 21.94754757982091675, 5.678558825948272215 ) ) ;
#63967=CARTESIAN_POINT ( 'NONE',  ( 65.96121609362643312, 68.98813676735653644, 2.519541258661097682 ) ) ;
#63971=CARTESIAN_POINT ( 'NONE',  ( 8.697374518098678564, 25.99752408145590366, 5.678558825948277544 ) ) ;
#63973=CARTESIAN_POINT ( 'NONE',  ( 17.84595736030643920, 25.70171378149918695, -9.188101187500004485 ) ) ;
#63977=CARTESIAN_POINT ( 'NONE',  ( 84.70579481679399692, 49.94286076369812832, -13.65556694543043825 ) ) ;
#63978=CARTESIAN_POINT ( 'NONE',  ( 88.09947609552301628, 44.13539611768646864, -1.715919295570225822 ) ) ;
#63984=CARTESIAN_POINT ( 'NONE',  ( 66.04918351466359638, 68.55101183580894997, 4.476786609762311464 ) ) ;
#63990=CARTESIAN_POINT ( 'NONE',  ( 86.19418860658703352, 47.68766159785528913, 10.81734670790828368 ) ) ;
#63992=CARTESIAN_POINT ( 'NONE',  ( 77.78144776439313546, 57.65517096718075862, 16.17772494993696242 ) ) ;
#63996=CARTESIAN_POINT ( 'NONE',  ( 78.39750752953510471, 61.37713215747155004, -15.85865527802526564 ) ) ;
#63998=CARTESIAN_POINT ( 'NONE',  ( 84.40523410500765067, 47.35716185244744025, -11.94365264890164546 ) ) ;
#64000=VERTEX_POINT ( 'NONE', #61603 ) ;
#64011=EDGE_CURVE ( 'NONE', #24668, #73177, #30839, .T. ) ;
#64014=VECTOR ( 'NONE', #20058, 1000.000000000000000 ) ;
#64021=CARTESIAN_POINT ( 'NONE',  ( 71.37153584347667845, 69.28727247378522236, 8.201935042734072923 ) ) ;
#64022=DIRECTION ( 'NONE',  ( -0.4145187862775162602, 0.7179675985244458047, -0.5591929034707565638 ) ) ;
#64024=DIRECTION ( 'NONE',  ( -0.8660254037844377084, -0.5000000000000014433, -0.000000000000000000 ) ) ;
#64027=CARTESIAN_POINT ( 'NONE',  ( 20.93478768117288524, 17.80170272979926338, 7.433330006724137462 ) ) ;
#64037=B_SPLINE_CURVE_WITH_KNOTS ( 'NONE', 3,
 ( #13089, #83502, #44450, #5472, #13579, #75383, #6471, #68252, #99177, #17556, #56030, #94591 ),
 .UNSPECIFIED., .F., .F.,
 ( 4, 2, 2, 2, 2, 4 ),
 ( 0.000000000000000000, 0.2315728839045457232, 0.3473593258568164477, 0.4631457678090872276, 0.6947186517136287875, 0.9262915356181703475 ),
 .UNSPECIFIED. ) ;
#64048=EDGE_CURVE ( 'NONE', #51005, #93753, #44094, .T. ) ;
#64052=AXIS2_PLACEMENT_3D ( 'NONE', #97796, #21283, #99286 ) ;
#64060=CARTESIAN_POINT ( 'NONE',  ( 67.24282661209741718, 68.88379657313680582, 3.801344451262675950 ) ) ;
#64062=CARTESIAN_POINT ( 'NONE',  ( 71.71174882302004505, 58.93038559421764688, -15.88944412480316970 ) ) ;
#64066=CARTESIAN_POINT ( 'NONE',  ( 74.15402199957247831, 68.42859570829774896, -11.65141325894000879 ) ) ;
#64071=CARTESIAN_POINT ( 'NONE',  ( 83.09507021368182222, 45.14153989563129699, 9.863572327592716960 ) ) ;
#64074=CARTESIAN_POINT ( 'NONE',  ( 68.73183574854552091, 64.12522977685954118, -11.96507596856094402 ) ) ;
#64087=CARTESIAN_POINT ( 'NONE',  ( 21.36958804686389612, 14.19860640527291906, 2.839279412974134775 ) ) ;
#64088=CARTESIAN_POINT ( 'NONE',  ( 79.43862237908915347, 58.57025095756571176, -16.60657855749719758 ) ) ;
#64109=CARTESIAN_POINT ( 'NONE',  ( 35.31444455405989657, 43.49540643055190969, 3.479690158560446702E-15 ) ) ;
#64116=ADVANCED_FACE ( 'NONE', ( #81360 ), #35207, .T. ) ;
#64117=CARTESIAN_POINT ( 'NONE',  ( 78.80495087215344086, 60.04985905707439997, 16.11149256888698389 ) ) ;
#64120=CARTESIAN_POINT ( 'NONE',  ( 88.43398120015881148, 44.08421024288151102, -2.684292198961160114 ) ) ;
#64122=CARTESIAN_POINT ( 'NONE',  ( 81.74119788692269140, 59.14441083166271795, -0.5000000000000000000 ) ) ;
#64127=ORIENTED_EDGE ( 'NONE', *, *, #63866, .F. ) ;
#64132=CARTESIAN_POINT ( 'NONE',  ( 77.22537433491581282, 49.19994283889470665, -15.34347781851081116 ) ) ;
#64133=ORIENTED_EDGE ( 'NONE', *, *, #92162, .T. ) ;
#64134=CARTESIAN_POINT ( 'NONE',  ( 88.37406050535491886, 44.20074384979837845, 0.1102876639795926650 ) ) ;
#64135=CARTESIAN_POINT ( 'NONE',  ( 78.07934852507207779, 48.52740830546968454, 14.36491527075813579 ) ) ;
#64136=ORIENTED_EDGE ( 'NONE', *, *, #91820, .F. ) ;
#64145=CARTESIAN_POINT ( 'NONE',  ( 70.68908763585848476, 61.42051710150978749, -14.81853427669291534 ) ) ;
#64146=CARTESIAN_POINT ( 'NONE',  ( 36.01387044229257128, 42.83396525600393545, -2.839279412974133887 ) ) ;
#64148=CARTESIAN_POINT ( 'NONE',  ( 87.88600403731702215, 43.93895673462996143, -3.527816320842273257 ) ) ;
#64165=CARTESIAN_POINT ( 'NONE',  ( 65.99146032466613576, 68.67736554541691874, -0.3373263738352356711 ) ) ;
#64177=CARTESIAN_POINT ( 'NONE',  ( 72.32238060516027645, 62.28520104033361804, -14.34112121930858308 ) ) ;
#64180=CARTESIAN_POINT ( 'NONE',  ( 75.70957059507740894, 64.79295583396756797, -14.21030040932456728 ) ) ;
#64181=CARTESIAN_POINT ( 'NONE',  ( 85.60311072857605552, 48.35646458700439609, 11.69947488989744677 ) ) ;
#64187=CARTESIAN_POINT ( 'NONE',  ( 88.03836335721405248, 44.60032456687661551, -4.083393883595300977 ) ) ;
#64188=LINE ( 'NONE', #48497, #91654 ) ;
#64191=CARTESIAN_POINT ( 'NONE',  ( 78.32387762194203162, 56.55609178520109737, 16.20249635714992564 ) ) ;
#64193=CARTESIAN_POINT ( 'NONE',  ( 67.53167658295855347, 67.09922345392760690, 8.942594108559751120 ) ) ;
#64196=LINE ( 'NONE', #35289, #3869 ) ;
#64197=CARTESIAN_POINT ( 'NONE',  ( 80.48174699225948814, 54.15325549600505184, -15.80187059250945047 ) ) ;
#64201=CARTESIAN_POINT ( 'NONE',  ( 73.59537120146498523, 69.79291368717997557, 9.952181187355030545 ) ) ;
#64203=CARTESIAN_POINT ( 'NONE',  ( 76.71798530001490235, 63.32448642232582614, -15.43374014074777989 ) ) ;
#64208=CARTESIAN_POINT ( 'NONE',  ( 87.76955579613945702, 43.67712966683451725, -2.576982100675560439 ) ) ;
#64211=CARTESIAN_POINT ( 'NONE',  ( 32.08968265630384309, 27.03085787977765264, 9.188101187500006262 ) ) ;
#64212=CARTESIAN_POINT ( 'NONE',  ( 82.63458119455265205, 48.44224962061904449, -13.47290339139292925 ) ) ;
#64215=CARTESIAN_POINT ( 'NONE',  ( 19.96532700332172183, 20.03085787977762422, 9.188101187500006262 ) ) ;
#64217=CARTESIAN_POINT ( 'NONE',  ( 76.69221233506321767, 63.60975152925200859, 15.32791472565302016 ) ) ;
#64218=VECTOR ( 'NONE', #49324, 1000.000000000000000 ) ;
#64224=CARTESIAN_POINT ( 'NONE',  ( 87.60591442325252842, 44.91970625728536959, -6.572271063428638982 ) ) ;
#64227=CARTESIAN_POINT ( 'NONE',  ( 75.37954934236186944, 53.16236703070756420, 16.48630273753103026 ) ) ;
#64229=CARTESIAN_POINT ( 'NONE',  ( 82.29734961797254300, 53.60383310410944802, 15.81226994477781567 ) ) ;
#64234=ORIENTED_EDGE ( 'NONE', *, *, #1488, .T. ) ;
#64236=VERTEX_POINT ( 'NONE', #4826 ) ;
#64238=DIRECTION ( 'NONE',  ( -0.8660254037844377084, -0.5000000000000014433, -0.000000000000000000 ) ) ;
#64243=CARTESIAN_POINT ( 'NONE',  ( 35.22902474502244274, 28.84335787977765619, 9.188101187500006262 ) ) ;
#64244=CARTESIAN_POINT ( 'NONE',  ( 79.88938969212057373, 44.69895041751207998, 11.22585976794914586 ) ) ;
#64245=CARTESIAN_POINT ( 'NONE',  ( 84.81344185393595581, 50.36986395726449928, -13.44794441900970483 ) ) ;
#64246=CARTESIAN_POINT ( 'NONE',  ( 80.78636346040434546, 48.92950834313149500, -13.82546426373123438 ) ) ;
#64247=FACE_OUTER_BOUND ( 'NONE', #94427, .T. ) ;
#64248=ADVANCED_FACE ( 'NONE', ( #97556 ), #96077, .T. ) ;
#64250=ADVANCED_FACE ( 'NONE', ( #80379 ), #33751, .T. ) ;
#64252=ORIENTED_EDGE ( 'NONE', *, *, #55148, .T. ) ;
#64262=CARTESIAN_POINT ( 'NONE',  ( 79.55938800887707885, 59.45545654668635649, 16.55147640184673108 ) ) ;
#64272=B_SPLINE_CURVE_WITH_KNOTS ( 'NONE', 3,
 ( #35923, #6027, #12654, #28322, #73944, #44006, #83067, #75442, #36416, #97753 ),
 .UNSPECIFIED., .F., .F.,
 ( 4, 2, 2, 2, 4 ),
 ( 0.000000000000000000, 0.2500000000000000000, 0.5000000000000000000, 0.7500000000000000000, 1.000000000000000000 ),
 .UNSPECIFIED. ) ;
#64273=CARTESIAN_POINT ( 'NONE',  ( 80.19651160619561381, 44.67774917954261582, -11.72988265430777055 ) ) ;
#64274=CARTESIAN_POINT ( 'NONE',  ( 67.05615745758373691, 67.62596409448416068, 6.666417839661090916 ) ) ;
#64275=CARTESIAN_POINT ( 'NONE',  ( 73.62250635243424313, 69.55784274833359859, 10.23584637956792776 ) ) ;
#64277=CARTESIAN_POINT ( 'NONE',  ( 82.97933013574042604, 41.49896216930607551, -2.766843078683310253 ) ) ;
#64278=CARTESIAN_POINT ( 'NONE',  ( 85.04283770205356063, 47.23198909375206966, -10.98040028159587322 ) ) ;
#64288=CARTESIAN_POINT ( 'NONE',  ( 68.01423091693212086, 69.07147863764068063, -4.702031134324633044 ) ) ;
#64289=CARTESIAN_POINT ( 'NONE',  ( 87.55613534105700069, 44.89236293052572790, -6.575074172489557611 ) ) ;
#64291=CARTESIAN_POINT ( 'NONE',  ( 88.14062891587492743, 44.42319542341160599, 4.630203861778126928 ) ) ;
#64294=CARTESIAN_POINT ( 'NONE',  ( 86.45475614751083526, 43.94238033638490748, -4.660792038277363325 ) ) ;
#64297=CARTESIAN_POINT ( 'NONE',  ( 80.47957521310596007, 43.62501291645610024, 9.811056319678726823 ) ) ;
#64298=CARTESIAN_POINT ( 'NONE',  ( 71.47272524832681029, 59.15296923211511171, -15.79140392200444332 ) ) ;
#64299=CARTESIAN_POINT ( 'NONE',  ( 74.24029763082349120, 55.47955095029949746, -16.12046342301015756 ) ) ;
#64304=CARTESIAN_POINT ( 'NONE',  ( 86.25587912986354411, 45.60430133017160870, 8.273538712114721250 ) ) ;
#64305=CARTESIAN_POINT ( 'NONE',  ( 21.09856983598611535, 20.38052372038640669, 10.00000000000000533 ) ) ;
#64306=CARTESIAN_POINT ( 'NONE',  ( 78.44203751522358914, 61.21016990572090322, 16.24725970467587999 ) ) ;
#64309=CARTESIAN_POINT ( 'NONE',  ( 35.77580382318486585, 22.78380873178790011, -6.180339887498949025 ) ) ;
#64311=EDGE_CURVE ( 'NONE', #80395, #67223, #31891, .T. ) ;
#64314=CARTESIAN_POINT ( 'NONE',  ( 79.51440259700740398, 53.51398053849010950, 16.18861449462646007 ) ) ;
#64315=CARTESIAN_POINT ( 'NONE',  ( 26.66754231763712824, 34.13478043621389446, 8.090169943749478065 ) ) ;
#64319=CARTESIAN_POINT ( 'NONE',  ( 85.85358028005475717, 43.51426421455354898, -4.436799439580211057 ) ) ;
#64325=CARTESIAN_POINT ( 'NONE',  ( 26.07871176553302917, 38.55466486950701466, 7.012934429366973338E-14 ) ) ;
#64326=CARTESIAN_POINT ( 'NONE',  ( 71.95199650962558735, 72.63932214931871556, -0.9219114722910072279 ) ) ;
#64330=CARTESIAN_POINT ( 'NONE',  ( 32.84085557565775559, 19.36477965099641452, 1.583844403245330712 ) ) ;
#64331=CARTESIAN_POINT ( 'NONE',  ( 33.33147356615550194, 41.01751292744059185, 6.180339887498949913 ) ) ;
#64336=CARTESIAN_POINT ( 'NONE',  ( 7.019590965729775256, 22.79103043416547081, 8.090169943749478065 ) ) ;
#64340=DIRECTION ( 'NONE',  ( -0.2359789242578327062, -0.9717581732643756354, 0.000000000000000000 ) ) ;
#64351=CARTESIAN_POINT ( 'NONE',  ( 71.66369827319218189, 72.02185750324218816, -1.551229696566573502 ) ) ;
#64353=CARTESIAN_POINT ( 'NONE',  ( 21.83270445532239989, 34.64646525600390703, -2.839279412974133887 ) ) ;
#64357=ORIENTED_EDGE ( 'NONE', *, *, #92741, .F. ) ;
#64359=CARTESIAN_POINT ( 'NONE',  ( 12.93244592517074487, 8.262165230724926701, -2.296566073217252530E-15 ) ) ;
#64361=CARTESIAN_POINT ( 'NONE',  ( 87.90770736294503251, 44.20194146633631505, 2.808464138919696484 ) ) ;
#64362=ORIENTED_EDGE ( 'NONE', *, *, #40001, .F. ) ;
#64364=EDGE_CURVE ( 'NONE', #82741, #71517, #57018, .T. ) ;
#64369=ORIENTED_EDGE ( 'NONE', *, *, #20805, .F. ) ;
#64372=FACE_OUTER_BOUND ( 'NONE', #33860, .T. ) ;
#64375=ORIENTED_EDGE ( 'NONE', *, *, #30343, .T. ) ;
#64378=CARTESIAN_POINT ( 'NONE',  ( 72.03933155393818311, 72.41131128147422658, -2.965003495713515402 ) ) ;
#64379=CARTESIAN_POINT ( 'NONE',  ( 73.09905864054320546, 57.42323756090770814, -15.88034204403881589 ) ) ;
#64380=CARTESIAN_POINT ( 'NONE',  ( 78.16855185334185308, 61.58847221756811052, -16.14202726422458767 ) ) ;
#64381=DIRECTION ( 'NONE',  ( -0.5000000000000013323, 0.8660254037844378194, 0.000000000000000000 ) ) ;
#64388=CARTESIAN_POINT ( 'NONE',  ( 30.11829213135327521, 40.49540643055189548, 3.479690158560446702E-15 ) ) ;
#64390=CARTESIAN_POINT ( 'NONE',  ( 65.82437655349816907, 69.12761348810170148, -0.3171013769033947383 ) ) ;
#64392=CARTESIAN_POINT ( 'NONE',  ( 74.40608543823466903, 68.34271654374390437, 11.35151599582641424 ) ) ;
#64393=( BOUNDED_CURVE ( )  B_SPLINE_CURVE ( 2, ( #31037, #61925, #92876, #50233, #11267, #25440, #41123, #86805, #64446, #94877, #42619, #88807, #11755 ),
 .UNSPECIFIED., .F., .T. ) 
 B_SPLINE_CURVE_WITH_KNOTS ( ( 3, 2, 2, 2, 2, 2, 3 ),
 ( 0.3624999999999999889, 0.3649999999999999911, 0.3699999999999999956, 0.3750000000000000000, 0.3800000000000000044, 0.3850000000000000089, 0.3875000000000000111 ),
 .UNSPECIFIED. ) 
 CURVE ( )  GEOMETRIC_REPRESENTATION_ITEM ( )  RATIONAL_B_SPLINE_CURVE ( ( 0.9755282581475768211, 0.9755282581475768211, 1.000000000000000000, 0.9510565162951535312, 1.000000000000000000, 0.9510565162951535312, 1.000000000000000000, 0.9510565162951535312, 1.000000000000000000, 0.9510565162951535312, 1.000000000000000000, 0.9755282581475768211, 0.9755282581475768211 ) ) 
 REPRESENTATION_ITEM ( '' )  );
#64398=CARTESIAN_POINT ( 'NONE',  ( 76.72068702196582990, 57.86501502775809058, -16.11583960702630591 ) ) ;
#64399=CARTESIAN_POINT ( 'NONE',  ( 85.95981172767709211, 43.29180227630435951, -3.360722111609490526 ) ) ;
#64417=CARTESIAN_POINT ( 'NONE',  ( 87.51397647008028002, 44.34712510374425420, -4.234924872237962212 ) ) ;
#64418=CARTESIAN_POINT ( 'NONE',  ( 82.57480368249606784, 41.04376301281222794, 1.111617510708536205 ) ) ;
#64421=CARTESIAN_POINT ( 'NONE',  ( 74.72979125799862743, 60.84138562765400593, 15.40639291555719481 ) ) ;
#64423=EDGE_LOOP ( 'NONE', ( #57653, #39594, #57675, #69768 ) ) ;
#64424=CARTESIAN_POINT ( 'NONE',  ( 80.44351032975033888, 57.11231280812273781, -16.22991141722204134 ) ) ;
#64426=CARTESIAN_POINT ( 'NONE',  ( 71.88200430141152708, 72.22488123539891092, 0.5832661070486506727 ) ) ;
#64429=CARTESIAN_POINT ( 'NONE',  ( 74.62796085038830540, 66.91441896689961766, 13.03852793085608397 ) ) ;
#64437=CARTESIAN_POINT ( 'NONE',  ( 77.09656746912297365, 60.26159968811153078, -16.27885049838763720 ) ) ;
#64446=CARTESIAN_POINT ( 'NONE',  ( 23.63615849558155446, 18.81029122506294726, 8.090169943749479842 ) ) ;
#64452=CARTESIAN_POINT ( 'NONE',  ( 14.27891468289787369, 30.01751292744055277, 6.180339887498949913 ) ) ;
#64453=CARTESIAN_POINT ( 'NONE',  ( 88.10161777267849459, 43.64076697146427364, 0.1132407729617426612 ) ) ;
#64457=CARTESIAN_POINT ( 'NONE',  ( 72.23865006290039048, 71.95475215217994958, 3.607730569270007237 ) ) ;
#64458=CARTESIAN_POINT ( 'NONE',  ( 11.77607482435655051, 8.927558733836240989, 6.180339887498953466 ) ) ;
#64460=CARTESIAN_POINT ( 'NONE',  ( 3.562051267137642085, 25.55466486950697558, -1.111400068045478839E-16 ) ) ;
#64471=CARTESIAN_POINT ( 'NONE',  ( 32.17510246534131113, 41.68290643055190259, 3.479690158560446702E-15 ) ) ;
#64475=CARTESIAN_POINT ( 'NONE',  ( 32.17510246534131113, 41.68290643055190259, 3.479690158560446702E-15 ) ) ;
#64478=CARTESIAN_POINT ( 'NONE',  ( 66.54264984482914258, 68.81226801441182772, 2.258477026830885581 ) ) ;
#64480=FACE_OUTER_BOUND ( 'NONE', #32874, .T. ) ;
#64482=CARTESIAN_POINT ( 'NONE',  ( 9.401013375279877238, 17.37878583063838889, 9.188101187500006262 ) ) ;
#64484=CARTESIAN_POINT ( 'NONE',  ( 15.60392711327956761, 29.98502408145592213, -5.678558825948271327 ) ) ;
#64492=CARTESIAN_POINT ( 'NONE',  ( 66.06021207013861840, 68.53184239669842270, 4.555218141334386850 ) ) ;
#64493=CARTESIAN_POINT ( 'NONE',  ( 87.31810034388520592, 45.47295687595354252, 7.117869854781806005 ) ) ;
#64499=CARTESIAN_POINT ( 'NONE',  ( 86.70421956006907749, 47.09494090442339598, 10.43848816880117525 ) ) ;
#64501=CARTESIAN_POINT ( 'NONE',  ( 77.94705490036190554, 58.67815114825116041, 16.13782593773457918 ) ) ;
#64506=CARTESIAN_POINT ( 'NONE',  ( 84.22051715105205005, 48.65629006738927842, -12.53906321451517059 ) ) ;
#64507=B_SPLINE_CURVE_WITH_KNOTS ( 'NONE', 3,
 ( #94347, #16305, #17304, #48208, #63904, #40590, #1115, #25926, #94842, #24901, #18323, #55777, #80153, #63408, #33003, #78122 ),
 .UNSPECIFIED., .F., .F.,
 ( 4, 1, 2, 2, 2, 1, 2, 2, 4 ),
 ( 0.000000000000000000, 0.1249999999999967804, 0.1874999999999966693, 0.2499999999999965583, 0.4999999999999932276, 0.6249999999999914513, 0.6874999999999918954, 0.7499999999999924505, 1.000000000000000000 ),
 .UNSPECIFIED. ) ;
#64509=CARTESIAN_POINT ( 'NONE',  ( 80.72348862661678481, 43.14103115498581076, 9.877424986543475782 ) ) ;
#64510=ORIENTED_EDGE ( 'NONE', *, *, #41016, .F. ) ;
#64514=B_SPLINE_SURFACE_WITH_KNOTS ( 'NONE', 3, 1, ( 
 ( #22988, #83849 ),
 ( #37201, #14415 ),
 ( #22503, #84839 ),
 ( #85344, #68103 ),
 ( #37686, #53396 ),
 ( #84346, #59990 ),
 ( #7296, #77721 ),
 ( #30105, #15377 ),
 ( #45780, #61974 ),
 ( #38176, #99521 ),
 ( #46275, #77198 ),
 ( #7805, #38691 ),
 ( #90960, #69596 ),
 ( #54371, #23480 ),
 ( #15889, #46801 ),
 ( #24497, #94436 ),
 ( #79748, #70086 ),
 ( #72118, #2219 ),
 ( #39668, #54890 ),
 ( #93943, #1206 ),
 ( #9824, #71118 ),
 ( #9303, #49307 ),
 ( #25501, #62999 ),
 ( #80245, #23992 ),
 ( #32085, #17395 ),
 ( #33100, #70592 ),
 ( #16891, #86865 ),
 ( #47781, #40685 ),
 ( #1719, #93439 ),
 ( #48307, #39171 ),
 ( #17917, #698 ) ),
 .UNSPECIFIED., .F., .F., .F.,
 ( 4, 3, 3, 3, 3, 3, 3, 3, 3, 3, 4 ),
 ( 2, 2 ),
 ( 0.000000000000000000, 0.1333490885032387052, 0.3007194338854507487, 0.4699862290245374608, 0.5844252810809412724, 0.6686540514502781196, 0.7354980260655558100, 0.8028463152565722405, 0.8633854507757224850, 0.9437142632667419040, 1.000000000000000000 ),
 ( 0.000000000000000000, 1.000000000000000000 ),
 .UNSPECIFIED. ) ;
#64527=CARTESIAN_POINT ( 'NONE',  ( 72.43095172406538040, 71.17131323670344045, 6.069991975535843132 ) ) ;
#64531=ORIENTED_EDGE ( 'NONE', *, *, #50952, .F. ) ;
#64533=CARTESIAN_POINT ( 'NONE',  ( 24.91850453858129910, 20.10170272979927475, -7.433330006724141015 ) ) ;
#64537=VERTEX_POINT ( 'NONE', #44310 ) ;
#64547=DIRECTION ( 'NONE',  ( 0.5000000000000013323, -0.8660254037844378194, 0.000000000000000000 ) ) ;
#64553=CARTESIAN_POINT ( 'NONE',  ( 82.44400793032374963, 40.43910385561510878, -1.368357710041455011 ) ) ;
#64555=CARTESIAN_POINT ( 'NONE',  ( 84.81057673196700364, 50.23847654986280276, 13.36435190918987459 ) ) ;
#64563=UNCERTAINTY_MEASURE_WITH_UNIT (LENGTH_MEASURE( 1.000000000000000082E-05 ), #13615, 'distance_accuracy_value', 'NONE');
#64567=CARTESIAN_POINT ( 'NONE',  ( 66.77752810875767864, 68.40544692769400115, 4.459354299965320401 ) ) ;
#64568=CARTESIAN_POINT ( 'NONE',  ( 84.61167648532155283, 44.54557622999233502, 8.014713256522945528 ) ) ;
#64572=CARTESIAN_POINT ( 'NONE',  ( 69.04680748359113807, 64.17805710937504671, 12.06412625981762865 ) ) ;
#64578=CARTESIAN_POINT ( 'NONE',  ( 83.14942813903591912, 45.25422836440832697, 9.956978268961167444 ) ) ;
#64581=AXIS2_PLACEMENT_3D ( 'NONE', #48394, #1800, #54460 ) ;
#64583=CARTESIAN_POINT ( 'NONE',  ( 68.55321753847707100, 64.55974346124446583, -12.18496927705354516 ) ) ;
#64596=CARTESIAN_POINT ( 'NONE',  ( 15.40246583222295129, 30.93396525600389424, 2.839279412974139660 ) ) ;
#64607=CARTESIAN_POINT ( 'NONE',  ( 81.77341040013584461, 55.39003076602018183, -15.93424821120281010 ) ) ;
#64612=EDGE_CURVE ( 'NONE', #15371, #41986, #5822, .T. ) ;
#64617=EDGE_CURVE ( 'NONE', #13423, #52319, #77859, .T. ) ;
#64620=CARTESIAN_POINT ( 'NONE',  ( 45.46674490716588224, 28.11110640527296312, -2.839279412974138328 ) ) ;
#64625=EDGE_CURVE ( 'NONE', #50553, #5374, #16302, .T. ) ;
#64626=CARTESIAN_POINT ( 'NONE',  ( 82.73417970902306706, 44.01214333168216086, -9.530255576316653432 ) ) ;
#64627=ORIENTED_EDGE ( 'NONE', *, *, #52083, .F. ) ;
#64629=CARTESIAN_POINT ( 'NONE',  ( 79.01330593081745235, 59.80254073573071594, 16.49416071572547793 ) ) ;
#64633=VECTOR ( 'NONE', #33959, 1000.000000000000000 ) ;
#64634=CARTESIAN_POINT ( 'NONE',  ( 84.47860975560725194, 49.82577972120142817, -13.24615549146050952 ) ) ;
#64635=CARTESIAN_POINT ( 'NONE',  ( 84.77891510154978505, 49.87095472550759467, -13.17003612441266469 ) ) ;
#64639=EDGE_CURVE ( 'NONE', #44339, #97853, #79762, .T. ) ;
#64640=VERTEX_POINT ( 'NONE', #65506 ) ;
#64642=VERTEX_POINT ( 'NONE', #12320 ) ;
#64643=CARTESIAN_POINT ( 'NONE',  ( 77.53316523795550097, 49.65407854046259928, 14.92632681611246603 ) ) ;
#64647=CARTESIAN_POINT ( 'NONE',  ( 86.35121876318000034, 43.08468197994678661, 0.3078304325362931637 ) ) ;
#64649=DIRECTION ( 'NONE',  ( -0.4827766168686632997, -0.5834231310750495059, 0.6531035050674843800 ) ) ;
#64653=CARTESIAN_POINT ( 'NONE',  ( 86.45815904198641988, 42.74312041874679124, -1.243629510017558948 ) ) ;
#64657=CARTESIAN_POINT ( 'NONE',  ( 70.62475623734151498, 60.97173318496616190, -14.46351272653383369 ) ) ;
#64658=CARTESIAN_POINT ( 'NONE',  ( 39.32338737416051089, 38.10171378149922106, 9.188101187500008038 ) ) ;
#64660=VECTOR ( 'NONE', #24600, 1000.000000000000114 ) ;
#64661=CARTESIAN_POINT ( 'NONE',  ( 87.39605152047933245, 43.82633161050914339, -4.148852963258624627 ) ) ;
#64666=LINE ( 'NONE', #95615, #19174 ) ;
#64675=CARTESIAN_POINT ( 'NONE',  ( 66.22087567261847596, 69.35898077670340456, 0.1737556617951544480 ) ) ;
#64676=ORIENTED_EDGE ( 'NONE', *, *, #11475, .F. ) ;
#64682=CYLINDRICAL_SURFACE ( 'NONE', #59774, 10.00000000000001066 ) ;
#64686=CARTESIAN_POINT ( 'NONE',  ( 71.39152386621661606, 62.51010730816707195, -13.96985413412476262 ) ) ;
#64688=CARTESIAN_POINT ( 'NONE',  ( 69.70715393495058265, 66.25057049622556349, -10.63165605719265372 ) ) ;
#64691=CARTESIAN_POINT ( 'NONE',  ( 80.80305022441423546, 43.21727299559393032, -9.912751086834814984 ) ) ;
#64692=CARTESIAN_POINT ( 'NONE',  ( 66.76210968348311781, 68.73313199512115546, 3.352754309929160126 ) ) ;
#64695=CARTESIAN_POINT ( 'NONE',  ( 88.07786909442063461, 44.67132779242000851, -4.228579230841192249 ) ) ;
#64700=B_SPLINE_CURVE_WITH_KNOTS ( 'NONE', 3,
 ( #91563, #91078, #38314, #84472, #44918, #22134, #79256, #83980, #53024, #69223, #84963, #15507, #14545, #45419, #94441, #76354 ),
 .UNSPECIFIED., .F., .F.,
 ( 4, 1, 2, 2, 2, 1, 2, 2, 4 ),
 ( 0.000000000000000000, 0.1249999999999967526, 0.1874999999999966416, 0.2499999999999965583, 0.4999999999999960032, 0.6249999999999975575, 0.6874999999999977796, 0.7499999999999980016, 1.000000000000000000 ),
 .UNSPECIFIED. ) ;
#64701=CARTESIAN_POINT ( 'NONE',  ( 75.31658791476552040, 55.15485285609985766, -16.13722419514472861 ) ) ;
#64703=DIRECTION ( 'NONE',  ( -0.8660254037844379305, -0.5000000000000015543, -0.000000000000000000 ) ) ;
#64708=CARTESIAN_POINT ( 'NONE',  ( 74.60185817734695490, 56.26757446378344696, -16.11404827356958336 ) ) ;
#64709=CARTESIAN_POINT ( 'NONE',  ( 81.20191240145091172, 53.29400499465850771, -15.90005951679047236 ) ) ;
#64715=CARTESIAN_POINT ( 'NONE',  ( 77.07812270435945834, 63.66946605146480209, -15.38604565157081794 ) ) ;
#64718=CARTESIAN_POINT ( 'NONE',  ( 72.49386282319785835, 57.57572440859879492, 15.80166580940835885 ) ) ;
#64723=AXIS2_PLACEMENT_3D ( 'NONE', #13987, #90539, #51482 ) ;
#64724=CARTESIAN_POINT ( 'NONE',  ( 37.50591675755416077, 22.44966523072497111, -2.296566073217252530E-15 ) ) ;
#64728=CARTESIAN_POINT ( 'NONE',  ( 17.84595736030643920, 25.70171378149918340, -9.188101187500004485 ) ) ;
#64734=ORIENTED_EDGE ( 'NONE', *, *, #44332, .F. ) ;
#64737=CARTESIAN_POINT ( 'NONE',  ( 72.50277233665612187, 71.58711300884623085, 5.243368462525016760 ) ) ;
#64739=CARTESIAN_POINT ( 'NONE',  ( 42.14088959202413776, 24.73415679381825782, -6.890680421881970419E-14 ) ) ;
#64741=FACE_OUTER_BOUND ( 'NONE', #6105, .T. ) ;
#64747=CARTESIAN_POINT ( 'NONE',  ( 72.82541052025236183, 57.63392727407249083, -16.30571033187239749 ) ) ;
#64748=ORIENTED_EDGE ( 'NONE', *, *, #26317, .F. ) ;
#64752=CARTESIAN_POINT ( 'NONE',  ( 72.11862359525288468, 71.68643115293319568, 5.491312638656038025 ) ) ;
#64758=CARTESIAN_POINT ( 'NONE',  ( 25.47001115121704373, 36.74646525600391556, 2.839279412974139660 ) ) ;
#64762=ORIENTED_EDGE ( 'NONE', *, *, #89319, .T. ) ;
#64763=ORIENTED_EDGE ( 'NONE', *, *, #92202, .F. ) ;
#64765=CARTESIAN_POINT ( 'NONE',  ( 68.21627857846966947, 65.89183038565549566, 10.81150700775086371 ) ) ;
#64767=CARTESIAN_POINT ( 'NONE',  ( 85.32371827457656366, 48.49939495466653483, 12.43282873216696593 ) ) ;
#64774=CARTESIAN_POINT ( 'NONE',  ( 79.58936028502597537, 59.22294857574252802, 16.56770033466462166 ) ) ;
#64777=CARTESIAN_POINT ( 'NONE',  ( 74.06977354252758516, 55.65288952014064705, -16.58740917872301068 ) ) ;
#64783=CARTESIAN_POINT ( 'NONE',  ( 79.91676478670554218, 44.69584264316313948, -11.20854373491701139 ) ) ;
#64790=ORIENTED_EDGE ( 'NONE', *, *, #91401, .F. ) ;
#64795=CARTESIAN_POINT ( 'NONE',  ( 22.57022264052298155, 36.52903772873359145, -1.583844403245329602 ) ) ;
#64800=CARTESIAN_POINT ( 'NONE',  ( 87.88540012852695327, 44.32205958948441094, 4.765779035299132715 ) ) ;
#64803=CARTESIAN_POINT ( 'NONE',  ( 81.06532563505241740, 46.71245566778327429, 12.32994159712216842 ) ) ;
#64808=LINE ( 'NONE', #55179, #93958 ) ;
#64811=CARTESIAN_POINT ( 'NONE',  ( 85.45558807839536541, 44.20360693575860012, 6.623748629729414361 ) ) ;
#64813=CARTESIAN_POINT ( 'NONE',  ( 78.30955769916529619, 61.43963167811125459, 15.82323565659766018 ) ) ;
#64814=DIRECTION ( 'NONE',  ( -0.8660254037844377084, -0.5000000000000014433, -0.000000000000000000 ) ) ;
#64816=EDGE_CURVE ( 'NONE', #22997, #81391, #75122, .T. ) ;
#64817=CARTESIAN_POINT ( 'NONE',  ( 75.94935831335567400, 63.33535154278327184, -14.87782447488597626 ) ) ;
#64820=CARTESIAN_POINT ( 'NONE',  ( 79.86382474383562169, 55.95619954358613057, 16.50767179695137798 ) ) ;
#64822=CARTESIAN_POINT ( 'NONE',  ( 36.87552185948406702, 26.45404122711136097, -8.090169943749478065 ) ) ;
#64827=CARTESIAN_POINT ( 'NONE',  ( 84.37266873162100467, 43.31764817757444064, -6.019247367396705961 ) ) ;
#64830=FACE_OUTER_BOUND ( 'NONE', #96217, .T. ) ;
#64831=ORIENTED_EDGE ( 'NONE', *, *, #5762, .F. ) ;
#64833=CARTESIAN_POINT ( 'NONE',  ( 86.92045001522136261, 45.99340221249899940, 8.966174604352282529 ) ) ;
#64835=CARTESIAN_POINT ( 'NONE',  ( 71.91251904240313308, 72.63095699448832931, -0.6620033135626105514 ) ) ;
#64839=CARTESIAN_POINT ( 'NONE',  ( 33.00035307926291495, 37.79103043416552055, 8.090169943749478065 ) ) ;
#64843=CARTESIAN_POINT ( 'NONE',  ( 81.38228331512368641, 42.18052851754683275, 8.075145019496556387 ) ) ;
#64857=CARTESIAN_POINT ( 'NONE',  ( 67.38972849331132409, 66.71699885800039453, -8.459198425301941882 ) ) ;
#64862=CARTESIAN_POINT ( 'NONE',  ( 85.33606590682254023, 45.99036976515365183, -10.09305720521511596 ) ) ;
#64863=CARTESIAN_POINT ( 'NONE',  ( 23.73796034364816521, 35.74646525600390845, 2.839279412974139660 ) ) ;
#64868=CARTESIAN_POINT ( 'NONE',  ( 17.58072690530697813, 12.01110640527291373, 2.839279412974134775 ) ) ;
#64871=CARTESIAN_POINT ( 'NONE',  ( 71.67936538144843439, 72.44724869688445779, -1.358217801655851931 ) ) ;
#64872=EDGE_CURVE ( 'NONE', #77711, #3380, #20324, .T. ) ;
#64874=CARTESIAN_POINT ( 'NONE',  ( 72.09555114463066161, 71.52603334931079360, -5.842164467371243397 ) ) ;
#64884=CARTESIAN_POINT ( 'NONE',  ( 37.05984716305037807, 40.13478043621391578, 8.090169943749478065 ) ) ;
#64886=CARTESIAN_POINT ( 'NONE',  ( 72.72170611769777793, 57.01385831347377575, -15.91061902151446183 ) ) ;
#64887=CARTESIAN_POINT ( 'NONE',  ( 78.33567785457334764, 61.58246172053951994, -15.80486485196054858 ) ) ;
#64895=CARTESIAN_POINT ( 'NONE',  ( 30.49295849316677831, 39.64646525600392835, -2.839279412974133887 ) ) ;
#64897=CARTESIAN_POINT ( 'NONE',  ( 78.45009037299155352, 47.91390430630379171, -14.50880498950433761 ) ) ;
#64899=CARTESIAN_POINT ( 'NONE',  ( 74.04232911944542650, 68.62205345152153768, 11.42009053252771800 ) ) ;
#64905=CARTESIAN_POINT ( 'NONE',  ( 83.75393680008980368, 42.85305525622027290, -5.701475753897882193 ) ) ;
#64909=CARTESIAN_POINT ( 'NONE',  ( 67.14771890113766517, 69.04852796021181405, -2.906451251998301011 ) ) ;
#64912=CARTESIAN_POINT ( 'NONE',  ( 78.57703514963246505, 53.48924796936273651, -16.27616477978846277 ) ) ;
#64922=CARTESIAN_POINT ( 'NONE',  ( 84.43795724362087185, 44.16455098980025440, -7.553542188705723248 ) ) ;
#64928=CARTESIAN_POINT ( 'NONE',  ( 76.29477762951383113, 51.62420456488434439, -15.67837010211920301 ) ) ;
#64930=CARTESIAN_POINT ( 'NONE',  ( 80.51866135781378375, 57.13713896268047421, -16.22916027019209650 ) ) ;
#64942=CARTESIAN_POINT ( 'NONE',  ( 17.63446822084836896, 18.38052372038639959, 10.00000000000000533 ) ) ;
#64950=EDGE_CURVE ( 'NONE', #89630, #77668, #96102, .T. ) ;
#64951=CARTESIAN_POINT ( 'NONE',  ( 81.07596274759146127, 51.75087684323265336, -15.00964593992177676 ) ) ;
#64954=CARTESIAN_POINT ( 'NONE',  ( 66.74069431502459793, 67.35994133444863508, -6.833594717235060401 ) ) ;
#64959=CARTESIAN_POINT ( 'NONE',  ( 13.51707852204697069, 30.73705186507753240, -3.090169943749475845 ) ) ;
#64964=CARTESIAN_POINT ( 'NONE',  ( 73.74547311384563386, 55.26076647750536353, -16.59506521500572518 ) ) ;
#64975=CARTESIAN_POINT ( 'NONE',  ( 35.16646543599519248, 35.70171378149922248, -9.188101187500004485 ) ) ;
#64978=CARTESIAN_POINT ( 'NONE',  ( 30.58134869734400851, 35.84336893147758474, -7.433330006724137462 ) ) ;
#64982=CARTESIAN_POINT ( 'NONE',  ( 34.30168821287347924, 42.73705186507756792, -3.090169943749475845 ) ) ;
#64984=CARTESIAN_POINT ( 'NONE',  ( 10.98031343905817714, 14.84335787977761001, 9.188101187500006262 ) ) ;
#64986=CARTESIAN_POINT ( 'NONE',  ( 18.92609651878039756, 19.43085787977762635, -9.188101187500008038 ) ) ;
#64988=FACE_OUTER_BOUND ( 'NONE', #49318, .T. ) ;
#64996=CARTESIAN_POINT ( 'NONE',  ( 74.14312167556930433, 66.30466486950707861, 1.224646799147354045E-15 ) ) ;
#64997=CARTESIAN_POINT ( 'NONE',  ( 87.49951909536234496, 45.04593868083597386, 6.937257679092502904 ) ) ;
#65002=CARTESIAN_POINT ( 'NONE',  ( 86.20802731503823679, 47.17721747253784770, 10.82151197958144273 ) ) ;
#65004=CARTESIAN_POINT ( 'NONE',  ( 77.00607721352450596, 53.74328018355883074, 15.98262156706233306 ) ) ;
#65006=VERTEX_POINT ( 'NONE', #1100 ) ;
#65008=CARTESIAN_POINT ( 'NONE',  ( 88.54549197286583251, 43.89854493182281203, -0.2370037879772138034 ) ) ;
#65010=CARTESIAN_POINT ( 'NONE',  ( 17.63446822084836896, 18.38052372038639959, 10.00000000000000533 ) ) ;
#65014=CARTESIAN_POINT ( 'NONE',  ( 81.89485588203808675, 55.22971306509116829, 16.24120679747551677 ) ) ;
#65025=CARTESIAN_POINT ( 'NONE',  ( 71.69220090349242014, 69.88970279385412709, 7.579357904728459161 ) ) ;
#65032=CARTESIAN_POINT ( 'NONE',  ( 20.82173017108080515, 32.99752408145591431, 5.678558825948277544 ) ) ;
#65046=LINE ( 'NONE', #66537, #54398 ) ;
#65056=ORIENTED_EDGE ( 'NONE', *, *, #79289, .F. ) ;
#65058=CARTESIAN_POINT ( 'NONE',  ( 67.41639658691251213, 69.05313671411084897, 3.556105138604360061 ) ) ;
#65059=CARTESIAN_POINT ( 'NONE',  ( 82.67950799182933963, 41.89762085301913430, 4.838269528849628465 ) ) ;
#65063=FACE_OUTER_BOUND ( 'NONE', #42947, .T. ) ;
#65066=ORIENTED_EDGE ( 'NONE', *, *, #69955, .T. ) ;
#65067=CARTESIAN_POINT ( 'NONE',  ( 83.95052478757145309, 47.16512906835476571, 11.42333699328953145 ) ) ;
#65072=CARTESIAN_POINT ( 'NONE',  ( 68.51023738315195999, 64.28149084335623797, -12.38465469846545730 ) ) ;
#65074=PLANE ( 'NONE',  #59681 ) ;
#65076=CARTESIAN_POINT ( 'NONE',  ( 69.54491560247440418, 68.33319813537798382, -8.868170946166037183 ) ) ;
#65082=CARTESIAN_POINT ( 'NONE',  ( 85.09877614057847950, 47.61067639237452909, 11.82617649972324259 ) ) ;
#65084=CARTESIAN_POINT ( 'NONE',  ( 21.69737781089059681, 21.03085787977762777, 9.188101187500006262 ) ) ;
#65085=CARTESIAN_POINT ( 'NONE',  ( 74.92881689719639837, 67.14644430943499742, 12.99852016367277052 ) ) ;
#65089=CARTESIAN_POINT ( 'NONE',  ( 11.95823279523498073, 29.83705186507753027, 3.090169943749475401 ) ) ;
#65095=CARTESIAN_POINT ( 'NONE',  ( 81.39533252797791363, 55.41833949407015325, -16.32393128051840137 ) ) ;
#65097=CARTESIAN_POINT ( 'NONE',  ( 69.93689855390263688, 65.90667941659796725, -11.72867282680260281 ) ) ;
#65099=B_SPLINE_CURVE_WITH_KNOTS ( 'NONE', 3,
 ( #93265, #23319, #53232, #69430, #76545, #70429, #54207, #68921, #77550, #61814, #99847, #53714, #62821, #23820, #93777, #86194 ),
 .UNSPECIFIED., .F., .F.,
 ( 4, 1, 2, 2, 2, 1, 2, 2, 4 ),
 ( 0.000000000000000000, 0.1250000000000020539, 0.1875000000000021927, 0.2500000000000023315, 0.5000000000000027756, 0.6250000000000039968, 0.6875000000000046629, 0.7500000000000052180, 1.000000000000000000 ),
 .UNSPECIFIED. ) ;
#65102=CARTESIAN_POINT ( 'NONE',  ( 72.13526286807632459, 72.32911410822552511, 1.080822308860484027 ) ) ;
#65104=B_SPLINE_CURVE_WITH_KNOTS ( 'NONE', 3,
 ( #54368, #92924, #31083, #14411, #68100, #5806, #99518, #6803, #45777, #61971, #36691, #22985, #85341, #99021, #53391, #7802, #59987, #69091, #76699, #77195, #98530, #68595, #22500, #100017, #30602, #38687, #75722, #21999, #46272, #23477, #7292, #15886, #38173, #29607, #61488, #67600, #92438, #46798, #69591, #30102, #91949, #52398, #90957, #29120, #21513, #37683 ),
 .UNSPECIFIED., .F., .F.,
 ( 4, 1, 2, 2, 1, 2, 2, 1, 1, 2, 2, 1, 1, 2, 2, 1, 1, 2, 2, 1, 1, 1, 2, 2, 1, 1, 1, 2, 2, 4 ),
 ( 0.000000000000000000, 0.06249999999999931999, 0.09374999999999898692, 0.1249999999999986677, 0.1875000000000011935, 0.2187500000000009437, 0.2500000000000007216, 0.3125000000000002776, 0.3437500000000017208, 0.3593750000000022204, 0.3750000000000026645, 0.4375000000000003886, 0.4687499999999992784, 0.4843749999999972244, 0.4999999999999951150, 0.5624999999999961142, 0.5937499999999952260, 0.6093749999999964473, 0.6249999999999977796, 0.6874999999999930056, 0.7187499999999892308, 0.7343749999999890088, 0.7421874999999888978, 0.7499999999999888978, 0.8124999999999964473, 0.8437499999999985567, 0.8593749999999996669, 0.8671874999999986677, 0.8749999999999976685, 1.000000000000000000 ),
 .UNSPECIFIED. ) ;
#65105=CARTESIAN_POINT ( 'NONE',  ( 80.48032370448046890, 56.76188079953907106, 16.17739337235778052 ) ) ;
#65111=CARTESIAN_POINT ( 'NONE',  ( 5.036790953515181357, 27.00034080476288523, -1.878358725466461243E-16 ) ) ;
#65113=VERTEX_POINT ( 'NONE', #29878 ) ;
#65114=CARTESIAN_POINT ( 'NONE',  ( 77.80736617348490824, 61.72758938687779562, 16.06622420362089798 ) ) ;
#65118=CARTESIAN_POINT ( 'NONE',  ( 78.73521911786851035, 59.96578626319077188, 16.11589682977616533 ) ) ;
#65123=CARTESIAN_POINT ( 'NONE',  ( 79.14797540978585744, 51.65882171989947125, -15.32139210428527321 ) ) ;
#65124=CARTESIAN_POINT ( 'NONE',  ( 81.40142225033505952, 41.96015433569891684, -7.703957233619936673 ) ) ;
#65130=VERTEX_POINT ( 'NONE', #90737 ) ;
#65132=CARTESIAN_POINT ( 'NONE',  ( 74.67627071976463071, 57.26912010096364725, 16.03321057786944692 ) ) ;
#65142=DIRECTION ( 'NONE',  ( -0.3213938048432640748, 0.5566703992264119272, -0.7660444431189857850 ) ) ;
#65146=CARTESIAN_POINT ( 'NONE',  ( 40.90268743793880901, 35.56628583063844218, 9.188101187500006262 ) ) ;
#65151=CARTESIAN_POINT ( 'NONE',  ( 78.28406713961415164, 47.42774444821681357, -13.76474501704126929 ) ) ;
#65152=CARTESIAN_POINT ( 'NONE',  ( 76.28172291344246503, 65.04177861043513076, -14.25052431483989324 ) ) ;
#65154=CARTESIAN_POINT ( 'NONE',  ( 70.91684448083535131, 60.93905801807242995, 14.54788300031792936 ) ) ;
#65157=CARTESIAN_POINT ( 'NONE',  ( 88.22170401875577284, 44.22125859644826562, -1.816381297913363779 ) ) ;
#65160=CARTESIAN_POINT ( 'NONE',  ( 66.01181605970899113, 68.68997318219119563, -0.06151385425865887879 ) ) ;
#65174=CARTESIAN_POINT ( 'NONE',  ( 73.45240594507248488, 61.98306700939508573, -14.75352172543200524 ) ) ;
#65176=ADVANCED_FACE ( 'NONE', ( #27883 ), #14245, .T. ) ;
#65178=CARTESIAN_POINT ( 'NONE',  ( 74.69145432289207065, 65.16111103690977302, -13.69219638301821185 ) ) ;
#65180=CARTESIAN_POINT ( 'NONE',  ( 80.78722682204974603, 43.18815817188708195, -9.889478511952381368 ) ) ;
#65186=CARTESIAN_POINT ( 'NONE',  ( 88.05624235485146301, 44.55787864911080476, -5.145732200269209855 ) ) ;
#65191=CARTESIAN_POINT ( 'NONE',  ( 75.84856439504059722, 51.76521084193598909, 15.76359423700355755 ) ) ;
#65200=CARTESIAN_POINT ( 'NONE',  ( 80.10468490011123777, 54.30569091379602753, -15.86741517739214125 ) ) ;
#65201=CARTESIAN_POINT ( 'NONE',  ( 79.40524497836292994, 46.23731968723249253, -13.25138998636449372 ) ) ;
#65206=CARTESIAN_POINT ( 'NONE',  ( 72.57191691350548979, 57.24899938748259132, 15.86174820108270112 ) ) ;
#65211=CARTESIAN_POINT ( 'NONE',  ( 35.02453322635827249, 23.14754757982092315, -5.678558825948275768 ) ) ;
#65212=CARTESIAN_POINT ( 'NONE',  ( 80.75896084256157792, 48.90990202073309945, -14.35679662723407368 ) ) ;
#65213=CARTESIAN_POINT ( 'NONE',  ( 84.99894282664955369, 46.71838944095585333, -10.45175089821682413 ) ) ;
#65214=ORIENTED_EDGE ( 'NONE', *, *, #80679, .T. ) ;
#65215=CARTESIAN_POINT ( 'NONE',  ( 15.95033727479334651, 30.18502408145591787, 5.678558825948277544 ) ) ;
#65221=CARTESIAN_POINT ( 'NONE',  ( 86.10128179547638183, 47.01522930412664181, 10.71950609365847384 ) ) ;
#65226=CARTESIAN_POINT ( 'NONE',  ( 74.85635044626891954, 53.33667049677163874, 16.05360532518207606 ) ) ;
#65233=CARTESIAN_POINT ( 'NONE',  ( 77.23930090163744921, 62.99565350650583895, -15.27869716933193445 ) ) ;
#65235=CARTESIAN_POINT ( 'NONE',  ( 72.24104924332462474, 71.74196171561413848, 5.528620549063430367 ) ) ;
#65239=ORIENTED_EDGE ( 'NONE', *, *, #42377, .F. ) ;
#65241=CARTESIAN_POINT ( 'NONE',  ( 30.18562306610639112, 29.37878583063842441, 9.188101187500006262 ) ) ;
#65244=EDGE_CURVE ( 'NONE', #21644, #67514, #46558, .T. ) ;
#65251=CARTESIAN_POINT ( 'NONE',  ( 85.76586952047404111, 48.61475482067446308, -11.85709152719317139 ) ) ;
#65255=DIRECTION ( 'NONE',  ( 0.5000000000000014433, -0.8660254037844378194, 0.000000000000000000 ) ) ;
#65262=CARTESIAN_POINT ( 'NONE',  ( 73.83780735420440067, 55.05980088889993596, -16.60220836681794054 ) ) ;
#65267=CARTESIAN_POINT ( 'NONE',  ( 87.17617632782311432, 45.93339551703158463, -8.679440343565334004 ) ) ;
#65270=CARTESIAN_POINT ( 'NONE',  ( 84.83489698312170901, 42.27858766766668452, -0.5892840222501907199 ) ) ;
#65277=ORIENTED_EDGE ( 'NONE', *, *, #47881, .F. ) ;
#65281=CARTESIAN_POINT ( 'NONE',  ( 23.18815102787819171, 35.16126292948896293, -6.180339887498951690 ) ) ;
#65283=CARTESIAN_POINT ( 'NONE',  ( 68.87368469670209947, 69.23618240007901647, -5.598517026418342368 ) ) ;
#65285=CARTESIAN_POINT ( 'NONE',  ( 69.66171794495750191, 62.30057999729555718, -13.54004527842230488 ) ) ;
#65288=EDGE_LOOP ( 'NONE', ( #86492, #14394, #50346, #3365 ) ) ;
#65289=B_SPLINE_CURVE_WITH_KNOTS ( 'NONE', 3,
 ( #13074, #36341, #99159, #53532, #76365, #21653, #20661, #90604, #30244, #15025, #60619, #6937, #6455, #29747, #68735, #83486, #75877, #37333, #14052, #45917, #61125, #98173, #13566, #67243, #44437, #5950, #98676, #21170, #82989, #68236, #91574, #51550, #76835, #22146, #7433, #22647, #38326, #69233, #100163, #30749, #82512, #74874, #5457, #48443, #93062, #55026 ),
 .UNSPECIFIED., .F., .F.,
 ( 4, 1, 2, 2, 1, 2, 2, 1, 1, 2, 2, 1, 1, 2, 2, 1, 1, 2, 2, 1, 1, 1, 2, 2, 1, 1, 1, 2, 2, 4 ),
 ( 0.000000000000000000, 0.06249999999999364397, 0.09374999999999052147, 0.1249999999999873990, 0.1874999999999764910, 0.2187499999999706346, 0.2499999999999647504, 0.3124999999999538147, 0.3437499999999505951, 0.3593749999999505396, 0.3749999999999504285, 0.4374999999999527600, 0.4687499999999538702, 0.4843749999999560352, 0.4999999999999581446, 0.5624999999999705791, 0.5937499999999786837, 0.6093749999999810152, 0.6249999999999832356, 0.6874999999999926725, 0.7187499999999995559, 0.7343750000000008882, 0.7421875000000018874, 0.7500000000000028866, 0.8125000000000117684, 0.8437500000000146549, 0.8593750000000178746, 0.8671875000000195399, 0.8750000000000210942, 1.000000000000000000 ),
 .UNSPECIFIED. ) ;
#65292=EDGE_CURVE ( 'NONE', #49291, #63028, #81474, .T. ) ;
#65293=CARTESIAN_POINT ( 'NONE',  ( 82.75024023773026727, 40.61788017064008471, -1.390363622740588223 ) ) ;
#65299=EDGE_CURVE ( 'NONE', #44213, #66291, #37164, .T. ) ;
#65300=CARTESIAN_POINT ( 'NONE',  ( 80.89006754182553038, 55.13283443129127193, 15.96266433881070945 ) ) ;
#65301=CARTESIAN_POINT ( 'NONE',  ( 66.59659379507385779, 69.02878726636450324, -0.1500247100265385269 ) ) ;
#65303=CARTESIAN_POINT ( 'NONE',  ( 83.38047668388445288, 51.78471284047383705, 14.96842148903410497 ) ) ;
#65306=EDGE_CURVE ( 'NONE', #50951, #17891, #1601, .T. ) ;
#65307=CARTESIAN_POINT ( 'NONE',  ( 71.28050843997250752, 64.71893044897940683, -12.66255568095732897 ) ) ;
#65312=CARTESIAN_POINT ( 'NONE',  ( 35.64779661956466583, 28.78052372038643369, -10.00000000000000355 ) ) ;
#65317=CARTESIAN_POINT ( 'NONE',  ( 86.28849223104248267, 43.59502242935581506, -3.924905614730060499 ) ) ;
#65320=CARTESIAN_POINT ( 'NONE',  ( 83.11190622883978563, 51.97173441866404886, 14.72729092114622063 ) ) ;
#65323=CARTESIAN_POINT ( 'NONE',  ( 86.63801457440831655, 46.38311672867401114, 9.077114030922938781 ) ) ;
#65325=FACE_OUTER_BOUND ( 'NONE', #11639, .T. ) ;
#65327=CARTESIAN_POINT ( 'NONE',  ( 87.01945182987638816, 46.04471723482853918, 8.958281803387862396 ) ) ;
#65329=CARTESIAN_POINT ( 'NONE',  ( 37.17256469204938440, 37.16454794089044356, -10.00000000000000355 ) ) ;
#65333=CARTESIAN_POINT ( 'NONE',  ( 81.34546223144695887, 42.12293715088343760, 8.018599761840913942 ) ) ;
#65335=CARTESIAN_POINT ( 'NONE',  ( 87.11953417171658032, 46.01840446382728800, -8.187078523733017477 ) ) ;
#65337=CARTESIAN_POINT ( 'NONE',  ( 87.63003801413758254, 45.43815880539863628, -6.688036734344514400 ) ) ;
#65339=CARTESIAN_POINT ( 'NONE',  ( 74.90746300446748762, 65.80853403655308398, -13.37832520640001910 ) ) ;
#65345=CARTESIAN_POINT ( 'NONE',  ( 67.25058181848319805, 66.49012357423811181, -8.666073719759312510 ) ) ;
#65346=ORIENTED_EDGE ( 'NONE', *, *, #91412, .T. ) ;
#65350=CARTESIAN_POINT ( 'NONE',  ( 25.85549604718420014, 26.87878583063842797, -9.188101187500006262 ) ) ;
#65352=CARTESIAN_POINT ( 'NONE',  ( 86.53352045429423356, 47.35036163402705967, -10.26701049652133513 ) ) ;
#65355=CARTESIAN_POINT ( 'NONE',  ( 13.17245041747802148, 29.64646525600389637, -2.839279412974133887 ) ) ;
#65369=ORIENTED_EDGE ( 'NONE', *, *, #58243, .F. ) ;
#65373=CARTESIAN_POINT ( 'NONE',  ( 78.08206365161463225, 61.83366292688850052, -15.70979438352861379 ) ) ;
#65381=CARTESIAN_POINT ( 'NONE',  ( 32.39821438149254362, 40.74646525600392977, 2.839279412974139660 ) ) ;
#65383=CARTESIAN_POINT ( 'NONE',  ( 78.19930204122441353, 47.67057537844316784, -14.46097917792036647 ) ) ;
#65391=ORIENTED_EDGE ( 'NONE', *, *, #98351, .F. ) ;
#65392=AXIS2_PLACEMENT_3D ( 'NONE', #409, #17097, #47995 ) ;
#65394=CARTESIAN_POINT ( 'NONE',  ( 87.42296356251033274, 43.77044090453171776, -1.503769482561249538 ) ) ;
#65399=DIRECTION ( 'NONE',  ( 0.5000000000000013323, -0.8660254037844378194, 0.000000000000000000 ) ) ;
#65409=ORIENTED_EDGE ( 'NONE', *, *, #32108, .T. ) ;
#65410=CARTESIAN_POINT ( 'NONE',  ( 86.75859043018910199, 44.26021819578813421, -5.163563606523318583 ) ) ;
#65415=CARTESIAN_POINT ( 'NONE',  ( 75.37392722170159232, 64.45239491791643616, 14.26364343640139332 ) ) ;
#65421=CYLINDRICAL_SURFACE ( 'NONE', #95339, 10.00000000000001066 ) ;
#65429=CARTESIAN_POINT ( 'NONE',  ( 22.49950015666239622, 18.15404122711133539, 8.090169943749479842 ) ) ;
#65443=CARTESIAN_POINT ( 'NONE',  ( 15.67984500357415278, 27.79103043416548502, 8.090169943749478065 ) ) ;
#65444=CARTESIAN_POINT ( 'NONE',  ( 88.19107160583139660, 43.69314304319705400, 0.1842422985582093387 ) ) ;
#65446=CARTESIAN_POINT ( 'NONE',  ( 72.23440922827423094, 71.91206544914358290, -3.821601542290089970 ) ) ;
#65448=CARTESIAN_POINT ( 'NONE',  ( 73.77371296639375942, 55.45649524975051037, -16.58834881926898674 ) ) ;
#65451=CARTESIAN_POINT ( 'NONE',  ( 76.30616544034060666, 50.97262258187969763, -15.53540872755634439 ) ) ;
#65452=CARTESIAN_POINT ( 'NONE',  ( 29.18428119120667574, 28.80066082961423390, 10.00000000000000533 ) ) ;
#65461=CARTESIAN_POINT ( 'NONE',  ( 36.24660459446916150, 29.43085787977765833, -9.188101187500008038 ) ) ;
#65465=CARTESIAN_POINT ( 'NONE',  ( 29.46033357383057449, 37.98502408145594700, -5.678558825948271327 ) ) ;
#65472=CARTESIAN_POINT ( 'NONE',  ( 5.869580825389008716, 26.49540643055185996, 3.479690158560446702E-15 ) ) ;
#65474=CARTESIAN_POINT ( 'NONE',  ( 13.87187630571069086, 28.98502408145591502, -5.678558825948271327 ) ) ;
#65476=CARTESIAN_POINT ( 'NONE',  ( 67.86860378221429357, 65.58690806574966814, -10.91583492536020294 ) ) ;
#65477=VERTEX_POINT ( 'NONE', #62633 ) ;
#65482=CARTESIAN_POINT ( 'NONE',  ( 29.26302659224649361, 17.86426979415090699, -3.090169943749474069 ) ) ;
#65483=CARTESIAN_POINT ( 'NONE',  ( 87.64408659938918333, 45.45982483689996911, 6.724836266884324232 ) ) ;
#65490=CARTESIAN_POINT ( 'NONE',  ( 76.79044849124564109, 52.81680254209042857, 15.85812468158750654 ) ) ;
#65494=CARTESIAN_POINT ( 'NONE',  ( 76.30616544034060666, 50.97262258187969763, -15.53540872755634439 ) ) ;
#65500=CARTESIAN_POINT ( 'NONE',  ( 73.26674808670287575, 57.93223743048974939, 15.81806325431525373 ) ) ;
#65504=ORIENTED_EDGE ( 'NONE', *, *, #61885, .F. ) ;
#65506=CARTESIAN_POINT ( 'NONE',  ( 46.74164954608104239, 27.39040679176987325, -6.890680421881970419E-14 ) ) ;
#65510=EDGE_LOOP ( 'NONE', ( #46566, #59271, #39414, #95685 ) ) ;
#65514=CARTESIAN_POINT ( 'NONE',  ( 69.93400769858298816, 66.24381931584940730, 10.75078203157522161 ) ) ;
#65516=CARTESIAN_POINT ( 'NONE',  ( 86.41859815849130655, 43.12384784049413611, 0.4076689040990972845 ) ) ;
#65518=EDGE_LOOP ( 'NONE', ( #98143, #89968 ) ) ;
#65520=CARTESIAN_POINT ( 'NONE',  ( 20.10065364775352847, 33.64646525600390703, -2.839279412974133887 ) ) ;
#65528=CARTESIAN_POINT ( 'NONE',  ( 37.67689025969888661, 40.49103043416553049, -8.090169943749479842 ) ) ;
#65533=EDGE_LOOP ( 'NONE', ( #12491, #47715, #67494, #73840 ) ) ;
#65549=EDGE_LOOP ( 'NONE', ( #32964, #29736, #5351, #60754 ) ) ;
#65551=CARTESIAN_POINT ( 'NONE',  ( 87.91539880103944427, 43.93416759974002872, 0.4624922486833659696 ) ) ;
#65552=CARTESIAN_POINT ( 'NONE',  ( 76.05733463510750880, 51.21219284135379013, 16.11160009721543318 ) ) ;
#65554=CARTESIAN_POINT ( 'NONE',  ( 3.562051267137642085, 25.55466486950697558, -1.111400068045478839E-16 ) ) ;
#65557=CARTESIAN_POINT ( 'NONE',  ( 73.92441827737660276, 68.29833774401778612, -11.64939612493447996 ) ) ;
#65560=ORIENTED_EDGE ( 'NONE', *, *, #16226, .F. ) ;
#65561=CARTESIAN_POINT ( 'NONE',  ( 79.09474592215634914, 60.19097512726884958, -16.45688605998253706 ) ) ;
#65565=VECTOR ( 'NONE', #16558, 1000.000000000000000 ) ;
#65567=CARTESIAN_POINT ( 'NONE',  ( 68.71080560055042952, 64.06082602079280264, -12.00658928456073227 ) ) ;
#65568=CARTESIAN_POINT ( 'NONE',  ( 73.49832466283049826, 68.39562707634591732, -11.34410690473859873 ) ) ;
#65573=CARTESIAN_POINT ( 'NONE',  ( 71.85869513609316073, 58.67586711399008692, -15.48493562761569287 ) ) ;
#65575=ORIENTED_EDGE ( 'NONE', *, *, #96063, .T. ) ;
#65580=CARTESIAN_POINT ( 'NONE',  ( 14.99289142922413021, 26.84336893147755276, -7.433330006724137462 ) ) ;
#65581=CARTESIAN_POINT ( 'NONE',  ( 74.78994931159289195, 67.11760897871008069, 12.96302903502454029 ) ) ;
#65585=DIRECTION ( 'NONE',  ( -0.8660254037844379305, -0.5000000000000014433, -0.000000000000000000 ) ) ;
#65591=CARTESIAN_POINT ( 'NONE',  ( 81.49556199178041993, 55.44509743070403118, -16.31886845347543513 ) ) ;
#65593=CARTESIAN_POINT ( 'NONE',  ( 73.95900928047775835, 65.06227567762803687, -13.94751918840041505 ) ) ;
#65595=CARTESIAN_POINT ( 'NONE',  ( 82.99478726538977469, 41.85582147743899384, 4.139490622842754597 ) ) ;
#65596=CARTESIAN_POINT ( 'NONE',  ( 80.41751025656814988, 56.26485224411339203, 16.12594336028984543 ) ) ;
#65599=CARTESIAN_POINT ( 'NONE',  ( 72.35257617177605027, 71.70739429922333841, -5.765621772327581773 ) ) ;
#65602=CARTESIAN_POINT ( 'NONE',  ( 12.53791098520745173, 8.208019796199266693, -3.090169943749474069 ) ) ;
#65604=ORIENTED_EDGE ( 'NONE', *, *, #46516, .F. ) ;
#65610=CARTESIAN_POINT ( 'NONE',  ( 78.70340902619774681, 59.85553566278375115, 16.12483691164164412 ) ) ;
#65615=CARTESIAN_POINT ( 'NONE',  ( 81.10660686981061929, 51.01353853940796768, -14.74231750527668261 ) ) ;
#65616=CARTESIAN_POINT ( 'NONE',  ( 84.60739412327551179, 49.90025452092439906, -13.66407646797534703 ) ) ;
#65619=EDGE_CURVE ( 'NONE', #37182, #19430, #64666, .T. ) ;
#65634=CARTESIAN_POINT ( 'NONE',  ( 87.34642337659644795, 43.20430561321286689, -4.696387144280492735E-07 ) ) ;
#65638=CARTESIAN_POINT ( 'NONE',  ( 75.67231652922859553, 54.75346391114741351, 16.12193936410828599 ) ) ;
#65639=CARTESIAN_POINT ( 'NONE',  ( 9.471979480098337234, 23.65586893147754566, -7.433330006724137462 ) ) ;
#65643=VERTEX_POINT ( 'NONE', #68012 ) ;
#65650=CARTESIAN_POINT ( 'NONE',  ( 87.63119364650854948, 45.29408460765224476, 6.394950601605615681 ) ) ;
#65661=CARTESIAN_POINT ( 'NONE',  ( 88.48118267945454818, 44.00993189541001271, 2.076335272536708576 ) ) ;
#65666=CARTESIAN_POINT ( 'NONE',  ( 74.23294069390520633, 67.58675612407668609, 12.40011470933238158 ) ) ;
#65668=CARTESIAN_POINT ( 'NONE',  ( 71.88039266631933799, 65.91489085601192244, -12.06854722625687337 ) ) ;
#65671=CARTESIAN_POINT ( 'NONE',  ( 80.87585157758311993, 42.95980323379527732, -9.554274543293205468 ) ) ;
#65676=CARTESIAN_POINT ( 'NONE',  ( 87.96405694255219032, 44.24133552746449283, -4.384643187820149279 ) ) ;
#65678=CARTESIAN_POINT ( 'NONE',  ( 77.55626133878482165, 49.73613333205595666, 14.95107568548285037 ) ) ;
#65680=CARTESIAN_POINT ( 'NONE',  ( 77.25846549316018752, 51.17059816455404331, 15.45812498229560639 ) ) ;
#65684=CARTESIAN_POINT ( 'NONE',  ( 84.37450382530433046, 50.67865889666357759, 13.77848111769147366 ) ) ;
#65690=EDGE_CURVE ( 'NONE', #13530, #86376, #74079, .T. ) ;
#65693=CARTESIAN_POINT ( 'NONE',  ( 78.61816319214723592, 52.61787231995300829, -16.10833693956800161 ) ) ;
#65699=CARTESIAN_POINT ( 'NONE',  ( 33.90351810284484202, 25.28920272979928896, -7.433330006724141015 ) ) ;
#65700=CARTESIAN_POINT ( 'NONE',  ( 86.32721218574307898, 47.55264674982593931, -11.12316258729871699 ) ) ;
#65701=CARTESIAN_POINT ( 'NONE',  ( 75.51649238510275097, 60.77114109127464303, 15.98312560776951230 ) ) ;
#65703=CARTESIAN_POINT ( 'NONE',  ( 16.11390655273756778, 24.70171378149918340, -9.188101187500004485 ) ) ;
#65704=CARTESIAN_POINT ( 'NONE',  ( 5.294102074706517058, 26.55466486950697558, -1.111400068045478839E-16 ) ) ;
#65708=CARTESIAN_POINT ( 'NONE',  ( 86.20802731503823679, 47.17721747253784770, 10.82151197958144273 ) ) ;
#65713=CARTESIAN_POINT ( 'NONE',  ( 74.75954543159157595, 53.46422244337664864, 16.07001580372355320 ) ) ;
#65721=ORIENTED_EDGE ( 'NONE', *, *, #9051, .F. ) ;
#65722=CARTESIAN_POINT ( 'NONE',  ( 71.95473880081605955, 71.54457537667215661, 5.606738443688809248 ) ) ;
#65725=CARTESIAN_POINT ( 'NONE',  ( 87.91725590613566510, 44.21674671100767284, -4.392329086374231473 ) ) ;
#65727=CARTESIAN_POINT ( 'NONE',  ( 46.41032958717836010, 27.76426979415094110, 3.090169943749476733 ) ) ;
#65728=CARTESIAN_POINT ( 'NONE',  ( 30.33837380989695731, 32.91421378149920685, 9.188101187500008038 ) ) ;
#65730=CARTESIAN_POINT ( 'NONE',  ( 79.06023636259786258, 58.49762800437630972, -16.20933576862745440 ) ) ;
#65740=CARTESIAN_POINT ( 'NONE',  ( 85.91498916281075537, 48.46192805135255099, 12.13455285288522667 ) ) ;
#65741=CARTESIAN_POINT ( 'NONE',  ( 66.54075137518580618, 68.81555626029071959, -2.231460399992863497 ) ) ;
#65748=CARTESIAN_POINT ( 'NONE',  ( 78.88256717313477395, 59.65579592159198086, 16.50129574805685806 ) ) ;
#65751=CARTESIAN_POINT ( 'NONE',  ( 73.82455155085514775, 55.55241100957154288, -16.58550341923981719 ) ) ;
#65755=ORIENTED_EDGE ( 'NONE', *, *, #70780, .F. ) ;
#65756=CARTESIAN_POINT ( 'NONE',  ( 87.22262286821016630, 46.01322853962243897, -8.753954545221112937 ) ) ;
#65759=CARTESIAN_POINT ( 'NONE',  ( 14.17036660571061368, 16.38052372038639604, 10.00000000000000533 ) ) ;
#65767=CARTESIAN_POINT ( 'NONE',  ( 29.68521398013932711, 18.10801979619930080, 3.090169943749476733 ) ) ;
#65771=CARTESIAN_POINT ( 'NONE',  ( 69.59872347107847190, 62.52290715608992144, -13.38904497502296920 ) ) ;
#65772=CARTESIAN_POINT ( 'NONE',  ( 72.26191451101281871, 71.91445694603925176, -5.118044210176695863 ) ) ;
#65777=CARTESIAN_POINT ( 'NONE',  ( 81.60462840567272735, 48.29055636627209225, 13.20316565662312236 ) ) ;
#65778=CARTESIAN_POINT ( 'NONE',  ( 82.17911912404201757, 40.65326309479461742, -3.506590647633029523 ) ) ;
#65782=DIRECTION ( 'NONE',  ( 0.000000000000000000, -1.000000000000000000, 1.060575238724906175E-16 ) ) ;
#65785=CARTESIAN_POINT ( 'NONE',  ( 80.78458207904813548, 54.24769972901211190, 15.79515950411193259 ) ) ;
#65786=CARTESIAN_POINT ( 'NONE',  ( 67.13575020204197585, 69.32447942518001582, -0.8057866954429201423 ) ) ;
#65788=CARTESIAN_POINT ( 'NONE',  ( 78.31539865234907438, 61.49392785109991166, 15.81390201164141196 ) ) ;
#65793=CARTESIAN_POINT ( 'NONE',  ( 74.17947873915457535, 55.31082063550417161, 16.12337822475624094 ) ) ;
#65794=CARTESIAN_POINT ( 'NONE',  ( 78.38478726132005647, 48.59772224786558326, 14.85394671703156178 ) ) ;
#65796=CARTESIAN_POINT ( 'NONE',  ( 34.30385554556135475, 35.50829794293883168, -10.00000000000000355 ) ) ;
#65798=CARTESIAN_POINT ( 'NONE',  ( 71.60534465744318311, 58.98582914060868632, -15.35957662280589275 ) ) ;
#65800=CARTESIAN_POINT ( 'NONE',  ( 81.50613923611670941, 43.19572371951541356, -8.552294727196889212 ) ) ;
#65805=CARTESIAN_POINT ( 'NONE',  ( 87.01945182987638816, 46.04471723482853918, 8.958281803387862396 ) ) ;
#65807=CARTESIAN_POINT ( 'NONE',  ( 82.03128457439912324, 41.77525573450511587, 5.434104432741746926 ) ) ;
#65811=CARTESIAN_POINT ( 'NONE',  ( 33.88626221353634804, 43.65659080271453973, -1.878358725466461243E-16 ) ) ;
#65815=CARTESIAN_POINT ( 'NONE',  ( 71.96486598315394190, 67.72978614143600851, -10.50385197199905285 ) ) ;
#65822=CARTESIAN_POINT ( 'NONE',  ( 31.26830227169403997, 36.79103043416551344, 8.090169943749478065 ) ) ;
#65828=CARTESIAN_POINT ( 'NONE',  ( 67.54350597765656516, 66.80466261606197520, -8.460816904384278914 ) ) ;
#65833=CARTESIAN_POINT ( 'NONE',  ( 27.91350267930052809, 31.51421378149921182, -9.188101187500004485 ) ) ;
#65835=CARTESIAN_POINT ( 'NONE',  ( 86.53753835918318771, 47.29678250252424476, -10.20988859552574013 ) ) ;
#65836=VECTOR ( 'NONE', #54957, 1000.000000000000114 ) ;
#65840=CARTESIAN_POINT ( 'NONE',  ( 16.86928618479235809, 18.24335787977762280, -9.188101187500008038 ) ) ;
#65841=CARTESIAN_POINT ( 'NONE',  ( 76.46509270602138031, 63.14577049208008930, 15.06850016415780935 ) ) ;
#65851=EDGE_CURVE ( 'NONE', #86376, #57995, #98316, .T. ) ;
#65858=CARTESIAN_POINT ( 'NONE',  ( 66.25519791831798955, 69.22521726602100500, -2.104850759282526962 ) ) ;
#65861=FACE_OUTER_BOUND ( 'NONE', #37211, .T. ) ;
#65871=VERTEX_POINT ( 'NONE', #27244 ) ;
#65873=CARTESIAN_POINT ( 'NONE',  ( 31.91767387367526609, 30.37878583063843152, 9.188101187500006262 ) ) ;
#65875=CARTESIAN_POINT ( 'NONE',  ( 75.27358033784481961, 66.49579001460178063, -13.13245767378105811 ) ) ;
#65878=EDGE_LOOP ( 'NONE', ( #38216, #3563, #20021, #94975 ) ) ;
#65885=CARTESIAN_POINT ( 'NONE',  ( 86.51620552470654957, 43.45092470964799247, -2.691706072484096879 ) ) ;
#65900=ORIENTED_EDGE ( 'NONE', *, *, #64625, .F. ) ;
#65901=CARTESIAN_POINT ( 'NONE',  ( 83.59145317797239727, 44.17686507203912782, -8.297778310668469715 ) ) ;
#65902=CARTESIAN_POINT ( 'NONE',  ( 83.25069437720389942, 41.52116721019276468, 1.986236189183263390 ) ) ;
#65905=CARTESIAN_POINT ( 'NONE',  ( 75.16962353025014920, 63.22591803360379004, 14.72285336180162396 ) ) ;
#65907=VERTEX_POINT ( 'NONE', #4950 ) ;
#65908=CARTESIAN_POINT ( 'NONE',  ( 77.14591628819390223, 58.19862468565533931, 16.13876800688947810 ) ) ;
#65915=CARTESIAN_POINT ( 'NONE',  ( 69.48133079272756163, 70.40394783201412565, 3.079148351843276288 ) ) ;
#65919=B_SPLINE_SURFACE_WITH_KNOTS ( 'NONE', 3, 1, ( 
 ( #81574, #36417 ),
 ( #4531, #81089 ),
 ( #19754, #50622 ),
 ( #20750, #65337 ),
 ( #67324, #73945 ),
 ( #29827, #91660 ),
 ( #61216, #75960 ),
 ( #21728, #83068 ),
 ( #22733, #53611 ),
 ( #7516, #29338 ),
 ( #52612, #100245 ),
 ( #75443, #23212 ),
 ( #54102, #15607 ),
 ( #77443, #38911 ),
 ( #69817, #9025 ),
 ( #77940, #94165 ),
 ( #63223, #18134 ),
 ( #16620, #63726 ),
 ( #70316, #87096 ),
 ( #64224, #32322 ),
 ( #86584, #17635 ),
 ( #17119, #78958 ),
 ( #49035, #72356 ),
 ( #93156, #85584 ),
 ( #9547, #74355 ),
 ( #49521, #73830 ),
 ( #27731, #20137 ),
 ( #51517, #72858 ),
 ( #34809, #26235 ),
 ( #43907, #96664 ),
 ( #43408, #33854 ) ),
 .UNSPECIFIED., .F., .F., .F.,
 ( 4, 3, 3, 3, 3, 3, 3, 3, 3, 3, 4 ),
 ( 2, 2 ),
 ( 0.000000000000000000, 0.1333490885032282969, 0.3007194338854215498, 0.4699862290245004903, 0.5844252810809279497, 0.6686540514502673505, 0.7354980260655414881, 0.8028463152565613603, 0.8633854507757170449, 0.9437142632667081532, 1.000000000000000000 ),
 ( 0.000000000000000000, 1.000000000000000000 ),
 .UNSPECIFIED. ) ;
#65920=CARTESIAN_POINT ( 'NONE',  ( 24.24684063885245422, 16.12755873383626337, -6.180339887498949025 ) ) ;
#65929=CARTESIAN_POINT ( 'NONE',  ( 87.86298961015023679, 44.89260222163543546, 6.207647304897661478 ) ) ;
#65939=CARTESIAN_POINT ( 'NONE',  ( 24.06687416953986514, 14.86426979415089633, -3.090169943749474069 ) ) ;
#65943=CARTESIAN_POINT ( 'NONE',  ( 72.01443008256866563, 72.40752555085421704, -2.913864408233449943 ) ) ;
#65947=CARTESIAN_POINT ( 'NONE',  ( 77.32817876982272765, 63.13942984521013813, 15.61058464551962111 ) ) ;
#65955=MECHANICAL_DESIGN_GEOMETRIC_PRESENTATION_REPRESENTATION('',(#44901),#23932);
#65959=CARTESIAN_POINT ( 'NONE',  ( 80.49432606691982528, 57.82183276640385117, -16.24662948867364420 ) ) ;
#65961=CARTESIAN_POINT ( 'NONE',  ( 31.53879454291322659, 39.18502408145594984, 5.678558825948277544 ) ) ;
#65962=CARTESIAN_POINT ( 'NONE',  ( 22.25607796093117230, 24.80066082961421969, 10.00000000000000533 ) ) ;
#65968=CARTESIAN_POINT ( 'NONE',  ( 6.527493107231251201, 21.95586893147753216, 7.433330006724141015 ) ) ;
#65970=CARTESIAN_POINT ( 'NONE',  ( 22.90017757337614768, 16.14754757982090183, -5.678558825948275768 ) ) ;
#65975=CARTESIAN_POINT ( 'NONE',  ( 74.98386055540046868, 53.36045814093387207, -16.04777311236104609 ) ) ;
#65981=CARTESIAN_POINT ( 'NONE',  ( 66.76556300634629793, 68.39317378885236565, 4.474931876891666604 ) ) ;
#65982=CARTESIAN_POINT ( 'NONE',  ( 87.16381268512610347, 45.36703396835236646, 7.086030772169831238 ) ) ;
#65983=ORIENTED_EDGE ( 'NONE', *, *, #87317, .T. ) ;
#65990=CARTESIAN_POINT ( 'NONE',  ( 76.77247148145950462, 52.74177840875945122, 15.84678155200985472 ) ) ;
#65992=VERTEX_POINT ( 'NONE', #96677 ) ;
#65993=CARTESIAN_POINT ( 'NONE',  ( 69.05014585453179166, 64.34709911403272997, -11.93475642575615758 ) ) ;
#65994=CARTESIAN_POINT ( 'NONE',  ( 88.54812304393657030, 43.90120638611161752, -0.3063217976418578514 ) ) ;
#65995=EDGE_CURVE ( 'NONE', #17891, #65871, #47500, .T. ) ;
#66003=CARTESIAN_POINT ( 'NONE',  ( 73.39892793531787163, 58.47633737766673079, 15.73411582304112422 ) ) ;
#66009=ORIENTED_EDGE ( 'NONE', *, *, #69063, .T. ) ;
#66013=VERTEX_POINT ( 'NONE', #77323 ) ;
#66018=CARTESIAN_POINT ( 'NONE',  ( 13.51924585473484974, 23.50829794293879615, -10.00000000000000355 ) ) ;
#66024=CARTESIAN_POINT ( 'NONE',  ( 76.32033379547380036, 57.26470140725930236, -16.14692908151009831 ) ) ;
#66031=B_SPLINE_CURVE_WITH_KNOTS ( 'NONE', 3,
 ( #50699, #66412, #27906, #58786, #28400, #49229, #80163, #10730, #34037, #44584, #67908, #14700, #91235, #61289, #36499, #46078, #22802, #83139, #21801, #61785, #67402, #84154, #20829, #36998 ),
 .UNSPECIFIED., .F., .F.,
 ( 4, 2, 2, 2, 2, 2, 2, 2, 2, 2, 2, 4 ),
 ( 0.000000000000000000, 0.1250000000000071332, 0.2500000000000142664, 0.3750000000000214273, 0.4375000000000193179, 0.5000000000000172085, 0.5625000000000150990, 0.6250000000000129896, 0.6875000000000108802, 0.7500000000000087708, 0.8750000000000044409, 1.000000000000000000 ),
 .UNSPECIFIED. ) ;
#66033=CARTESIAN_POINT ( 'NONE',  ( 83.34286953481752391, 51.57169424047764750, -14.50199425999806735 ) ) ;
#66042=DIRECTION ( 'NONE',  ( -0.7905172007421662483, 0.000000000000000000, -0.6124398381316892293 ) ) ;
#66057=CARTESIAN_POINT ( 'NONE',  ( 70.11469351433765951, 71.12949179974985725, -0.2432596123983654379 ) ) ;
#66059=LINE ( 'NONE', #50352, #43006 ) ;
#66061=CARTESIAN_POINT ( 'NONE',  ( 73.95565718806818722, 68.30423517461105121, -11.66005733018688773 ) ) ;
#66065=VERTEX_POINT ( 'NONE', #23102 ) ;
#66066=LINE ( 'NONE', #97973, #91764 ) ;
#66072=CARTESIAN_POINT ( 'NONE',  ( 68.84812201532827203, 64.26021157803218387, -11.91067767038833480 ) ) ;
#66074=CARTESIAN_POINT ( 'NONE',  ( 79.38214399233697804, 46.87024971659150907, 13.67178478057998525 ) ) ;
#66079=CARTESIAN_POINT ( 'NONE',  ( 70.43502381298807791, 70.21998739243254306, 5.513655153572781131 ) ) ;
#66086=CARTESIAN_POINT ( 'NONE',  ( 22.44070990177030112, 31.14336893147756413, 7.433330006724141015 ) ) ;
#66087=CARTESIAN_POINT ( 'NONE',  ( 74.70353909524752112, 67.05423462026553239, 12.97237599094835936 ) ) ;
#66089=CARTESIAN_POINT ( 'NONE',  ( 82.10523990517461357, 41.85707133252695655, -5.529865280922476423 ) ) ;
#66090=CARTESIAN_POINT ( 'NONE',  ( 74.63372323989780455, 66.93453420673688470, 13.02704161780705761 ) ) ;
#66096=CARTESIAN_POINT ( 'NONE',  ( 81.44589832458051148, 55.42546683620729908, -16.32034488869437894 ) ) ;
#66098=CARTESIAN_POINT ( 'NONE',  ( 68.55578159652473857, 66.09187073463988327, 10.06848484671900756 ) ) ;
#66100=CARTESIAN_POINT ( 'NONE',  ( 71.73821799984662562, 72.51259063078050815, 0.9720659048468541785 ) ) ;
#66101=CARTESIAN_POINT ( 'NONE',  ( 82.70906748317777613, 41.57766049848077472, 3.737552679734466032 ) ) ;
#66107=CARTESIAN_POINT ( 'NONE',  ( 8.995063969029878592, 17.14441083166259006, 10.00000000000000533 ) ) ;
#66108=CARTESIAN_POINT ( 'NONE',  ( 83.51785737385900177, 46.57979345909983238, 11.73479753357512401 ) ) ;
#66110=CARTESIAN_POINT ( 'NONE',  ( 73.67824366217406862, 55.52431661998091528, 16.58293631993679540 ) ) ;
#66114=CARTESIAN_POINT ( 'NONE',  ( 78.87940645753282354, 60.08920343663678665, 16.11186154035030782 ) ) ;
#66120=CARTESIAN_POINT ( 'NONE',  ( 84.31620464638353951, 49.88582837545166626, -13.33668689155092757 ) ) ;
#66121=CARTESIAN_POINT ( 'NONE',  ( 84.68407782013028395, 49.81677542588726482, -13.17038101989053622 ) ) ;
#66122=CARTESIAN_POINT ( 'NONE',  ( 81.30093862219625578, 42.22353087488599499, -7.211150227892720643 ) ) ;
#66126=ORIENTED_EDGE ( 'NONE', *, *, #30590, .F. ) ;
#66134=CARTESIAN_POINT ( 'NONE',  ( 82.21410988463139802, 40.73976263607374193, 3.762362152811430160 ) ) ;
#66140=CARTESIAN_POINT ( 'NONE',  ( 18.55511606660780899, 34.21091486745861232, -1.111400068045478839E-16 ) ) ;
#66143=CARTESIAN_POINT ( 'NONE',  ( 75.88266154223501303, 55.68909319084332310, 16.14856353405036771 ) ) ;
#66145=CARTESIAN_POINT ( 'NONE',  ( 16.39654754030849659, 10.26216523072493203, -2.296566073217252530E-15 ) ) ;
#66151=CARTESIAN_POINT ( 'NONE',  ( 85.35583701238070375, 48.33319239702164083, -12.28927654967824701 ) ) ;
#66158=CARTESIAN_POINT ( 'NONE',  ( 85.04454326977196388, 42.52624631695034907, 2.010354791463878410 ) ) ;
#66159=CARTESIAN_POINT ( 'NONE',  ( 87.99802445900249381, 44.07685147378857238, -1.716111015435727527 ) ) ;
#66164=CARTESIAN_POINT ( 'NONE',  ( 65.86576390661227265, 69.15346480495860249, 0.2105079060664491741 ) ) ;
#66171=CARTESIAN_POINT ( 'NONE',  ( 71.47791206682282450, 72.34364865201938244, -1.216664393387148380 ) ) ;
#66172=CARTESIAN_POINT ( 'NONE',  ( 88.13962338646859962, 43.88173199026377347, 2.505344897735772847 ) ) ;
#66177=ORIENTED_EDGE ( 'NONE', *, *, #78036, .T. ) ;
#66178=CARTESIAN_POINT ( 'NONE',  ( 72.03258563326085095, 62.35762028613417840, -14.22870005908225544 ) ) ;
#66179=CARTESIAN_POINT ( 'NONE',  ( 80.44411425790228520, 57.92825487739349200, 16.25450948704126830 ) ) ;
#66181=CARTESIAN_POINT ( 'NONE',  ( 70.66815415073801887, 66.12807013279959278, -11.28611302301944441 ) ) ;
#66184=CARTESIAN_POINT ( 'NONE',  ( 81.00087151702695110, 43.68496140122994120, -9.524658774912921899 ) ) ;
#66197=CARTESIAN_POINT ( 'NONE',  ( 84.62070576355738183, 50.25222463068733703, 13.86530520652494758 ) ) ;
#66209=VECTOR ( 'NONE', #37034, 1000.000000000000114 ) ;
#66212=CARTESIAN_POINT ( 'NONE',  ( 85.68213310926148552, 42.83582516110543992, -1.677889640976326868 ) ) ;
#66213=CARTESIAN_POINT ( 'NONE',  ( 75.71688963635942571, 65.45405155058689672, 14.28099675560567228 ) ) ;
#66214=CARTESIAN_POINT ( 'NONE',  ( 80.31380282231825163, 44.31269810431638945, 11.34184801982937429 ) ) ;
#66215=CARTESIAN_POINT ( 'NONE',  ( 29.36891313204580456, 35.14336893147757479, 7.433330006724141015 ) ) ;
#66219=CARTESIAN_POINT ( 'NONE',  ( 16.96131155903493593, 31.83396525600390348, -2.839279412974133887 ) ) ;
#66221=CARTESIAN_POINT ( 'NONE',  ( 17.25239830753785952, 10.36477965099639498, 1.583844403245364907 ) ) ;
#66225=CARTESIAN_POINT ( 'NONE',  ( 86.15223587325151300, 47.11913640227773925, 10.79538652562921541 ) ) ;
#66231=CARTESIAN_POINT ( 'NONE',  ( 74.89001754810668388, 53.31247712445269826, 16.04945090674765851 ) ) ;
#66233=CARTESIAN_POINT ( 'NONE',  ( 85.61210927225859280, 46.71934343149948887, 10.13913704453490539 ) ) ;
#66236=CARTESIAN_POINT ( 'NONE',  ( 86.86805282215009072, 44.88340327883143743, 6.465678163750347984 ) ) ;
#66239=VERTEX_POINT ( 'NONE', #7930 ) ;
#66240=CARTESIAN_POINT ( 'NONE',  ( 71.97624815057693581, 71.57072644777218784, 5.573434703584684513 ) ) ;
#66243=CARTESIAN_POINT ( 'NONE',  ( 87.87366831029828518, 44.19753277059973584, -4.411077605820552527 ) ) ;
#66247=CARTESIAN_POINT ( 'NONE',  ( 34.35336353842534152, 22.76004757982091675, 5.678558825948272215 ) ) ;
#66254=CARTESIAN_POINT ( 'NONE',  ( 84.43973019491031096, 50.14528805649905507, 13.86389828189430062 ) ) ;
#66255=CARTESIAN_POINT ( 'NONE',  ( 68.26472058833583390, 65.55548226720446792, 10.44615040622151803 ) ) ;
#66257=CARTESIAN_POINT ( 'NONE',  ( 85.93470712620026575, 48.23248545518190866, 11.93606436224419376 ) ) ;
#66258=CARTESIAN_POINT ( 'NONE',  ( 66.08029938247301516, 68.49631965208827467, -2.562324766759315420 ) ) ;
#66272=CARTESIAN_POINT ( 'NONE',  ( 87.23690874686347740, 46.15778144619924461, -8.941654336830676897 ) ) ;
#66279=FACE_OUTER_BOUND ( 'NONE', #97081, .T. ) ;
#66286=CARTESIAN_POINT ( 'NONE',  ( 82.30283500558374499, 44.69232536722564930, 9.873559656175117993 ) ) ;
#66288=CARTESIAN_POINT ( 'NONE',  ( 69.51817709403496792, 62.60037355296611850, -13.88906238228599577 ) ) ;
#66289=FACE_OUTER_BOUND ( 'NONE', #13172, .T. ) ;
#66291=VERTEX_POINT ( 'NONE', #42298 ) ;
#66293=CARTESIAN_POINT ( 'NONE',  ( 71.30005785884924308, 62.11168698697181156, 14.13435735937659388 ) ) ;
#66294=CARTESIAN_POINT ( 'NONE',  ( 82.23170604078318036, 40.61139441586372101, -3.203312919990458418 ) ) ;
#66295=CARTESIAN_POINT ( 'NONE',  ( 80.95862166114621061, 43.54618974350823635, 9.386765060990684972 ) ) ;
#66300=VECTOR ( 'NONE', #49984, 1000.000000000000227 ) ;
#66301=CARTESIAN_POINT ( 'NONE',  ( 80.54656262287409163, 52.70628843406199593, 15.42795475958373252 ) ) ;
#66302=CARTESIAN_POINT ( 'NONE',  ( 16.16012747849099540, 9.734156793818206310, 1.333680081654574804E-15 ) ) ;
#66312=CARTESIAN_POINT ( 'NONE',  ( 37.57390229391633341, 33.64441083166263979, -10.00000000000000533 ) ) ;
#66315=CARTESIAN_POINT ( 'NONE',  ( 86.09177458334599464, 43.55638514111210213, -4.160762740161195516 ) ) ;
#66317=CARTESIAN_POINT ( 'NONE',  ( 80.99988074727858134, 44.69027685233859870, 10.63760621275858576 ) ) ;
#66319=B_SPLINE_CURVE_WITH_KNOTS ( 'NONE', 3,
 ( #69434, #46627, #10650, #17752, #25333, #2047, #34438, #81087, #10149, #18750, #79079, #49147, #41525, #57720, #94771, #11653, #2557, #33440, #9661, #40521, #80081, #42514, #73451, #55704, #18252, #72468, #17226, #11164, #19269, #3557, #3074 ),
 .UNSPECIFIED., .F., .F.,
 ( 4, 3, 3, 3, 3, 3, 3, 3, 3, 3, 4 ),
 ( 0.000000000000000000, 0.1333490885032338480, 0.3007194338854361493, 0.4699862290245140906, 0.5844252810809331677, 0.6686540514502653521, 0.7354980260655413771, 0.8028463152565569194, 0.8633854507757173780, 0.9437142632667304687, 1.000000000000000000 ),
 .UNSPECIFIED. ) ;
#66321=CARTESIAN_POINT ( 'NONE',  ( 87.13698410836482822, 46.33067510313777859, 8.599260793297284877 ) ) ;
#66323=CARTESIAN_POINT ( 'NONE',  ( 71.89024115076192345, 72.14005084039141025, -1.691652508062526650 ) ) ;
#66325=CARTESIAN_POINT ( 'NONE',  ( 86.92045001522136261, 45.99340221249899940, 8.966174604352282529 ) ) ;
#66328=CARTESIAN_POINT ( 'NONE',  ( 37.86538501507695287, 37.56454794089044213, 10.00000000000000355 ) ) ;
#66332=CARTESIAN_POINT ( 'NONE',  ( 68.22205435738101187, 65.90345407221148832, 10.80313017757570471 ) ) ;
#66333=CARTESIAN_POINT ( 'NONE',  ( 87.05121076158607707, 45.95104493586815408, -8.147482009912135226 ) ) ;
#66336=CARTESIAN_POINT ( 'NONE',  ( 75.33387806111561247, 65.67578613345442307, -13.61108734441214807 ) ) ;
#66338=ORIENTED_EDGE ( 'NONE', *, *, #69723, .T. ) ;
#66343=CARTESIAN_POINT ( 'NONE',  ( 67.67908650673803095, 66.83328552386096533, -8.531651213308034443 ) ) ;
#66348=CARTESIAN_POINT ( 'NONE',  ( 31.37760429443829224, 33.51421378149921537, -9.188101187500004485 ) ) ;
#66350=CARTESIAN_POINT ( 'NONE',  ( 86.50792306782743424, 47.43283652443698628, -10.36525212966502174 ) ) ;
#66351=CARTESIAN_POINT ( 'NONE',  ( 34.61729389309891758, 20.39040679176985549, -6.890680421881970419E-14 ) ) ;
#66354=CARTESIAN_POINT ( 'NONE',  ( 13.45569633750675465, 25.95586893147754282, 7.433330006724141015 ) ) ;
#66355=CARTESIAN_POINT ( 'NONE',  ( 76.31365291358306990, 61.99157619597451685, 15.38880639136091233 ) ) ;
#66359=CARTESIAN_POINT ( 'NONE',  ( 77.21042888011766081, 57.50458007534377458, 16.59863515784280352 ) ) ;
#66362=ORIENTED_EDGE ( 'NONE', *, *, #45370, .T. ) ;
#66366=CARTESIAN_POINT ( 'NONE',  ( 85.49318370521093868, 48.99722645306705715, -12.73116331006621493 ) ) ;
#66369=CARTESIAN_POINT ( 'NONE',  ( 66.52541744028246740, 68.80911811048743232, -2.215339755367858210 ) ) ;
#66372=DIRECTION ( 'NONE',  ( 0.5000000000000013323, -0.8660254037844378194, 0.000000000000000000 ) ) ;
#66387=CARTESIAN_POINT ( 'NONE',  ( 81.63113279203287220, 55.88178493786749357, 16.01941705845313280 ) ) ;
#66390=ORIENTED_EDGE ( 'NONE', *, *, #74241, .F. ) ;
#66394=CYLINDRICAL_SURFACE ( 'NONE', #86900, 16.60714546451156792 ) ;
#66396=EDGE_CURVE ( 'NONE', #48842, #19318, #23270, .T. ) ;
#66407=CARTESIAN_POINT ( 'NONE',  ( 83.13178773832562740, 44.19191255805648666, -8.679323957351682495 ) ) ;
#66412=CARTESIAN_POINT ( 'NONE',  ( 79.24143198459856308, 59.88451820689867588, -16.14143938394746414 ) ) ;
#66413=CARTESIAN_POINT ( 'NONE',  ( 74.97830149814869571, 62.15334231524035147, 15.06231098758508402 ) ) ;
#66416=CARTESIAN_POINT ( 'NONE',  ( 77.44539015164885143, 60.39115425616281385, 15.91752098216395162 ) ) ;
#66422=CARTESIAN_POINT ( 'NONE',  ( 69.53218774831623250, 70.45193905447369787, 3.001416003324469450 ) ) ;
#66427=CARTESIAN_POINT ( 'NONE',  ( 20.05933935144479463, 19.78052372038640527, -10.00000000000000355 ) ) ;
#66439=FACE_OUTER_BOUND ( 'NONE', #2717, .T. ) ;
#66444=CARTESIAN_POINT ( 'NONE',  ( 85.08976737157280468, 48.95938582862681443, 12.42920128896121668 ) ) ;
#66446=CARTESIAN_POINT ( 'NONE',  ( 72.30409372968703963, 72.02947187496847903, -3.500239827782243296 ) ) ;
#66447=CARTESIAN_POINT ( 'NONE',  ( 73.74733062278515661, 55.38161606902450984, -16.59075967854369438 ) ) ;
#66448=EDGE_CURVE ( 'NONE', #26733, #40804, #93278, .T. ) ;
#66458=CARTESIAN_POINT ( 'NONE',  ( 72.73269248836918166, 71.16345857084105830, -7.307540741686431751 ) ) ;
#66459=CARTESIAN_POINT ( 'NONE',  ( 79.31104985338477320, 59.89077999431003008, 16.15264230762560516 ) ) ;
#66460=CARTESIAN_POINT ( 'NONE',  ( 34.51455378690028652, 28.43085787977765477, -9.188101187500008038 ) ) ;
#66467=CARTESIAN_POINT ( 'NONE',  ( 15.78914702631840328, 24.51421378149918695, -9.188101187500004485 ) ) ;
#66469=CARTESIAN_POINT ( 'NONE',  ( 82.48148221723897677, 54.22512503293472719, 15.59203162474583415 ) ) ;
#66478=CARTESIAN_POINT ( 'NONE',  ( 66.24598407424289803, 68.55598904622115697, 4.800278518307799835 ) ) ;
#66486=CARTESIAN_POINT ( 'NONE',  ( 88.44819812734249354, 44.06706281553302773, -2.545729839345954204 ) ) ;
#66487=CARTESIAN_POINT ( 'NONE',  ( 80.24292271875241056, 58.10242382007938744, 16.26432532982812518 ) ) ;
#66490=CARTESIAN_POINT ( 'NONE',  ( 78.25048285508148638, 61.03959493798094371, -15.91191902859591778 ) ) ;
#66493=CARTESIAN_POINT ( 'NONE',  ( 80.91343449481020400, 43.02608183091172123, 9.608889258680049394 ) ) ;
#66498=CARTESIAN_POINT ( 'NONE',  ( 73.72813317336040484, 59.85036616854785763, 15.47704302871372839 ) ) ;
#66507=ORIENTED_EDGE ( 'NONE', *, *, #97588, .T. ) ;
#66509=CARTESIAN_POINT ( 'NONE',  ( 87.62257652462700719, 43.83610729166736064, 1.029400949057958314 ) ) ;
#66514=EDGE_CURVE ( 'NONE', #57272, #74992, #26818, .T. ) ;
#66518=CARTESIAN_POINT ( 'NONE',  ( 79.83679441914436836, 55.88931611243568653, -16.12940057729960230 ) ) ;
#66525=ORIENTED_EDGE ( 'NONE', *, *, #15983, .T. ) ;
#66527=CARTESIAN_POINT ( 'NONE',  ( 82.64744444949904789, 51.85429353291556254, -14.77163707229560963 ) ) ;
#66530=CARTESIAN_POINT ( 'NONE',  ( 10.46840290624634306, 27.81751292744054993, -6.180339887498951690 ) ) ;
#66537=CARTESIAN_POINT ( 'NONE',  ( 89.82826426823238819, 45.13720097505219542, 0.2499999999999960032 ) ) ;
#66546=CARTESIAN_POINT ( 'NONE',  ( 43.27754793094329244, 25.39040679176986970, -6.890680421881970419E-14 ) ) ;
#66549=CARTESIAN_POINT ( 'NONE',  ( 74.46971312594514814, 68.19886894342141659, -11.52194869617921569 ) ) ;
#66553=CARTESIAN_POINT ( 'NONE',  ( 81.78771499908393139, 41.70666495146470254, -5.605238045589925555 ) ) ;
#66554=CARTESIAN_POINT ( 'NONE',  ( 7.283862947486896999, 19.90829794293878408, 10.00000000000000355 ) ) ;
#66569=CARTESIAN_POINT ( 'NONE',  ( 66.33611483106668061, 68.05323429769379118, -4.754337940927038098 ) ) ;
#66572=CARTESIAN_POINT ( 'NONE',  ( 72.53559621566675730, 57.32287681765896536, 16.32930890408951541 ) ) ;
#66573=CARTESIAN_POINT ( 'NONE',  ( 69.43155330386302637, 68.70253108992608304, 7.308829108440537681 ) ) ;
#66576=EDGE_LOOP ( 'NONE', ( #2979, #45393, #71146, #15130 ) ) ;
#66577=VECTOR ( 'NONE', #20133, 1000.000000000000000 ) ;
#66581=CARTESIAN_POINT ( 'NONE',  ( 20.42541317417268942, 33.83396525600390703, -2.839279412974133887 ) ) ;
#66584=CARTESIAN_POINT ( 'NONE',  ( 83.80447776121599190, 52.10292630681441040, -14.99896445683751622 ) ) ;
#66585=CARTESIAN_POINT ( 'NONE',  ( 76.62413771374467331, 63.45693921867285070, 15.36854489724363759 ) ) ;
#66586=CARTESIAN_POINT ( 'NONE',  ( 76.28872632190457637, 51.00282802105010660, -16.03419075268625349 ) ) ;
#66589=ORIENTED_EDGE ( 'NONE', *, *, #37319, .T. ) ;
#66594=CARTESIAN_POINT ( 'NONE',  ( 13.25720545158990937, 8.449665230724928477, -2.296566073217252530E-15 ) ) ;
#66596=CARTESIAN_POINT ( 'NONE',  ( 68.81099849051250317, 66.60367167969251057, 9.666683708442542766 ) ) ;
#66598=CARTESIAN_POINT ( 'NONE',  ( 77.54947637239327207, 49.71488793443786136, 14.94482653940103134 ) ) ;
#66601=CARTESIAN_POINT ( 'NONE',  ( 69.67981129362297565, 70.80532903890349417, 1.547790508053775937 ) ) ;
#66602=CARTESIAN_POINT ( 'NONE',  ( 74.08065690531797998, 54.82731643721707826, -16.13522336645905142 ) ) ;
#66604=CARTESIAN_POINT ( 'NONE',  ( 12.36470590445056317, 8.108019796199268825, 3.090169943749476733 ) ) ;
#66615=ORIENTED_EDGE ( 'NONE', *, *, #14490, .T. ) ;
#66618=CARTESIAN_POINT ( 'NONE',  ( 84.42663183290281381, 49.91580812419739033, -13.73522929182741947 ) ) ;
#66631=CARTESIAN_POINT ( 'NONE',  ( 82.49834280522868823, 40.76233756830425392, 3.189866935900057765 ) ) ;
#66634=EDGE_CURVE ( 'NONE', #54109, #44579, #30445, .T. ) ;
#66638=CARTESIAN_POINT ( 'NONE',  ( 76.45176290624858950, 58.46688331479428058, 16.04654028584893055 ) ) ;
#66639=CARTESIAN_POINT ( 'NONE',  ( 13.40518456965460281, 16.24335787977761925, -9.188101187500008038 ) ) ;
#66646=CARTESIAN_POINT ( 'NONE',  ( 76.12311946169329246, 64.72429642162367713, -14.36203512785002090 ) ) ;
#66651=EDGE_CURVE ( 'NONE', #69830, #77062, #61829, .T. ) ;
#66660=CARTESIAN_POINT ( 'NONE',  ( 82.34616035088453145, 44.74534029615586661, -9.883898186199504110 ) ) ;
#66663=CARTESIAN_POINT ( 'NONE',  ( 88.30945731027941292, 43.97049527616570685, 2.452112525173328450 ) ) ;
#66666=VERTEX_POINT ( 'NONE', #82739 ) ;
#66669=CARTESIAN_POINT ( 'NONE',  ( 85.68734770396230260, 48.85621462398719217, -12.54449143327926208 ) ) ;
#66672=CARTESIAN_POINT ( 'NONE',  ( 80.76429156517131958, 43.10381631070730890, -9.805890018733025570 ) ) ;
#66678=CARTESIAN_POINT ( 'NONE',  ( 79.39086535420604207, 59.11638920646624484, 16.20638822945242197 ) ) ;
#66679=ADVANCED_FACE ( 'NONE', ( #82242 ), #76548, .T. ) ;
#66686=CARTESIAN_POINT ( 'NONE',  ( 84.34693788441749973, 50.67364717229969528, 13.78469515595785033 ) ) ;
#66692=CARTESIAN_POINT ( 'NONE',  ( 12.16146256644911539, 9.947547579820877672, 5.678558825948272215 ) ) ;
#66699=CARTESIAN_POINT ( 'NONE',  ( 79.95866072124864843, 44.52494782656018657, 11.71661119140258300 ) ) ;
#66700=CARTESIAN_POINT ( 'NONE',  ( 35.11595366814305663, 25.98920272979928470, 7.433330006724137462 ) ) ;
#66702=CARTESIAN_POINT ( 'NONE',  ( 83.99374970662998408, 46.89514837332161790, -11.15785913519821015 ) ) ;
#66704=CARTESIAN_POINT ( 'NONE',  ( 21.31005897544419980, 27.70171378149919050, -9.188101187500004485 ) ) ;
#66708=ORIENTED_EDGE ( 'NONE', *, *, #95261, .F. ) ;
#66709=CARTESIAN_POINT ( 'NONE',  ( 70.36476379532911096, 61.16554131547574968, 14.31790743328406101 ) ) ;
#66710=CARTESIAN_POINT ( 'NONE',  ( 67.61549177878170269, 66.83199286464724764, -8.481431920729969320 ) ) ;
#66717=ORIENTED_EDGE ( 'NONE', *, *, #80820, .T. ) ;
#66718=CARTESIAN_POINT ( 'NONE',  ( 81.15728453326165948, 46.74340589432950566, -12.91012880180904432 ) ) ;
#66720=ORIENTED_EDGE ( 'NONE', *, *, #86296, .F. ) ;
#66723=ADVANCED_FACE ( 'NONE', ( #61858 ), #92807, .T. ) ;
#66724=EDGE_LOOP ( 'NONE', ( #38426, #17172, #60477, #803 ) ) ;
#66725=CARTESIAN_POINT ( 'NONE',  ( 77.19959510277064396, 63.54604015844361697, -15.07525604178641565 ) ) ;
#66732=CARTESIAN_POINT ( 'NONE',  ( 41.62797693021462209, 26.96004757982093025, -5.678558825948275768 ) ) ;
#66733=CARTESIAN_POINT ( 'NONE',  ( 72.70942444841369934, 60.67579778368086352, -15.05243087098393495 ) ) ;
#66739=( BOUNDED_CURVE ( )  B_SPLINE_CURVE ( 2, ( #96751, #10617, #56706, #64309, #34406, #35399, #97240, #26809, #72437, #57191, #19238, #87687, #18719 ),
 .UNSPECIFIED., .F., .T. ) 
 B_SPLINE_CURVE_WITH_KNOTS ( ( 3, 2, 2, 2, 2, 2, 3 ),
 ( 0.6875000000000000000, 0.6899999999999999467, 0.6949999999999999512, 0.6999999999999999556, 0.7049999999999999600, 0.7099999999999999645, 0.7125000000000000222 ),
 .UNSPECIFIED. ) 
 CURVE ( )  GEOMETRIC_REPRESENTATION_ITEM ( )  RATIONAL_B_SPLINE_CURVE ( ( 0.9755282581475768211, 0.9755282581475768211, 1.000000000000000000, 0.9510565162951535312, 1.000000000000000000, 0.9510565162951535312, 1.000000000000000000, 0.9510565162951535312, 1.000000000000000000, 0.9510565162951535312, 1.000000000000000000, 0.9755282581475761550, 0.9755282581475767101 ) ) 
 REPRESENTATION_ITEM ( '' )  );
#66742=CARTESIAN_POINT ( 'NONE',  ( 85.39369755680034757, 48.58767798792116821, 12.46940421135661481 ) ) ;
#66743=CARTESIAN_POINT ( 'NONE',  ( 66.17343954913512505, 68.52301864461630032, -2.711686016849372827 ) ) ;
#66746=LINE ( 'NONE', #97681, #91638 ) ;
#66754=ORIENTED_EDGE ( 'NONE', *, *, #88646, .T. ) ;
#66758=ORIENTED_EDGE ( 'NONE', *, *, #56864, .T. ) ;
#66759=CARTESIAN_POINT ( 'NONE',  ( 87.02976255443718401, 46.40020681703909133, -8.772238895811881321 ) ) ;
#66761=B_SPLINE_SURFACE_WITH_KNOTS ( 'NONE', 3, 1, ( 
 ( #22556, #83397 ),
 ( #13966, #69645 ),
 ( #53441, #14938 ),
 ( #45829, #75782 ),
 ( #69144, #100073 ),
 ( #30660, #6368 ),
 ( #28657, #59540 ),
 ( #37252, #29660 ),
 ( #68151, #60537 ),
 ( #90519, #51968 ),
 ( #82908, #13480 ),
 ( #44351, #16941 ),
 ( #1770, #47827 ),
 ( #62026, #77771 ),
 ( #78766, #9353 ),
 ( #63545, #32649 ),
 ( #70644, #24047 ),
 ( #85399, #8846 ),
 ( #2270, #63049 ),
 ( #70132, #86410 ),
 ( #8356, #32141 ),
 ( #15946, #39716 ),
 ( #47341, #54942 ),
 ( #46849, #94486 ),
 ( #85919, #39225 ),
 ( #745, #71679 ),
 ( #31629, #25045 ),
 ( #1259, #93993 ),
 ( #40231, #24543 ),
 ( #17451, #62528 ),
 ( #92977, #48359 ) ),
 .UNSPECIFIED., .F., .F., .F.,
 ( 4, 3, 3, 3, 3, 3, 3, 3, 3, 3, 4 ),
 ( 2, 2 ),
 ( 0.000000000000000000, 0.1333490885032479201, 0.3007194338854572990, 0.4699862290245473417, 0.5844252810809665855, 0.6686540514502945509, 0.7354980260655585855, 0.8028463152565719074, 0.8633854507757248165, 0.9437142632667163689, 1.000000000000000000 ),
 ( 0.000000000000000000, 1.000000000000000000 ),
 .UNSPECIFIED. ) ;
#66766=DIRECTION ( 'NONE',  ( 0.2359789242578333723, 0.9717581732643754133, 0.000000000000000000 ) ) ;
#66768=ADVANCED_FACE ( 'NONE', ( #47661 ), #83859, .T. ) ;
#66769=ORIENTED_EDGE ( 'NONE', *, *, #80216, .T. ) ;
#66771=EDGE_CURVE ( 'NONE', #58122, #46236, #48595, .T. ) ;
#66775=PLANE ( 'NONE',  #88689 ) ;
#66777=CARTESIAN_POINT ( 'NONE',  ( 84.00458678407764523, 49.73832886490323801, 13.34265766643008000 ) ) ;
#66779=CARTESIAN_POINT ( 'NONE',  ( 80.32771389996757705, 57.94408260071153194, -16.24746918486169633 ) ) ;
#66780=PLANE ( 'NONE',  #43001 ) ;
#66783=CARTESIAN_POINT ( 'NONE',  ( 81.84975730146675232, 49.11728276204326704, 13.61519513745881582 ) ) ;
#66789=CARTESIAN_POINT ( 'NONE',  ( 81.68921996421825327, 59.23443923465870142, 0.4890738003669021228 ) ) ;
#66790=CARTESIAN_POINT ( 'NONE',  ( 80.49194482161659892, 52.40313326226726076, 15.34488516401063229 ) ) ;
#66795=CARTESIAN_POINT ( 'NONE',  ( 77.73453021100772276, 61.59708935479353897, 16.08607222837813922 ) ) ;
#66797=CARTESIAN_POINT ( 'NONE',  ( 67.47767788923495402, 69.56616349044860215, -0.01493465584580692777 ) ) ;
#66798=DIRECTION ( 'NONE',  ( -0.3213938048432640748, 0.5566703992264119272, -0.7660444431189857850 ) ) ;
#66799=CARTESIAN_POINT ( 'NONE',  ( 78.91181281398866076, 50.63267699903087049, 15.50297620496208317 ) ) ;
#66800=CARTESIAN_POINT ( 'NONE',  ( 33.24377527499414242, 31.14441083166263269, 10.00000000000000533 ) ) ;
#66801=CARTESIAN_POINT ( 'NONE',  ( 79.40381832342256985, 56.26532398263896795, -16.55503524308543462 ) ) ;
#66802=CARTESIAN_POINT ( 'NONE',  ( 82.70408928404155802, 54.02126990151200658, 15.49668869734769672 ) ) ;
#66803=CARTESIAN_POINT ( 'NONE',  ( 71.79701493962480185, 71.88116747554488484, 2.917949182627429305 ) ) ;
#66805=CARTESIAN_POINT ( 'NONE',  ( 67.73185026608422277, 68.24509447089671710, 7.391104519061957312 ) ) ;
#66810=CARTESIAN_POINT ( 'NONE',  ( 34.30385554556135475, 35.50829794293883168, -10.00000000000000355 ) ) ;
#66813=EDGE_CURVE ( 'NONE', #37857, #82804, #97302, .T. ) ;
#66817=CARTESIAN_POINT ( 'NONE',  ( 42.68871737883920048, 29.81029122506298634, 8.090169943749479842 ) ) ;
#66822=CARTESIAN_POINT ( 'NONE',  ( 67.99639869681988102, 67.83379250622242296, -7.292278942132766062 ) ) ;
#66824=AXIS2_PLACEMENT_3D ( 'NONE', #26199, #81929, #50976 ) ;
#66827=CARTESIAN_POINT ( 'NONE',  ( 81.52469153597657225, 59.51941083166271795, 0.2499999999999960032 ) ) ;
#66834=CARTESIAN_POINT ( 'NONE',  ( 67.20567196973209434, 67.17854346287718670, -8.569229914137681092 ) ) ;
#66839=CARTESIAN_POINT ( 'NONE',  ( 81.17232691891706509, 55.55242957854174080, 16.36487835605630536 ) ) ;
#66840=CARTESIAN_POINT ( 'NONE',  ( 34.35336353842534152, 22.76004757982091320, 5.678558825948272215 ) ) ;
#66845=CARTESIAN_POINT ( 'NONE',  ( 19.31277771287585310, 13.01110640527291551, 2.839279412974134775 ) ) ;
#66847=CARTESIAN_POINT ( 'NONE',  ( 66.88651227603331506, 69.13534811060253560, -1.466183419788135378 ) ) ;
#66849=ORIENTED_EDGE ( 'NONE', *, *, #47713, .F. ) ;
#66850=CARTESIAN_POINT ( 'NONE',  ( 76.74641017894596473, 54.96141969970745578, 16.56981576960984626 ) ) ;
#66851=CARTESIAN_POINT ( 'NONE',  ( 65.82437655349816907, 69.12761348810170148, -0.3171013769033947383 ) ) ;
#66858=ORIENTED_EDGE ( 'NONE', *, *, #33705, .F. ) ;
#66859=CARTESIAN_POINT ( 'NONE',  ( 66.29454943682360124, 69.24199052645600716, -2.144636311120903471 ) ) ;
#66861=CARTESIAN_POINT ( 'NONE',  ( 72.41389820116259557, 70.72247311216294463, 7.745007521649668547 ) ) ;
#66875=CARTESIAN_POINT ( 'NONE',  ( 81.58121470000600084, 55.78443411318616540, 16.36431025809738671 ) ) ;
#66879=CARTESIAN_POINT ( 'NONE',  ( 87.68151411726066158, 45.11153824597519701, 6.862463844403660751 ) ) ;
#66881=EDGE_CURVE ( 'NONE', #55501, #19903, #59750, .T. ) ;
#66885=ORIENTED_EDGE ( 'NONE', *, *, #97007, .T. ) ;
#66887=CARTESIAN_POINT ( 'NONE',  ( 76.21618662203624694, 51.03057968305066083, -16.05037395188493576 ) ) ;
#66899=CARTESIAN_POINT ( 'NONE',  ( 86.13696227940769745, 44.49281544815586642, 6.407054959019385265 ) ) ;
#66900=CARTESIAN_POINT ( 'NONE',  ( 87.88174357402824910, 44.02160025480015548, -1.794566980668626188 ) ) ;
#66905=CARTESIAN_POINT ( 'NONE',  ( 76.96774782091593181, 57.10333325502509183, 16.17939703112071825 ) ) ;
#66915=CARTESIAN_POINT ( 'NONE',  ( 20.78273902371470072, 14.12755873383625627, -6.180339887498949025 ) ) ;
#66919=CARTESIAN_POINT ( 'NONE',  ( 88.28592015977814356, 44.16006502160688996, -0.2344584660017056954 ) ) ;
#66920=CARTESIAN_POINT ( 'NONE',  ( 71.85042758235270810, 71.69843285251393183, -3.789477364735254650 ) ) ;
#66929=CARTESIAN_POINT ( 'NONE',  ( 28.12420092063944566, 24.43677371833802781, -10.00000000000000355 ) ) ;
#66930=CARTESIAN_POINT ( 'NONE',  ( 85.29121890838305831, 49.09086179670648420, 12.44079179351374442 ) ) ;
#66932=CARTESIAN_POINT ( 'NONE',  ( 72.19712139806571827, 71.87787970473654298, -3.871494628622227818 ) ) ;
#66936=CARTESIAN_POINT ( 'NONE',  ( 74.59816150844692118, 67.00000980971049103, 12.52809777808814751 ) ) ;
#66943=CARTESIAN_POINT ( 'NONE',  ( 72.86429505109984461, 70.96802964124920265, -7.768747002037670768 ) ) ;
#66944=EDGE_CURVE ( 'NONE', #47529, #65006, #83102, .T. ) ;
#66945=CARTESIAN_POINT ( 'NONE',  ( 79.42866338260434134, 59.50128377535573776, 16.18467811310512872 ) ) ;
#66946=CARTESIAN_POINT ( 'NONE',  ( 39.17063663036994114, 34.56628583063844928, 9.188101187500006262 ) ) ;
#66950=CARTESIAN_POINT ( 'NONE',  ( 18.62433137644124059, 29.49103043416549141, -8.090169943749479842 ) ) ;
#66954=CARTESIAN_POINT ( 'NONE',  ( 17.03285546273658113, 12.76004757982088655, 5.678558825948272215 ) ) ;
#66966=CARTESIAN_POINT ( 'NONE',  ( 66.67158450822250870, 68.31487490133181950, 4.544081535773483616 ) ) ;
#66977=CARTESIAN_POINT ( 'NONE',  ( 80.35079170152107508, 57.80872192622025807, 16.60075256504293506 ) ) ;
#66982=CARTESIAN_POINT ( 'NONE',  ( 80.93680789325865987, 43.53691286975769970, 9.390856855332286202 ) ) ;
#66993=ORIENTED_EDGE ( 'NONE', *, *, #9491, .T. ) ;
#66996=CARTESIAN_POINT ( 'NONE',  ( 76.00669415887497848, 52.71670032653177174, -16.39932529399118977 ) ) ;
#66999=CARTESIAN_POINT ( 'NONE',  ( 66.57026871561890857, 68.76443072695623471, 4.738950751700697239 ) ) ;
#67003=EDGE_CURVE ( 'NONE', #61768, #63364, #58263, .T. ) ;
#67005=VERTEX_POINT ( 'NONE', #90721 ) ;
#67006=LINE ( 'NONE', #37103, #46384 ) ;
#67008=CARTESIAN_POINT ( 'NONE',  ( 36.78445495848383473, 29.43677371833804202, -10.00000000000000355 ) ) ;
#67016=CARTESIAN_POINT ( 'NONE',  ( 70.83287887816190675, 66.76925213766115519, 10.79410789241422108 ) ) ;
#67018=CARTESIAN_POINT ( 'NONE',  ( 12.92385338608513123, 23.16454794089040092, -10.00000000000000355 ) ) ;
#67035=EDGE_LOOP ( 'NONE', ( #33792, #19459, #20522, #92364 ) ) ;
#67039=CARTESIAN_POINT ( 'NONE',  ( 70.77272717507024424, 71.48227800853128144, -1.166185980175507897 ) ) ;
#67041=CARTESIAN_POINT ( 'NONE',  ( 81.81727448962737981, 41.72775616384396358, -5.614370285570522867 ) ) ;
#67043=CARTESIAN_POINT ( 'NONE',  ( 12.10719531124914283, 12.15404122711131585, 8.090169943749479842 ) ) ;
#67047=B_SPLINE_SURFACE_WITH_KNOTS ( 'NONE', 3, 1, ( 
 ( #37639, #38128 ),
 ( #53351, #44249 ),
 ( #51357, #44740 ),
 ( #83297, #90915 ),
 ( #7246, #76658 ),
 ( #5274, #12895 ),
 ( #89905, #45250 ),
 ( #75674, #29562 ),
 ( #91901, #51874 ),
 ( #97980, #68550 ),
 ( #69046, #60436 ),
 ( #59438, #58935 ),
 ( #82326, #20993 ),
 ( #67057, #20485 ),
 ( #67555, #75185 ),
 ( #82812, #43751 ),
 ( #76186, #5759 ),
 ( #36649, #6259 ),
 ( #98488, #99975 ),
 ( #68055, #98978 ),
 ( #91392, #21956 ),
 ( #29079, #36153 ),
 ( #21464, #99475 ),
 ( #22456, #52850 ),
 ( #45735, #52352 ),
 ( #13861, #83800 ),
 ( #653, #30560 ),
 ( #54842, #69552 ),
 ( #40637, #71572 ),
 ( #32036, #8261 ),
 ( #23942, #78670 ) ),
 .UNSPECIFIED., .F., .F., .F.,
 ( 4, 3, 3, 3, 3, 3, 3, 3, 3, 3, 4 ),
 ( 2, 2 ),
 ( 0.000000000000000000, 0.1122669598086620951, 0.2243161639709352062, 0.3396355846218801489, 0.4553962076584853746, 0.5677860799922156421, 0.6749047109689344515, 0.7773884377078110752, 0.8775581155833879210, 0.9782364162377753525, 1.000000000000000000 ),
 ( 0.000000000000000000, 1.000000000000000000 ),
 .UNSPECIFIED. ) ;
#67049=CARTESIAN_POINT ( 'NONE',  ( 79.23201746742374496, 59.47846325219749986, -16.53522573291430930 ) ) ;
#67055=CARTESIAN_POINT ( 'NONE',  ( 68.40639375505929820, 68.82859656397151582, -7.014046578571599966 ) ) ;
#67057=CARTESIAN_POINT ( 'NONE',  ( 71.47511348553831567, 59.31721159656467535, -15.74457036355328476 ) ) ;
#67058=CARTESIAN_POINT ( 'NONE',  ( 73.50077695243341225, 69.82892408322040012, 9.256215393081268061 ) ) ;
#67059=EDGE_CURVE ( 'NONE', #47030, #95936, #84860, .T. ) ;
#67062=CARTESIAN_POINT ( 'NONE',  ( 69.82829231741662568, 69.33103082410355000, 6.611500818549685299 ) ) ;
#67063=CARTESIAN_POINT ( 'NONE',  ( 66.07805075493222091, 68.50101230898945914, -4.678130671095277471 ) ) ;
#67068=CARTESIAN_POINT ( 'NONE',  ( 28.29779127713939602, 18.19860640527293327, 2.839279412974134775 ) ) ;
#67070=ADVANCED_FACE ( 'NONE', ( #95080 ), #25644, .T. ) ;
#67071=CARTESIAN_POINT ( 'NONE',  ( 80.55977923466276991, 44.53388773495297670, 11.41474457630164707 ) ) ;
#67075=CARTESIAN_POINT ( 'NONE',  ( 68.76218780538779640, 64.26753984631646688, 12.50656271950832732 ) ) ;
#67076=ORIENTED_EDGE ( 'NONE', *, *, #79471, .T. ) ;
#67082=CARTESIAN_POINT ( 'NONE',  ( 71.19507340556562269, 70.62739261389883438, 5.583761667735746670 ) ) ;
#67084=ADVANCED_FACE ( 'NONE', ( #55505 ), #37696, .T. ) ;
#67085=CARTESIAN_POINT ( 'NONE',  ( 71.99345368292625835, 72.28405599045356666, 0.6575919626761969061 ) ) ;
#67087=CARTESIAN_POINT ( 'NONE',  ( 84.79335445094056922, 44.01882294191926093, 6.915891294802152700 ) ) ;
#67092=CARTESIAN_POINT ( 'NONE',  ( 72.75642134338202993, 56.99959235729843954, -16.39691005310872640 ) ) ;
#67095=CARTESIAN_POINT ( 'NONE',  ( 10.74796456262465050, 21.90829794293879473, 10.00000000000000355 ) ) ;
#67098=CARTESIAN_POINT ( 'NONE',  ( 73.99760485042780545, 55.07988560541686951, 16.60354421704504801 ) ) ;
#67099=CARTESIAN_POINT ( 'NONE',  ( 86.40472769894839189, 47.00022269315729773, -10.52150423465796436 ) ) ;
#67106=ORIENTED_EDGE ( 'NONE', *, *, #69031, .T. ) ;
#67118=ORIENTED_EDGE ( 'NONE', *, *, #87242, .F. ) ;
#67119=CARTESIAN_POINT ( 'NONE',  ( 75.75188460778494459, 62.48029762007487165, 15.10107052133506578 ) ) ;
#67122=EDGE_CURVE ( 'NONE', #27651, #87546, #44077, .T. ) ;
#67128=CARTESIAN_POINT ( 'NONE',  ( 71.30800587088177167, 68.37826660670813794, -9.385020971228579256 ) ) ;
#67132=CARTESIAN_POINT ( 'NONE',  ( 76.63225857491576676, 59.44759824736555487, 15.94375019732647125 ) ) ;
#67133=CARTESIAN_POINT ( 'NONE',  ( 6.417452267959404821, 25.74646525600388003, 2.839279412974139660 ) ) ;
#67146=CARTESIAN_POINT ( 'NONE',  ( 86.88629399543513898, 44.27340696768450812, 4.932537521029398242 ) ) ;
#67147=CARTESIAN_POINT ( 'NONE',  ( 88.33748333995926316, 44.07075497373336503, -2.898134731201835290 ) ) ;
#67148=ORIENTED_EDGE ( 'NONE', *, *, #70341, .F. ) ;
#67155=CARTESIAN_POINT ( 'NONE',  ( 85.30422478396575059, 44.62533895320201083, -7.491170275040920146 ) ) ;
#67158=CARTESIAN_POINT ( 'NONE',  ( 87.81592712917142762, 44.13559768126560812, 2.731183658606283871 ) ) ;
#67159=AXIS2_PLACEMENT_3D ( 'NONE', #60470, #37674, #53383 ) ;
#67165=CARTESIAN_POINT ( 'NONE',  ( 85.72965280032694579, 48.53761792183082946, -12.28028246049512973 ) ) ;
#67167=CARTESIAN_POINT ( 'NONE',  ( 86.56321455801250409, 43.53278834282398435, 3.082621468869548575 ) ) ;
#67174=CARTESIAN_POINT ( 'NONE',  ( 78.31378090380852086, 52.71380825594539488, 15.69171095534893290 ) ) ;
#67176=CARTESIAN_POINT ( 'NONE',  ( 80.81957833366946886, 53.31777243922379483, -15.54131231963324744 ) ) ;
#67181=CARTESIAN_POINT ( 'NONE',  ( 84.14087309183582875, 50.46766762800921668, 13.73480842938780278 ) ) ;
#67187=CYLINDRICAL_SURFACE ( 'NONE', #33605, 16.60714546451156792 ) ;
#67189=CARTESIAN_POINT ( 'NONE',  ( 3.104905098483929482, 23.83396525600387506, -2.839279412974133887 ) ) ;
#67200=CARTESIAN_POINT ( 'NONE',  ( 43.33837710268888088, 27.94754757982093096, 5.678558825948272215 ) ) ;
#67202=FACE_BOUND ( 'NONE', #46392, .T. ) ;
#67204=CARTESIAN_POINT ( 'NONE',  ( 16.58664519722142927, 32.68290643055186706, 3.479690158560446702E-15 ) ) ;
#67210=DIRECTION ( 'NONE',  ( 0.3213938048432692374, -0.5566703992264209200, -0.7660444431189770143 ) ) ;
#67214=CARTESIAN_POINT ( 'NONE',  ( 75.04705542663356255, 53.02407537203858823, -16.49187436516719529 ) ) ;
#67217=CARTESIAN_POINT ( 'NONE',  ( 71.81491595147093676, 67.99074982944202361, 10.79843746604593413 ) ) ;
#67220=CARTESIAN_POINT ( 'NONE',  ( 82.89008403434760908, 41.16675059735047171, 0.2050283597234445476 ) ) ;
#67222=CARTESIAN_POINT ( 'NONE',  ( 86.43538639504456000, 43.24186732757627993, 1.603548621781322625 ) ) ;
#67223=VERTEX_POINT ( 'NONE', #10095 ) ;
#67230=CARTESIAN_POINT ( 'NONE',  ( 34.67813663163181559, 40.99752408145594984, 5.678558825948276656 ) ) ;
#67237=CARTESIAN_POINT ( 'NONE',  ( 87.20542010897281671, 46.22683608894070062, -9.058801420718495478 ) ) ;
#67243=CARTESIAN_POINT ( 'NONE',  ( 74.40936191869957383, 60.98710938593095676, -15.30741647548370921 ) ) ;
#67246=CARTESIAN_POINT ( 'NONE',  ( 77.03696703343622687, 62.90724515748721757, -15.26905322870460502 ) ) ;
#67257=CARTESIAN_POINT ( 'NONE',  ( 87.06454106189060838, 46.38688501933356179, -8.729080971554649793 ) ) ;
#67258=EDGE_CURVE ( 'NONE', #18732, #68256, #60570, .T. ) ;
#67272=CARTESIAN_POINT ( 'NONE',  ( 69.39665958681418090, 62.79313245896668860, -13.73716500047468969 ) ) ;
#67278=CARTESIAN_POINT ( 'NONE',  ( 82.61675266362445313, 40.93810794203632497, -3.632981533375318595 ) ) ;
#67281=CARTESIAN_POINT ( 'NONE',  ( 71.98582063699875278, 72.29727681381652360, 3.337216071139553542 ) ) ;
#67284=CARTESIAN_POINT ( 'NONE',  ( 80.94861998693302496, 55.71865610027163029, 16.05787193106602118 ) ) ;
#67285=CARTESIAN_POINT ( 'NONE',  ( 68.99683503679369778, 70.12789505165764581, -3.015407314609216183 ) ) ;
#67288=CARTESIAN_POINT ( 'NONE',  ( 77.72420466810140738, 61.55156736199941037, 16.09483585134336536 ) ) ;
#67295=CARTESIAN_POINT ( 'NONE',  ( 73.43921776615482599, 70.07059797397528200, -9.512040028895288657 ) ) ;
#67297=CARTESIAN_POINT ( 'NONE',  ( 6.214053113703209341, 25.36126292948893379, 6.180339887498949913 ) ) ;
#67298=CARTESIAN_POINT ( 'NONE',  ( 36.03590635313024393, 36.50829794293883168, -10.00000000000000355 ) ) ;
#67299=CARTESIAN_POINT ( 'NONE',  ( 78.26099034771921481, 56.73960120100890236, -16.61664413875233492 ) ) ;
#67301=VECTOR ( 'NONE', #43823, 1000.000000000000000 ) ;
#67302=CARTESIAN_POINT ( 'NONE',  ( 72.01901178328436970, 72.02624153141685781, 2.845887144479070319 ) ) ;
#67308=CARTESIAN_POINT ( 'NONE',  ( 71.90447592081905270, 72.59379857415109427, -1.170934825568553439 ) ) ;
#67310=CARTESIAN_POINT ( 'NONE',  ( 26.01786902700012405, 17.94754757982089899, 5.678558825948272215 ) ) ;
#67313=CARTESIAN_POINT ( 'NONE',  ( 37.67689025969888661, 40.49103043416553049, -8.090169943749479842 ) ) ;
#67317=CARTESIAN_POINT ( 'NONE',  ( 82.18753490691527475, 40.78579184768808830, -0.6546124752527386903 ) ) ;
#67318=CARTESIAN_POINT ( 'NONE',  ( 69.83940448949712732, 67.89019746407828393, -8.846351444184202606 ) ) ;
#67321=VECTOR ( 'NONE', #45490, 1000.000000000000227 ) ;
#67322=EDGE_CURVE ( 'NONE', #38047, #26159, #83603, .T. ) ;
#67324=CARTESIAN_POINT ( 'NONE',  ( 87.74659634842467426, 45.27479573043824246, -7.097702524348068920 ) ) ;
#67337=CARTESIAN_POINT ( 'NONE',  ( 79.07401460044036412, 46.11122150352828442, -12.69419382828625054 ) ) ;
#67343=CARTESIAN_POINT ( 'NONE',  ( 16.63655203261577498, 31.64646525600389637, -2.839279412974133887 ) ) ;
#67344=CARTESIAN_POINT ( 'NONE',  ( 76.27123136624052790, 61.69503254033130446, 15.45961916291305194 ) ) ;
#67345=CARTESIAN_POINT ( 'NONE',  ( 69.85412049919082733, 70.10641299775195989, -4.912549986004115965 ) ) ;
#67356=CARTESIAN_POINT ( 'NONE',  ( 66.01686776079472452, 69.09486339843543590, -2.055003258001108613 ) ) ;
#67357=FACE_OUTER_BOUND ( 'NONE', #56256, .T. ) ;
#67358=CARTESIAN_POINT ( 'NONE',  ( 81.80121988122709809, 55.57996685460995678, 16.31202477726384004 ) ) ;
#67371=ORIENTED_EDGE ( 'NONE', *, *, #99272, .T. ) ;
#67381=CARTESIAN_POINT ( 'NONE',  ( 73.03289083599693754, 63.56301371183312199, -13.95017985831326257 ) ) ;
#67383=CARTESIAN_POINT ( 'NONE',  ( 66.08613192275012693, 68.48609657996226474, -4.736323467610598748 ) ) ;
#67384=ORIENTED_EDGE ( 'NONE', *, *, #35886, .T. ) ;
#67386=CARTESIAN_POINT ( 'NONE',  ( 76.07260682810830588, 51.20992803192402931, -15.61887773062573181 ) ) ;
#67389=B_SPLINE_CURVE_WITH_KNOTS ( 'NONE', 3,
 ( #51521, #4944, #21146, #2572, #64862, #52025, #82965, #13539, #35823, #95809, #97652, #66718, #26363, #58604, #7404, #53505 ),
 .UNSPECIFIED., .F., .F.,
 ( 4, 1, 2, 2, 2, 1, 2, 2, 4 ),
 ( 0.000000000000000000, 0.1249999999999996947, 0.1874999999999995837, 0.2499999999999995004, 0.5000000000000003331, 0.6250000000000009992, 0.6874999999999995559, 0.7499999999999981126, 1.000000000000000000 ),
 .UNSPECIFIED. ) ;
#67393=AXIS2_PLACEMENT_3D ( 'NONE', #6002, #60672, #97725 ) ;
#67394=ORIENTED_EDGE ( 'NONE', *, *, #36945, .T. ) ;
#67397=EDGE_LOOP ( 'NONE', ( #30206, #30114, #5569, #33075 ) ) ;
#67398=CARTESIAN_POINT ( 'NONE',  ( 88.14062891587492743, 44.42319542341160599, 4.630203861778127816 ) ) ;
#67402=CARTESIAN_POINT ( 'NONE',  ( 79.32006575253170411, 59.07617305244814787, -16.22726605023456870 ) ) ;
#67404=VERTEX_POINT ( 'NONE', #84512 ) ;
#67405=CARTESIAN_POINT ( 'NONE',  ( 76.73836869982963549, 55.83238297101823377, 16.17114945624216560 ) ) ;
#67408=CARTESIAN_POINT ( 'NONE',  ( 79.87836239028537477, 47.43443509841839756, 13.25449791563737456 ) ) ;
#67412=CARTESIAN_POINT ( 'NONE',  ( 71.33706390578697665, 71.87455509392472663, 0.2141773752858076585 ) ) ;
#67413=FACE_BOUND ( 'NONE', #3241, .T. ) ;
#67414=CARTESIAN_POINT ( 'NONE',  ( 25.96360177180014972, 20.15404122711134249, 8.090169943749479842 ) ) ;
#67423=CARTESIAN_POINT ( 'NONE',  ( 66.54077760113520412, 67.98430679024006906, -6.561883603421821753 ) ) ;
#67428=CARTESIAN_POINT ( 'NONE',  ( 29.26302659224649361, 17.86426979415090699, -3.090169943749474069 ) ) ;
#67435=CARTESIAN_POINT ( 'NONE',  ( 84.43598368786032893, 47.43396312368651024, 11.99281069980813896 ) ) ;
#67447=EDGE_CURVE ( 'NONE', #60091, #55813, #69013, .T. ) ;
#67449=CARTESIAN_POINT ( 'NONE',  ( 37.59133656659163591, 37.10171378149920685, 9.188101187500008038 ) ) ;
#67453=CARTESIAN_POINT ( 'NONE',  ( 74.14312167556930433, 66.30466486950707861, 1.224646799147354045E-15 ) ) ;
#67456=CARTESIAN_POINT ( 'NONE',  ( 17.58072690530697813, 12.01110640527291373, 2.839279412974134775 ) ) ;
#67457=CARTESIAN_POINT ( 'NONE',  ( 71.96852905813888412, 72.61068693531508700, 1.394764389614176148 ) ) ;
#67458=CARTESIAN_POINT ( 'NONE',  ( 82.77428392532827672, 53.84857159627674150, 15.43231797370390623 ) ) ;
#67461=ORIENTED_EDGE ( 'NONE', *, *, #95893, .T. ) ;
#67465=CARTESIAN_POINT ( 'NONE',  ( 74.96743300375965191, 53.32485851529158793, -16.04568551637340335 ) ) ;
#67466=CARTESIAN_POINT ( 'NONE',  ( 81.34506373925208322, 42.08414435209094506, 7.957546939141312947 ) ) ;
#67467=ORIENTED_EDGE ( 'NONE', *, *, #88646, .F. ) ;
#67468=DIRECTION ( 'NONE',  ( -0.8660254037844379305, -0.5000000000000014433, -0.000000000000000000 ) ) ;
#67470=CARTESIAN_POINT ( 'NONE',  ( 81.81010722587693351, 59.02505635547797169, -0.4806308479691593916 ) ) ;
#67479=CARTESIAN_POINT ( 'NONE',  ( 80.54858391640954096, 57.70359709413047966, 16.24103893543703592 ) ) ;
#67483=CARTESIAN_POINT ( 'NONE',  ( 81.27023270499687158, 43.21841413807894838, 9.592188031249742508 ) ) ;
#67486=CARTESIAN_POINT ( 'NONE',  ( 75.02043720394767945, 65.61285698292792290, 13.53072932596785272 ) ) ;
#67494=ORIENTED_EDGE ( 'NONE', *, *, #29269, .F. ) ;
#67495=ORIENTED_EDGE ( 'NONE', *, *, #71902, .T. ) ;
#67496=CARTESIAN_POINT ( 'NONE',  ( 77.87286301834419078, 52.13848254994933740, -16.08542584302312051 ) ) ;
#67497=CARTESIAN_POINT ( 'NONE',  ( 87.34409271548551601, 43.66013200155327922, 0.5981997646405022850 ) ) ;
#67498=DIRECTION ( 'NONE',  ( -0.8660254037844378194, -0.5000000000000013323, -0.000000000000000000 ) ) ;
#67499=CARTESIAN_POINT ( 'NONE',  ( 82.50452235219570696, 53.86480448276187616, 15.85105177732746817 ) ) ;
#67504=ORIENTED_EDGE ( 'NONE', *, *, #36705, .T. ) ;
#67505=CARTESIAN_POINT ( 'NONE',  ( 77.17331351098810899, 56.95370604848049823, -16.18904554513164484 ) ) ;
#67514=VERTEX_POINT ( 'NONE', #85004 ) ;
#67518=CARTESIAN_POINT ( 'NONE',  ( 78.96518011614999466, 46.19984413241925836, 12.79727321583966493 ) ) ;
#67520=CARTESIAN_POINT ( 'NONE',  ( 78.63357992691169329, 55.03961015548562585, -16.49924009853327078 ) ) ;
#67531=CARTESIAN_POINT ( 'NONE',  ( 84.32777827622054190, 50.66816837149428210, 13.78787580221864140 ) ) ;
#67536=EDGE_LOOP ( 'NONE', ( #36706, #91808, #61755, #17130 ) ) ;
#67544=CARTESIAN_POINT ( 'NONE',  ( 68.83366497510655790, 64.72209559286066849, -12.18477093088157481 ) ) ;
#67548=VERTEX_POINT ( 'NONE', #86531 ) ;
#67549=DIRECTION ( 'NONE',  ( -0.8660254037844378194, -0.5000000000000013323, -0.000000000000000000 ) ) ;
#67551=CARTESIAN_POINT ( 'NONE',  ( 84.55206357306229847, 46.71456743556125701, -11.30110183101671062 ) ) ;
#67553=CARTESIAN_POINT ( 'NONE',  ( 7.019590965729775256, 22.79103043416547081, 8.090169943749478065 ) ) ;
#67555=CARTESIAN_POINT ( 'NONE',  ( 71.48584797926407930, 59.35514066858884519, -15.73530635236135922 ) ) ;
#67560=CARTESIAN_POINT ( 'NONE',  ( 72.48211761085248384, 57.49817692938951552, 15.81360302781613036 ) ) ;
#67563=EDGE_LOOP ( 'NONE', ( #72345, #64357, #43910, #84239 ) ) ;
#67568=CARTESIAN_POINT ( 'NONE',  ( 25.16147942602835386, 23.03085787977763843, 9.188101187500006262 ) ) ;
#67575=CARTESIAN_POINT ( 'NONE',  ( 68.79717273036834513, 64.27923393059754176, 12.51298953402340963 ) ) ;
#67577=CARTESIAN_POINT ( 'NONE',  ( 80.34760537404680747, 47.87480626140324347, 13.91709158461522655 ) ) ;
#67582=ORIENTED_EDGE ( 'NONE', *, *, #91875, .F. ) ;
#67584=AXIS2_PLACEMENT_3D ( 'NONE', #80891, #3360, #10438 ) ;
#67586=CARTESIAN_POINT ( 'NONE',  ( 71.78242053751054641, 72.53632993589367572, 0.9980050652678308376 ) ) ;
#67587=B_SPLINE_SURFACE_WITH_KNOTS ( 'NONE', 3, 1, ( 
 ( #46499, #84073 ),
 ( #53116, #85576 ),
 ( #54096, #15599 ),
 ( #54594, #62197 ),
 ( #420, #31309 ),
 ( #61208, #29820 ),
 ( #76438, #77933 ),
 ( #77435, #69810 ),
 ( #93148, #16120 ),
 ( #23205, #8524 ),
 ( #62701, #39393 ),
 ( #92175, #14626 ),
 ( #22725, #7507 ),
 ( #7013, #38404 ),
 ( #78437, #24223 ),
 ( #37898, #100239 ),
 ( #99234, #68806 ),
 ( #70310, #923 ),
 ( #69317, #55103 ),
 ( #30823, #47510 ),
 ( #86090, #37405 ),
 ( #68311, #91652 ),
 ( #22218, #33318 ),
 ( #64217, #1929 ),
 ( #39890, #56097 ),
 ( #10031, #51373 ),
 ( #32815, #87090 ),
 ( #56616, #63720 ),
 ( #48007, #80467 ),
 ( #66585, #88084 ),
 ( #95168, #87600 ) ),
 .UNSPECIFIED., .F., .F., .F.,
 ( 4, 3, 3, 3, 3, 3, 3, 3, 3, 3, 4 ),
 ( 2, 2 ),
 ( 0.000000000000000000, 0.1333490885032357909, 0.3007194338854210502, 0.4699862290245036545, 0.5844252810809178467, 0.6686540514502550270, 0.7354980260655467061, 0.8028463152565693539, 0.8633854507757410257, 0.9437142632667440134, 1.000000000000000000 ),
 ( 0.000000000000000000, 1.000000000000000000 ),
 .UNSPECIFIED. ) ;
#67588=DIRECTION ( 'NONE',  ( 0.5000000000000013323, -0.8660254037844378194, 0.000000000000000000 ) ) ;
#67591=CARTESIAN_POINT ( 'NONE',  ( 67.98269450004784176, 69.23742185243530400, 4.145183063120581934 ) ) ;
#67595=CARTESIAN_POINT ( 'NONE',  ( 7.184267760421183091, 27.08080186712590631, -3.090169943749475845 ) ) ;
#67596=CARTESIAN_POINT ( 'NONE',  ( 82.48921279030038534, 44.14273019941255427, 9.857891367207361810 ) ) ;
#67599=CARTESIAN_POINT ( 'NONE',  ( 86.55406513359314147, 47.25665231443431935, -10.69898602647500496 ) ) ;
#67600=CARTESIAN_POINT ( 'NONE',  ( 81.57461113938337860, 45.47094929192444113, -11.08393736095532844 ) ) ;
#67612=B_SPLINE_SURFACE_WITH_KNOTS ( 'NONE', 3, 1, ( 
 ( #70943, #55208 ),
 ( #61316, #92279 ),
 ( #68918, #78544 ),
 ( #86189, #39009 ),
 ( #530, #93261 ),
 ( #38515, #77019 ),
 ( #16725, #22826 ),
 ( #45611, #40 ),
 ( #47617, #7623 ),
 ( #30925, #9132 ),
 ( #40003, #7121 ),
 ( #41001, #19257 ),
 ( #34425, #80068 ),
 ( #11152, #95286 ),
 ( #32920, #26829 ),
 ( #49620, #42502 ),
 ( #96262, #25846 ),
 ( #17740, #73439 ),
 ( #95782, #18736 ),
 ( #71445, #49134 ),
 ( #34907, #80573 ),
 ( #57708, #11643 ),
 ( #42021, #2033 ),
 ( #4023, #33948 ),
 ( #71943, #65807 ),
 ( #96767, #63824 ),
 ( #79066, #55695 ),
 ( #56723, #94759 ),
 ( #81077, #40510 ),
 ( #25323, #56209 ),
 ( #26334, #87705 ) ),
 .UNSPECIFIED., .F., .F., .F.,
 ( 4, 3, 3, 3, 3, 3, 3, 3, 3, 3, 4 ),
 ( 2, 2 ),
 ( 0.000000000000000000, 0.1122669598086724063, 0.2243161639709572719, 0.3396355846218986341, 0.4553962076585058583, 0.5677860799922284096, 0.6749047109689497725, 0.7773884377078336128, 0.8775581155834173419, 0.9782364162377894523, 1.000000000000000000 ),
 ( 0.000000000000000000, 1.000000000000000000 ),
 .UNSPECIFIED. ) ;
#67616=CARTESIAN_POINT ( 'NONE',  ( 88.28323348104321155, 43.74655523625713016, 0.1991997974169892882 ) ) ;
#67618=CARTESIAN_POINT ( 'NONE',  ( 81.66405316814116588, 51.22542360033385478, 14.71426855131227462 ) ) ;
#67620=CARTESIAN_POINT ( 'NONE',  ( 76.14474959763187201, 64.73882662526121123, 14.33715962598121152 ) ) ;
#67621=ORIENTED_EDGE ( 'NONE', *, *, #14843, .F. ) ;
#67625=CARTESIAN_POINT ( 'NONE',  ( 82.57676729861134390, 54.19068042909008653, -15.92587557605581061 ) ) ;
#67628=CARTESIAN_POINT ( 'NONE',  ( 66.41068231923046028, 68.91878406202458507, 0.07809209811752516883 ) ) ;
#67630=CARTESIAN_POINT ( 'NONE',  ( 12.38457448260035143, 9.011106405272903075, 2.839279412974134775 ) ) ;
#67640=PLANE ( 'NONE',  #2061 ) ;
#67644=CARTESIAN_POINT ( 'NONE',  ( 77.72205534048291042, 61.52847525230062331, 16.09962475150208405 ) ) ;
#67647=CARTESIAN_POINT ( 'NONE',  ( 70.09145387123612636, 63.58422643240743355, -12.93064994232666010 ) ) ;
#67656=CARTESIAN_POINT ( 'NONE',  ( 84.43667057297049894, 44.63661754160224149, -8.257540914285325329 ) ) ;
#67657=AXIS2_PLACEMENT_3D ( 'NONE', #11982, #49972, #96116 ) ;
#67662=ORIENTED_EDGE ( 'NONE', *, *, #37885, .T. ) ;
#67667=EDGE_CURVE ( 'NONE', #5574, #37857, #55714, .T. ) ;
#67670=CARTESIAN_POINT ( 'NONE',  ( 81.98204644731730184, 41.14170830008083612, -5.380964918418897902 ) ) ;
#67672=CARTESIAN_POINT ( 'NONE',  ( 72.10617024684209753, 72.18421392457030095, 4.031754617348218162 ) ) ;
#67678=CARTESIAN_POINT ( 'NONE',  ( 79.16712529945354504, 57.32610516721600646, 16.21374135531271321 ) ) ;
#67679=AXIS2_PLACEMENT_3D ( 'NONE', #93137, #62689, #38393 ) ;
#67681=CARTESIAN_POINT ( 'NONE',  ( 38.67678797688638070, 22.73415679381825072, -6.890680421881970419E-14 ) ) ;
#67687=CARTESIAN_POINT ( 'NONE',  ( 84.29444876203692161, 50.65533303003044807, 13.79152508277374345 ) ) ;
#67696=CARTESIAN_POINT ( 'NONE',  ( 9.878523645489616811, 21.10171378149917487, 9.188101187500008038 ) ) ;
#67698=EDGE_CURVE ( 'NONE', #11479, #38046, #31131, .T. ) ;
#67699=CARTESIAN_POINT ( 'NONE',  ( 79.14312167556931854, 57.64441083166269664, 0.000000000000000000 ) ) ;
#67706=CARTESIAN_POINT ( 'NONE',  ( 45.61829935282815995, 28.19860640527296525, 2.839279412974134775 ) ) ;
#67710=CARTESIAN_POINT ( 'NONE',  ( 17.13451663979182626, 31.93396525600390135, 2.839279412974139660 ) ) ;
#67716=EDGE_LOOP ( 'NONE', ( #29769, #65391, #55663, #41060 ) ) ;
#67717=CARTESIAN_POINT ( 'NONE',  ( 70.44740873159727812, 60.97318155419277019, 14.95046560365730137 ) ) ;
#67727=CARTESIAN_POINT ( 'NONE',  ( 66.05805092528737532, 68.60151024935468911, 4.334430423793950382 ) ) ;
#67735=CARTESIAN_POINT ( 'NONE',  ( 88.11801461435689475, 44.35549720747543745, -4.463913325698411150 ) ) ;
#67739=CARTESIAN_POINT ( 'NONE',  ( 37.18479240120036167, 39.65586893147759895, -7.433330006724137462 ) ) ;
#67740=CARTESIAN_POINT ( 'NONE',  ( 78.87587414727704527, 58.57443402504730301, -16.19777088011071342 ) ) ;
#67742=CARTESIAN_POINT ( 'NONE',  ( 87.66739418633859771, 45.39771433737033135, 6.570038411687281865 ) ) ;
#67745=CARTESIAN_POINT ( 'NONE',  ( 72.07243891101380484, 72.25875221884653854, -1.540673756851268283 ) ) ;
#67751=CARTESIAN_POINT ( 'NONE',  ( 68.24228953960120236, 68.25579693966338368, 7.841510002861836526 ) ) ;
#67753=CARTESIAN_POINT ( 'NONE',  ( 82.10540399970709302, 40.78094143542895011, 1.224565905253431675 ) ) ;
#67755=CARTESIAN_POINT ( 'NONE',  ( 77.05240863693448716, 63.46827552167501096, -15.45063268884610785 ) ) ;
#67760=CARTESIAN_POINT ( 'NONE',  ( 39.54951596113196644, 25.76004757982093096, 5.678558825948272215 ) ) ;
#67766=CARTESIAN_POINT ( 'NONE',  ( 73.95565718806818722, 68.30423517461105121, -11.66005733018688773 ) ) ;
#67769=CARTESIAN_POINT ( 'NONE',  ( 34.66168140297119038, 20.41603393254328580, -1.583844403245396437 ) ) ;
#67774=EDGE_LOOP ( 'NONE', ( #59225, #99127, #84373, #90181 ) ) ;
#67778=CARTESIAN_POINT ( 'NONE',  ( 82.95635226107660287, 46.18328785982301810, 11.04540840999154661 ) ) ;
#67784=CARTESIAN_POINT ( 'NONE',  ( 71.32140601477664177, 62.18330075258982959, 14.10657701148000065 ) ) ;
#67785=CARTESIAN_POINT ( 'NONE',  ( 82.59165424625105345, 40.92964489041076348, -3.656265280277670282 ) ) ;
#67791=CARTESIAN_POINT ( 'NONE',  ( 84.25902073258765768, 45.00982432294706825, 8.916331552282562356 ) ) ;
#67794=CARTESIAN_POINT ( 'NONE',  ( 71.99494277328302871, 70.73507547392100037, -6.404330814823480544 ) ) ;
#67795=AXIS2_PLACEMENT_3D ( 'NONE', #55051, #39340, #69759 ) ;
#67800=DIRECTION ( 'NONE',  ( 0.3213938048432692374, -0.5566703992264209200, -0.7660444431189770143 ) ) ;
#67804=CARTESIAN_POINT ( 'NONE',  ( 66.10780414051450293, 68.63670250712272036, 1.777645618418523865 ) ) ;
#67806=( NAMED_UNIT ( * ) PLANE_ANGLE_UNIT ( ) SI_UNIT ( $, .RADIAN. ) );
#67807=CARTESIAN_POINT ( 'NONE',  ( 43.29939952211008602, 27.12755873383629890, -6.180339887498949025 ) ) ;
#67810=CARTESIAN_POINT ( 'NONE',  ( 71.97049335289784722, 72.00104994887270493, 2.833700686527681256 ) ) ;
#67819=CARTESIAN_POINT ( 'NONE',  ( 71.59149729713742261, 72.39908022291972145, -1.330894502438451754 ) ) ;
#67821=VECTOR ( 'NONE', #51887, 1000.000000000000114 ) ;
#67822=CARTESIAN_POINT ( 'NONE',  ( 24.12224894148702248, 22.43085787977763701, -9.188101187500008038 ) ) ;
#67825=CARTESIAN_POINT ( 'NONE',  ( 43.71265818875933462, 33.43677371833804557, -10.00000000000000355 ) ) ;
#67828=CARTESIAN_POINT ( 'NONE',  ( 75.71473607284134744, 57.60838419999664239, 16.52739276483602993 ) ) ;
#67834=EDGE_CURVE ( 'NONE', #14298, #121, #51364, .T. ) ;
#67835=CARTESIAN_POINT ( 'NONE',  ( 71.47791206682282450, 72.34364865201936823, -1.216664393387151488 ) ) ;
#67841=ORIENTED_EDGE ( 'NONE', *, *, #87685, .T. ) ;
#67842=CARTESIAN_POINT ( 'NONE',  ( 76.67567146729663818, 63.34086528488000312, -15.41964329106467346 ) ) ;
#67844=B_SPLINE_CURVE_WITH_KNOTS ( 'NONE', 3,
 ( #88678, #19251, #88181, #34416, #43499, #3540, #42014, #72947, #11633, #58209, #95772, #65317, #66315, #64319, #96256, #50116, #96757, #26328, #42986, #89186, #56714, #87697, #81070, #97248, #64827, #57202, #51095, #4508, #26821, #57702, #42494, #80061, #73427, #72447, #95277, #18229, #58689, #27814, #4016, #73924, #89663, #3053, #19735, #65800, #12120, #50601 ),
 .UNSPECIFIED., .F., .F.,
 ( 4, 1, 2, 2, 1, 2, 2, 1, 1, 2, 2, 1, 1, 2, 2, 1, 1, 2, 2, 1, 1, 1, 2, 2, 1, 1, 1, 2, 2, 4 ),
 ( 0.000000000000000000, 0.06250000000001718070, 0.09375000000002577105, 0.1250000000000343614, 0.1875000000000512090, 0.2187500000000597578, 0.2500000000000683342, 0.3125000000000877076, 0.3437500000000959788, 0.3593750000001001976, 0.3750000000001043610, 0.4375000000001160738, 0.4687500000001217915, 0.4843750000001234568, 0.5000000000001250111, 0.5625000000001235678, 0.5937500000001214584, 0.6093750000001189049, 0.6250000000001162404, 0.6875000000000976996, 0.7187500000000870415, 0.7343750000000816014, 0.7421875000000790479, 0.7500000000000763833, 0.8125000000000579536, 0.8437500000000504041, 0.8593750000000451861, 0.8671875000000426326, 0.8750000000000400791, 1.000000000000000000 ),
 .UNSPECIFIED. ) ;
#67848=CARTESIAN_POINT ( 'NONE',  ( 79.35516988872859656, 46.20647275665685783, -13.25012323394358127 ) ) ;
#67850=CARTESIAN_POINT ( 'NONE',  ( 73.10697178893200032, 70.59305037885800971, -7.867401265066643390 ) ) ;
#67854=CARTESIAN_POINT ( 'NONE',  ( 23.25741983583088413, 25.37878583063841376, 9.188101187500006262 ) ) ;
#67855=CARTESIAN_POINT ( 'NONE',  ( 79.74231254351767006, 44.89165149099596874, 11.47344340298346133 ) ) ;
#67856=CARTESIAN_POINT ( 'NONE',  ( 72.34276783205245920, 70.28584662377375025, -7.644984185308641322 ) ) ;
#67859=CARTESIAN_POINT ( 'NONE',  ( 76.38954935904880017, 53.24951976528166853, 16.44149648979542278 ) ) ;
#67868=CARTESIAN_POINT ( 'NONE',  ( 81.62315923969183018, 55.76054528319124159, 16.35706999678057727 ) ) ;
#67870=ADVANCED_FACE ( 'NONE', ( #79791 ), #72164, .T. ) ;
#67872=VECTOR ( 'NONE', #70817, 1000.000000000000114 ) ;
#67880=ORIENTED_EDGE ( 'NONE', *, *, #82939, .F. ) ;
#67886=CARTESIAN_POINT ( 'NONE',  ( 81.67557174052036828, 55.75159692325900096, 15.99231456053679423 ) ) ;
#67892=B_SPLINE_SURFACE_WITH_KNOTS ( 'NONE', 3, 1, ( 
 ( #96128, #10487 ),
 ( #42363, #48991 ),
 ( #65671, #18093 ),
 ( #34283, #81921 ),
 ( #74313, #4895 ),
 ( #41368, #79927 ),
 ( #56577, #11996 ),
 ( #73296, #27192 ),
 ( #97130, #18597 ),
 ( #34770, #87564 ),
 ( #66672, #58081 ),
 ( #72306, #2915 ),
 ( #33807, #89060 ),
 ( #65180, #72817 ),
 ( #64691, #95643 ),
 ( #26682, #26190 ),
 ( #3408, #57068 ),
 ( #27696, #58566 ),
 ( #19613, #88049 ),
 ( #42853, #4378 ),
 ( #89537, #88543 ),
 ( #80432, #81424 ),
 ( #50471, #19109 ),
 ( #49985, #49476 ),
 ( #80941, #11509 ),
 ( #35278, #11005 ),
 ( #20098, #66184 ),
 ( #50969, #12497 ),
 ( #41879, #35779 ),
 ( #25697, #45357 ),
 ( #36269, #13978 ) ),
 .UNSPECIFIED., .F., .F., .F.,
 ( 4, 3, 3, 3, 3, 3, 3, 3, 3, 3, 4 ),
 ( 2, 2 ),
 ( 0.000000000000000000, 0.1122669598086675907, 0.2243161639709637112, 0.3396355846219057395, 0.4553962076585009733, 0.5677860799922324064, 0.6749047109689443324, 0.7773884377078320584, 0.8775581155834342173, 0.9782364162377927830, 1.000000000000000000 ),
 ( 0.000000000000000000, 1.000000000000000000 ),
 .UNSPECIFIED. ) ;
#67894=ORIENTED_EDGE ( 'NONE', *, *, #65995, .T. ) ;
#67904=CARTESIAN_POINT ( 'NONE',  ( 81.28967588850363768, 44.30488066837197181, -10.06605756411466857 ) ) ;
#67905=CARTESIAN_POINT ( 'NONE',  ( 73.03327713030915902, 67.29942500083180335, -12.06190433575985210 ) ) ;
#67907=EDGE_CURVE ( 'NONE', #90329, #61768, #26690, .T. ) ;
#67908=CARTESIAN_POINT ( 'NONE',  ( 79.51860058571794809, 59.43534202413220413, -16.20610000061713407 ) ) ;
#67910=CARTESIAN_POINT ( 'NONE',  ( 71.09310640586875252, 67.27851065979278644, -10.44888890291803030 ) ) ;
#67912=CARTESIAN_POINT ( 'NONE',  ( 75.84856439504059722, 51.76521084193598909, 15.76359423700355755 ) ) ;
#67914=CARTESIAN_POINT ( 'NONE',  ( 72.62875853510576007, 71.42134003127335973, -5.810135019581663229 ) ) ;
#67915=CARTESIAN_POINT ( 'NONE',  ( 80.57406551557809848, 49.71488727638417515, 14.27527881381214847 ) ) ;
#67922=CARTESIAN_POINT ( 'NONE',  ( 19.73933908736162124, 30.13478043621388380, 8.090169943749478065 ) ) ;
#67927=CARTESIAN_POINT ( 'NONE',  ( 72.29835728126460026, 71.99361178985304832, -3.639781104770197562 ) ) ;
#67934=CARTESIAN_POINT ( 'NONE',  ( 66.90338203151232221, 68.17684508661041320, -6.595631787949806757 ) ) ;
#67935=CARTESIAN_POINT ( 'NONE',  ( 72.95589830849367274, 70.34902050982091737, -8.120948148125345156 ) ) ;
#67939=CARTESIAN_POINT ( 'NONE',  ( 24.66009930550170282, 22.43677371833801715, -10.00000000000000355 ) ) ;
#67940=CARTESIAN_POINT ( 'NONE',  ( 85.45224931747254971, 49.07960547787612882, 12.36068907126763960 ) ) ;
#67942=CARTESIAN_POINT ( 'NONE',  ( 71.91831898124014799, 71.71822762647316551, -3.866383333238705866 ) ) ;
#67950=CARTESIAN_POINT ( 'NONE',  ( 41.28778705816291961, 32.03677371833806120, 10.00000000000000533 ) ) ;
#67954=CARTESIAN_POINT ( 'NONE',  ( 37.43858582280105907, 33.56628583063844218, 9.188101187500006262 ) ) ;
#67962=CARTESIAN_POINT ( 'NONE',  ( 18.06126741312425921, 22.37878583063840310, 9.188101187500006262 ) ) ;
#67964=CARTESIAN_POINT ( 'NONE',  ( 71.70303330742534342, 59.04301762528319131, 15.35811543448661531 ) ) ;
#67968=CARTESIAN_POINT ( 'NONE',  ( 88.28714907786486776, 44.35112667690796684, 2.372838034520684314 ) ) ;
#67971=CARTESIAN_POINT ( 'NONE',  ( 68.86429500837576256, 70.35746111282902859, -0.7754140821421253715 ) ) ;
#67972=CARTESIAN_POINT ( 'NONE',  ( 24.85415417228448121, 26.30066082961422680, -10.00000000000000533 ) ) ;
#67979=ORIENTED_EDGE ( 'NONE', *, *, #44364, .F. ) ;
#67981=CARTESIAN_POINT ( 'NONE',  ( 70.27209832060933081, 65.59710146439343248, 12.14989064463910040 ) ) ;
#67982=CARTESIAN_POINT ( 'NONE',  ( 80.32304696881857353, 58.04909235870844952, 16.26133398640363126 ) ) ;
#67989=CARTESIAN_POINT ( 'NONE',  ( 74.84928291413068280, 64.80482755438514175, 13.90247044424336309 ) ) ;
#67997=CARTESIAN_POINT ( 'NONE',  ( 33.00035307926291495, 37.79103043416552055, 8.090169943749478065 ) ) ;
#68000=CARTESIAN_POINT ( 'NONE',  ( 73.61712177582347749, 69.75295271933504182, 9.424901393032142138 ) ) ;
#68001=CARTESIAN_POINT ( 'NONE',  ( 81.82006362146523770, 42.66096406068295011, -7.441249945456725357 ) ) ;
#68010=CARTESIAN_POINT ( 'NONE',  ( 68.04803862442108198, 70.41495816557659282, 0.2082392626603555841 ) ) ;
#68011=CARTESIAN_POINT ( 'NONE',  ( 71.47791206682282450, 72.34364865201936823, -1.216664393387151488 ) ) ;
#68012=CARTESIAN_POINT ( 'NONE',  ( 39.81344631580554250, 23.39040679176985904, -6.890680421881970419E-14 ) ) ;
#68022=CARTESIAN_POINT ( 'NONE',  ( 73.69427750731760796, 56.72192345538155678, -16.50807356290637173 ) ) ;
#68028=CARTESIAN_POINT ( 'NONE',  ( 72.40589440182066028, 71.76200285602328677, 5.709577571112527394 ) ) ;
#68033=CARTESIAN_POINT ( 'NONE',  ( 66.85524610400479162, 67.34209505064850987, -6.990925417236247164 ) ) ;
#68038=ORIENTED_EDGE ( 'NONE', *, *, #3598, .T. ) ;
#68041=CARTESIAN_POINT ( 'NONE',  ( 71.11777852545861833, 71.64480956778183440, -1.649610073217940398 ) ) ;
#68043=CARTESIAN_POINT ( 'NONE',  ( 81.69476477490047728, 41.61625632775264449, -5.521120823311375325 ) ) ;
#68053=CARTESIAN_POINT ( 'NONE',  ( 6.688470478837179378, 19.56454794089038884, 10.00000000000000355 ) ) ;
#68055=CARTESIAN_POINT ( 'NONE',  ( 71.59361115369081574, 59.50488489875972675, -15.70950865668593188 ) ) ;
#68056=CARTESIAN_POINT ( 'NONE',  ( 73.17035075335006411, 69.75913569003169812, 9.110019559117217725 ) ) ;
#68060=CARTESIAN_POINT ( 'NONE',  ( 73.60341520791058656, 55.46590081124723071, 16.11001259655113316 ) ) ;
#68062=CARTESIAN_POINT ( 'NONE',  ( 66.33274517095223644, 68.13410765588996298, -4.505544708085248651 ) ) ;
#68067=CARTESIAN_POINT ( 'NONE',  ( 30.02984208470827454, 19.19860640527293327, 2.839279412974134775 ) ) ;
#68069=CARTESIAN_POINT ( 'NONE',  ( 83.83309058964263727, 51.93283190383716885, -14.92096955093740362 ) ) ;
#68071=CARTESIAN_POINT ( 'NONE',  ( 84.08513284186659575, 41.35086568230796189, -1.059521581035436366 ) ) ;
#68072=CARTESIAN_POINT ( 'NONE',  ( 74.72173318163055455, 67.07206250228034605, 12.96729955693541569 ) ) ;
#68074=CARTESIAN_POINT ( 'NONE',  ( 69.13163807604178146, 64.30638122866986350, 12.00391912781525505 ) ) ;
#68076=CARTESIAN_POINT ( 'NONE',  ( 79.70677143361787387, 46.01134058561531504, 12.98241517792750699 ) ) ;
#68081=CARTESIAN_POINT ( 'NONE',  ( 6.414422030351863313, 19.10171378149916777, 9.188101187500008038 ) ) ;
#68085=CARTESIAN_POINT ( 'NONE',  ( 75.40537576526305941, 53.18750470143674391, 16.48738048042240223 ) ) ;
#68086=CARTESIAN_POINT ( 'NONE',  ( 71.47384123275854506, 72.35069954344791654, 1.100233114707650506 ) ) ;
#68089=FACE_OUTER_BOUND ( 'NONE', #34126, .T. ) ;
#68094=CARTESIAN_POINT ( 'NONE',  ( 7.357472841178069878, 27.18080186712591484, 3.090169943749475401 ) ) ;
#68095=CARTESIAN_POINT ( 'NONE',  ( 84.01508409052884474, 48.27837738685627045, 12.82889063469658630 ) ) ;
#68098=EDGE_CURVE ( 'NONE', #45306, #51277, #87226, .T. ) ;
#68100=CARTESIAN_POINT ( 'NONE',  ( 86.60342109795770682, 45.00234098353818979, -6.966275957478193170 ) ) ;
#68101=ORIENTED_EDGE ( 'NONE', *, *, #95869, .T. ) ;
#68103=CARTESIAN_POINT ( 'NONE',  ( 79.33144427914538710, 59.81174478577791831, -16.15603203001268540 ) ) ;
#68105=CARTESIAN_POINT ( 'NONE',  ( 69.33797530432867973, 62.88103157235104845, 13.66491503495263871 ) ) ;
#68110=CARTESIAN_POINT ( 'NONE',  ( 81.74299993193413627, 42.33909358938161205, -7.997327082880324234 ) ) ;
#68112=ORIENTED_EDGE ( 'NONE', *, *, #38188, .T. ) ;
#68114=CARTESIAN_POINT ( 'NONE',  ( 81.30167161776530804, 49.59675704108522609, 14.04897986542503041 ) ) ;
#68116=CARTESIAN_POINT ( 'NONE',  ( 68.59458835999485871, 68.94540003394581618, 5.879567767820735646 ) ) ;
#68122=CARTESIAN_POINT ( 'NONE',  ( 68.41665967678483184, 68.37445157850072519, -6.807967649046275049 ) ) ;
#68125=CARTESIAN_POINT ( 'NONE',  ( 77.22649460905378760, 63.31555197798695644, 15.15381191669832184 ) ) ;
#68126=CARTESIAN_POINT ( 'NONE',  ( 13.54711677929152636, 28.79752408145592213, -5.678558825948271327 ) ) ;
#68127=VERTEX_POINT ( 'NONE', #80034 ) ;
#68135=FACE_OUTER_BOUND ( 'NONE', #96942, .T. ) ;
#68141=CARTESIAN_POINT ( 'NONE',  ( 70.41420743703629626, 63.52079831010913580, -13.09409908041479831 ) ) ;
#68145=CARTESIAN_POINT ( 'NONE',  ( 82.87333762504050583, 53.62476702604639200, -15.35949376849550596 ) ) ;
#68151=CARTESIAN_POINT ( 'NONE',  ( 76.11661262897267477, 65.38883171293761620, 14.43021505105785174 ) ) ;
#68154=ORIENTED_EDGE ( 'NONE', *, *, #79614, .T. ) ;
#68161=CARTESIAN_POINT ( 'NONE',  ( 84.95073541789081162, 48.44820618829425740, 12.09123390135387766 ) ) ;
#68166=CARTESIAN_POINT ( 'NONE',  ( 80.74974841587442143, 43.27611110060701805, 10.01619596027649806 ) ) ;
#68168=DIRECTION ( 'NONE',  ( -0.8660254037844378194, -0.5000000000000014433, -0.000000000000000000 ) ) ;
#68169=CARTESIAN_POINT ( 'NONE',  ( 79.06689284147950048, 53.93734539651928372, -15.86389558664243538 ) ) ;
#68174=CARTESIAN_POINT ( 'NONE',  ( 70.65333620286477867, 60.57558753426528142, -14.63893798347084818 ) ) ;
#68179=CARTESIAN_POINT ( 'NONE',  ( 81.84472095112539591, 41.18814569898182043, -5.689628007502441243 ) ) ;
#68181=CARTESIAN_POINT ( 'NONE',  ( 11.30507296547734697, 15.03085787977761179, 9.188101187500006262 ) ) ;
#68184=CARTESIAN_POINT ( 'NONE',  ( 66.27049696474395546, 68.63756696002002400, 2.357326866573562718 ) ) ;
#68190=CARTESIAN_POINT ( 'NONE',  ( 35.77750112005064409, 38.84336893147759184, -7.433330006724137462 ) ) ;
#68194=CARTESIAN_POINT ( 'NONE',  ( 18.69336236660381090, 32.83396525600390703, -2.839279412974133887 ) ) ;
#68197=DIRECTION ( 'NONE',  ( -0.3940053768033626169, 0.6824373310787468228, 0.6156614753256509642 ) ) ;
#68200=B_SPLINE_CURVE_WITH_KNOTS ( 'NONE', 3,
 ( #90660, #23677, #68174, #76303, #75307, #90542, #22579, #84416, #99101, #14964 ),
 .UNSPECIFIED., .F., .F.,
 ( 4, 2, 2, 2, 4 ),
 ( 0.000000000000000000, 0.2500000000000000000, 0.5000000000000000000, 0.7500000000000000000, 1.000000000000000000 ),
 .UNSPECIFIED. ) ;
#68201=CARTESIAN_POINT ( 'NONE',  ( 70.51409906297000418, 60.89179027048928106, 14.47183175352521722 ) ) ;
#68202=CARTESIAN_POINT ( 'NONE',  ( 75.98877566108227199, 65.64741556006092082, -14.26224329751477349 ) ) ;
#68203=ADVANCED_FACE ( 'NONE', ( #88657 ), #45791, .T. ) ;
#68205=CARTESIAN_POINT ( 'NONE',  ( 75.06758043940683933, 52.95706437108803755, -16.00702414185586164 ) ) ;
#68207=ORIENTED_EDGE ( 'NONE', *, *, #46516, .T. ) ;
#68208=CARTESIAN_POINT ( 'NONE',  ( 73.02433024948126672, 69.66517378990661769, 9.714162469163332148 ) ) ;
#68210=CARTESIAN_POINT ( 'NONE',  ( 81.37996698483264879, 42.05785630660916752, -7.883612591813013104 ) ) ;
#68214=CARTESIAN_POINT ( 'NONE',  ( 71.90400658755810070, 72.53437165389429708, 1.750395423964772990 ) ) ;
#68216=CARTESIAN_POINT ( 'NONE',  ( 85.01541621076924571, 50.02003410940323391, 13.59443226853714926 ) ) ;
#68219=CARTESIAN_POINT ( 'NONE',  ( 70.81316579126401223, 61.41551742065354347, -14.85192641751565823 ) ) ;
#68220=CARTESIAN_POINT ( 'NONE',  ( 36.41018743920069056, 41.99752408145594984, 5.678558825948276656 ) ) ;
#68221=CARTESIAN_POINT ( 'NONE',  ( 81.56781671333388317, 55.98423300004855463, -16.39433532902864954 ) ) ;
#68228=CARTESIAN_POINT ( 'NONE',  ( 72.10191719723457027, 72.28141447668717490, -1.471618146119747284 ) ) ;
#68230=CARTESIAN_POINT ( 'NONE',  ( 79.66714386024425210, 56.18315950032808104, 16.16506256184515777 ) ) ;
#68235=CARTESIAN_POINT ( 'NONE',  ( 69.88766240224211401, 70.52056060877789889, 5.189453427646838257 ) ) ;
#68236=CARTESIAN_POINT ( 'NONE',  ( 73.22046044295466061, 61.35883500877204710, -14.94439587469189945 ) ) ;
#68239=CARTESIAN_POINT ( 'NONE',  ( 77.29607140482774241, 63.09965268300504704, -15.25444628986662998 ) ) ;
#68244=CARTESIAN_POINT ( 'NONE',  ( 37.97985170016632850, 33.87878583063844928, -9.188101187500006262 ) ) ;
#68252=CARTESIAN_POINT ( 'NONE',  ( 69.59618255175185197, 71.01531595566491717, 2.954799671095214020 ) ) ;
#68255=FACE_OUTER_BOUND ( 'NONE', #4835, .T. ) ;
#68256=VERTEX_POINT ( 'NONE', #70777 ) ;
#68263=EDGE_CURVE ( 'NONE', #27838, #76194, #76228, .T. ) ;
#68266=CARTESIAN_POINT ( 'NONE',  ( 83.63236669786769539, 48.19556681045689572, 12.42628442967038538 ) ) ;
#68267=DIRECTION ( 'NONE',  ( 0.6793907169778464761, 0.000000000000000000, -0.7337767056021385903 ) ) ;
#68273=CARTESIAN_POINT ( 'NONE',  ( 82.35088575792271115, 40.80351433566520569, -3.705252894541431363 ) ) ;
#68274=EDGE_CURVE ( 'NONE', #49112, #50075, #34766, .T. ) ;
#68277=DIRECTION ( 'NONE',  ( -0.8660254037844379305, -0.5000000000000014433, -0.000000000000000000 ) ) ;
#68282=CARTESIAN_POINT ( 'NONE',  ( 82.74895235971042950, 53.70034252712168410, -15.76590362002541035 ) ) ;
#68294=CARTESIAN_POINT ( 'NONE',  ( 37.76795716069910469, 37.50829794293884589, -10.00000000000000355 ) ) ;
#68296=CARTESIAN_POINT ( 'NONE',  ( 82.14587413470448496, 54.18172936202615375, 15.63325719219342957 ) ) ;
#68297=CARTESIAN_POINT ( 'NONE',  ( 71.86118671916545964, 71.93196444170322934, 2.859464606235072370 ) ) ;
#68301=CARTESIAN_POINT ( 'NONE',  ( 74.91863663735624357, 66.38413888100485849, -13.07019282884167843 ) ) ;
#68302=CARTESIAN_POINT ( 'NONE',  ( 81.23729515884194541, 50.24360654307113094, -14.35787940686896569 ) ) ;
#68303=CARTESIAN_POINT ( 'NONE',  ( 71.77728350350676578, 72.07728907414252717, -1.665459805617878652 ) ) ;
#68306=CARTESIAN_POINT ( 'NONE',  ( 23.04210978301306767, 28.70171378149919406, -9.188101187500004485 ) ) ;
#68309=CARTESIAN_POINT ( 'NONE',  ( 3.479571460297436136, 22.98502408145589726, -5.678558825948271327 ) ) ;
#68311=CARTESIAN_POINT ( 'NONE',  ( 76.72979488479921883, 63.64413466080264214, 15.32332512078611053 ) ) ;
#68314=CARTESIAN_POINT ( 'NONE',  ( 82.13437494121951943, 40.75881571130759085, -0.7180065468227782022 ) ) ;
#68316=EDGE_CURVE ( 'NONE', #63769, #16015, #96698, .T. ) ;
#68317=CARTESIAN_POINT ( 'NONE',  ( 73.33599517600377737, 57.35580166543588376, -15.91338689994087652 ) ) ;
#68329=B_SPLINE_CURVE_WITH_KNOTS ( 'NONE', 3,
 ( #58126, #4948, #52028, #28223, #68210, #20147, #51018, #35827, #82491, #74853 ),
 .UNSPECIFIED., .F., .F.,
 ( 4, 2, 2, 2, 4 ),
 ( 0.000000000000000000, 0.0002622400424272762205, 0.0005244800848545524410, 0.0007867201272818286073, 0.001048960169709104882 ),
 .UNSPECIFIED. ) ;
#68331=CARTESIAN_POINT ( 'NONE',  ( 79.15343291076531784, 46.26937536990111255, -12.76842876231724055 ) ) ;
#68333=CARTESIAN_POINT ( 'NONE',  ( 73.10407572603702420, 70.56422230472695389, -7.912081317950750758 ) ) ;
#68338=CARTESIAN_POINT ( 'NONE',  ( 21.67811977205258245, 27.91421378149919263, 9.188101187500008038 ) ) ;
#68339=CARTESIAN_POINT ( 'NONE',  ( 68.18103004421558921, 69.66170404906247882, -2.995069279367296389 ) ) ;
#68340=CARTESIAN_POINT ( 'NONE',  ( 74.90372969979991069, 67.45002815973559507, -12.77473495645215174 ) ) ;
#68346=EDGE_LOOP ( 'NONE', ( #97582, #46047, #13255, #69724 ) ) ;
#68347=ORIENTED_EDGE ( 'NONE', *, *, #7725, .F. ) ;
#68348=CARTESIAN_POINT ( 'NONE',  ( 82.60366837242126792, 49.14327676238544740, -13.42131973624779917 ) ) ;
#68353=CARTESIAN_POINT ( 'NONE',  ( 81.19656099875513178, 43.43094936621162105, -9.896970666190503252 ) ) ;
#68361=CYLINDRICAL_SURFACE ( 'NONE', #64052, 16.60714546451156792 ) ;
#68362=CARTESIAN_POINT ( 'NONE',  ( 71.45645241242529266, 60.59795021819308403, -15.33783228552337441 ) ) ;
#68370=CARTESIAN_POINT ( 'NONE',  ( 67.13485331027831648, 67.70160943399379505, 6.609904295312462708 ) ) ;
#68371=FACE_OUTER_BOUND ( 'NONE', #87453, .T. ) ;
#68375=CARTESIAN_POINT ( 'NONE',  ( 70.76444730179969156, 64.91245173198861096, 12.28581614439569591 ) ) ;
#68383=CARTESIAN_POINT ( 'NONE',  ( 76.08688909832571312, 65.40073596803624412, -14.00630179347337290 ) ) ;
#68390=CARTESIAN_POINT ( 'NONE',  ( 88.25642124133898392, 44.32248799199468436, 4.097629997315075379 ) ) ;
#68392=CARTESIAN_POINT ( 'NONE',  ( 68.79582220353250932, 67.86037842356454064, -8.901523894718444296 ) ) ;
#68394=CARTESIAN_POINT ( 'NONE',  ( 73.05626849676114887, 70.73388556528652771, 7.585159314558868715 ) ) ;
#68395=CARTESIAN_POINT ( 'NONE',  ( 67.87977117728330256, 67.41497322856321261, -7.879648046888831026 ) ) ;
#68399=CARTESIAN_POINT ( 'NONE',  ( 80.99695547787925420, 51.41970790135942337, 14.90329327012050697 ) ) ;
#68402=ORIENTED_EDGE ( 'NONE', *, *, #54719, .F. ) ;
#68408=FACE_BOUND ( 'NONE', #16286, .T. ) ;
#68409=AXIS2_PLACEMENT_3D ( 'NONE', #52266, #67468, #45161 ) ;
#68410=B_SPLINE_SURFACE_WITH_KNOTS ( 'NONE', 3, 1, ( 
 ( #90665, #6998 ),
 ( #51611, #52592 ),
 ( #29805, #75937 ),
 ( #61191, #74929 ),
 ( #21222, #97730 ),
 ( #22712, #5512 ),
 ( #76426, #91145 ),
 ( #20726, #83046 ),
 ( #59697, #13619 ),
 ( #75423, #37882 ),
 ( #52101, #60678 ),
 ( #68792, #21707 ),
 ( #6007, #43987 ),
 ( #91639, #44492 ),
 ( #83549, #22205 ),
 ( #90150, #36396 ),
 ( #98228, #14111 ),
 ( #30306, #67302 ),
 ( #99718, #37393 ),
 ( #36900, #67810 ),
 ( #44992, #53590 ),
 ( #53100, #6515 ),
 ( #28810, #98738 ),
 ( #15088, #29316 ),
 ( #60181, #68297 ),
 ( #84056, #92159 ),
 ( #76893, #45976 ),
 ( #35903, #66803 ),
 ( #1416, #100223 ),
 ( #46484, #86560 ),
 ( #17093, #77415 ) ),
 .UNSPECIFIED., .F., .F., .F.,
 ( 4, 3, 3, 3, 3, 3, 3, 3, 3, 3, 4 ),
 ( 2, 2 ),
 ( 0.000000000000000000, 0.1333490885032329043, 0.3007194338854160542, 0.4699862290244992691, 0.5844252810809290599, 0.6686540514502579136, 0.7354980260655432645, 0.8028463152565632477, 0.8633854507757217078, 0.9437142632667381292, 1.000000000000000000 ),
 ( 0.000000000000000000, 1.000000000000000000 ),
 .UNSPECIFIED. ) ;
#68411=CARTESIAN_POINT ( 'NONE',  ( 22.17949989257922638, 28.50829794293881037, -10.00000000000000355 ) ) ;
#68420=CARTESIAN_POINT ( 'NONE',  ( 66.46987139367209352, 67.81550840317085260, -6.813679838459789195 ) ) ;
#68421=CARTESIAN_POINT ( 'NONE',  ( 72.60008616680403293, 70.69752196365912766, -7.958780822297740976 ) ) ;
#68424=CARTESIAN_POINT ( 'NONE',  ( 32.31170220804710880, 20.78380873178788590, -6.180339887498949025 ) ) ;
#68425=CARTESIAN_POINT ( 'NONE',  ( 85.04811473893079210, 48.86618300925753999, 12.37604778915560466 ) ) ;
#68436=CARTESIAN_POINT ( 'NONE',  ( 72.64601778605845084, 70.71744408260789783, -7.969226289351845516 ) ) ;
#68447=CARTESIAN_POINT ( 'NONE',  ( 14.59716579798650571, 20.37878583063839955, 9.188101187500006262 ) ) ;
#68449=CARTESIAN_POINT ( 'NONE',  ( 71.98731340802646628, 59.17192410441948169, 15.36756879449314361 ) ) ;
#68453=CARTESIAN_POINT ( 'NONE',  ( 85.75095561453852611, 45.41483102380262693, -9.096727499225101710 ) ) ;
#68454=CARTESIAN_POINT ( 'NONE',  ( 88.20309331078988180, 44.34480599067857298, 2.645673501954918905 ) ) ;
#68460=CARTESIAN_POINT ( 'NONE',  ( 23.31615823149839173, 29.16454794089042224, -10.00000000000000355 ) ) ;
#68463=VERTEX_POINT ( 'NONE', #4890 ) ;
#68467=ORIENTED_EDGE ( 'NONE', *, *, #28064, .F. ) ;
#68469=CARTESIAN_POINT ( 'NONE',  ( 20.88255934282640425, 35.55466486950700045, -1.111400068045478839E-16 ) ) ;
#68470=CARTESIAN_POINT ( 'NONE',  ( 80.45778748667572700, 57.56998633490270123, -16.59146305250142817 ) ) ;
#68473=CARTESIAN_POINT ( 'NONE',  ( 87.70425917765611246, 45.32258268275877811, -6.393467233578020270 ) ) ;
#68479=CARTESIAN_POINT ( 'NONE',  ( 78.21017654319952328, 47.49421537874133037, -13.82074165126671161 ) ) ;
#68482=B_SPLINE_CURVE_WITH_KNOTS ( 'NONE', 3,
 ( #87187, #33932, #2015, #1531, #63307, #64817, #79559, #41497, #95765, #40981, #94249, #80052, #10619, #24803, #57193, #88173, #18720, #49602, #80556, #55681, #86668, #17201, #79046, #9636, #34407, #96249, #50108, #11626, #81063, #65307, #57694, #26812, #42486, #88670, #73420, #19241, #93354, #129, #14327, #70514, #78135, #60902, #29529, #69514, #54294, #61409 ),
 .UNSPECIFIED., .F., .F.,
 ( 4, 1, 2, 2, 1, 2, 2, 1, 1, 2, 2, 1, 1, 2, 2, 1, 1, 2, 2, 1, 1, 1, 2, 2, 1, 1, 1, 2, 2, 4 ),
 ( 0.000000000000000000, 0.06249999999999741873, 0.09374999999999802935, 0.1249999999999986400, 0.1875000000000015266, 0.2187500000000030531, 0.2500000000000046074, 0.3125000000000126565, 0.3437500000000192069, 0.3593750000000220379, 0.3750000000000248135, 0.4375000000000291989, 0.4687500000000297540, 0.4843750000000322520, 0.5000000000000347500, 0.5625000000000445199, 0.5937500000000497380, 0.6093750000000524025, 0.6250000000000550671, 0.6875000000000631717, 0.7187500000000650591, 0.7343750000000655032, 0.7421875000000640599, 0.7500000000000626166, 0.8125000000000711653, 0.8437500000000753841, 0.8593750000000757172, 0.8671875000000740519, 0.8750000000000723865, 1.000000000000000000 ),
 .UNSPECIFIED. ) ;
#68485=CARTESIAN_POINT ( 'NONE',  ( 78.33451385638642250, 47.33805271545526239, -14.25445639310817825 ) ) ;
#68486=CARTESIAN_POINT ( 'NONE',  ( 83.83376537196386380, 51.97730738287452823, 14.54470171158602732 ) ) ;
#68489=B_SPLINE_CURVE_WITH_KNOTS ( 'NONE', 3,
 ( #64843, #65333, #17224, #33957, #94273, #2555, #70951, #33438, #1554, #24828 ),
 .UNSPECIFIED., .F., .F.,
 ( 4, 2, 2, 2, 4 ),
 ( 0.000000000000000000, 0.0002622400424272748110, 0.0005244800848545496221, 0.0007867201272818244873, 0.001048960169709099244 ),
 .UNSPECIFIED. ) ;
#68491=CARTESIAN_POINT ( 'NONE',  ( 73.48837899454035494, 69.83143880527059366, 9.244587476903205925 ) ) ;
#68492=CARTESIAN_POINT ( 'NONE',  ( 83.46095475844008149, 42.81445974211163730, -5.980450563400608210 ) ) ;
#68495=CARTESIAN_POINT ( 'NONE',  ( 82.30387339498274457, 53.64944443644738215, 15.82386716188995557 ) ) ;
#68503=CARTESIAN_POINT ( 'NONE',  ( 70.58255314538416769, 68.84473063892380651, 8.184723017349652352 ) ) ;
#68508=CARTESIAN_POINT ( 'NONE',  ( 78.43104943820020480, 47.80709632928548558, 13.91158340242805025 ) ) ;
#68512=CARTESIAN_POINT ( 'NONE',  ( 71.97367111486161662, 69.50864518808729997, 8.459197605334548342 ) ) ;
#68515=CARTESIAN_POINT ( 'NONE',  ( 79.32956177646403262, 46.17935033225089825, 12.63826207646849120 ) ) ;
#68516=DIRECTION ( 'NONE',  ( 0.5000000000000014433, -0.8660254037844378194, 0.000000000000000000 ) ) ;
#68519=ORIENTED_EDGE ( 'NONE', *, *, #73090, .F. ) ;
#68523=CARTESIAN_POINT ( 'NONE',  ( 72.38244233070295763, 71.76593646792086645, 5.668245152086877958 ) ) ;
#68537=CARTESIAN_POINT ( 'NONE',  ( 81.95415531698857592, 41.13631750917600982, -5.408051707503558347 ) ) ;
#68538=CARTESIAN_POINT ( 'NONE',  ( 81.92698409329203457, 58.82261968288553078, -0.3345653031794284527 ) ) ;
#68548=CARTESIAN_POINT ( 'NONE',  ( 9.459751770947381289, 21.16454794089040092, -10.00000000000000355 ) ) ;
#68550=CARTESIAN_POINT ( 'NONE',  ( 71.62750703794239371, 58.90906671320517773, -15.38493269445189426 ) ) ;
#68551=DIRECTION ( 'NONE',  ( -0.8660254037844379305, -0.5000000000000014433, -0.000000000000000000 ) ) ;
#68555=CARTESIAN_POINT ( 'NONE',  ( 72.83054026352687060, 57.09011829142805539, 16.39008592795239494 ) ) ;
#68557=CARTESIAN_POINT ( 'NONE',  ( 66.06942622996319869, 68.50909977235997417, -4.639585442171386021 ) ) ;
#68562=VECTOR ( 'NONE', #60674, 1000.000000000000114 ) ;
#68564=CARTESIAN_POINT ( 'NONE',  ( 25.79477067763620468, 36.93396525600391556, 2.839279412974139660 ) ) ;
#68568=CARTESIAN_POINT ( 'NONE',  ( 83.21354822495420933, 40.96322299393881394, -2.105546863297833582 ) ) ;
#68570=CARTESIAN_POINT ( 'NONE',  ( 69.03518170980191826, 64.49507618479454152, 12.45339560626615949 ) ) ;
#68574=CARTESIAN_POINT ( 'NONE',  ( 72.51084313652232538, 66.78536858707103363, -12.23974485817613100 ) ) ;
#68590=CARTESIAN_POINT ( 'NONE',  ( 7.946103921272086090, 26.36126292948893735, 6.180339887498949913 ) ) ;
#68594=CARTESIAN_POINT ( 'NONE',  ( 86.33167747996513697, 46.96304910452010262, -10.52679092302835251 ) ) ;
#68595=CARTESIAN_POINT ( 'NONE',  ( 83.75784171508648512, 45.20434354284536482, -9.539610091384043145 ) ) ;
#68600=CARTESIAN_POINT ( 'NONE',  ( 69.84702423369627411, 62.74498161306693333, 13.91467287971852329 ) ) ;
#68604=CARTESIAN_POINT ( 'NONE',  ( 73.36513840663161545, 69.69468182635826281, -9.911920066630193205 ) ) ;
#68606=CARTESIAN_POINT ( 'NONE',  ( 81.50676111512028399, 42.61959527892759070, -7.662561320371898077 ) ) ;
#68608=ORIENTED_EDGE ( 'NONE', *, *, #26647, .T. ) ;
#68612=CARTESIAN_POINT ( 'NONE',  ( 68.34715014356760321, 68.60616615819722597, 6.278734008161547919 ) ) ;
#68613=CARTESIAN_POINT ( 'NONE',  ( 87.88245627177123254, 44.92329797532172364, 6.249457923817313798 ) ) ;
#68616=EDGE_CURVE ( 'NONE', #63738, #81254, #63054, .T. ) ;
#68619=CARTESIAN_POINT ( 'NONE',  ( 68.61954826535414043, 68.39247321939140534, -6.997216880091692737 ) ) ;
#68620=ORIENTED_EDGE ( 'NONE', *, *, #78491, .F. ) ;
#68621=DIRECTION ( 'NONE',  ( -0.5000000000000014433, 0.8660254037844378194, 0.000000000000000000 ) ) ;
#68622=CARTESIAN_POINT ( 'NONE',  ( 19.86064915544625009, 12.26216523072493914, -2.296566073217252530E-15 ) ) ;
#68624=B_SPLINE_CURVE_WITH_KNOTS ( 'NONE', 3,
 ( #20482, #65568, #92394, #76184, #75183, #30049, #20991, #82324, #22454, #44737, #52350, #67055, #21954, #98976, #5272, #59942 ),
 .UNSPECIFIED., .F., .F.,
 ( 4, 1, 2, 2, 2, 1, 2, 2, 4 ),
 ( 0.000000000000000000, 0.1250000000000021649, 0.1875000000000032474, 0.2500000000000043299, 0.5000000000000027756, 0.6250000000000019984, 0.6875000000000016653, 0.7500000000000013323, 1.000000000000000000 ),
 .UNSPECIFIED. ) ;
#68625=CARTESIAN_POINT ( 'NONE',  ( 80.03143596134809457, 57.61873189500684589, 16.60059503390608882 ) ) ;
#68627=VERTEX_POINT ( 'NONE', #94491 ) ;
#68630=CARTESIAN_POINT ( 'NONE',  ( 80.24160137367489654, 44.78810531146535823, 11.12097059984180980 ) ) ;
#68637=CARTESIAN_POINT ( 'NONE',  ( 73.75273084276152247, 62.67190600634478415, -14.57620950672273707 ) ) ;
#68641=CARTESIAN_POINT ( 'NONE',  ( 82.86119955336803855, 53.69823230216047705, -15.38187069736933665 ) ) ;
#68645=CARTESIAN_POINT ( 'NONE',  ( 82.45365866864536031, 44.73731268782142934, -9.806852841930714604 ) ) ;
#68662=CARTESIAN_POINT ( 'NONE',  ( 79.24882819772426501, 57.92845866569951596, 16.22381856495110597 ) ) ;
#68671=CARTESIAN_POINT ( 'NONE',  ( 70.37262225357338252, 70.61908426682903439, 4.266529024624744260 ) ) ;
#68673=CARTESIAN_POINT ( 'NONE',  ( 79.14312167556931854, 57.64441083166269664, 0.000000000000000000 ) ) ;
#68676=CARTESIAN_POINT ( 'NONE',  ( 81.85743566648118019, 41.23085629097093374, -5.772627936764054724 ) ) ;
#68678=CARTESIAN_POINT ( 'NONE',  ( 12.70933400901951416, 9.198606405272903075, 2.839279412974134775 ) ) ;
#68686=CARTESIAN_POINT ( 'NONE',  ( 36.38853680410607438, 41.98502408145596121, -5.678558825948271327 ) ) ;
#68689=CARTESIAN_POINT ( 'NONE',  ( 23.88951478931043937, 35.83396525600391413, -2.839279412974133887 ) ) ;
#68694=B_SPLINE_CURVE_WITH_KNOTS ( 'NONE', 3,
 ( #90299, #5641, #59319, #88825, #89316, #57844, #19390, #81203, #50249, #11772, #74068, #4147, #73564, #27943, #35043, #65947 ),
 .UNSPECIFIED., .F., .F.,
 ( 4, 1, 2, 2, 2, 1, 2, 2, 4 ),
 ( 0.000000000000000000, 0.1249999999999996114, 0.1874999999999998612, 0.2500000000000001110, 0.5000000000000000000, 0.6249999999999997780, 0.6874999999999998890, 0.7499999999999998890, 1.000000000000000000 ),
 .UNSPECIFIED. ) ;
#68695=EDGE_CURVE ( 'NONE', #1759, #81254, #8009, .T. ) ;
#68708=CARTESIAN_POINT ( 'NONE',  ( 36.52324494929276710, 26.80170272979929180, 7.433330006724137462 ) ) ;
#68714=ORIENTED_EDGE ( 'NONE', *, *, #57133, .F. ) ;
#68720=CARTESIAN_POINT ( 'NONE',  ( 41.82943821127123840, 26.01110640527295814, 2.839279412974134775 ) ) ;
#68721=CARTESIAN_POINT ( 'NONE',  ( 81.62646408706272894, 55.64454924624774890, -16.33875670839028516 ) ) ;
#68735=CARTESIAN_POINT ( 'NONE',  ( 75.96712627484227198, 60.44064756120551607, -15.70488828003969672 ) ) ;
#68736=CARTESIAN_POINT ( 'NONE',  ( 82.32788549632455499, 40.35540550160623496, 1.181641335447100483 ) ) ;
#68746=AXIS2_PLACEMENT_3D ( 'NONE', #67470, #42662, #98397 ) ;
#68748=CARTESIAN_POINT ( 'NONE',  ( 77.86555730066852732, 62.20866292688850052, -15.95979438352862445 ) ) ;
#68750=CARTESIAN_POINT ( 'NONE',  ( 34.61729389309891758, 20.39040679176985549, -6.890680421881970419E-14 ) ) ;
#68751=CARTESIAN_POINT ( 'NONE',  ( 81.68759648889933089, 55.58869686435339474, 15.96161034574013904 ) ) ;
#68753=CARTESIAN_POINT ( 'NONE',  ( 81.97299385056439291, 58.74292844564591576, 0.1873032967079579780 ) ) ;
#68768=CARTESIAN_POINT ( 'NONE',  ( 72.98844966468033135, 67.52117381499635940, 11.29058222731423555 ) ) ;
#68772=CARTESIAN_POINT ( 'NONE',  ( 71.64065041137482126, 72.08859242525181799, 3.376608021325386844 ) ) ;
#68775=CARTESIAN_POINT ( 'NONE',  ( 84.96561085921061363, 46.52165563237655022, 10.26214194272153080 ) ) ;
#68784=AXIS2_PLACEMENT_3D ( 'NONE', #15354, #91924, #23457 ) ;
#68787=CARTESIAN_POINT ( 'NONE',  ( 73.32155222933093341, 69.66094733087366819, -9.921889652296787432 ) ) ;
#68788=CARTESIAN_POINT ( 'NONE',  ( 76.27945191441585848, 51.11642808127202642, 16.06162126745443075 ) ) ;
#68789=CARTESIAN_POINT ( 'NONE',  ( 33.33823495471120424, 42.18080186712595747, 3.090169943749475401 ) ) ;
#68792=CARTESIAN_POINT ( 'NONE',  ( 72.03850700256526807, 72.31288868693221161, 3.399215934587869636 ) ) ;
#68797=CARTESIAN_POINT ( 'NONE',  ( 81.29157559341378203, 42.21858700188892044, -7.212111827135544218 ) ) ;
#68798=CARTESIAN_POINT ( 'NONE',  ( 79.13486416932684619, 50.85352373906047063, -15.04773823355513507 ) ) ;
#68802=CARTESIAN_POINT ( 'NONE',  ( 22.99159801516092472, 18.98920272979926693, 7.433330006724137462 ) ) ;
#68804=CARTESIAN_POINT ( 'NONE',  ( 17.35761498915574563, 12.94754757982088300, 5.678558825948272215 ) ) ;
#68806=CARTESIAN_POINT ( 'NONE',  ( 76.75696856028530135, 63.87261700412425114, 14.87451922956917016 ) ) ;
#68807=CARTESIAN_POINT ( 'NONE',  ( 80.07812099633126479, 57.44764983040322193, -16.59488970948941500 ) ) ;
#68811=EDGE_CURVE ( 'NONE', #59206, #2820, #69422, .T. ) ;
#68814=CARTESIAN_POINT ( 'NONE',  ( 75.43400731199886877, 56.71754055093797575, -16.11584012409328182 ) ) ;
#68827=CARTESIAN_POINT ( 'NONE',  ( 79.24070844107342282, 45.72899464571315775, -12.97329291253947936 ) ) ;
#68830=CARTESIAN_POINT ( 'NONE',  ( 83.10776606998568639, 40.75710275334526500, -2.573362665496658816E-06 ) ) ;
#68833=CARTESIAN_POINT ( 'NONE',  ( 21.37261828447143586, 20.84335787977762777, 9.188101187500006262 ) ) ;
#68834=VECTOR ( 'NONE', #94557, 1000.000000000000114 ) ;
#68835=CARTESIAN_POINT ( 'NONE',  ( 75.05636926434671352, 55.10128444218372579, 16.14643111463205472 ) ) ;
#68844=CARTESIAN_POINT ( 'NONE',  ( 71.11357831182630207, 63.84590708448217811, 13.70173731491832392 ) ) ;
#68845=CARTESIAN_POINT ( 'NONE',  ( 68.01214654971191464, 65.20889497348429131, -10.65419055744410315 ) ) ;
#68861=CARTESIAN_POINT ( 'NONE',  ( 66.65733650514845010, 67.51765459828601479, 6.434609397296672029 ) ) ;
#68864=CARTESIAN_POINT ( 'NONE',  ( 84.14312167556933275, 48.98415679381830756, 0.000000000000000000 ) ) ;
#68867=CARTESIAN_POINT ( 'NONE',  ( 87.33294734268930881, 44.88192199842172414, 6.808005391826766228 ) ) ;
#68869=CARTESIAN_POINT ( 'NONE',  ( 24.66226663818958187, 15.20801979619928979, -3.090169943749474069 ) ) ;
#68871=ORIENTED_EDGE ( 'NONE', *, *, #22069, .T. ) ;
#68872=CARTESIAN_POINT ( 'NONE',  ( 76.04487332539315503, 51.27808848417036103, -16.12710007477251750 ) ) ;
#68873=CARTESIAN_POINT ( 'NONE',  ( 75.98877566108227199, 65.64741556006092082, -14.26224329751477349 ) ) ;
#68883=CARTESIAN_POINT ( 'NONE',  ( 80.01804950108486025, 44.42439889875981152, -10.91110617052017773 ) ) ;
#68885=B_SPLINE_CURVE_WITH_KNOTS ( 'NONE', 3,
 ( #69232, #31228, #100162, #67751, #29256, #52535, #14051, #6454, #68235, #14555, #6936, #9954, #9442, #833, #78860, #72263 ),
 .UNSPECIFIED., .F., .F.,
 ( 4, 1, 2, 2, 2, 1, 2, 2, 4 ),
 ( 0.000000000000000000, 0.1250000000000008049, 0.1875000000000010270, 0.2500000000000014433, 0.5000000000000019984, 0.6250000000000022204, 0.6875000000000025535, 0.7500000000000027756, 1.000000000000000000 ),
 .UNSPECIFIED. ) ;
#68887=CARTESIAN_POINT ( 'NONE',  ( 72.76085654771455324, 70.95487523876634839, 7.692118034595666565 ) ) ;
#68888=CARTESIAN_POINT ( 'NONE',  ( 66.85524610400479162, 67.34209505064850987, -6.990925417236247164 ) ) ;
#68892=CARTESIAN_POINT ( 'NONE',  ( 82.15463706511577868, 40.84277258114416043, 1.595534587534165549 ) ) ;
#68893=CARTESIAN_POINT ( 'NONE',  ( 81.10131807291612915, 51.90498691781395735, 15.05979867673087291 ) ) ;
#68894=CARTESIAN_POINT ( 'NONE',  ( 83.31927764570698969, 52.39912095965794947, 14.85548028051290181 ) ) ;
#68906=CARTESIAN_POINT ( 'NONE',  ( 17.16114660649731860, 34.00034080476290654, -1.878358725466461243E-16 ) ) ;
#68911=VECTOR ( 'NONE', #14350, 1000.000000000000114 ) ;
#68916=CARTESIAN_POINT ( 'NONE',  ( 67.05214125078322240, 67.71989302486406359, -6.480270855117335138 ) ) ;
#68917=CARTESIAN_POINT ( 'NONE',  ( 72.78963790118943677, 71.14248580567581826, -7.401817665068018748 ) ) ;
#68918=CARTESIAN_POINT ( 'NONE',  ( 81.84240242494415440, 41.28568805806720832, 5.918639025823554611 ) ) ;
#68920=CARTESIAN_POINT ( 'NONE',  ( 29.18428119120667574, 28.80066082961423390, 10.00000000000000533 ) ) ;
#68921=CARTESIAN_POINT ( 'NONE',  ( 77.57594518282449769, 55.55670249163367913, 16.58798725124399454 ) ) ;
#68934=CARTESIAN_POINT ( 'NONE',  ( 77.28526253906952093, 49.15772476309707173, -14.80239747722083621 ) ) ;
#68941=CARTESIAN_POINT ( 'NONE',  ( 22.77687932801360660, 15.01110640527292261, 2.839279412974134775 ) ) ;
#68943=CARTESIAN_POINT ( 'NONE',  ( 71.59150237832598407, 59.07131284048556807, 15.83293140498724050 ) ) ;
#68947=CARTESIAN_POINT ( 'NONE',  ( 86.99519960183430101, 45.47778473895603923, -7.388714814205115111 ) ) ;
#68952=CARTESIAN_POINT ( 'NONE',  ( 88.26419143691403235, 44.30358433922314276, 2.120137394640778883 ) ) ;
#68956=CARTESIAN_POINT ( 'NONE',  ( 72.29675234079142854, 71.91852905550483399, -5.160928375136445645 ) ) ;
#68958=CARTESIAN_POINT ( 'NONE',  ( 27.61987535298997187, 21.11029122506295508, -8.090169943749478065 ) ) ;
#68959=CARTESIAN_POINT ( 'NONE',  ( 86.84691188820112018, 44.77746935395023087, 7.166350442650676555 ) ) ;
#68961=ORIENTED_EDGE ( 'NONE', *, *, #67258, .F. ) ;
#68962=CARTESIAN_POINT ( 'NONE',  ( 68.68909986782581711, 64.16576715805911135, -12.55144644517788421 ) ) ;
#68963=CARTESIAN_POINT ( 'NONE',  ( 85.70718678116344336, 42.98724156638103722, -2.704305901507331189 ) ) ;
#68966=CARTESIAN_POINT ( 'NONE',  ( 70.59980718957763202, 66.46770090284240950, 11.57891045287148479 ) ) ;
#68967=CARTESIAN_POINT ( 'NONE',  ( 79.98470177819076810, 58.12003377381869029, 16.26822267875589390 ) ) ;
#68973=AXIS2_PLACEMENT_3D ( 'NONE', #61305, #16710, #47603 ) ;
#68979=CARTESIAN_POINT ( 'NONE',  ( 78.15521468916944059, 47.58268334285837398, -13.88154174790995832 ) ) ;
#68984=CARTESIAN_POINT ( 'NONE',  ( 83.40377981393274354, 52.41387144640057727, 14.84149447075486350 ) ) ;
#68988=CARTESIAN_POINT ( 'NONE',  ( 87.13786027870773410, 46.31489396970533789, 8.575336957479223088 ) ) ;
#68995=CARTESIAN_POINT ( 'NONE',  ( 72.04811769650321196, 71.35602353065118564, 5.168332083721268511 ) ) ;
#68996=CARTESIAN_POINT ( 'NONE',  ( 66.31795133325435643, 69.20145725284447735, 2.477662600225432055 ) ) ;
#68997=CARTESIAN_POINT ( 'NONE',  ( 66.98349674211237925, 66.92588320361704746, 8.745657410628504991 ) ) ;
#68999=CARTESIAN_POINT ( 'NONE',  ( 77.93929205318025311, 48.04607352951135368, 14.17332408082497963 ) ) ;
#69002=CARTESIAN_POINT ( 'NONE',  ( 71.00886383429117643, 67.21468722179194799, 10.46115210183619659 ) ) ;
#69004=CARTESIAN_POINT ( 'NONE',  ( 79.45999046205805882, 46.29338198536788695, 12.66529585336078156 ) ) ;
#69006=CARTESIAN_POINT ( 'NONE',  ( 74.53665744383957303, 56.45882270339276232, -16.57090531272829637 ) ) ;
#69011=CARTESIAN_POINT ( 'NONE',  ( 72.37171713508972459, 71.57547101742603957, 5.089270018883309987 ) ) ;
#69013=B_SPLINE_CURVE_WITH_KNOTS ( 'NONE', 3,
 ( #86038, #63167, #77380, #16566, #23155, #14582, #54046, #8968 ),
 .UNSPECIFIED., .F., .F.,
 ( 4, 2, 2, 4 ),
 ( 0.000000000000000000, 0.2251665007938979668, 0.3377497511908476580, 0.4503330015877973214 ),
 .UNSPECIFIED. ) ;
#69017=CARTESIAN_POINT ( 'NONE',  ( 66.79137522077492406, 67.56334705497756943, -6.492718058864330288 ) ) ;
#69023=CARTESIAN_POINT ( 'NONE',  ( 85.71030961992515529, 48.80922481583876049, -12.49884386288095151 ) ) ;
#69025=CARTESIAN_POINT ( 'NONE',  ( 71.64267482440028800, 65.36664440745120430, 12.36713528089073399 ) ) ;
#69027=ADVANCED_FACE ( 'NONE', ( #64830 ), #26824, .T. ) ;
#69030=VECTOR ( 'NONE', #3616, 1000.000000000000114 ) ;
#69031=EDGE_CURVE ( 'NONE', #36202, #38035, #72452, .T. ) ;
#69040=CARTESIAN_POINT ( 'NONE',  ( 84.04720468787148491, 46.80380424559275809, -11.65275933647250639 ) ) ;
#69043=CARTESIAN_POINT ( 'NONE',  ( 6.173449292434340485, 27.65659080271448644, -1.878358725466461243E-16 ) ) ;
#69044=CIRCLE ( 'NONE', #35068, 15.10714546451156792 ) ;
#69046=CARTESIAN_POINT ( 'NONE',  ( 71.47065342991831471, 59.20086974812521419, -15.77730099079427362 ) ) ;
#69047=CARTESIAN_POINT ( 'NONE',  ( 73.06086572573603632, 69.73927861498383152, 9.650215327041465230 ) ) ;
#69052=CARTESIAN_POINT ( 'NONE',  ( 9.331744567327184825, 27.16126292948893806, -6.180339887498951690 ) ) ;
#69060=CARTESIAN_POINT ( 'NONE',  ( 36.95804531498377798, 23.19860640527294748, 2.839279412974134775 ) ) ;
#69061=CARTESIAN_POINT ( 'NONE',  ( 81.82670292275410873, 58.99631176529970844, 0.4698463103929552132 ) ) ;
#69063=EDGE_CURVE ( 'NONE', #16291, #38703, #79831, .T. ) ;
#69065=CARTESIAN_POINT ( 'NONE',  ( 88.40933139567989940, 44.00655032011064804, 2.323659332633154495 ) ) ;
#69068=CARTESIAN_POINT ( 'NONE',  ( 68.86379457292682105, 64.30659086896544352, 12.52137705277578661 ) ) ;
#69073=CARTESIAN_POINT ( 'NONE',  ( 6.943673075435187414, 24.98502408145590437, -5.678558825948271327 ) ) ;
#69076=CARTESIAN_POINT ( 'NONE',  ( 41.24097861217908445, 35.76159833115055164, -9.594050593750004907 ) ) ;
#69087=CARTESIAN_POINT ( 'NONE',  ( 73.05796794158769103, 70.59459209629945065, 7.799841062623454668 ) ) ;
#69091=CARTESIAN_POINT ( 'NONE',  ( 84.50184486765282088, 45.13281382370418271, -8.938886561040149559 ) ) ;
#69096=CARTESIAN_POINT ( 'NONE',  ( 69.33684657993413225, 62.91444721635136261, 13.64444443003713658 ) ) ;
#69102=CARTESIAN_POINT ( 'NONE',  ( 81.64076222525299897, 42.65095382059221407, -7.589903255537720383 ) ) ;
#69103=B_SPLINE_CURVE_WITH_KNOTS ( 'NONE', 3,
 ( #13533, #44402, #28214, #14019, #75335, #91058, #37303, #27232, #58116, #19648, #81461, #12036, #73828, #76806, #77825, #85457 ),
 .UNSPECIFIED., .F., .F.,
 ( 4, 1, 2, 2, 2, 1, 2, 2, 4 ),
 ( 0.000000000000000000, 0.1249999999999977796, 0.1874999999999976130, 0.2499999999999974465, 0.4999999999999986677, 0.6249999999999964473, 0.6874999999999977796, 0.7499999999999991118, 1.000000000000000000 ),
 .UNSPECIFIED. ) ;
#69104=VERTEX_POINT ( 'NONE', #35411 ) ;
#69109=CARTESIAN_POINT ( 'NONE',  ( 67.87260471423661556, 67.92298336072001064, 7.036170726210575488 ) ) ;
#69113=( BOUNDED_CURVE ( )  B_SPLINE_CURVE ( 2, ( #78818, #40278, #57483, #43651, #74591, #5168, #36047, #9918, #66950, #17500, #40776, #97879, #1811 ),
 .UNSPECIFIED., .F., .T. ) 
 B_SPLINE_CURVE_WITH_KNOTS ( ( 3, 2, 2, 2, 2, 2, 3 ),
 ( 0.3875000000000000111, 0.3900000000000000133, 0.3950000000000000178, 0.4000000000000000222, 0.4050000000000000266, 0.4099999999999999756, 0.4124999999999999778 ),
 .UNSPECIFIED. ) 
 CURVE ( )  GEOMETRIC_REPRESENTATION_ITEM ( )  RATIONAL_B_SPLINE_CURVE ( ( 0.9755282581475768211, 0.9755282581475768211, 1.000000000000000000, 0.9510565162951535312, 1.000000000000000000, 0.9510565162951535312, 1.000000000000000000, 0.9510565162951535312, 1.000000000000000000, 0.9510565162951535312, 1.000000000000000000, 0.9755282581475768211, 0.9755282581475768211 ) ) 
 REPRESENTATION_ITEM ( '' )  );
#69114=DIRECTION ( 'NONE',  ( 0.9563064286990885510, -0.2923662333936583035, 0.000000000000000000 ) ) ;
#69118=CARTESIAN_POINT ( 'NONE',  ( 67.46170827899872791, 68.25562313450184604, -5.901104080436347488 ) ) ;
#69120=CARTESIAN_POINT ( 'NONE',  ( 15.18774714507562962, 26.95586893147754992, 7.433330006724141015 ) ) ;
#69125=AXIS2_PLACEMENT_3D ( 'NONE', #43083, #80160, #87791 ) ;
#69128=LINE ( 'NONE', #100055, #82943 ) ;
#69137=CARTESIAN_POINT ( 'NONE',  ( 82.80324341411446198, 53.35862238445501049, -15.29491566309662431 ) ) ;
#69138=B_SPLINE_CURVE_WITH_KNOTS ( 'NONE', 3,
 ( #45330, #84871, #52934, #52434, #37720, #61018, #7841, #68630, #15414, #69628 ),
 .UNSPECIFIED., .F., .F.,
 ( 4, 2, 2, 2, 4 ),
 ( 0.000000000000000000, 0.2500000000000000000, 0.5000000000000000000, 0.7500000000000000000, 1.000000000000000000 ),
 .UNSPECIFIED. ) ;
#69141=CARTESIAN_POINT ( 'NONE',  ( 72.00034353288134525, 72.28740038217357267, 0.6661088224210791608 ) ) ;
#69144=CARTESIAN_POINT ( 'NONE',  ( 76.25214315863026115, 65.18377266038437767, 14.56725100193072464 ) ) ;
#69150=CARTESIAN_POINT ( 'NONE',  ( 86.41412918452650160, 45.91353383111829345, -8.603224342125431079 ) ) ;
#69154=CARTESIAN_POINT ( 'NONE',  ( 82.85052922654625718, 43.48557670598759728, 7.868807238270560056 ) ) ;
#69163=CARTESIAN_POINT ( 'NONE',  ( 76.63628273442517980, 54.74213442968584076, -16.10156611425468753 ) ) ;
#69167=CARTESIAN_POINT ( 'NONE',  ( 83.37296956034944628, 51.74080471427829764, 14.95189368521466733 ) ) ;
#69172=CARTESIAN_POINT ( 'NONE',  ( 80.84168478348897224, 44.34659258387878111, 10.38138091060227275 ) ) ;
#69175=CARTESIAN_POINT ( 'NONE',  ( 75.25561967922160989, 63.20475890752934589, 15.17030042159924008 ) ) ;
#69178=CARTESIAN_POINT ( 'NONE',  ( 81.91900929568903678, 41.12952449508415498, -5.442184166135863421 ) ) ;
#69180=CARTESIAN_POINT ( 'NONE',  ( 16.06339478488542127, 14.98920272979925272, 7.433330006724137462 ) ) ;
#69182=PLANE ( 'NONE',  #69205 ) ;
#69183=AXIS2_PLACEMENT_3D ( 'NONE', #1727, #21641, #23112 ) ;
#69184=CARTESIAN_POINT ( 'NONE',  ( 66.54264984482914258, 68.81226801441182772, 2.258477026830895795 ) ) ;
#69189=CARTESIAN_POINT ( 'NONE',  ( 34.56506555475243658, 38.14336893147758900, 7.433330006724141015 ) ) ;
#69190=PLANE ( 'NONE',  #24057 ) ;
#69191=FACE_BOUND ( 'NONE', #86981, .T. ) ;
#69193=CARTESIAN_POINT ( 'NONE',  ( 31.21402144970675607, 20.94754757982090609, 5.678558825948272215 ) ) ;
#69200=CARTESIAN_POINT ( 'NONE',  ( 84.79901702372750094, 50.05075620941028092, -13.68787013058487290 ) ) ;
#69201=CARTESIAN_POINT ( 'NONE',  ( 83.09612612754671090, 41.63338805721024016, 5.024036258903810115 ) ) ;
#69205=AXIS2_PLACEMENT_3D ( 'NONE', #21123, #61075, #6406 ) ;
#69208=CARTESIAN_POINT ( 'NONE',  ( 38.91320803870388545, 23.26216523072497466, -2.296566073217252530E-15 ) ) ;
#69213=CARTESIAN_POINT ( 'NONE',  ( 86.48586980954701176, 47.12904147948177069, -10.06668187157390904 ) ) ;
#69215=CARTESIAN_POINT ( 'NONE',  ( 84.62070576355738183, 50.25222463068733703, 13.86530520652494758 ) ) ;
#69221=CARTESIAN_POINT ( 'NONE',  ( 79.98969732019267553, 44.69009452991755893, 11.16475366590057483 ) ) ;
#69222=CARTESIAN_POINT ( 'NONE',  ( 81.29586503113306151, 55.42867650357229081, -16.33480133305122095 ) ) ;
#69223=CARTESIAN_POINT ( 'NONE',  ( 72.37973851903267075, 63.38476940627418799, -14.36017998060057721 ) ) ;
#69228=CARTESIAN_POINT ( 'NONE',  ( 87.07436038242185816, 45.84038486297258430, -8.630882807222770126 ) ) ;
#69231=CARTESIAN_POINT ( 'NONE',  ( 80.32560484147226987, 44.93948968179056180, -11.21518412823304800 ) ) ;
#69232=CARTESIAN_POINT ( 'NONE',  ( 67.53167658295855347, 67.09922345392760690, 8.942594108559751120 ) ) ;
#69233=CARTESIAN_POINT ( 'NONE',  ( 71.72451190509423213, 61.77407603521598389, -14.41855241212332750 ) ) ;
#69234=CARTESIAN_POINT ( 'NONE',  ( 79.16903247652662401, 46.12461580907955749, 12.66491118591851972 ) ) ;
#69237=CARTESIAN_POINT ( 'NONE',  ( 77.13937272485186725, 63.60852409164084520, -15.03876710342725076 ) ) ;
#69241=CARTESIAN_POINT ( 'NONE',  ( 43.45144817956826699, 30.80170272979930601, 7.433330006724137462 ) ) ;
#69244=ORIENTED_EDGE ( 'NONE', *, *, #52083, .T. ) ;
#69246=CARTESIAN_POINT ( 'NONE',  ( 86.87376599001147781, 45.86940958085830999, -8.177027763546412586 ) ) ;
#69247=CARTESIAN_POINT ( 'NONE',  ( 70.21756736500132945, 64.16742292537257697, -12.57977312374782919 ) ) ;
#69250=CARTESIAN_POINT ( 'NONE',  ( 72.68991634181023187, 64.30301886947491141, 13.46146812301844164 ) ) ;
#69257=CARTESIAN_POINT ( 'NONE',  ( 79.38841588403847993, 49.82580522342896501, 15.10957065665274257 ) ) ;
#69264=CARTESIAN_POINT ( 'NONE',  ( 81.71431622648833581, 43.56938202975830166, 8.897122998445636810 ) ) ;
#69270=B_SPLINE_SURFACE_WITH_KNOTS ( 'NONE', 3, 1, ( 
 ( #59121, #51039 ),
 ( #44931, #13075 ),
 ( #81996, #29748 ),
 ( #83993, #75370 ),
 ( #60620, #29258 ),
 ( #45432, #75878 ),
 ( #5951, #37828 ),
 ( #21171, #12569 ),
 ( #68736, #43444 ),
 ( #74387, #91575 ),
 ( #74875, #67753 ),
 ( #35852, #20662 ),
 ( #51551, #43936 ),
 ( #36844, #5458 ),
 ( #98174, #59632 ),
 ( #52052, #98677 ),
 ( #60126, #55027 ),
 ( #32734, #39313 ),
 ( #47923, #16534 ),
 ( #8940, #77344 ),
 ( #24142, #17030 ),
 ( #76836, #62620 ),
 ( #86008, #15026 ),
 ( #32235, #23124 ),
 ( #30750, #8444 ),
 ( #93573, #7434 ),
 ( #71258, #39806 ),
 ( #38327, #84484 ),
 ( #15519, #339 ),
 ( #47431, #31230 ),
 ( #70230, #85489 ) ),
 .UNSPECIFIED., .F., .F., .F.,
 ( 4, 3, 3, 3, 3, 3, 3, 3, 3, 3, 4 ),
 ( 2, 2 ),
 ( 0.000000000000000000, 0.1122669598086814685, 0.2243161639709671529, 0.3396355846219190067, 0.4553962076585229557, 0.5677860799922529456, 0.6749047109689662038, 0.7773884377078499330, 0.8775581155834387692, 0.9782364162377882311, 1.000000000000000000 ),
 ( 0.000000000000000000, 1.000000000000000000 ),
 .UNSPECIFIED. ) ;
#69271=CARTESIAN_POINT ( 'NONE',  ( 72.66276004730617899, 66.52099816311097413, 11.94923289124634103 ) ) ;
#69272=CARTESIAN_POINT ( 'NONE',  ( 72.31501564753065736, 60.31777401518989024, 15.59333315930887309 ) ) ;
#69277=CARTESIAN_POINT ( 'NONE',  ( 31.43297906638544603, 41.08080186712595605, -3.090169943749475845 ) ) ;
#69278=ADVANCED_FACE ( 'NONE', ( #4793 ), #15062, .T. ) ;
#69282=CARTESIAN_POINT ( 'NONE',  ( 72.93270222632347100, 70.75261854202813083, -7.421515863126944446 ) ) ;
#69283=EDGE_CURVE ( 'NONE', #43244, #12691, #82503, .T. ) ;
#69285=CARTESIAN_POINT ( 'NONE',  ( 67.43966565062764573, 66.61250739341410565, 8.643685538913882027 ) ) ;
#69287=DIRECTION ( 'NONE',  ( 0.4924038765061026779, -0.8528685319524446085, -0.1736481776669273058 ) ) ;
#69288=EDGE_CURVE ( 'NONE', #749, #21377, #13229, .T. ) ;
#69292=CARTESIAN_POINT ( 'NONE',  ( 20.88255934282640425, 35.55466486950700755, -1.111400068045478839E-16 ) ) ;
#69294=CARTESIAN_POINT ( 'NONE',  ( 76.48813647825510031, 51.17232029059452714, 16.04681448753369821 ) ) ;
#69295=CARTESIAN_POINT ( 'NONE',  ( 1.830000459568766003, 24.55466486950697202, 1.000260061240931054E-15 ) ) ;
#69302=AXIS2_PLACEMENT_3D ( 'NONE', #3624, #58294, #18817 ) ;
#69305=CARTESIAN_POINT ( 'NONE',  ( 88.12195951149128348, 43.65269896049575493, 0.1370767085644951921 ) ) ;
#69312=CARTESIAN_POINT ( 'NONE',  ( 23.42942861845947178, 22.03085787977763133, 9.188101187500006262 ) ) ;
#69315=CARTESIAN_POINT ( 'NONE',  ( 15.46199490364264406, 17.43085787977761925, -9.188101187500008038 ) ) ;
#69317=CARTESIAN_POINT ( 'NONE',  ( 76.80413851785759505, 63.68367294747309870, 15.32454931363362149 ) ) ;
#69318=CARTESIAN_POINT ( 'NONE',  ( 78.24536471662285919, 58.27182448786981439, -16.57828156733082636 ) ) ;
#69321=CARTESIAN_POINT ( 'NONE',  ( 69.61542750552385428, 62.56132062511080250, -13.94275833699888345 ) ) ;
#69329=CARTESIAN_POINT ( 'NONE',  ( 76.91550034648578560, 49.81933278187382541, 15.10848294682921811 ) ) ;
#69330=CARTESIAN_POINT ( 'NONE',  ( 82.56035143084491779, 53.86840602817221679, 15.84327991562212112 ) ) ;
#69337=CARTESIAN_POINT ( 'NONE',  ( 79.11200284437833830, 46.21030595555048137, -12.74531297726273316 ) ) ;
#69343=CARTESIAN_POINT ( 'NONE',  ( 16.91979795264450459, 27.95586893147755347, 7.433330006724141015 ) ) ;
#69344=CARTESIAN_POINT ( 'NONE',  ( 75.64215183828173394, 57.94545888253220767, 16.05204495045250468 ) ) ;
#69353=CARTESIAN_POINT ( 'NONE',  ( 67.91860044382929118, 65.38732574981587220, -10.41618022401985755 ) ) ;
#69363=ORIENTED_EDGE ( 'NONE', *, *, #27630, .T. ) ;
#69365=CARTESIAN_POINT ( 'NONE',  ( 79.11275361910446691, 46.11146926033848104, 13.27945046499836579 ) ) ;
#69366=ORIENTED_EDGE ( 'NONE', *, *, #6493, .F. ) ;
#69371=CARTESIAN_POINT ( 'NONE',  ( 66.97748580458319623, 68.05911003915983315, 6.908000617419038036 ) ) ;
#69376=CARTESIAN_POINT ( 'NONE',  ( 70.78021245458822364, 64.95631462881182472, 12.26071011676762978 ) ) ;
#69382=AXIS2_PLACEMENT_3D ( 'NONE', #25361, #55734, #79106 ) ;
#69384=CARTESIAN_POINT ( 'NONE',  ( 83.70099988003033786, 41.63496273699991690, 0.2210104254450260541 ) ) ;
#69392=ORIENTED_EDGE ( 'NONE', *, *, #66771, .T. ) ;
#69395=CARTESIAN_POINT ( 'NONE',  ( 37.50785463075374793, 23.78380873178789656, -6.180339887498949025 ) ) ;
#69397=CARTESIAN_POINT ( 'NONE',  ( 72.60240557621898461, 70.90654587215668414, 7.620139211458048401 ) ) ;
#69398=CARTESIAN_POINT ( 'NONE',  ( 74.27291791270538113, 66.59407379392037285, -12.66298293614721970 ) ) ;
#69405=CARTESIAN_POINT ( 'NONE',  ( 79.95853045724066988, 47.67161661237850723, 13.37152120557419543 ) ) ;
#69406=CARTESIAN_POINT ( 'NONE',  ( 84.02300986820688422, 51.73893231647484470, 14.78971152351953222 ) ) ;
#69408=ADVANCED_FACE ( 'NONE', ( #34555 ), #40644, .T. ) ;
#69415=CARTESIAN_POINT ( 'NONE',  ( 74.13069305858248015, 55.11053013652369259, 16.60422064088523442 ) ) ;
#69416=CARTESIAN_POINT ( 'NONE',  ( 20.62524822163506144, 36.00034080476291365, -1.878358725466461243E-16 ) ) ;
#69422=LINE ( 'NONE', #54702, #72758 ) ;
#69424=CARTESIAN_POINT ( 'NONE',  ( 66.86435824960236118, 68.17012062228093328, -6.563951195314443154 ) ) ;
#69425=CARTESIAN_POINT ( 'NONE',  ( 72.86910405259970958, 71.04354916989079527, -7.648857478963554613 ) ) ;
#69426=FACE_OUTER_BOUND ( 'NONE', #7783, .T. ) ;
#69429=CARTESIAN_POINT ( 'NONE',  ( 32.29641253342593643, 23.81029122506296503, 8.090169943749479842 ) ) ;
#69430=CARTESIAN_POINT ( 'NONE',  ( 77.02919517786544645, 53.03642993313334841, 16.34676611183340356 ) ) ;
#69432=DIRECTION ( 'NONE',  ( 0.8503781557569334293, -0.05328141121994506291, -0.5234673661555683255 ) ) ;
#69433=CARTESIAN_POINT ( 'NONE',  ( 81.89930626873778863, 42.21375885382297355, 7.647715624843501203 ) ) ;
#69434=CARTESIAN_POINT ( 'NONE',  ( 84.06604358195920668, 51.46910565605918464, 14.65639964578790710 ) ) ;
#69436=CARTESIAN_POINT ( 'NONE',  ( 81.89117822404196545, 41.17241246689844303, 5.587214106818517934 ) ) ;
#69439=CARTESIAN_POINT ( 'NONE',  ( 72.44129552685039641, 70.67501955208014408, -7.848061272651214004 ) ) ;
#69441=CARTESIAN_POINT ( 'NONE',  ( 77.13184676329899503, 49.35096920870304871, -14.90321232162610521 ) ) ;
#69449=CARTESIAN_POINT ( 'NONE',  ( 22.57541804695699028, 15.96004757982090183, -5.678558825948276656 ) ) ;
#69450=CARTESIAN_POINT ( 'NONE',  ( 15.56473500984127512, 9.390406791769814632, -7.779800476318352071E-15 ) ) ;
#69451=CARTESIAN_POINT ( 'NONE',  ( 71.77793909028444830, 59.04410539788438683, 15.86942587573766517 ) ) ;
#69457=CARTESIAN_POINT ( 'NONE',  ( 76.04865552100373804, 58.90167082828886436, -15.97767159145053739 ) ) ;
#69462=CARTESIAN_POINT ( 'NONE',  ( 70.11804512340412998, 70.92857369726408479, -2.377407488624244447 ) ) ;
#69463=CARTESIAN_POINT ( 'NONE',  ( 73.16956295238907160, 57.33411781477383329, 16.38320611710937058 ) ) ;
#69466=VERTEX_POINT ( 'NONE', #41139 ) ;
#69468=CARTESIAN_POINT ( 'NONE',  ( 82.62769229327159337, 42.34900205467494771, -6.013828860758981598 ) ) ;
#69471=CARTESIAN_POINT ( 'NONE',  ( 21.21387930172907588, 35.18080186712593616, 3.090169943749475401 ) ) ;
#69472=CARTESIAN_POINT ( 'NONE',  ( 80.10302014060799536, 57.75140007922345831, 16.60262925785714927 ) ) ;
#69473=CARTESIAN_POINT ( 'NONE',  ( 71.88753435814669501, 69.77153974756373600, -8.727078283019331195 ) ) ;
#69479=VERTEX_POINT ( 'NONE', #87833 ) ;
#69483=DIRECTION ( 'NONE',  ( 0.5000000000000014433, -0.8660254037844378194, 0.000000000000000000 ) ) ;
#69485=ORIENTED_EDGE ( 'NONE', *, *, #30226, .T. ) ;
#69489=CARTESIAN_POINT ( 'NONE',  ( 83.15757460905810206, 52.25129517175852811, 14.83307945656489579 ) ) ;
#69492=CARTESIAN_POINT ( 'NONE',  ( 87.04716231175454766, 46.44793212610622390, 8.841005624941981722 ) ) ;
#69503=CARTESIAN_POINT ( 'NONE',  ( 67.06041821067908870, 66.87374097978496934, 8.879190047928029017 ) ) ;
#69504=CARTESIAN_POINT ( 'NONE',  ( 76.67018723664637037, 63.82874193578962263, -14.84970574671165089 ) ) ;
#69505=CARTESIAN_POINT ( 'NONE',  ( 78.71583768155939254, 47.58229240978521091, 14.26676363293138117 ) ) ;
#69509=CARTESIAN_POINT ( 'NONE',  ( 69.68716675523791082, 63.66678453457147668, 12.72030219626601522 ) ) ;
#69510=CARTESIAN_POINT ( 'NONE',  ( 87.76806118867082773, 45.25231315247835084, -7.033483185435909668 ) ) ;
#69511=CARTESIAN_POINT ( 'NONE',  ( 79.15613078697549554, 46.13387411693875606, 12.67635992270581724 ) ) ;
#69514=CARTESIAN_POINT ( 'NONE',  ( 68.85329997757726517, 65.11108416569004476, -11.21866815422285057 ) ) ;
#69518=CARTESIAN_POINT ( 'NONE',  ( 72.19330168037886608, 71.72436257440323004, 5.504111378373467645 ) ) ;
#69524=CARTESIAN_POINT ( 'NONE',  ( 67.09206164238648284, 67.73860045507836958, -6.489367457569042763 ) ) ;
#69525=B_SPLINE_CURVE_WITH_KNOTS ( 'NONE', 3,
 ( #44720, #12876, #75654, #6239, #37133, #52827, #76168, #6745, #85279, #70023, #93370, #54823, #23925, #16828, #53812, #62929, #78653, #24437, #78149, #15312, #47716, #15825, #38623, #7227, #69025, #61917, #84776, #99955, #92865, #55313, #23419, #46728, #22925, #8736, #77656, #8242, #46211, #30538, #54309, #86294, #85804, #69532, #39108, #142, #16333, #77130 ),
 .UNSPECIFIED., .F., .F.,
 ( 4, 1, 2, 2, 1, 2, 2, 1, 1, 2, 2, 1, 1, 2, 2, 1, 1, 2, 2, 1, 1, 1, 2, 2, 1, 1, 1, 2, 2, 4 ),
 ( 0.000000000000000000, 0.06249999999999114597, 0.09374999999998707978, 0.1249999999999830136, 0.1874999999999724387, 0.2187499999999692746, 0.2499999999999661382, 0.3124999999999595324, 0.3437499999999579225, 0.3593749999999570899, 0.3749999999999562572, 0.4374999999999593103, 0.4687499999999615308, 0.4843749999999631406, 0.4999999999999648059, 0.5624999999999759082, 0.5937499999999826805, 0.6093749999999872324, 0.6249999999999917843, 0.6875000000000135447, 0.7187500000000266454, 0.7343750000000331957, 0.7421875000000341949, 0.7500000000000351941, 0.8125000000000338618, 0.8437500000000348610, 0.8593750000000358602, 0.8671875000000351941, 0.8750000000000327516, 1.000000000000000000 ),
 .UNSPECIFIED. ) ;
#69530=CARTESIAN_POINT ( 'NONE',  ( 85.59595933630416198, 48.93054318311647677, -12.16992291861468978 ) ) ;
#69532=CARTESIAN_POINT ( 'NONE',  ( 70.75100853377770704, 62.48207123928882822, 13.79848856511652500 ) ) ;
#69534=CARTESIAN_POINT ( 'NONE',  ( 87.99879469594441161, 44.76326497867475496, -4.617324391349451496 ) ) ;
#69535=EDGE_CURVE ( 'NONE', #38046, #1759, #50089, .T. ) ;
#69538=CARTESIAN_POINT ( 'NONE',  ( 82.16790899789049263, 41.47445355465299599, -5.920440453570812167 ) ) ;
#69543=B_SPLINE_SURFACE_WITH_KNOTS ( 'NONE', 3, 1, ( 
 ( #74216, #4805 ),
 ( #50880, #58953 ),
 ( #28083, #89925 ),
 ( #82344, #43771 ),
 ( #74716, #44272 ),
 ( #75202, #51891 ),
 ( #46248, #22963 ),
 ( #83318, #92414 ),
 ( #53370, #7267 ),
 ( #83820, #98997 ),
 ( #84812, #75694 ),
 ( #61465, #76680 ),
 ( #13880, #15351 ),
 ( #76204, #36667 ),
 ( #99495, #14386 ),
 ( #45271, #29581 ),
 ( #6780, #38149 ),
 ( #67075, #5779 ),
 ( #67575, #5292 ),
 ( #59963, #84321 ),
 ( #69068, #60458 ),
 ( #37659, #14867 ),
 ( #37175, #53851 ),
 ( #98507, #99995 ),
 ( #29097, #90935 ),
 ( #59457, #44762 ),
 ( #21485, #36172 ),
 ( #30577, #97998 ),
 ( #28578, #68074 ),
 ( #52376, #21010 ),
 ( #68570, #91413 ) ),
 .UNSPECIFIED., .F., .F., .F.,
 ( 4, 3, 3, 3, 3, 3, 3, 3, 3, 3, 4 ),
 ( 2, 2 ),
 ( 0.000000000000000000, 0.1122669598086597914, 0.2243161639709469468, 0.3396355846218949703, 0.4553962076584887608, 0.5677860799922231916, 0.6749047109689442214, 0.7773884377078188468, 0.8775581155834150104, 0.9782364162377956696, 1.000000000000000000 ),
 ( 0.000000000000000000, 1.000000000000000000 ),
 .UNSPECIFIED. ) ;
#69544=CARTESIAN_POINT ( 'NONE',  ( 82.66777534753497036, 40.88273136530058594, 3.288167606880417981 ) ) ;
#69545=ORIENTED_EDGE ( 'NONE', *, *, #42188, .F. ) ;
#69547=CARTESIAN_POINT ( 'NONE',  ( 85.85663799992927636, 46.49267404192337239, -10.33588943598014076 ) ) ;
#69550=CARTESIAN_POINT ( 'NONE',  ( 18.44000607287492954, 15.81029122506293838, 8.090169943749479842 ) ) ;
#69552=CARTESIAN_POINT ( 'NONE',  ( 72.00777348356190544, 59.31339889834504930, -15.33186759774624264 ) ) ;
#69557=CARTESIAN_POINT ( 'NONE',  ( 73.03981800122609513, 57.14498309348731908, 16.39931138066937066 ) ) ;
#69559=CARTESIAN_POINT ( 'NONE',  ( 66.55005611329578130, 68.31410343647267780, -4.333635880301643262 ) ) ;
#69565=CARTESIAN_POINT ( 'NONE',  ( 35.11595366814305663, 25.98920272979928470, 7.433330006724137462 ) ) ;
#69570=CARTESIAN_POINT ( 'NONE',  ( 66.06852073167053163, 68.55763805071961769, 2.146522798610484006 ) ) ;
#69572=CARTESIAN_POINT ( 'NONE',  ( 81.89485588203808675, 55.22971306509116829, 16.24120679747551677 ) ) ;
#69575=CARTESIAN_POINT ( 'NONE',  ( 10.31635424878816742, 24.14336893147753926, 7.433330006724141015 ) ) ;
#69585=ORIENTED_EDGE ( 'NONE', *, *, #45266, .F. ) ;
#69591=CARTESIAN_POINT ( 'NONE',  ( 80.76777501163020645, 45.58789323913284619, -11.58370361122461567 ) ) ;
#69596=CARTESIAN_POINT ( 'NONE',  ( 79.51408477526288721, 59.30329753914238466, -16.21762607725251470 ) ) ;
#69599=CARTESIAN_POINT ( 'NONE',  ( 69.51115086706674617, 62.59482774454561138, 13.31802496749108222 ) ) ;
#69604=CARTESIAN_POINT ( 'NONE',  ( 81.44338780819921908, 42.58957322285800728, -7.672848007371197987 ) ) ;
#69608=EDGE_CURVE ( 'NONE', #15648, #91729, #23824, .T. ) ;
#69612=CARTESIAN_POINT ( 'NONE',  ( 69.44013160124610806, 70.00334490696101852, 4.490412902077236978 ) ) ;
#69615=DIRECTION ( 'NONE',  ( -0.8660254037844379305, -0.5000000000000014433, -0.000000000000000000 ) ) ;
#69618=CARTESIAN_POINT ( 'NONE',  ( 66.43953443436691941, 68.06212878376058484, -4.898982275787033380 ) ) ;
#69620=CARTESIAN_POINT ( 'NONE',  ( 15.46319120177094142, 20.87878583063840665, -9.188101187500006262 ) ) ;
#69625=EDGE_CURVE ( 'NONE', #97296, #22952, #69924, .T. ) ;
#69628=CARTESIAN_POINT ( 'NONE',  ( 80.33508072308801218, 44.92307697338561212, 11.19555900290710326 ) ) ;
#69629=CARTESIAN_POINT ( 'NONE',  ( 67.67903030099223827, 65.78857475430520196, -10.59918437212530762 ) ) ;
#69641=CARTESIAN_POINT ( 'NONE',  ( 16.20451498836328241, 9.759783934591631294, -1.583844403245362020 ) ) ;
#69643=CARTESIAN_POINT ( 'NONE',  ( 72.91771958014867039, 70.92947700147982459, 7.881516594485337812 ) ) ;
#69645=CARTESIAN_POINT ( 'NONE',  ( 76.20853621364400965, 65.14312063949556375, 14.16830839953977872 ) ) ;
#69647=ORIENTED_EDGE ( 'NONE', *, *, #26647, .F. ) ;
#69648=EDGE_CURVE ( 'NONE', #56685, #37549, #66319, .T. ) ;
#69651=CARTESIAN_POINT ( 'NONE',  ( 82.49917951009925332, 46.56262670516255753, -11.60890028354300085 ) ) ;
#69653=CARTESIAN_POINT ( 'NONE',  ( 81.62374368218522136, 41.76230689378201788, 5.959470817902202455 ) ) ;
#69662=CARTESIAN_POINT ( 'NONE',  ( 78.86219776201926379, 59.55369065033505649, 16.50996775951927020 ) ) ;
#69663=B_SPLINE_CURVE_WITH_KNOTS ( 'NONE', 3,
 ( #6104, #98828, #84638, #69398, #7597, #36999, #60279, #54172, #45099, #54675, #52688, #61290, #8110, #15178, #29410, #85659, #93230, #61786, #83649, #91237, #67910, #76512, #21802, #62276, #23790, #38484, #84155, #14208, #29900, #92254, #77518, #501, #14701, #76034, #46079, #31390, #6612, #7096, #37485, #44585, #37977, #15688, #68395, #75520, #14, #68888 ),
 .UNSPECIFIED., .F., .F.,
 ( 4, 1, 2, 2, 1, 2, 2, 1, 1, 2, 2, 1, 1, 2, 2, 1, 1, 2, 2, 1, 1, 1, 2, 2, 1, 1, 1, 2, 2, 4 ),
 ( 0.000000000000000000, 0.06249999999998147315, 0.09374999999997439548, 0.1249999999999673317, 0.1874999999999541755, 0.2187499999999455991, 0.2499999999999369948, 0.3124999999999205635, 0.3437499999999136802, 0.3593749999999097944, 0.3749999999999058531, 0.4374999999999018563, 0.4687499999998997469, 0.4843749999999002465, 0.4999999999999008571, 0.5624999999998997469, 0.5937499999998977485, 0.6093749999998983036, 0.6249999999998988587, 0.6874999999999000799, 0.7187499999999023004, 0.7343749999999018563, 0.7421874999999029665, 0.7499999999999040767, 0.8124999999999173994, 0.8437499999999240607, 0.8593749999999276135, 0.8671874999999309441, 0.8749999999999341638, 1.000000000000000000 ),
 .UNSPECIFIED. ) ;
#69669=CARTESIAN_POINT ( 'NONE',  ( 71.54829379733448036, 63.11566098394168023, 14.24659271140924055 ) ) ;
#69672=CARTESIAN_POINT ( 'NONE',  ( 68.17950952005891452, 67.62522511356370103, 7.807613421983940150 ) ) ;
#69681=CARTESIAN_POINT ( 'NONE',  ( 16.72130706672765754, 10.44966523072493203, -2.296566073217252530E-15 ) ) ;
#69683=FACE_OUTER_BOUND ( 'NONE', #61772, .T. ) ;
#69690=CARTESIAN_POINT ( 'NONE',  ( 36.72872667615778397, 36.90829794293883737, 10.00000000000000355 ) ) ;
#69692=ORIENTED_EDGE ( 'NONE', *, *, #72194, .T. ) ;
#69694=CARTESIAN_POINT ( 'NONE',  ( 26.34264212020660167, 36.18502408145594273, 5.678558825948277544 ) ) ;
#69695=CARTESIAN_POINT ( 'NONE',  ( 77.16259408558386212, 62.51244760150711954, -15.78298705770125920 ) ) ;
#69696=CARTESIAN_POINT ( 'NONE',  ( 81.83903537127142158, 50.54224542843174106, 14.83243049913419753 ) ) ;
#69699=CARTESIAN_POINT ( 'NONE',  ( 84.64469814230420752, 50.57817590239302064, -14.03985074783417630 ) ) ;
#69700=CARTESIAN_POINT ( 'NONE',  ( 75.65276086696347591, 65.13941327059393416, -14.42100060933655570 ) ) ;
#69706=CARTESIAN_POINT ( 'NONE',  ( 33.95706010830453181, 41.64646525600393545, -2.839279412974133887 ) ) ;
#69712=CARTESIAN_POINT ( 'NONE',  ( 86.42645758268480449, 47.01732744055364321, -10.52632212332719064 ) ) ;
#69715=B_SPLINE_CURVE_WITH_KNOTS ( 'NONE', 3,
 ( #16002, #16993, #94540, #79356, #47883, #92546, #78321, #17503, #798, #94045, #84941, #39771, #38794, #69201, #31680, #63099 ),
 .UNSPECIFIED., .F., .F.,
 ( 4, 1, 2, 2, 2, 1, 2, 2, 4 ),
 ( 0.000000000000000000, 0.1249999999999995004, 0.1874999999999998335, 0.2500000000000001665, 0.5000000000000008882, 0.6250000000000018874, 0.6875000000000016653, 0.7500000000000014433, 1.000000000000000000 ),
 .UNSPECIFIED. ) ;
#69716=CARTESIAN_POINT ( 'NONE',  ( 81.90730358699052260, 44.58729832355561484, -10.71401170549568427 ) ) ;
#69717=CARTESIAN_POINT ( 'NONE',  ( 45.46674490716588224, 28.11110640527296312, -2.839279412974138328 ) ) ;
#69718=CARTESIAN_POINT ( 'NONE',  ( 84.88788782112796127, 50.10586950722157695, -13.27192515002011497 ) ) ;
#69723=EDGE_CURVE ( 'NONE', #76194, #89530, #49629, .T. ) ;
#69724=ORIENTED_EDGE ( 'NONE', *, *, #58243, .T. ) ;
#69725=CARTESIAN_POINT ( 'NONE',  ( 81.54419519852100962, 59.48562949720209048, 0.3078307376628255376 ) ) ;
#69729=PLANE ( 'NONE',  #10373 ) ;
#69731=CARTESIAN_POINT ( 'NONE',  ( 32.62753302031853053, 27.03677371833804344, 10.00000000000000533 ) ) ;
#69738=FACE_OUTER_BOUND ( 'NONE', #41423, .T. ) ;
#69739=CARTESIAN_POINT ( 'NONE',  ( 40.50696180670117741, 29.10170272979929962, -7.433330006724141015 ) ) ;
#69743=CARTESIAN_POINT ( 'NONE',  ( 74.09829895435802882, 68.37032454858436381, -11.67432565205426620 ) ) ;
#69744=CARTESIAN_POINT ( 'NONE',  ( 76.92921310806362101, 62.30676013583172335, -15.39267375184458153 ) ) ;
#69747=CARTESIAN_POINT ( 'NONE',  ( 73.47311079653673005, 67.27134392232589732, 11.78844781490330185 ) ) ;
#69750=VERTEX_POINT ( 'NONE', #79586 ) ;
#69752=AXIS2_PLACEMENT_3D ( 'NONE', #93921, #63477, #9282 ) ;
#69753=CARTESIAN_POINT ( 'NONE',  ( 76.94285302476421862, 54.04301539206709037, -16.48480982881932988 ) ) ;
#69759=DIRECTION ( 'NONE',  ( 0.5000000000000014433, -0.8660254037844378194, 0.000000000000000000 ) ) ;
#69768=ORIENTED_EDGE ( 'NONE', *, *, #11902, .F. ) ;
#69770=CARTESIAN_POINT ( 'NONE',  ( 71.75782458564195565, 63.63093110014494869, 13.49702202809486984 ) ) ;
#69779=CARTESIAN_POINT ( 'NONE',  ( 74.78835937171426451, 65.46884208322394727, -13.99351343922952218 ) ) ;
#69781=DIRECTION ( 'NONE',  ( -0.6270036013472530811, -0.3336146661356822474, -0.7039657224870768948 ) ) ;
#69786=CARTESIAN_POINT ( 'NONE',  ( 84.88524026444144965, 50.15864675185714106, -13.30353507586484163 ) ) ;
#69788=CARTESIAN_POINT ( 'NONE',  ( 73.43716180859617282, 69.78348016549323063, -9.856747356917667346 ) ) ;
#69789=CARTESIAN_POINT ( 'NONE',  ( 75.83926582415926987, 51.72761679342552554, 15.75719939435382955 ) ) ;
#69800=CARTESIAN_POINT ( 'NONE',  ( 88.31461815508600921, 44.17477163632586468, -0.1894090640934013026 ) ) ;
#69805=CARTESIAN_POINT ( 'NONE',  ( 28.18775043786755319, 21.98920272979927759, 7.433330006724137462 ) ) ;
#69807=CARTESIAN_POINT ( 'NONE',  ( 79.71556424985024591, 47.75035343155403211, -13.49447772176174531 ) ) ;
#69808=CARTESIAN_POINT ( 'NONE',  ( 7.926391159377050855, 27.68290643055185285, 3.479690158560446702E-15 ) ) ;
#69810=CARTESIAN_POINT ( 'NONE',  ( 77.10487046911684672, 63.70698652748915691, 15.00300083360309067 ) ) ;
#69816=CARTESIAN_POINT ( 'NONE',  ( 77.94754277669224507, 55.87611658206658660, -16.15100785399431160 ) ) ;
#69817=CARTESIAN_POINT ( 'NONE',  ( 87.71125355519491507, 45.00661457325054471, -6.624481356856373182 ) ) ;
#69823=CARTESIAN_POINT ( 'NONE',  ( 82.83837546952335629, 53.74639695667534056, 15.76443799962147452 ) ) ;
#69830=VERTEX_POINT ( 'NONE', #89204 ) ;
#69831=CARTESIAN_POINT ( 'NONE',  ( 79.52155086799245964, 46.24721992604344223, -13.21381413403579863 ) ) ;
#69835=CARTESIAN_POINT ( 'NONE',  ( 26.72152145096863762, 27.37878583063842086, 9.188101187500006262 ) ) ;
#69836=CARTESIAN_POINT ( 'NONE',  ( 79.76359975193354046, 44.98417069036880633, 11.54310746654911135 ) ) ;
#69838=CARTESIAN_POINT ( 'NONE',  ( 75.07571136114331978, 67.05229642490535014, -13.12030194816077788 ) ) ;
#69845=CARTESIAN_POINT ( 'NONE',  ( 67.97956794376455036, 65.69536696150683497, 10.87159683219886297 ) ) ;
#69846=CARTESIAN_POINT ( 'NONE',  ( 68.07222591375136744, 65.60410304735803777, -10.28098472668225050 ) ) ;
#69847=CARTESIAN_POINT ( 'NONE',  ( 81.69437891932362561, 55.22934985428000232, -15.91580060879360659 ) ) ;
#69850=CARTESIAN_POINT ( 'NONE',  ( 71.98264401366868981, 72.39816763649429276, -2.869464145551836598 ) ) ;
#69863=CARTESIAN_POINT ( 'NONE',  ( 66.77969908731566306, 67.50642965742754598, 6.591304754949472766 ) ) ;
#69866=B_SPLINE_SURFACE_WITH_KNOTS ( 'NONE', 3, 1, ( 
 ( #31365, #16173 ),
 ( #30874, #62249 ),
 ( #47069, #77985 ),
 ( #8580, #39445 ),
 ( #98804, #37458 ),
 ( #95729, #72398 ),
 ( #40456, #11092 ),
 ( #70366, #24276 ),
 ( #63271, #33370 ),
 ( #25790, #10081 ),
 ( #17164, #976 ),
 ( #87651, #16668 ),
 ( #1489, #55152 ),
 ( #25267, #64783 ),
 ( #17680, #39946 ),
 ( #71391, #88136 ),
 ( #32370, #80013 ),
 ( #94705, #56151 ),
 ( #40945, #47563 ),
 ( #31855, #1980 ),
 ( #64273, #87148 ),
 ( #49565, #78490 ),
 ( #62757, #26279 ),
 ( #70883, #80516 ),
 ( #57155, #95224 ),
 ( #94211, #56667 ),
 ( #48064, #18682 ),
 ( #49080, #41455 ),
 ( #71892, #32866 ),
 ( #93714, #79006 ),
 ( #2488, #48580 ) ),
 .UNSPECIFIED., .F., .F., .F.,
 ( 4, 3, 3, 3, 3, 3, 3, 3, 3, 3, 4 ),
 ( 2, 2 ),
 ( 0.000000000000000000, 0.1122669598086694226, 0.2243161639709572996, 0.3396355846219043517, 0.4553962076585063579, 0.5677860799922249679, 0.6749047109689459978, 0.7773884377078082997, 0.8775581155834093483, 0.9782364162377646943, 1.000000000000000000 ),
 ( 0.000000000000000000, 1.000000000000000000 ),
 .UNSPECIFIED. ) ;
#69869=CARTESIAN_POINT ( 'NONE',  ( 71.45638833778239984, 66.77805383252390925, 11.11285407077601306 ) ) ;
#69876=CARTESIAN_POINT ( 'NONE',  ( 76.34612012204810583, 51.62224941536150880, -15.67199456353200127 ) ) ;
#69877=CARTESIAN_POINT ( 'NONE',  ( 76.04102746794296763, 65.42908112640478180, -14.38850911432199098 ) ) ;
#69882=B_SPLINE_CURVE_WITH_KNOTS ( 'NONE', 3,
 ( #95189, #85601, #25761, #41426, #444, #62220, #93172, #80998, #26743, #4436, #41939, #95704, #89592, #58617, #3466, #74373 ),
 .UNSPECIFIED., .F., .F.,
 ( 4, 1, 2, 2, 2, 1, 2, 2, 4 ),
 ( 0.000000000000000000, 0.1250000000000004441, 0.1875000000000006661, 0.2500000000000008882, 0.5000000000000014433, 0.6250000000000022204, 0.6875000000000012212, 0.7500000000000002220, 1.000000000000000000 ),
 .UNSPECIFIED. ) ;
#69886=CARTESIAN_POINT ( 'NONE',  ( 80.51198428680065433, 43.68793065238016737, 9.861687463089015893 ) ) ;
#69888=CARTESIAN_POINT ( 'NONE',  ( 72.48986692580926672, 70.61770627562482616, 7.247109231847176147 ) ) ;
#69893=CARTESIAN_POINT ( 'NONE',  ( 82.52387326870589845, 41.00991866554480225, 1.047277955764182700 ) ) ;
#69903=FACE_BOUND ( 'NONE', #89843, .T. ) ;
#69905=CARTESIAN_POINT ( 'NONE',  ( 30.45164419685804091, 25.78052372038641948, -10.00000000000000355 ) ) ;
#69907=CARTESIAN_POINT ( 'NONE',  ( 79.14312167556931854, 57.64441083166269664, 0.000000000000000000 ) ) ;
#69914=FACE_OUTER_BOUND ( 'NONE', #77499, .T. ) ;
#69919=CARTESIAN_POINT ( 'NONE',  ( 24.32480936679734640, 35.81751292744057480, -6.180339887498951690 ) ) ;
#69920=CARTESIAN_POINT ( 'NONE',  ( 82.54706635703216477, 41.64549635078170553, -4.312970195963365505 ) ) ;
#69922=CARTESIAN_POINT ( 'NONE',  ( 72.27059105936884009, 62.71376582020941726, 14.64825672156503522 ) ) ;
#69924=LINE ( 'NONE', #16735, #6417 ) ;
#69927=CARTESIAN_POINT ( 'NONE',  ( 71.70518999464594856, 66.55211070663439443, -11.44409006190726608 ) ) ;
#69930=CARTESIAN_POINT ( 'NONE',  ( 72.71813417941989144, 70.76084006159408091, -7.966439650937871875 ) ) ;
#69931=CARTESIAN_POINT ( 'NONE',  ( 79.14312167556931854, 57.64441083166269664, 0.000000000000000000 ) ) ;
#69933=FACE_OUTER_BOUND ( 'NONE', #6613, .T. ) ;
#69935=AXIS2_PLACEMENT_3D ( 'NONE', #33654, #9861, #94980 ) ;
#69940=CARTESIAN_POINT ( 'NONE',  ( 26.24098094315136009, 17.01110640527292972, 2.839279412974134775 ) ) ;
#69941=CARTESIAN_POINT ( 'NONE',  ( 10.99774771173347432, 18.30066082961419838, -10.00000000000000533 ) ) ;
#69945=CARTESIAN_POINT ( 'NONE',  ( 43.91732790946529263, 25.75978393459167748, -1.583844403245362020 ) ) ;
#69946=CARTESIAN_POINT ( 'NONE',  ( 7.976297994771393896, 26.64646525600388571, -2.839279412974133887 ) ) ;
#69947=CARTESIAN_POINT ( 'NONE',  ( 72.40192626949962573, 60.07796831195529563, -15.19260960954916584 ) ) ;
#69948=CARTESIAN_POINT ( 'NONE',  ( 88.28941560846926961, 44.33790759572318052, 2.269834333188780473 ) ) ;
#69951=CARTESIAN_POINT ( 'NONE',  ( 71.31109310106401722, 71.30997890262395345, -3.879444360706853168 ) ) ;
#69953=CARTESIAN_POINT ( 'NONE',  ( 77.12096872831645555, 63.68411177576406601, 15.01383154859763280 ) ) ;
#69954=CARTESIAN_POINT ( 'NONE',  ( 86.21323549116458196, 43.83733327322993745, 5.984240272472757027 ) ) ;
#69955=EDGE_CURVE ( 'NONE', #95607, #23731, #30667, .T. ) ;
#69959=CARTESIAN_POINT ( 'NONE',  ( 86.05652331311144110, 43.10072823858845936, -2.262228719805865484 ) ) ;
#69963=CARTESIAN_POINT ( 'NONE',  ( 80.28041774221068749, 57.81736701477463924, 16.60186235868147619 ) ) ;
#69964=CARTESIAN_POINT ( 'NONE',  ( 77.07103148522583069, 63.64506183647083759, 15.39324216548719626 ) ) ;
#69969=DIRECTION ( 'NONE',  ( 0.3213938048432692374, -0.5566703992264209200, -0.7660444431189770143 ) ) ;
#69972=CARTESIAN_POINT ( 'NONE',  ( 28.45357225853751260, 28.37878583063842441, 9.188101187500006262 ) ) ;
#69974=FACE_OUTER_BOUND ( 'NONE', #66724, .T. ) ;
#69979=CARTESIAN_POINT ( 'NONE',  ( 83.42767843756884361, 52.41288616963773705, 14.83540219176039798 ) ) ;
#69981=VERTEX_POINT ( 'NONE', #86303 ) ;
#69984=CARTESIAN_POINT ( 'NONE',  ( 69.13686587061594935, 64.31895405193962745, 11.99662287724232357 ) ) ;
#69987=VERTEX_POINT ( 'NONE', #16837 ) ;
#69994=CARTESIAN_POINT ( 'NONE',  ( 69.69662549137501628, 67.03661573462981949, 9.803235490692268073 ) ) ;
#69996=CARTESIAN_POINT ( 'NONE',  ( 67.64562412842587946, 66.75646473445011964, 8.610110601876797887 ) ) ;
#69997=CARTESIAN_POINT ( 'NONE',  ( 69.28028072256803682, 65.61004360350007403, -10.97831167068993352 ) ) ;
#69998=CARTESIAN_POINT ( 'NONE',  ( 77.95184231570208055, 47.94166338610092026, 14.11904032283977806 ) ) ;
#70002=CARTESIAN_POINT ( 'NONE',  ( 69.83162332184129184, 64.07449313801377855, 12.49715358904647466 ) ) ;
#70003=CARTESIAN_POINT ( 'NONE',  ( 68.22205435738101187, 65.90345407221148832, 10.80313017757570826 ) ) ;
#70004=VECTOR ( 'NONE', #59974, 1000.000000000000114 ) ;
#70007=CARTESIAN_POINT ( 'NONE',  ( 83.42542119994749328, 51.64995580955419996, -14.90072893730333270 ) ) ;
#70011=CARTESIAN_POINT ( 'NONE',  ( 72.11459644421852033, 71.43304111169508985, 5.074525307012419439 ) ) ;
#70021=CARTESIAN_POINT ( 'NONE',  ( 69.59316709322138195, 66.26231169737734206, -10.55197826579468057 ) ) ;
#70023=CARTESIAN_POINT ( 'NONE',  ( 72.49757734898066985, 67.98224297600880561, 10.61344264115449576 ) ) ;
#70024=CARTESIAN_POINT ( 'NONE',  ( 87.97078667614408687, 44.76483236400627419, -4.665040245107967110 ) ) ;
#70028=ADVANCED_FACE ( 'NONE', ( #71063 ), #62421, .T. ) ;
#70030=CARTESIAN_POINT ( 'NONE',  ( 81.53115339410011586, 41.92267797703283350, -7.515177224638169839 ) ) ;
#70032=CARTESIAN_POINT ( 'NONE',  ( 45.64937871703416761, 26.75978393459169880, -1.583844403245396437 ) ) ;
#70036=CARTESIAN_POINT ( 'NONE',  ( 9.939249538635717585, 29.23654200823201421, 1.583844403245363353 ) ) ;
#70038=CARTESIAN_POINT ( 'NONE',  ( 20.60277255440211164, 12.86426979415089278, -3.090169943749474069 ) ) ;
#70045=CARTESIAN_POINT ( 'NONE',  ( 72.90739036693749142, 57.16012815389416346, 15.90261827893724167 ) ) ;
#70047=CARTESIAN_POINT ( 'NONE',  ( 66.75732258258473450, 68.40744662148340183, -4.417456331192459729 ) ) ;
#70052=CARTESIAN_POINT ( 'NONE',  ( 32.17146729527596705, 24.28920272979928541, -7.433330006724141015 ) ) ;
#70058=CARTESIAN_POINT ( 'NONE',  ( 66.10824223320386750, 68.56859800295461582, 2.217169679141618666 ) ) ;
#70059=EDGE_LOOP ( 'NONE', ( #88526, #50286, #16705, #37344 ) ) ;
#70063=CARTESIAN_POINT ( 'NONE',  ( 6.332637391379750014, 21.84336893147753855, -7.433330006724137462 ) ) ;
#70069=CARTESIAN_POINT ( 'NONE',  ( 71.51113537273405996, 72.37632541024544253, 1.045464050329093286 ) ) ;
#70070=CARTESIAN_POINT ( 'NONE',  ( 31.08397696812772182, 23.11029122506295863, -8.090169943749478065 ) ) ;
#70075=VERTEX_POINT ( 'NONE', #69544 ) ;
#70079=ORIENTED_EDGE ( 'NONE', *, *, #23730, .T. ) ;
#70080=CARTESIAN_POINT ( 'NONE',  ( 71.59728507587232116, 70.99594489426432631, 6.387564926741087667 ) ) ;
#70081=EDGE_CURVE ( 'NONE', #65113, #53392, #64393, .T. ) ;
#70085=ADVANCED_FACE ( 'NONE', ( #56833 ), #87818, .T. ) ;
#70086=CARTESIAN_POINT ( 'NONE',  ( 79.46674400240780756, 59.17914826126551731, -16.22576502784502139 ) ) ;
#70090=CARTESIAN_POINT ( 'NONE',  ( 69.71741781551351380, 62.54328943123160656, 13.41580856235687769 ) ) ;
#70098=CARTESIAN_POINT ( 'NONE',  ( 74.45444392623342367, 66.27966151248681115, 12.94663026855831411 ) ) ;
#70103=CARTESIAN_POINT ( 'NONE',  ( 83.35356881092343428, 49.56826083113291759, 13.41475373279179095 ) ) ;
#70109=CARTESIAN_POINT ( 'NONE',  ( 79.49634071307748684, 55.47133629792779175, -16.47986696218380587 ) ) ;
#70110=CARTESIAN_POINT ( 'NONE',  ( 21.21803360120161486, 14.11110640527291871, -2.839279412974138328 ) ) ;
#70112=CARTESIAN_POINT ( 'NONE',  ( 80.03994542435373205, 57.65115798690545290, 16.60126445886217539 ) ) ;
#70114=ORIENTED_EDGE ( 'NONE', *, *, #95300, .F. ) ;
#70120=FACE_OUTER_BOUND ( 'NONE', #488, .T. ) ;
#70128=CARTESIAN_POINT ( 'NONE',  ( 16.16012747849099540, 9.734156793818206310, 1.333680081654574804E-15 ) ) ;
#70132=CARTESIAN_POINT ( 'NONE',  ( 75.74251350868291865, 65.46771939187904366, 14.28157630633085518 ) ) ;
#70133=EDGE_CURVE ( 'NONE', #86521, #38635, #14284, .T. ) ;
#70140=CARTESIAN_POINT ( 'NONE',  ( 85.97138696049607631, 45.97668872975567211, -9.009752818326484558 ) ) ;
#70147=EDGE_LOOP ( 'NONE', ( #2908, #16998, #93212, #53128 ) ) ;
#70149=EDGE_CURVE ( 'NONE', #68627, #47421, #12251, .T. ) ;
#70150=CARTESIAN_POINT ( 'NONE',  ( 88.22000632671871756, 44.27423112938743088, 4.003506518527984781 ) ) ;
#70153=CARTESIAN_POINT ( 'NONE',  ( 80.65296072109273950, 57.47057263566300378, -16.23811142086485759 ) ) ;
#70167=ORIENTED_EDGE ( 'NONE', *, *, #19104, .T. ) ;
#70172=CARTESIAN_POINT ( 'NONE',  ( 16.50122538818396478, 18.03085787977762422, 9.188101187500006262 ) ) ;
#70181=CARTESIAN_POINT ( 'NONE',  ( 33.33823495471120424, 42.18080186712595747, 3.090169943749475401 ) ) ;
#70182=CARTESIAN_POINT ( 'NONE',  ( 86.31939919580703702, 47.65601329950942500, 10.71069801041972447 ) ) ;
#70191=CARTESIAN_POINT ( 'NONE',  ( 72.39195994751899832, 71.88450172447629427, -5.391213119607743742 ) ) ;
#70196=CARTESIAN_POINT ( 'NONE',  ( 40.27059248445925732, 25.11110640527295601, -2.839279412974138328 ) ) ;
#70202=CARTESIAN_POINT ( 'NONE',  ( 79.58936028502597537, 59.22294857574253513, 16.56770033466461811 ) ) ;
#70205=B_SPLINE_CURVE_WITH_KNOTS ( 'NONE', 3,
 ( #79405, #2377, #4871, #42829, #19082, #49959, #98065, #59524, #81893, #51445, #74287, #89037, #43339, #73763, #20070, #59020 ),
 .UNSPECIFIED., .F., .F.,
 ( 4, 1, 2, 2, 2, 1, 2, 2, 4 ),
 ( 0.000000000000000000, 0.1249999999999980016, 0.1874999999999987232, 0.2499999999999994449, 0.4999999999999982236, 0.6249999999999958922, 0.6874999999999965583, 0.7499999999999972244, 1.000000000000000000 ),
 .UNSPECIFIED. ) ;
#70207=CARTESIAN_POINT ( 'NONE',  ( 83.31676998715261107, 44.47964662621878063, -9.710295204768222277 ) ) ;
#70210=CARTESIAN_POINT ( 'NONE',  ( 43.97106342183892735, 31.10170272979931028, -7.433330006724141015 ) ) ;
#70211=CARTESIAN_POINT ( 'NONE',  ( 80.44421536292240660, 44.39010815972903146, 11.34380831960723945 ) ) ;
#70212=CARTESIAN_POINT ( 'NONE',  ( 84.79901702372750094, 50.05075620941028092, -13.68787013058487290 ) ) ;
#70220=CARTESIAN_POINT ( 'NONE',  ( 77.14916621374221961, 49.44515670615653136, -15.44477560956883799 ) ) ;
#70223=CARTESIAN_POINT ( 'NONE',  ( 87.00169912441755571, 45.80253757415765392, -8.636720921146656238 ) ) ;
#70224=CARTESIAN_POINT ( 'NONE',  ( 78.92544819766602870, 51.82601731205822659, 15.40366229040229484 ) ) ;
#70226=LINE ( 'NONE', #99155, #41072 ) ;
#70230=CARTESIAN_POINT ( 'NONE',  ( 82.81737761417261368, 40.62361263855670046, 0.9906565628550747515 ) ) ;
#70236=CARTESIAN_POINT ( 'NONE',  ( 70.67277294938870114, 60.56909423328382047, -14.64600609532338993 ) ) ;
#70237=CARTESIAN_POINT ( 'NONE',  ( 36.06377727768691699, 41.79752408145595410, -5.678558825948271327 ) ) ;
#70246=CARTESIAN_POINT ( 'NONE',  ( 71.75200176415748388, 60.74830010697920812, 14.83125165669016177 ) ) ;
#70247=CARTESIAN_POINT ( 'NONE',  ( 66.51217979237357270, 68.21896002327083863, 4.555124048972479578 ) ) ;
#70249=CARTESIAN_POINT ( 'NONE',  ( 36.94473716931751284, 21.73415679381824361, -6.890680421881970419E-14 ) ) ;
#70265=CARTESIAN_POINT ( 'NONE',  ( 73.25245674375855742, 68.31447868205536622, 10.71232302521148405 ) ) ;
#70266=CARTESIAN_POINT ( 'NONE',  ( 72.15234558402282516, 59.70125055744302500, 15.74980178838212730 ) ) ;
#70272=CARTESIAN_POINT ( 'NONE',  ( 74.11561865490956791, 68.62363639872573629, 10.95723244528671714 ) ) ;
#70273=CARTESIAN_POINT ( 'NONE',  ( 71.85042758235270810, 71.69843285251393183, -3.789477364735254650 ) ) ;
#70279=EDGE_CURVE ( 'NONE', #5574, #79014, #552, .T. ) ;
#70281=CARTESIAN_POINT ( 'NONE',  ( 78.30031128316109346, 56.39945258195061228, 16.19534353207165012 ) ) ;
#70282=CARTESIAN_POINT ( 'NONE',  ( 84.88560255493293027, 50.09086853330895650, -13.26386351457619206 ) ) ;
#70285=CARTESIAN_POINT ( 'NONE',  ( 76.18389692386300283, 51.34301906948758187, 15.63209118771619366 ) ) ;
#70290=( BOUNDED_SURFACE ( )  B_SPLINE_SURFACE ( 1, 2, ( 
 ( #20612, #81937, #51493, #52987, #67189, #91036, #92044, #35798, #13515, #83432, #6886, #60074, #83935, #66692, #68678, #13998, #44877, #75817, #6402, #12515, #90550, #98624, #59575, #43387, #82462, #60569, #37286, #36787, #13024, #74329, #43887, #68181, #99110, #4918, #29693, #36290, #98113, #99609, #91525, #22089, #45381, #30187, #97628, #28192, #74826, #28698, #21122, #51998, #75316, #67696, #16483, #61574, #14975, #84922, #62063, #69681, #8884, #47865, #32682, #39752, #45862, #779, #78802, #93012, #47377, #38269, #31666, #92525, #63582, #23566, #85956, #31173, #69180, #7900, #39260, #55462, #9390, #54457, #100110, #93525, #40266, #76787, #1798, #24579, #85436, #22589, #15985, #62562, #16974, #53479, #71206, #70172, #46884, #78302, #24082, #30694, #84430, #54978, #70681, #285, #1295, #77809, #8392, #32180, #7380, #63083, #94028, #86449, #23071, #53965, #15468, #46363, #77292, #38775, #64087, #57470, #25595, #88453, #26596, #2306, #33703, #27098, #65580, #79830, #41267, #18501, #10398, #49387, #25076, #34678, #55956, #33187, #86951, #3313, #80332, #17484, #9905, #50378, #48896, #56481, #34193, #19012, #49886, #48392, #87956, #95031, #64596, #4276, #87469, #10900, #57981, #65084, #79335, #35175, #42760, #11415, #80845, #18004, #42269, #96528, #73202, #3797, #72210, #73692, #95549, #81331, #88964, #11903, #94524, #19518, #40763, #71714, #2814, #72722, #26097, #56971, #41776, #96035, #91405, #75688, #37169, #89439, #52863, #29091, #36165, #12398, #43264, #21970, #83813, #75197, #44755, #67568, #82338, #36661, #67068, #13394, #52367, #20498, #97992, #21004, #51370, #6274, #14380, #5772, #66581, #97505, #6774, #74209, #66086, #21479, #45264, #98991, #59451, #51885, #68067, #44265, #83312, #76198, #35680, #90929, #90432, #29574, #13874, #5286, #97032, #4799, #60452, #58467, #59957, #27601, #98501, #19995, #12906, #50874, #81823, #74709, #28075, #58947, #28571, #89918, #43765, #82826, #31552, #78685, #15345, #99489, #8769, #77691, #8274, #47748, #22470, #172, #39139, #62963, #15858, #70560, #53364, #55347, #70052, #667, #62441, #46765, #37653, #77167, #85312, #46241, #68564, #76673, #47259, #93408, #92897, #7260, #30067, #38143, #23957, #54860, #60956, #85838, #92408, #22956, #93913, #16368, #78180, #1177, #16861, #39638, #32051, #91915, #24467, #86324, #84314, #14861, #69565, #45748, #69060, #99989, #30573, #7769, #84805, #61458, #53845, #38662, #31056, #61945, #23450, #54340, #48781, #34085, #24958, #87840, #48269, #50257, #79713, #72596, #17883, #55834, #94902, #25984, #42153, #65461, #10276, #86829, #80211, #96403, #63468, #88834, #11294, #41146, #19398, #72084, #49274, #3682, #9274, #34561, #56854, #2685, #3201, #10779, #17362, #40147, #18379, #64975, #87354, #41654, #33576, #64471, #95918, #26972, #95431, #26478, #73088, #79216, #71088, #1687, #88330, #32572, #57354, #9790, #18885, #40650, #49765, #80720, #71588, #2183, #33066, #57854, #94404, #63960, #25465, #56354, #47437, #78870, #8946, #9455, #49442, #63645, #25661, #40326, #39814, #87016, #41331, #17544, #94088, #32740, #64146, #80397, #3377, #48453, #55521, #64658, #65146, #63143, #70746, #10967, #79396, #71266, #40824, #57032, #25137, #71768, #2368 ),
 ( #88015, #33245, #95097, #56540, #18564, #59516, #75256, #59011, #19577, #50438, #60019, #27158, #19074, #74769, #67630, #51944, #12460, #4861, #28631, #97569, #36228, #36725, #89027, #43829, #43331, #21067, #5347, #58529, #49948, #96595, #90494, #11478, #12968, #5836, #51436, #82883, #35241, #89978, #20557, #27661, #82402, #98563, #50934, #81393, #13458, #11959, #67133, #80906, #97092, #42332, #44324, #98055, #20061, #29148, #73259, #66145, #81883, #74277, #35743, #66639, #3854, #34738, #65639, #58045, #42821, #28138, #73752, #52426, #6337, #46824, #45321, #52926, #30633, #15406, #53906, #83373, #84368, #29636, #61009, #719, #99054, #76729, #54397, #61519, #75753, #31607, #39198, #7833, #77226, #60509, #46300, #99544, #92465, #77747, #22531, #68622, #92952, #91466, #90983, #13937, #69620, #21543, #38714, #22026, #84864, #83878, #227, #23011, #14440, #76256, #37228, #31112, #62000, #23505, #30126, #91981, #70110, #6828, #44817, #37713, #85374, #53419, #15918, #68126, #14916, #45805, #8330, #7322, #69120, #38201, #100047, #80273, #64027, #2247, #94968, #40712, #3256, #1747, #9853, #71148, #62497, #1231, #72147, #33126, #17423, #32113, #93467, #63023, #25533, #56420, #72661, #17945, #16918, #47806, #18444, #87417, #48844, #95491, #41715, #71655, #26043, #24019, #49333, #79776, #87900, #10341, #94463, #41207, #93968, #54917, #24521, #32626, #9330, #2750, #10837, #85896, #33641, #16421, #64533, #47316, #63524, #56913, #78241, #8822, #55400, #39690, #25016, #70619, #55896, #86385, #78741, #79279, #40202, #86889, #48332, #26540, #96470, #11843, #95978, #42701, #50318, #42212, #73633, #73148, #65520, #81269, #34138, #65032, #57920, #27035, #57413, #19461, #49827, #88394, #18948, #80784, #88899, #11358, #3745, #34620, #17800, #63385, #71508, #16281, #71006, #1608, #39556, #94325, #10199, #62876, #586, #32979, #23873, #24880, #72000, #8687, #92817, #2099, #32494, #70480, #63884, #94820, #47175, #78096, #55261, #1094, #86243, #61866, #25384, #23371, #69972, #54257, #40064, #16779, #85228, #46680, #87269, #85752, #93319, #55754, #86747, #17281, #15774, #24388, #31471, #31971, #41063, #39059, #47671, #56272, #48185, #77606, #30979, #79633, #79131, #9711, #62362, #40568, #48699, #8191, #54773, #93834, #78603, #9189, #91095, #73997, #60135, #83494, #34971, #49199, #65873, #21663, #81136, #34010, #18797, #14060, #98685, #29265, #12193, #5960, #25907, #52543, #96829, #73011, #80133, #10696, #44941, #2605, #11702, #81620, #4079, #49679, #73496, #3603, #50182, #89251, #57273, #34482, #57772, #88249, #43052, #33493, #42562, #3125, #64895, #64388, #41575, #95352, #58275, #56779, #36851, #96324, #88746, #67760, #27392, #19801, #87762, #72516, #50668, #26894, #18301, #95841, #42079, #26396, #80635, #11212, #65381, #19319, #8450, #55033, #23130, #39321, #16542, #62626, #54025, #841, #46427, #7441, #69739, #14564, #68244, #37837, #15034, #22657, #62122, #31722, #86015, #93070, #99168, #84980, #93581, #45926, #348, #91582, #15526, #45439, #75885, #76843, #38833, #84491, #22156, #61135, #92587, #70237, #24148, #38333, #53046, #77352, #6463, #29756, #37342, #77864, #69241, #60628, #100171, #7959, #84003, #76374, #6945, #31236, #30757 ) ),
 .UNSPECIFIED., .F., .F., .T. ) 
 B_SPLINE_SURFACE_WITH_KNOTS ( ( 2, 2 ),
 ( 3, 2, 2, 2, 2, 2, 2, 2, 2, 2, 2, 2, 2, 2, 2, 2, 2, 2, 2, 2, 2, 2, 2, 2, 2, 2, 2, 2, 2, 2, 2, 2, 2, 2, 2, 2, 2, 2, 2, 2, 2, 2, 2, 2, 2, 2, 2, 2, 2, 2, 2, 2, 2, 2, 2, 2, 2, 2, 2, 2, 2, 2, 2, 2, 2, 2, 2, 2, 2, 2, 2, 2, 2, 2, 2, 2, 2, 2, 2, 2, 2, 2, 2, 2, 2, 2, 2, 2, 2, 2, 2, 2, 2, 2, 2, 2, 2, 2, 2, 2, 2, 2, 2, 2, 2, 2, 2, 2, 2, 2, 2, 2, 2, 2, 2, 2, 2, 2, 2, 2, 2, 2, 2, 2, 2, 2, 2, 2, 2, 2, 2, 2, 2, 2, 2, 2, 2, 2, 2, 2, 2, 2, 2, 2, 2, 2, 2, 2, 2, 2, 2, 2, 2, 2, 2, 2, 2, 2, 2, 2, 2, 2, 2, 2, 2, 2, 2, 2, 2, 2, 2, 2, 2, 2, 2, 2, 2, 2, 2, 2, 2, 2, 2, 2, 2, 2, 2, 2, 2, 2, 2, 2, 2, 2, 2, 2, 2, 2, 2, 2, 3 ),
 ( 0.000000000000000000, 1.000000000000000000 ),
 ( 0.000000000000000000, 0.005000000000000000104, 0.01000000000000000021, 0.01499999999999999944, 0.02000000000000000042, 0.02500000000000000139, 0.02999999999999999889, 0.03500000000000000333, 0.04000000000000000083, 0.04499999999999999833, 0.05000000000000000278, 0.05500000000000000028, 0.05999999999999999778, 0.06500000000000000222, 0.07000000000000000666, 0.07499999999999999722, 0.08000000000000000167, 0.08500000000000000611, 0.08999999999999999667, 0.09500000000000000111, 0.1000000000000000056, 0.1049999999999999961, 0.1100000000000000006, 0.1150000000000000050, 0.1199999999999999956, 0.1250000000000000000, 0.1300000000000000044, 0.1350000000000000089, 0.1400000000000000133, 0.1449999999999999900, 0.1499999999999999944, 0.1549999999999999989, 0.1600000000000000033, 0.1650000000000000078, 0.1700000000000000122, 0.1749999999999999889, 0.1799999999999999933, 0.1849999999999999978, 0.1900000000000000022, 0.1950000000000000067, 0.2000000000000000111, 0.2049999999999999878, 0.2099999999999999922, 0.2149999999999999967, 0.2200000000000000011, 0.2250000000000000056, 0.2300000000000000100, 0.2349999999999999867, 0.2399999999999999911, 0.2449999999999999956, 0.2500000000000000000, 0.2550000000000000044, 0.2600000000000000089, 0.2650000000000000133, 0.2700000000000000178, 0.2750000000000000222, 0.2800000000000000266, 0.2849999999999999756, 0.2899999999999999800, 0.2949999999999999845, 0.2999999999999999889, 0.3049999999999999933, 0.3099999999999999978, 0.3150000000000000022, 0.3200000000000000067, 0.3250000000000000111, 0.3300000000000000155, 0.3350000000000000200, 0.3400000000000000244, 0.3449999999999999734, 0.3499999999999999778, 0.3549999999999999822, 0.3599999999999999867, 0.3649999999999999911, 0.3699999999999999956, 0.3750000000000000000, 0.3800000000000000044, 0.3850000000000000089, 0.3900000000000000133, 0.3950000000000000178, 0.4000000000000000222, 0.4050000000000000266, 0.4099999999999999756, 0.4149999999999999800, 0.4199999999999999845, 0.4249999999999999889, 0.4299999999999999933, 0.4349999999999999978, 0.4400000000000000022, 0.4450000000000000067, 0.4500000000000000111, 0.4550000000000000155, 0.4600000000000000200, 0.4650000000000000244, 0.4699999999999999734, 0.4749999999999999778, 0.4799999999999999822, 0.4849999999999999867, 0.4899999999999999911, 0.4949999999999999956, 0.5000000000000000000, 0.5050000000000000044, 0.5100000000000000089, 0.5150000000000000133, 0.5200000000000000178, 0.5250000000000000222, 0.5300000000000000266, 0.5350000000000000311, 0.5400000000000000355, 0.5450000000000000400, 0.5500000000000000444, 0.5550000000000000488, 0.5600000000000000533, 0.5649999999999999467, 0.5699999999999999512, 0.5749999999999999556, 0.5799999999999999600, 0.5849999999999999645, 0.5899999999999999689, 0.5949999999999999734, 0.5999999999999999778, 0.6049999999999999822, 0.6099999999999999867, 0.6149999999999999911, 0.6199999999999999956, 0.6250000000000000000, 0.6300000000000000044, 0.6350000000000000089, 0.6400000000000000133, 0.6450000000000000178, 0.6500000000000000222, 0.6550000000000000266, 0.6600000000000000311, 0.6650000000000000355, 0.6700000000000000400, 0.6750000000000000444, 0.6800000000000000488, 0.6850000000000000533, 0.6899999999999999467, 0.6949999999999999512, 0.6999999999999999556, 0.7049999999999999600, 0.7099999999999999645, 0.7149999999999999689, 0.7199999999999999734, 0.7249999999999999778, 0.7299999999999999822, 0.7349999999999999867, 0.7399999999999999911, 0.7449999999999999956, 0.7500000000000000000, 0.7550000000000000044, 0.7600000000000000089, 0.7650000000000000133, 0.7700000000000000178, 0.7750000000000000222, 0.7800000000000000266, 0.7850000000000000311, 0.7900000000000000355, 0.7950000000000000400, 0.8000000000000000444, 0.8050000000000000488, 0.8100000000000000533, 0.8149999999999999467, 0.8199999999999999512, 0.8249999999999999556, 0.8299999999999999600, 0.8349999999999999645, 0.8399999999999999689, 0.8449999999999999734, 0.8499999999999999778, 0.8549999999999999822, 0.8599999999999999867, 0.8649999999999999911, 0.8699999999999999956, 0.8750000000000000000, 0.8800000000000000044, 0.8850000000000000089, 0.8900000000000000133, 0.8950000000000000178, 0.9000000000000000222, 0.9050000000000000266, 0.9100000000000000311, 0.9150000000000000355, 0.9200000000000000400, 0.9250000000000000444, 0.9300000000000000488, 0.9350000000000000533, 0.9399999999999999467, 0.9449999999999999512, 0.9499999999999999556, 0.9549999999999999600, 0.9599999999999999645, 0.9649999999999999689, 0.9699999999999999734, 0.9749999999999999778, 0.9799999999999999822, 0.9849999999999999867, 0.9899999999999999911, 0.9949999999999999956, 1.000000000000000000 ),
 .UNSPECIFIED. ) 
 GEOMETRIC_REPRESENTATION_ITEM ( )  RATIONAL_B_SPLINE_SURFACE ( (
 ( 1.000000000000000000, 0.9510565162951535312, 1.000000000000000000, 0.9510565162951535312, 1.000000000000000000, 0.9510565162951535312, 1.000000000000000000, 0.9510565162951535312, 1.000000000000000000, 0.9510565162951535312, 1.000000000000000000, 0.9510565162951535312, 1.000000000000000000, 0.9510565162951535312, 1.000000000000000000, 0.9510565162951535312, 1.000000000000000000, 0.9510565162951535312, 1.000000000000000000, 0.9510565162951535312, 1.000000000000000000, 0.9510565162951535312, 1.000000000000000000, 0.9510565162951535312, 1.000000000000000000, 0.9510565162951535312, 1.000000000000000000, 0.9510565162951535312, 1.000000000000000000, 0.9510565162951535312, 1.000000000000000000, 0.9510565162951535312, 1.000000000000000000, 0.9510565162951535312, 1.000000000000000000, 0.9510565162951535312, 1.000000000000000000, 0.9510565162951535312, 1.000000000000000000, 0.9510565162951535312, 1.000000000000000000, 0.9510565162951535312, 1.000000000000000000, 0.9510565162951535312, 1.000000000000000000, 0.9510565162951535312, 1.000000000000000000, 0.9510565162951535312, 1.000000000000000000, 0.9510565162951535312, 1.000000000000000000, 0.9510565162951535312, 1.000000000000000000, 0.9510565162951535312, 1.000000000000000000, 0.9510565162951535312, 1.000000000000000000, 0.9510565162951535312, 1.000000000000000000, 0.9510565162951535312, 1.000000000000000000, 0.9510565162951535312, 1.000000000000000000, 0.9510565162951535312, 1.000000000000000000, 0.9510565162951535312, 1.000000000000000000, 0.9510565162951535312, 1.000000000000000000, 0.9510565162951535312, 1.000000000000000000, 0.9510565162951535312, 1.000000000000000000, 0.9510565162951535312, 1.000000000000000000, 0.9510565162951535312, 1.000000000000000000, 0.9510565162951535312, 1.000000000000000000, 0.9510565162951535312, 1.000000000000000000, 0.9510565162951535312, 1.000000000000000000, 0.9510565162951535312, 1.000000000000000000, 0.9510565162951535312, 1.000000000000000000, 0.9510565162951535312, 1.000000000000000000, 0.9510565162951535312, 1.000000000000000000, 0.9510565162951535312, 1.000000000000000000, 0.9510565162951535312, 1.000000000000000000, 0.9510565162951535312, 1.000000000000000000, 0.9510565162951535312, 1.000000000000000000, 0.9510565162951535312, 1.000000000000000000, 0.9510565162951535312, 1.000000000000000000, 0.9510565162951535312, 1.000000000000000000, 0.9510565162951535312, 1.000000000000000000, 0.9510565162951535312, 1.000000000000000000, 0.9510565162951535312, 1.000000000000000000, 0.9510565162951535312, 1.000000000000000000, 0.9510565162951535312, 1.000000000000000000, 0.9510565162951535312, 1.000000000000000000, 0.9510565162951535312, 1.000000000000000000, 0.9510565162951535312, 1.000000000000000000, 0.9510565162951535312, 1.000000000000000000, 0.9510565162951535312, 1.000000000000000000, 0.9510565162951535312, 1.000000000000000000, 0.9510565162951535312, 1.000000000000000000, 0.9510565162951535312, 1.000000000000000000, 0.9510565162951535312, 1.000000000000000000, 0.9510565162951535312, 1.000000000000000000, 0.9510565162951535312, 1.000000000000000000, 0.9510565162951535312, 1.000000000000000000, 0.9510565162951535312, 1.000000000000000000, 0.9510565162951535312, 1.000000000000000000, 0.9510565162951535312, 1.000000000000000000, 0.9510565162951535312, 1.000000000000000000, 0.9510565162951535312, 1.000000000000000000, 0.9510565162951535312, 1.000000000000000000, 0.9510565162951535312, 1.000000000000000000, 0.9510565162951535312, 1.000000000000000000, 0.9510565162951535312, 1.000000000000000000, 0.9510565162951535312, 1.000000000000000000, 0.9510565162951535312, 1.000000000000000000, 0.9510565162951535312, 1.000000000000000000, 0.9510565162951535312, 1.000000000000000000, 0.9510565162951535312, 1.000000000000000000, 0.9510565162951535312, 1.000000000000000000, 0.9510565162951535312, 1.000000000000000000, 0.9510565162951535312, 1.000000000000000000, 0.9510565162951535312, 1.000000000000000000, 0.9510565162951535312, 1.000000000000000000, 0.9510565162951535312, 1.000000000000000000, 0.9510565162951535312, 1.000000000000000000, 0.9510565162951535312, 1.000000000000000000, 0.9510565162951535312, 1.000000000000000000, 0.9510565162951535312, 1.000000000000000000, 0.9510565162951535312, 1.000000000000000000, 0.9510565162951535312, 1.000000000000000000, 0.9510565162951535312, 1.000000000000000000, 0.9510565162951535312, 1.000000000000000000, 0.9510565162951535312, 1.000000000000000000, 0.9510565162951535312, 1.000000000000000000, 0.9510565162951535312, 1.000000000000000000, 0.9510565162951535312, 1.000000000000000000, 0.9510565162951535312, 1.000000000000000000, 0.9510565162951535312, 1.000000000000000000, 0.9510565162951535312, 1.000000000000000000, 0.9510565162951535312, 1.000000000000000000, 0.9510565162951535312, 1.000000000000000000, 0.9510565162951535312, 1.000000000000000000, 0.9510565162951535312, 1.000000000000000000, 0.9510565162951535312, 1.000000000000000000, 0.9510565162951535312, 1.000000000000000000, 0.9510565162951535312, 1.000000000000000000, 0.9510565162951535312, 1.000000000000000000, 0.9510565162951535312, 1.000000000000000000, 0.9510565162951535312, 1.000000000000000000, 0.9510565162951535312, 1.000000000000000000, 0.9510565162951535312, 1.000000000000000000, 0.9510565162951535312, 1.000000000000000000, 0.9510565162951535312, 1.000000000000000000, 0.9510565162951535312, 1.000000000000000000, 0.9510565162951535312, 1.000000000000000000, 0.9510565162951535312, 1.000000000000000000, 0.9510565162951535312, 1.000000000000000000, 0.9510565162951535312, 1.000000000000000000, 0.9510565162951535312, 1.000000000000000000, 0.9510565162951535312, 1.000000000000000000, 0.9510565162951535312, 1.000000000000000000, 0.9510565162951535312, 1.000000000000000000, 0.9510565162951535312, 1.000000000000000000, 0.9510565162951535312, 1.000000000000000000, 0.9510565162951535312, 1.000000000000000000, 0.9510565162951535312, 1.000000000000000000, 0.9510565162951535312, 1.000000000000000000, 0.9510565162951535312, 1.000000000000000000, 0.9510565162951535312, 1.000000000000000000, 0.9510565162951535312, 1.000000000000000000, 0.9510565162951535312, 1.000000000000000000, 0.9510565162951535312, 1.000000000000000000, 0.9510565162951535312, 1.000000000000000000, 0.9510565162951535312, 1.000000000000000000, 0.9510565162951535312, 1.000000000000000000, 0.9510565162951535312, 1.000000000000000000, 0.9510565162951535312, 1.000000000000000000, 0.9510565162951535312, 1.000000000000000000, 0.9510565162951535312, 1.000000000000000000, 0.9510565162951535312, 1.000000000000000000, 0.9510565162951535312, 1.000000000000000000, 0.9510565162951535312, 1.000000000000000000, 0.9510565162951535312, 1.000000000000000000, 0.9510565162951535312, 1.000000000000000000, 0.9510565162951535312, 1.000000000000000000, 0.9510565162951535312, 1.000000000000000000, 0.9510565162951535312, 1.000000000000000000, 0.9510565162951535312, 1.000000000000000000, 0.9510565162951535312, 1.000000000000000000, 0.9510565162951535312, 1.000000000000000000, 0.9510565162951535312, 1.000000000000000000, 0.9510565162951535312, 1.000000000000000000, 0.9510565162951535312, 1.000000000000000000, 0.9510565162951535312, 1.000000000000000000, 0.9510565162951535312, 1.000000000000000000, 0.9510565162951535312, 1.000000000000000000, 0.9510565162951535312, 1.000000000000000000, 0.9510565162951535312, 1.000000000000000000, 0.9510565162951535312, 1.000000000000000000, 0.9510565162951535312, 1.000000000000000000, 0.9510565162951535312, 1.000000000000000000, 0.9510565162951535312, 1.000000000000000000, 0.9510565162951535312, 1.000000000000000000, 0.9510565162951535312, 1.000000000000000000, 0.9510565162951535312, 1.000000000000000000, 0.9510565162951535312, 1.000000000000000000, 0.9510565162951535312, 1.000000000000000000, 0.9510565162951535312, 1.000000000000000000, 0.9510565162951535312, 1.000000000000000000, 0.9510565162951535312, 1.000000000000000000, 0.9510565162951535312, 1.000000000000000000, 0.9510565162951535312, 1.000000000000000000, 0.9510565162951535312, 1.000000000000000000, 0.9510565162951535312, 1.000000000000000000, 0.9510565162951535312, 1.000000000000000000, 0.9510565162951535312, 1.000000000000000000, 0.9510565162951535312, 1.000000000000000000, 0.9510565162951535312, 1.000000000000000000, 0.9510565162951535312, 1.000000000000000000, 0.9510565162951535312, 1.000000000000000000, 0.9510565162951535312, 1.000000000000000000, 0.9510565162951535312, 1.000000000000000000, 0.9510565162951535312, 1.000000000000000000, 0.9510565162951535312, 1.000000000000000000, 0.9510565162951535312, 1.000000000000000000, 0.9510565162951535312, 1.000000000000000000, 0.9510565162951535312, 1.000000000000000000, 0.9510565162951535312, 1.000000000000000000, 0.9510565162951535312, 1.000000000000000000, 0.9510565162951535312, 1.000000000000000000, 0.9510565162951535312, 1.000000000000000000, 0.9510565162951535312, 1.000000000000000000, 0.9510565162951535312, 1.000000000000000000, 0.9510565162951535312, 1.000000000000000000, 0.9510565162951535312, 1.000000000000000000),
 ( 1.000000000000000000, 0.9510565162951535312, 1.000000000000000000, 0.9510565162951535312, 1.000000000000000000, 0.9510565162951535312, 1.000000000000000000, 0.9510565162951535312, 1.000000000000000000, 0.9510565162951535312, 1.000000000000000000, 0.9510565162951535312, 1.000000000000000000, 0.9510565162951535312, 1.000000000000000000, 0.9510565162951535312, 1.000000000000000000, 0.9510565162951535312, 1.000000000000000000, 0.9510565162951535312, 1.000000000000000000, 0.9510565162951535312, 1.000000000000000000, 0.9510565162951535312, 1.000000000000000000, 0.9510565162951535312, 1.000000000000000000, 0.9510565162951535312, 1.000000000000000000, 0.9510565162951535312, 1.000000000000000000, 0.9510565162951535312, 1.000000000000000000, 0.9510565162951535312, 1.000000000000000000, 0.9510565162951535312, 1.000000000000000000, 0.9510565162951535312, 1.000000000000000000, 0.9510565162951535312, 1.000000000000000000, 0.9510565162951535312, 1.000000000000000000, 0.9510565162951535312, 1.000000000000000000, 0.9510565162951535312, 1.000000000000000000, 0.9510565162951535312, 1.000000000000000000, 0.9510565162951535312, 1.000000000000000000, 0.9510565162951535312, 1.000000000000000000, 0.9510565162951535312, 1.000000000000000000, 0.9510565162951535312, 1.000000000000000000, 0.9510565162951535312, 1.000000000000000000, 0.9510565162951535312, 1.000000000000000000, 0.9510565162951535312, 1.000000000000000000, 0.9510565162951535312, 1.000000000000000000, 0.9510565162951535312, 1.000000000000000000, 0.9510565162951535312, 1.000000000000000000, 0.9510565162951535312, 1.000000000000000000, 0.9510565162951535312, 1.000000000000000000, 0.9510565162951535312, 1.000000000000000000, 0.9510565162951535312, 1.000000000000000000, 0.9510565162951535312, 1.000000000000000000, 0.9510565162951535312, 1.000000000000000000, 0.9510565162951535312, 1.000000000000000000, 0.9510565162951535312, 1.000000000000000000, 0.9510565162951535312, 1.000000000000000000, 0.9510565162951535312, 1.000000000000000000, 0.9510565162951535312, 1.000000000000000000, 0.9510565162951535312, 1.000000000000000000, 0.9510565162951535312, 1.000000000000000000, 0.9510565162951535312, 1.000000000000000000, 0.9510565162951535312, 1.000000000000000000, 0.9510565162951535312, 1.000000000000000000, 0.9510565162951535312, 1.000000000000000000, 0.9510565162951535312, 1.000000000000000000, 0.9510565162951535312, 1.000000000000000000, 0.9510565162951535312, 1.000000000000000000, 0.9510565162951535312, 1.000000000000000000, 0.9510565162951535312, 1.000000000000000000, 0.9510565162951535312, 1.000000000000000000, 0.9510565162951535312, 1.000000000000000000, 0.9510565162951535312, 1.000000000000000000, 0.9510565162951535312, 1.000000000000000000, 0.9510565162951535312, 1.000000000000000000, 0.9510565162951535312, 1.000000000000000000, 0.9510565162951535312, 1.000000000000000000, 0.9510565162951535312, 1.000000000000000000, 0.9510565162951535312, 1.000000000000000000, 0.9510565162951535312, 1.000000000000000000, 0.9510565162951535312, 1.000000000000000000, 0.9510565162951535312, 1.000000000000000000, 0.9510565162951535312, 1.000000000000000000, 0.9510565162951535312, 1.000000000000000000, 0.9510565162951535312, 1.000000000000000000, 0.9510565162951535312, 1.000000000000000000, 0.9510565162951535312, 1.000000000000000000, 0.9510565162951535312, 1.000000000000000000, 0.9510565162951535312, 1.000000000000000000, 0.9510565162951535312, 1.000000000000000000, 0.9510565162951535312, 1.000000000000000000, 0.9510565162951535312, 1.000000000000000000, 0.9510565162951535312, 1.000000000000000000, 0.9510565162951535312, 1.000000000000000000, 0.9510565162951535312, 1.000000000000000000, 0.9510565162951535312, 1.000000000000000000, 0.9510565162951535312, 1.000000000000000000, 0.9510565162951535312, 1.000000000000000000, 0.9510565162951535312, 1.000000000000000000, 0.9510565162951535312, 1.000000000000000000, 0.9510565162951535312, 1.000000000000000000, 0.9510565162951535312, 1.000000000000000000, 0.9510565162951535312, 1.000000000000000000, 0.9510565162951535312, 1.000000000000000000, 0.9510565162951535312, 1.000000000000000000, 0.9510565162951535312, 1.000000000000000000, 0.9510565162951535312, 1.000000000000000000, 0.9510565162951535312, 1.000000000000000000, 0.9510565162951535312, 1.000000000000000000, 0.9510565162951535312, 1.000000000000000000, 0.9510565162951535312, 1.000000000000000000, 0.9510565162951535312, 1.000000000000000000, 0.9510565162951535312, 1.000000000000000000, 0.9510565162951535312, 1.000000000000000000, 0.9510565162951535312, 1.000000000000000000, 0.9510565162951535312, 1.000000000000000000, 0.9510565162951535312, 1.000000000000000000, 0.9510565162951535312, 1.000000000000000000, 0.9510565162951535312, 1.000000000000000000, 0.9510565162951535312, 1.000000000000000000, 0.9510565162951535312, 1.000000000000000000, 0.9510565162951535312, 1.000000000000000000, 0.9510565162951535312, 1.000000000000000000, 0.9510565162951535312, 1.000000000000000000, 0.9510565162951535312, 1.000000000000000000, 0.9510565162951535312, 1.000000000000000000, 0.9510565162951535312, 1.000000000000000000, 0.9510565162951535312, 1.000000000000000000, 0.9510565162951535312, 1.000000000000000000, 0.9510565162951535312, 1.000000000000000000, 0.9510565162951535312, 1.000000000000000000, 0.9510565162951535312, 1.000000000000000000, 0.9510565162951535312, 1.000000000000000000, 0.9510565162951535312, 1.000000000000000000, 0.9510565162951535312, 1.000000000000000000, 0.9510565162951535312, 1.000000000000000000, 0.9510565162951535312, 1.000000000000000000, 0.9510565162951535312, 1.000000000000000000, 0.9510565162951535312, 1.000000000000000000, 0.9510565162951535312, 1.000000000000000000, 0.9510565162951535312, 1.000000000000000000, 0.9510565162951535312, 1.000000000000000000, 0.9510565162951535312, 1.000000000000000000, 0.9510565162951535312, 1.000000000000000000, 0.9510565162951535312, 1.000000000000000000, 0.9510565162951535312, 1.000000000000000000, 0.9510565162951535312, 1.000000000000000000, 0.9510565162951535312, 1.000000000000000000, 0.9510565162951535312, 1.000000000000000000, 0.9510565162951535312, 1.000000000000000000, 0.9510565162951535312, 1.000000000000000000, 0.9510565162951535312, 1.000000000000000000, 0.9510565162951535312, 1.000000000000000000, 0.9510565162951535312, 1.000000000000000000, 0.9510565162951535312, 1.000000000000000000, 0.9510565162951535312, 1.000000000000000000, 0.9510565162951535312, 1.000000000000000000, 0.9510565162951535312, 1.000000000000000000, 0.9510565162951535312, 1.000000000000000000, 0.9510565162951535312, 1.000000000000000000, 0.9510565162951535312, 1.000000000000000000, 0.9510565162951535312, 1.000000000000000000, 0.9510565162951535312, 1.000000000000000000, 0.9510565162951535312, 1.000000000000000000, 0.9510565162951535312, 1.000000000000000000, 0.9510565162951535312, 1.000000000000000000, 0.9510565162951535312, 1.000000000000000000, 0.9510565162951535312, 1.000000000000000000, 0.9510565162951535312, 1.000000000000000000, 0.9510565162951535312, 1.000000000000000000, 0.9510565162951535312, 1.000000000000000000, 0.9510565162951535312, 1.000000000000000000, 0.9510565162951535312, 1.000000000000000000, 0.9510565162951535312, 1.000000000000000000, 0.9510565162951535312, 1.000000000000000000, 0.9510565162951535312, 1.000000000000000000, 0.9510565162951535312, 1.000000000000000000, 0.9510565162951535312, 1.000000000000000000, 0.9510565162951535312, 1.000000000000000000, 0.9510565162951535312, 1.000000000000000000, 0.9510565162951535312, 1.000000000000000000, 0.9510565162951535312, 1.000000000000000000, 0.9510565162951535312, 1.000000000000000000, 0.9510565162951535312, 1.000000000000000000, 0.9510565162951535312, 1.000000000000000000, 0.9510565162951535312, 1.000000000000000000, 0.9510565162951535312, 1.000000000000000000, 0.9510565162951535312, 1.000000000000000000, 0.9510565162951535312, 1.000000000000000000, 0.9510565162951535312, 1.000000000000000000, 0.9510565162951535312, 1.000000000000000000, 0.9510565162951535312, 1.000000000000000000, 0.9510565162951535312, 1.000000000000000000, 0.9510565162951535312, 1.000000000000000000, 0.9510565162951535312, 1.000000000000000000, 0.9510565162951535312, 1.000000000000000000, 0.9510565162951535312, 1.000000000000000000, 0.9510565162951535312, 1.000000000000000000, 0.9510565162951535312, 1.000000000000000000, 0.9510565162951535312, 1.000000000000000000, 0.9510565162951535312, 1.000000000000000000, 0.9510565162951535312, 1.000000000000000000, 0.9510565162951535312, 1.000000000000000000, 0.9510565162951535312, 1.000000000000000000, 0.9510565162951535312, 1.000000000000000000, 0.9510565162951535312, 1.000000000000000000, 0.9510565162951535312, 1.000000000000000000, 0.9510565162951535312, 1.000000000000000000, 0.9510565162951535312, 1.000000000000000000, 0.9510565162951535312, 1.000000000000000000, 0.9510565162951535312, 1.000000000000000000, 0.9510565162951535312, 1.000000000000000000, 0.9510565162951535312, 1.000000000000000000, 0.9510565162951535312, 1.000000000000000000) ) ) 
 REPRESENTATION_ITEM ( '' )  SURFACE ( )  );
#70294=CARTESIAN_POINT ( 'NONE',  ( 72.95830788359974406, 56.77128196665827176, -15.96545419981962333 ) ) ;
#70299=CARTESIAN_POINT ( 'NONE',  ( 88.49101168009576668, 43.86507591752568658, 0.01250564173601438969 ) ) ;
#70300=CARTESIAN_POINT ( 'NONE',  ( 5.272250483539713706, 24.81751292744053217, -6.180339887498951690 ) ) ;
#70305=CARTESIAN_POINT ( 'NONE',  ( 32.94607225727562394, 21.94754757982091320, 5.678558825948272215 ) ) ;
#70307=CARTESIAN_POINT ( 'NONE',  ( 81.09489198153239897, 47.45865598376690997, -12.84490686960000794 ) ) ;
#70308=CARTESIAN_POINT ( 'NONE',  ( 13.11890841201833169, 13.28920272979925166, -7.433330006724141015 ) ) ;
#70310=CARTESIAN_POINT ( 'NONE',  ( 76.83059214691050443, 63.69233987691562504, 15.32693845983791547 ) ) ;
#70313=CARTESIAN_POINT ( 'NONE',  ( 69.49445684968409864, 63.05235503358468208, -13.61616618888627883 ) ) ;
#70315=CARTESIAN_POINT ( 'NONE',  ( 79.03501320358060411, 55.48393193879000762, -16.09017401043118056 ) ) ;
#70316=CARTESIAN_POINT ( 'NONE',  ( 87.62838477539726512, 44.93552847577709031, -6.577990587745525808 ) ) ;
#70321=CARTESIAN_POINT ( 'NONE',  ( 77.41302249286091808, 49.21411113510112045, 15.30941459159846119 ) ) ;
#70329=ADVANCED_FACE ( 'NONE', ( #25342 ), #25657, .T. ) ;
#70337=CARTESIAN_POINT ( 'NONE',  ( 33.71705561599726053, 20.26216523072496045, -2.296566073217252530E-15 ) ) ;
#70339=CARTESIAN_POINT ( 'NONE',  ( 74.96814850772595662, 66.86370092720997604, -13.20453066047569024 ) ) ;
#70341=EDGE_CURVE ( 'NONE', #20756, #59093, #10159, .T. ) ;
#70345=ORIENTED_EDGE ( 'NONE', *, *, #23704, .F. ) ;
#70347=CARTESIAN_POINT ( 'NONE',  ( 67.97326575654918202, 65.43911154409434516, 10.39403152487275506 ) ) ;
#70348=CARTESIAN_POINT ( 'NONE',  ( 67.93422661307175758, 66.05804427658543432, -10.47009145265134933 ) ) ;
#70366=CARTESIAN_POINT ( 'NONE',  ( 80.03788392018469722, 44.31502134952003757, -11.48980017305513179 ) ) ;
#70369=CARTESIAN_POINT ( 'NONE',  ( 81.17232691891707930, 55.55242957854174080, 16.36487835605631602 ) ) ;
#70370=CARTESIAN_POINT ( 'NONE',  ( 82.74137886417670984, 47.78502673368306120, -12.47258107324418930 ) ) ;
#70381=CARTESIAN_POINT ( 'NONE',  ( 15.66455532895297331, 30.81751292744056059, -6.180339887498951690 ) ) ;
#70386=CARTESIAN_POINT ( 'NONE',  ( 88.10887562929657690, 44.41668309952778060, 4.665177569529613599 ) ) ;
#70388=CARTESIAN_POINT ( 'NONE',  ( 81.04961468568201610, 43.68546784643918812, -9.492462169003031747 ) ) ;
#70392=CARTESIAN_POINT ( 'NONE',  ( 72.55393231385352237, 70.87694079910581024, 7.622851120052408724 ) ) ;
#70402=ADVANCED_FACE ( 'NONE', ( #86207 ), #15734, .T. ) ;
#70409=CARTESIAN_POINT ( 'NONE',  ( 73.60933432321982650, 55.64367109616565443, 16.10230547196764661 ) ) ;
#70412=CARTESIAN_POINT ( 'NONE',  ( 26.23682664367882111, 38.08080186712594184, -3.090169943749475845 ) ) ;
#70415=DIRECTION ( 'NONE',  ( -0.8660254037844377084, -0.5000000000000014433, -0.000000000000000000 ) ) ;
#70417=ADVANCED_FACE ( 'NONE', ( #69933 ), #6975, .T. ) ;
#70423=CARTESIAN_POINT ( 'NONE',  ( 68.68909986782581711, 64.16576715805911135, -12.55144644517788777 ) ) ;
#70424=PLANE ( 'NONE',  #82061 ) ;
#70428=CARTESIAN_POINT ( 'NONE',  ( 34.54807858326547176, 25.11029122506296929, -8.090169943749478065 ) ) ;
#70429=CARTESIAN_POINT ( 'NONE',  ( 77.17250858205457575, 53.66386925528713192, 16.42442879155417756 ) ) ;
#70431=CARTESIAN_POINT ( 'NONE',  ( 81.46466179813324970, 56.08326244678959682, 16.06754189170436575 ) ) ;
#70436=CARTESIAN_POINT ( 'NONE',  ( 72.84204051986223760, 66.34192636652406350, -12.17031965754431866 ) ) ;
#70441=CARTESIAN_POINT ( 'NONE',  ( 35.14347105191519205, 25.45404122711135741, -8.090169943749478065 ) ) ;
#70445=CARTESIAN_POINT ( 'NONE',  ( 67.08714283343131513, 66.81104840727229544, -8.985171576933360882 ) ) ;
#70449=CARTESIAN_POINT ( 'NONE',  ( 24.91850453858129910, 20.10170272979927475, -7.433330006724141015 ) ) ;
#70454=CARTESIAN_POINT ( 'NONE',  ( 5.233272902960924178, 23.99752408145589655, 5.678558825948276656 ) ) ;
#70456=CARTESIAN_POINT ( 'NONE',  ( 79.35086191672368727, 57.56414197016153622, -16.24676580536099735 ) ) ;
#70457=CARTESIAN_POINT ( 'NONE',  ( 88.08794642153516463, 44.30065689091529890, 2.777777743264004506 ) ) ;
#70459=CARTESIAN_POINT ( 'NONE',  ( 69.45630962237427752, 70.64887205696791739, -1.534870757239616301 ) ) ;
#70465=CARTESIAN_POINT ( 'NONE',  ( 82.42451625089289280, 42.32467009663571389, -6.203346966617362845 ) ) ;
#70466=ORIENTED_EDGE ( 'NONE', *, *, #9616, .F. ) ;
#70468=CARTESIAN_POINT ( 'NONE',  ( 71.78553924664423391, 72.10835861452468976, -3.632824164035485470 ) ) ;
#70480=CARTESIAN_POINT ( 'NONE',  ( 28.99364183777449000, 25.24335787977764767, -9.188101187500008038 ) ) ;
#70481=DIRECTION ( 'NONE',  ( 0.1039558454088763267, -0.1800568059919503139, 0.9781476007338069101 ) ) ;
#70482=CARTESIAN_POINT ( 'NONE',  ( 78.29365456329206552, 47.43229965770008505, -13.76414149961745714 ) ) ;
#70490=CARTESIAN_POINT ( 'NONE',  ( 87.12872031379318116, 46.22333408697501511, 8.447664276980741960 ) ) ;
#70495=DIRECTION ( 'NONE',  ( -0.8660254037844378194, -0.5000000000000013323, -0.000000000000000000 ) ) ;
#70501=CARTESIAN_POINT ( 'NONE',  ( 76.20608723644332372, 65.18883345732480450, 14.14645056589919214 ) ) ;
#70502=CARTESIAN_POINT ( 'NONE',  ( 70.44493300807654634, 65.46586672381103256, -11.71043221882291263 ) ) ;
#70509=CARTESIAN_POINT ( 'NONE',  ( 87.67135465677671391, 44.96834575157770075, -6.594061650049633627 ) ) ;
#70513=CARTESIAN_POINT ( 'NONE',  ( 83.70911819089758410, 52.26791303372475994, -15.08805761434582848 ) ) ;
#70514=CARTESIAN_POINT ( 'NONE',  ( 69.38297557973733376, 65.04212082436336573, -11.54860170590457180 ) ) ;
#70525=CARTESIAN_POINT ( 'NONE',  ( 69.61542750552385428, 62.56132062511080250, -13.94275833699888345 ) ) ;
#70530=CARTESIAN_POINT ( 'NONE',  ( 71.50069359034532113, 71.04066487116593009, -5.105904657311576500 ) ) ;
#70537=ADVANCED_FACE ( 'NONE', ( #73460 ), #75452, .T. ) ;
#70538=ORIENTED_EDGE ( 'NONE', *, *, #29795, .F. ) ;
#70544=CARTESIAN_POINT ( 'NONE',  ( 20.18734655506498754, 13.78380873178786636, -6.180339887498949025 ) ) ;
#70545=CARTESIAN_POINT ( 'NONE',  ( 83.68959111172128473, 48.84214776367139166, -13.33749660644718205 ) ) ;
#70547=CARTESIAN_POINT ( 'NONE',  ( 66.54034002427947314, 67.76616102596386781, -6.984587242053489575 ) ) ;
#70553=CARTESIAN_POINT ( 'NONE',  ( 18.69751666607634988, 11.76426979415088958, 3.090169943749476733 ) ) ;
#70560=CARTESIAN_POINT ( 'NONE',  ( 34.04181514241641082, 20.44966523072496756, -2.296566073217252530E-15 ) ) ;
#70565=CARTESIAN_POINT ( 'NONE',  ( 87.97782240006738164, 43.76496563450900368, 2.369043524150745927 ) ) ;
#70566=CARTESIAN_POINT ( 'NONE',  ( 66.53847098313150354, 68.80888956264922740, 2.264020422531420440 ) ) ;
#70567=ORIENTED_EDGE ( 'NONE', *, *, #97843, .F. ) ;
#70571=CARTESIAN_POINT ( 'NONE',  ( 9.796739006517501736, 23.84336893147754566, -7.433330006724137462 ) ) ;
#70580=CARTESIAN_POINT ( 'NONE',  ( 87.63119364650853527, 45.29408460765225897, 6.394950601605620122 ) ) ;
#70586=CARTESIAN_POINT ( 'NONE',  ( 73.06253000732938574, 70.71164709794337000, 7.625195754903023371 ) ) ;
#70590=ORIENTED_EDGE ( 'NONE', *, *, #44364, .T. ) ;
#70592=CARTESIAN_POINT ( 'NONE',  ( 79.25000469529436486, 59.07415148808540550, -16.22410911865845762 ) ) ;
#70593=B_SPLINE_CURVE_WITH_KNOTS ( 'NONE', 3,
 ( #58809, #12757, #36018, #51743, #21823, #36518, #14231, #52709, #67927, #39372, #43620, #82183, #83162, #20852, #23678, #83668, #29427, #74561, #98851, #52216, #45118, #76053, #90782, #66920 ),
 .UNSPECIFIED., .F., .F.,
 ( 4, 2, 2, 2, 2, 2, 2, 2, 2, 2, 2, 4 ),
 ( 0.000000000000000000, 0.1250000000000000833, 0.2500000000000001665, 0.3750000000000002220, 0.4375000000000002776, 0.5000000000000003331, 0.5625000000000003331, 0.6250000000000004441, 0.6875000000000004441, 0.7500000000000004441, 0.8750000000000005551, 1.000000000000000000 ),
 .UNSPECIFIED. ) ;
#70596=CARTESIAN_POINT ( 'NONE',  ( 78.21454416846142976, 48.89259193441272089, -15.02001292579780234 ) ) ;
#70598=CARTESIAN_POINT ( 'NONE',  ( 80.58471728211203811, 43.44896785130639927, 9.531559131089510473 ) ) ;
#70602=CARTESIAN_POINT ( 'NONE',  ( 74.14312167556930433, 66.30466486950707861, 1.224646799147354045E-15 ) ) ;
#70605=ORIENTED_EDGE ( 'NONE', *, *, #1768, .T. ) ;
#70606=CARTESIAN_POINT ( 'NONE',  ( 73.46883546717839408, 61.70975325623787455, 14.87585405357015844 ) ) ;
#70611=CARTESIAN_POINT ( 'NONE',  ( 83.50408885241421331, 50.19109076061639030, 13.73202446986405612 ) ) ;
#70619=CARTESIAN_POINT ( 'NONE',  ( 19.08967936351193373, 31.99752408145592497, 5.678558825948277544 ) ) ;
#70620=VECTOR ( 'NONE', #7456, 1000.000000000000114 ) ;
#70622=LINE ( 'NONE', #26543, #100063 ) ;
#70624=ORIENTED_EDGE ( 'NONE', *, *, #70870, .T. ) ;
#70629=CYLINDRICAL_SURFACE ( 'NONE', #69935, 10.00000000000001066 ) ;
#70631=CARTESIAN_POINT ( 'NONE',  ( 85.27809249074009301, 45.59539938871965603, -8.958021638074621151 ) ) ;
#70640=CARTESIAN_POINT ( 'NONE',  ( 82.32795736216652926, 40.34849779494332012, -1.094049968420492513 ) ) ;
#70641=CARTESIAN_POINT ( 'NONE',  ( 13.13113612116928763, 15.78052372038639106, -10.00000000000000355 ) ) ;
#70644=CARTESIAN_POINT ( 'NONE',  ( 75.82286285680700644, 65.49053554218845363, 14.29367836297803329 ) ) ;
#70652=CARTESIAN_POINT ( 'NONE',  ( 84.27726345673161745, 46.24452505070916430, -10.39517579047728013 ) ) ;
#70654=CARTESIAN_POINT ( 'NONE',  ( 24.93549151006825326, 33.13478043621389446, 8.090169943749478065 ) ) ;
#70664=PLANE ( 'NONE',  #94355 ) ;
#70666=CARTESIAN_POINT ( 'NONE',  ( 68.65502763568917999, 64.17108234953235524, -12.53269806771906580 ) ) ;
#70670=CARTESIAN_POINT ( 'NONE',  ( 71.60580622982271848, 63.30568055998580945, 14.16434923562446535 ) ) ;
#70673=CARTESIAN_POINT ( 'NONE',  ( 68.31449789920554849, 67.83967261433821250, 7.597146809165362669 ) ) ;
#70679=CARTESIAN_POINT ( 'NONE',  ( 79.36263291408793918, 45.67866562566761957, -12.88899626193393821 ) ) ;
#70681=CARTESIAN_POINT ( 'NONE',  ( 18.31506083472495661, 16.28920272979926054, -7.433330006724141015 ) ) ;
#70687=CARTESIAN_POINT ( 'NONE',  ( 25.44954664093420149, 26.64441083166262203, -10.00000000000000533 ) ) ;
#70692=CARTESIAN_POINT ( 'NONE',  ( 85.99011874742393502, 47.63415234044297364, 10.88239874243195260 ) ) ;
#70700=CARTESIAN_POINT ( 'NONE',  ( 79.24868352219918677, 50.32229833407618713, 14.83203819062691764 ) ) ;
#70703=CARTESIAN_POINT ( 'NONE',  ( 82.28003896795380001, 40.62557011406286733, -3.142018250819523129 ) ) ;
#70707=FACE_OUTER_BOUND ( 'NONE', #96540, .T. ) ;
#70708=CARTESIAN_POINT ( 'NONE',  ( 34.24030602833327208, 37.95586893147758900, 7.433330006724141015 ) ) ;
#70709=CARTESIAN_POINT ( 'NONE',  ( 72.75811361349980189, 70.26368998748593242, -8.075100041229438474 ) ) ;
#70714=ORIENTED_EDGE ( 'NONE', *, *, #5220, .T. ) ;
#70715=CARTESIAN_POINT ( 'NONE',  ( 86.54479369881731543, 47.18726309986306688, -10.63286291588202204 ) ) ;
#70716=DIRECTION ( 'NONE',  ( 0.9563064286990893281, -0.2923662333936556945, 0.000000000000000000 ) ) ;
#70729=CARTESIAN_POINT ( 'NONE',  ( 77.16668814154863298, 49.29486154796829567, -15.38919878964156496 ) ) ;
#70731=CARTESIAN_POINT ( 'NONE',  ( 74.54670819670354831, 56.70307473271788723, 16.07195883519789703 ) ) ;
#70732=CARTESIAN_POINT ( 'NONE',  ( 79.39877852727147456, 54.29655282685389039, 15.92112751935395920 ) ) ;
#70738=CARTESIAN_POINT ( 'NONE',  ( 79.41088169706156918, 46.22695399816395678, 12.63871909588431564 ) ) ;
#70746=CARTESIAN_POINT ( 'NONE',  ( 43.77620770598743150, 30.98920272979930601, 7.433330006724137462 ) ) ;
#70748=CARTESIAN_POINT ( 'NONE',  ( 85.74825148587619594, 48.61567592689142003, -12.33318615817161934 ) ) ;
#70754=CARTESIAN_POINT ( 'NONE',  ( 71.92913702268965892, 61.41965493978950263, 14.61815708677550418 ) ) ;
#70756=CARTESIAN_POINT ( 'NONE',  ( 78.72526120150082818, 53.56602875328650981, 16.28398236204086302 ) ) ;
#70762=CARTESIAN_POINT ( 'NONE',  ( 66.01919585322798412, 68.69228577893747456, -0.4091825812074046942 ) ) ;
#70774=VECTOR ( 'NONE', #33842, 1000.000000000000114 ) ;
#70777=CARTESIAN_POINT ( 'NONE',  ( 66.17343954913512505, 68.52301864461630032, -2.711686016849372827 ) ) ;
#70780=EDGE_CURVE ( 'NONE', #826, #50951, #5542, .T. ) ;
#70783=CARTESIAN_POINT ( 'NONE',  ( 85.68485941944550177, 48.66523437743575187, 11.91861461389294163 ) ) ;
#70784=CARTESIAN_POINT ( 'NONE',  ( 74.40608543823466903, 68.34271654374390437, 11.85151599582641424 ) ) ;
#70788=CARTESIAN_POINT ( 'NONE',  ( 68.56904214663958896, 70.19644423968159686, 0.8067628227658676376 ) ) ;
#70797=CARTESIAN_POINT ( 'NONE',  ( 78.07803331781863676, 55.04206026085086023, 16.09808790484326835 ) ) ;
#70798=CARTESIAN_POINT ( 'NONE',  ( 84.72317995036203797, 49.82855470703300682, -13.16391237593562025 ) ) ;
#70799=VECTOR ( 'NONE', #84856, 1000.000000000000114 ) ;
#70800=CARTESIAN_POINT ( 'NONE',  ( 77.95473461231914314, 62.00593549909827118, 15.66743434672346424 ) ) ;
#70801=CARTESIAN_POINT ( 'NONE',  ( 66.95957972044308804, 66.97324061659901417, 8.659915215018605394 ) ) ;
#70802=CARTESIAN_POINT ( 'NONE',  ( 76.04288044954796533, 51.24135356845017242, 16.11949329745968384 ) ) ;
#70810=CARTESIAN_POINT ( 'NONE',  ( 73.03680373040982943, 57.44200512075386911, -15.87150009157571873 ) ) ;
#70815=CARTESIAN_POINT ( 'NONE',  ( 88.54549197286583251, 43.89854493182281203, -0.2370037879772141087 ) ) ;
#70816=CARTESIAN_POINT ( 'NONE',  ( 84.44366846031314822, 49.29134167535947597, -12.87259635285258952 ) ) ;
#70817=DIRECTION ( 'NONE',  ( -0.8660254037844378194, -0.5000000000000014433, -0.000000000000000000 ) ) ;
#70818=CARTESIAN_POINT ( 'NONE',  ( 72.17108608572740991, 71.17802923003300464, -6.704596218806396557 ) ) ;
#70820=CARTESIAN_POINT ( 'NONE',  ( 22.15746398174156440, 34.83396525600390703, -2.839279412974133887 ) ) ;
#70821=CYLINDRICAL_SURFACE ( 'NONE', #98427, 16.60714546451156792 ) ;
#70822=CARTESIAN_POINT ( 'NONE',  ( 79.94121550646556784, 47.70160699126887494, -13.39487937175259091 ) ) ;
#70823=CARTESIAN_POINT ( 'NONE',  ( 13.03712377304622194, 16.03085787977761356, 9.188101187500006262 ) ) ;
#70825=FACE_OUTER_BOUND ( 'NONE', #49310, .T. ) ;
#70828=CARTESIAN_POINT ( 'NONE',  ( 73.83071771892932134, 66.06232275870847559, 12.79940641639033672 ) ) ;
#70830=CARTESIAN_POINT ( 'NONE',  ( 76.63808522071934703, 56.32536596566799858, -16.16213633644409242 ) ) ;
#70835=CARTESIAN_POINT ( 'NONE',  ( 77.49963593495350267, 49.62430142007526257, 14.92239454847386959 ) ) ;
#70837=CARTESIAN_POINT ( 'NONE',  ( 82.30387339498274457, 53.64944443644737504, 15.82386716188995734 ) ) ;
#70841=CARTESIAN_POINT ( 'NONE',  ( 72.54644133328486078, 68.79346617608341319, -9.755494697606795995 ) ) ;
#70852=CARTESIAN_POINT ( 'NONE',  ( 27.26159103020561147, 24.24335787977764767, -9.188101187500008038 ) ) ;
#70854=CARTESIAN_POINT ( 'NONE',  ( 75.09735448162263083, 66.37212636226136908, -13.14697353001001545 ) ) ;
#70855=CARTESIAN_POINT ( 'NONE',  ( 79.90451369755943745, 49.15256129334691337, -14.17871552535267909 ) ) ;
#70858=DIRECTION ( 'NONE',  ( -0.8660254037844377084, -0.5000000000000014433, -0.000000000000000000 ) ) ;
#70860=ORIENTED_EDGE ( 'NONE', *, *, #44476, .F. ) ;
#70864=CARTESIAN_POINT ( 'NONE',  ( 68.09452353918298684, 66.09134662472550303, -10.53294727184536406 ) ) ;
#70865=CARTESIAN_POINT ( 'NONE',  ( 81.77434258213597218, 55.39018043030689853, -15.93420164564364150 ) ) ;
#70870=EDGE_CURVE ( 'NONE', #18263, #18179, #18967, .T. ) ;
#70873=CARTESIAN_POINT ( 'NONE',  ( 79.09523395582193928, 59.82262253747457237, 16.49691284064748231 ) ) ;
#70876=CARTESIAN_POINT ( 'NONE',  ( 34.73896580337741113, 43.55466486950702887, 7.012934429366973338E-14 ) ) ;
#70877=CARTESIAN_POINT ( 'NONE',  ( 78.08878743907096975, 62.01730706715306951, -16.03713534414099939 ) ) ;
#70878=VERTEX_POINT ( 'NONE', #16630 ) ;
#70883=CARTESIAN_POINT ( 'NONE',  ( 80.29316516335838116, 44.72160512723912973, -11.71951212942682119 ) ) ;
#70884=PLANE ( 'NONE',  #81819 ) ;
#70885=EDGE_CURVE ( 'NONE', #93322, #62754, #2091, .T. ) ;
#70887=CARTESIAN_POINT ( 'NONE',  ( 67.76563652183371289, 65.64620069392987034, 10.05537879187873074 ) ) ;
#70897=CARTESIAN_POINT ( 'NONE',  ( 75.93601443309867705, 65.18730796954976370, -14.47772449952195117 ) ) ;
#70900=CARTESIAN_POINT ( 'NONE',  ( 87.75230366022445594, 44.21248639555269477, 4.670146826978180954 ) ) ;
#70902=CARTESIAN_POINT ( 'NONE',  ( 83.07363809413841693, 43.66347682277865516, -7.925384865395641576 ) ) ;
#70915=CARTESIAN_POINT ( 'NONE',  ( 83.94554275650895647, 42.35676708697683068, 4.096087114950127450 ) ) ;
#70917=CARTESIAN_POINT ( 'NONE',  ( 83.82333528792250377, 52.03156133651413739, 14.57194887151437968 ) ) ;
#70919=ORIENTED_EDGE ( 'NONE', *, *, #45650, .T. ) ;
#70928=CARTESIAN_POINT ( 'NONE',  ( 73.74393169614602073, 55.22324961333944060, 16.59624740907808871 ) ) ;
#70929=CARTESIAN_POINT ( 'NONE',  ( 70.01283242295176024, 62.80173547756309915, -13.36538303052352283 ) ) ;
#70930=CARTESIAN_POINT ( 'NONE',  ( 34.29273532275193759, 21.92755873383628185, 6.180339887498953466 ) ) ;
#70940=B_SPLINE_CURVE_WITH_KNOTS ( 'NONE', 3,
 ( #79398, #24151, #86017, #88017, #49446, #47931, #72273, #80399, #78368, #39817, #70748, #9964, #63145, #40826, #86510, #71772, #33248, #41842, #73262, #80909, #34251, #20064, #73756, #4348, #58049, #11481, #3856, #35244, #19579, #66151, #57536 ),
 .UNSPECIFIED., .F., .F.,
 ( 4, 3, 3, 3, 3, 3, 3, 3, 3, 3, 4 ),
 ( 0.000000000000000000, 0.1333490885032397044, 0.3007194338854659588, 0.4699862290245639951, 0.5844252810809660303, 0.6686540514503046539, 0.7354980260655714641, 0.8028463152565815664, 0.8633854507757389163, 0.9437142632667553377, 1.000000000000000000 ),
 .UNSPECIFIED. ) ;
#70943=CARTESIAN_POINT ( 'NONE',  ( 81.87359138905077316, 41.32955797133629972, 5.976920566261187950 ) ) ;
#70946=CARTESIAN_POINT ( 'NONE',  ( 34.45917901495312208, 20.86426979415091765, -3.090169943749474069 ) ) ;
#70947=B_SPLINE_CURVE_WITH_KNOTS ( 'NONE', 3,
 ( #11246, #33526, #63421, #72035, #1128, #56813, #49714, #64928, #94854, #87302 ),
 .UNSPECIFIED., .F., .F.,
 ( 4, 2, 2, 2, 4 ),
 ( 0.000000000000000000, 0.2500000000000000000, 0.5000000000000000000, 0.7500000000000000000, 1.000000000000000000 ),
 .UNSPECIFIED. ) ;
#70951=CARTESIAN_POINT ( 'NONE',  ( 81.64195525244801388, 42.01227061513564109, 7.558743156282623055 ) ) ;
#70956=CARTESIAN_POINT ( 'NONE',  ( 68.63741997012778029, 66.83210094663463963, -9.273233233882304916 ) ) ;
#70963=EDGE_CURVE ( 'NONE', #45691, #35211, #29885, .T. ) ;
#70964=DIRECTION ( 'NONE',  ( -0.8660254037844377084, -0.5000000000000014433, -0.000000000000000000 ) ) ;
#70972=CARTESIAN_POINT ( 'NONE',  ( 28.14623683147711830, 18.11110640527293114, -2.839279412974138328 ) ) ;
#70979=CARTESIAN_POINT ( 'NONE',  ( 9.553764119070450533, 20.91421378149917132, 9.188101187500008038 ) ) ;
#70980=CARTESIAN_POINT ( 'NONE',  ( 78.13494257139964816, 58.08983479524191296, -16.20152750994855495 ) ) ;
#70981=CARTESIAN_POINT ( 'NONE',  ( 71.85962433970722429, 72.56121191805073067, -1.249447308665279088 ) ) ;
#70984=CARTESIAN_POINT ( 'NONE',  ( 71.98137461515177904, 71.49844079294172161, -5.753101040561137580 ) ) ;
#70990=CARTESIAN_POINT ( 'NONE',  ( 81.35748880148537410, 42.22347387491733173, -7.155507324468848296 ) ) ;
#70995=CARTESIAN_POINT ( 'NONE',  ( 79.95899844298520520, 58.10650356627559887, 16.26824798947572148 ) ) ;
#71006=CARTESIAN_POINT ( 'NONE',  ( 21.83270445532239989, 34.64646525600390703, -2.839279412974133887 ) ) ;
#71008=CARTESIAN_POINT ( 'NONE',  ( 78.54120617833643792, 48.00853119821599790, -13.98189004695917959 ) ) ;
#71011=CARTESIAN_POINT ( 'NONE',  ( 74.01669459151050035, 68.61891074470059948, 10.90943161386742055 ) ) ;
#71012=CARTESIAN_POINT ( 'NONE',  ( 35.16829885187633664, 20.70852965304481685, 1.583844403245364907 ) ) ;
#71019=CARTESIAN_POINT ( 'NONE',  ( 86.05859607216220297, 43.31872955745066633, -3.244090947481843568 ) ) ;
#71030=CARTESIAN_POINT ( 'NONE',  ( 67.34387953621143197, 66.59329343503119958, 8.595237674194807553 ) ) ;
#71031=CARTESIAN_POINT ( 'NONE',  ( 72.42134570124093784, 65.10669864484587777, -12.85055710188708566 ) ) ;
#71036=CARTESIAN_POINT ( 'NONE',  ( 84.09826433023697234, 41.84909642707336985, -0.5111001068266544101 ) ) ;
#71043=ADVANCED_FACE ( 'NONE', ( #52391 ), #82848, .T. ) ;
#71053=CARTESIAN_POINT ( 'NONE',  ( 85.60276959248551520, 48.33120518904961926, -11.70778487545583602 ) ) ;
#71054=CARTESIAN_POINT ( 'NONE',  ( 88.07430803657909735, 44.66886354398342007, -4.226991484831405188 ) ) ;
#71056=CARTESIAN_POINT ( 'NONE',  ( 80.36752454425955250, 44.74486481172305474, -11.70255150684123002 ) ) ;
#71063=FACE_OUTER_BOUND ( 'NONE', #43455, .T. ) ;
#71067=CARTESIAN_POINT ( 'NONE',  ( 12.21574338843640284, 25.79103043416548147, 8.090169943749478065 ) ) ;
#71070=CARTESIAN_POINT ( 'NONE',  ( 18.45529574749610902, 12.78380873178786281, -6.180339887498949025 ) ) ;
#71076=CARTESIAN_POINT ( 'NONE',  ( 6.591042624459347188, 19.50829794293877839, -10.00000000000000355 ) ) ;
#71079=CARTESIAN_POINT ( 'NONE',  ( 66.45302924825351454, 68.82209965975525279, -4.357771214034995566 ) ) ;
#71088=CARTESIAN_POINT ( 'NONE',  ( 40.31210609084968866, 28.98920272979929535, 7.433330006724137462 ) ) ;
#71089=CARTESIAN_POINT ( 'NONE',  ( 80.32771389996757705, 57.94408260071153194, -16.24746918486169633 ) ) ;
#71095=CARTESIAN_POINT ( 'NONE',  ( 65.83313805523765438, 68.98304839603784444, 2.094471952982813523 ) ) ;
#71101=CARTESIAN_POINT ( 'NONE',  ( 8.584303441219292452, 23.14336893147753571, 7.433330006724141015 ) ) ;
#71108=CARTESIAN_POINT ( 'NONE',  ( 87.66825142739060084, 45.41049311418420587, 6.595692451674659118 ) ) ;
#71118=CARTESIAN_POINT ( 'NONE',  ( 79.38384574407295702, 59.10269726290196246, -16.22807843983317255 ) ) ;
#71125=CARTESIAN_POINT ( 'NONE',  ( 66.59506449235166770, 69.13094975345107684, 3.575540226172965408 ) ) ;
#71132=CARTESIAN_POINT ( 'NONE',  ( 73.81332162787411733, 63.24887547442293112, 14.34933433100697009 ) ) ;
#71136=ORIENTED_EDGE ( 'NONE', *, *, #3307, .F. ) ;
#71137=CARTESIAN_POINT ( 'NONE',  ( 81.52669532789981588, 44.57943870447123658, 10.20249863168784721 ) ) ;
#71140=CARTESIAN_POINT ( 'NONE',  ( 71.47986246715085201, 69.49463484872732977, 7.994332015353252885 ) ) ;
#71144=CARTESIAN_POINT ( 'NONE',  ( 82.65877604426773928, 53.27536003831319533, -15.29495776700401954 ) ) ;
#71146=ORIENTED_EDGE ( 'NONE', *, *, #47881, .T. ) ;
#71148=CARTESIAN_POINT ( 'NONE',  ( 20.33338779993010803, 20.24335787977762990, -9.188101187500008038 ) ) ;
#71164=B_SPLINE_CURVE_WITH_KNOTS ( 'NONE', 3,
 ( #24215, #85567, #16112, #84556, #914, #8026, #1425, #94151, #9010, #31302 ),
 .UNSPECIFIED., .F., .F.,
 ( 4, 2, 2, 2, 4 ),
 ( 0.000000000000000000, 0.0002622400424273183960, 0.0005244800848546367919, 0.0007867201272819552421, 0.001048960169709273584 ),
 .UNSPECIFIED. ) ;
#71169=CARTESIAN_POINT ( 'NONE',  ( 72.44129552685039641, 70.67501955208014408, -7.848061272651214004 ) ) ;
#71177=VERTEX_POINT ( 'NONE', #39658 ) ;
#71180=CARTESIAN_POINT ( 'NONE',  ( 69.06100142215747439, 70.44252798373366886, 1.237476299740512431 ) ) ;
#71181=CARTESIAN_POINT ( 'NONE',  ( 83.26693017028203769, 42.57865931657983083, 5.729871548751052757 ) ) ;
#71184=CARTESIAN_POINT ( 'NONE',  ( 74.09769653082098273, 68.87686179987508694, -11.21282387169916284 ) ) ;
#71194=CARTESIAN_POINT ( 'NONE',  ( 68.56886429688491091, 64.21317091390413623, -12.46312428434479358 ) ) ;
#71206=CARTESIAN_POINT ( 'NONE',  ( 14.92192532440567199, 20.56628583063839955, 9.188101187500006262 ) ) ;
#71207=CARTESIAN_POINT ( 'NONE',  ( 71.21816854543845920, 61.31929265152032826, -14.99493774206449359 ) ) ;
#71209=CARTESIAN_POINT ( 'NONE',  ( 71.98264401366868981, 72.39816763649429276, -2.869464145551836598 ) ) ;
#71213=CARTESIAN_POINT ( 'NONE',  ( 21.04067422097218909, 35.08080186712593473, -3.090169943749475845 ) ) ;
#71215=CARTESIAN_POINT ( 'NONE',  ( 82.00597693497557827, 40.98120758155860699, -2.954347521771857554 ) ) ;
#71223=CARTESIAN_POINT ( 'NONE',  ( 78.87602572105338083, 48.98972573457342605, 14.36228915801518369 ) ) ;
#71224=CARTESIAN_POINT ( 'NONE',  ( 83.87863349871378205, 51.97949305273395737, -14.54186584096833279 ) ) ;
#71227=CARTESIAN_POINT ( 'NONE',  ( 74.91412036032340893, 53.21648545400848462, -16.51781489608933384 ) ) ;
#71232=CARTESIAN_POINT ( 'NONE',  ( 35.45274159363147959, 38.65586893147759184, -7.433330006724137462 ) ) ;
#71234=ORIENTED_EDGE ( 'NONE', *, *, #77063, .T. ) ;
#71239=CARTESIAN_POINT ( 'NONE',  ( 79.39869110645544481, 59.73379174629956623, 16.16845418028724524 ) ) ;
#71242=CARTESIAN_POINT ( 'NONE',  ( 24.56267145112387240, 22.38052372038641735, 10.00000000000000533 ) ) ;
#71244=ORIENTED_EDGE ( 'NONE', *, *, #24790, .F. ) ;
#71245=B_SPLINE_CURVE_WITH_KNOTS ( 'NONE', 3,
 ( #46653, #30955, #68952, #77580, #69948, #67968, #98889, #29468, #60343, #37548, #31448, #68454, #62340, #13767, #99383, #93806, #70457, #47150, #8660, #1068, #64361, #9166, #94797, #87738 ),
 .UNSPECIFIED., .F., .F.,
 ( 4, 2, 2, 2, 2, 2, 2, 2, 2, 2, 2, 4 ),
 ( 0.000000000000000000, 0.1250000000000041633, 0.2500000000000083267, 0.3750000000000124900, 0.4375000000000112133, 0.5000000000000099920, 0.5625000000000087708, 0.6250000000000074385, 0.6875000000000062172, 0.7500000000000049960, 0.8750000000000024425, 1.000000000000000000 ),
 .UNSPECIFIED. ) ;
#71246=ORIENTED_EDGE ( 'NONE', *, *, #66944, .T. ) ;
#71249=CARTESIAN_POINT ( 'NONE',  ( 77.20279821355711647, 49.64797377247255383, -14.99054536557791906 ) ) ;
#71258=CARTESIAN_POINT ( 'NONE',  ( 82.78178186318515941, 40.60033419795881571, 0.9506087024331607571 ) ) ;
#71266=CARTESIAN_POINT ( 'NONE',  ( 46.16617079539854984, 27.44966523072498177, -2.296566073217252530E-15 ) ) ;
#71267=VERTEX_POINT ( 'NONE', #25 ) ;
#71268=CARTESIAN_POINT ( 'NONE',  ( 86.32427409670840746, 43.64500876675992203, -5.374088149502346923 ) ) ;
#71275=CARTESIAN_POINT ( 'NONE',  ( 72.06635965893990203, 61.93972394716566043, 14.43705991168542546 ) ) ;
#71280=ORIENTED_EDGE ( 'NONE', *, *, #54719, .T. ) ;
#71284=DIRECTION ( 'NONE',  ( -0.2938926261462390666, 0.5090369604551334692, 0.8090169943749425663 ) ) ;
#71302=CARTESIAN_POINT ( 'NONE',  ( 74.28280957949721142, 68.55643958410426819, 11.10420501780135893 ) ) ;
#71311=CARTESIAN_POINT ( 'NONE',  ( 77.59148524364135824, 52.59450808426719703, 15.75520512475421953 ) ) ;
#71323=CARTESIAN_POINT ( 'NONE',  ( 76.86303881961467255, 63.31387137873053916, -15.46595148530503927 ) ) ;
#71327=CARTESIAN_POINT ( 'NONE',  ( 88.30697365647166919, 43.76017805630483792, 0.1929712240254208011 ) ) ;
#71328=CARTESIAN_POINT ( 'NONE',  ( 13.83268420227240014, 8.390406791769812855, -2.889640176918245968E-15 ) ) ;
#71329=CARTESIAN_POINT ( 'NONE',  ( 85.48636484970303684, 43.17023849599863183, -5.434256565237638448 ) ) ;
#71331=CARTESIAN_POINT ( 'NONE',  ( 31.65185205300530313, 23.98920272979928114, 7.433330006724137462 ) ) ;
#71335=CARTESIAN_POINT ( 'NONE',  ( 12.13982549814181411, 27.98502408145591502, -5.678558825948271327 ) ) ;
#71348=CARTESIAN_POINT ( 'NONE',  ( 82.10840107674059141, 54.12326372724951540, 15.62324998714231050 ) ) ;
#71352=CARTESIAN_POINT ( 'NONE',  ( 69.48308982531537481, 68.85812419773016302, -7.057691085508246864 ) ) ;
#71356=CARTESIAN_POINT ( 'NONE',  ( 65.81996430066485004, 68.94383839650693346, -2.301213135912207886 ) ) ;
#71360=CARTESIAN_POINT ( 'NONE',  ( 26.56877070717806433, 23.84335787977763843, 9.188101187500006262 ) ) ;
#71361=CARTESIAN_POINT ( 'NONE',  ( 79.97118972361107581, 44.44405107747005701, 11.63932608780695510 ) ) ;
#71362=CARTESIAN_POINT ( 'NONE',  ( 84.64469814230420752, 50.57817590239302064, -14.03985074783417630 ) ) ;
#71365=ADVANCED_FACE ( 'NONE', ( #81544 ), #8638, .T. ) ;
#71373=CARTESIAN_POINT ( 'NONE',  ( 67.84078594043214139, 65.66857331658644625, 10.81805557313897737 ) ) ;
#71377=CARTESIAN_POINT ( 'NONE',  ( 40.97195624589149077, 25.78380873178789656, -6.180339887498949025 ) ) ;
#71381=CARTESIAN_POINT ( 'NONE',  ( 75.48556727315214232, 61.63299524387726080, -15.75020862335680150 ) ) ;
#71387=CARTESIAN_POINT ( 'NONE',  ( 78.11917150362724271, 61.95746172053952705, -16.05486485196055568 ) ) ;
#71390=ORIENTED_EDGE ( 'NONE', *, *, #23850, .F. ) ;
#71391=CARTESIAN_POINT ( 'NONE',  ( 80.06816492365965132, 44.55418465396458316, -11.68679231591616308 ) ) ;
#71395=CARTESIAN_POINT ( 'NONE',  ( 81.91428016588723438, 47.98820967271630877, -12.92198026695155910 ) ) ;
#71403=CARTESIAN_POINT ( 'NONE',  ( 76.00174837439909936, 64.70029647188280819, -14.33957986251690997 ) ) ;
#71404=CARTESIAN_POINT ( 'NONE',  ( 68.07113691668065769, 69.08423509312365240, -4.762053786030961966 ) ) ;
#71406=CARTESIAN_POINT ( 'NONE',  ( 87.89236927835047197, 44.79168309952778060, 4.915177569529609158 ) ) ;
#71407=ORIENTED_EDGE ( 'NONE', *, *, #44210, .F. ) ;
#71418=CARTESIAN_POINT ( 'NONE',  ( 84.22395731584195744, 42.64873031269722503, 4.526430362304276755 ) ) ;
#71420=CARTESIAN_POINT ( 'NONE',  ( 83.26710953215496147, 52.37668708275160867, 14.85863008173918942 ) ) ;
#71427=FACE_BOUND ( 'NONE', #79606, .T. ) ;
#71430=CARTESIAN_POINT ( 'NONE',  ( 29.80052344588228408, 32.90829794293883026, 10.00000000000000355 ) ) ;
#71431=CARTESIAN_POINT ( 'NONE',  ( 78.01406954259199722, 47.82291453140933157, 14.04263472196524098 ) ) ;
#71439=CARTESIAN_POINT ( 'NONE',  ( 82.21261018562424283, 47.88076305863328486, 12.73987827041416843 ) ) ;
#71440=EDGE_LOOP ( 'NONE', ( #64136, #71244, #100257, #82066 ) ) ;
#71443=CARTESIAN_POINT ( 'NONE',  ( 27.87997788293534285, 34.83478043621390441, -8.090169943749479842 ) ) ;
#71445=CARTESIAN_POINT ( 'NONE',  ( 82.13419662640586694, 41.24805531849482065, 5.427534581471942232 ) ) ;
#71448=CARTESIAN_POINT ( 'NONE',  ( 35.24645901769773815, 32.30066082961424456, -10.00000000000000533 ) ) ;
#71452=CARTESIAN_POINT ( 'NONE',  ( 81.44543282719071442, 56.09797068433638145, 16.07152707150316928 ) ) ;
#71460=CARTESIAN_POINT ( 'NONE',  ( 73.79739402942419702, 66.12004107874481917, -12.74733577929619521 ) ) ;
#71467=CARTESIAN_POINT ( 'NONE',  ( 67.03142477407426725, 66.84972006921925924, -8.889086588726858196 ) ) ;
#71473=CARTESIAN_POINT ( 'NONE',  ( 28.30082151474694641, 24.84335787977763843, 9.188101187500006262 ) ) ;
#71478=CARTESIAN_POINT ( 'NONE',  ( 43.87294039959300562, 25.73415679381825427, 1.333680081654574804E-15 ) ) ;
#71479=CARTESIAN_POINT ( 'NONE',  ( 12.79414888559916719, 13.10170272979925166, -7.433330006724141015 ) ) ;
#71480=CARTESIAN_POINT ( 'NONE',  ( 74.29045190397653187, 59.50555543665407043, -15.65878564717055177 ) ) ;
#71481=CARTESIAN_POINT ( 'NONE',  ( 71.90447592081905270, 72.59379857415109427, -1.170934825568553439 ) ) ;
#71484=CARTESIAN_POINT ( 'NONE',  ( 72.50273111209941135, 71.24117241184434590, -6.063735550250077821 ) ) ;
#71485=CARTESIAN_POINT ( 'NONE',  ( 82.18753490691527475, 40.78579184768808830, -0.6546124752527386903 ) ) ;
#71488=VERTEX_POINT ( 'NONE', #40375 ) ;
#71490=ADVANCED_FACE ( 'NONE', ( #72321 ), #41889, .T. ) ;
#71496=CARTESIAN_POINT ( 'NONE',  ( 72.86052486178445520, 57.38405094451463384, -15.86408618498019685 ) ) ;
#71497=CARTESIAN_POINT ( 'NONE',  ( 76.70982964007059479, 63.62857842591434832, 15.32478313419208149 ) ) ;
#71505=CARTESIAN_POINT ( 'NONE',  ( 74.73487060833782891, 53.69418506457893869, 16.08953207461605928 ) ) ;
#71507=EDGE_CURVE ( 'NONE', #11479, #63738, #38637, .T. ) ;
#71508=CARTESIAN_POINT ( 'NONE',  ( 23.32838594064934767, 31.65586893147757408, -7.433330006724137462 ) ) ;
#71510=CARTESIAN_POINT ( 'NONE',  ( 78.35220796506176555, 47.87217679057071251, -14.51592191970564727 ) ) ;
#71512=CARTESIAN_POINT ( 'NONE',  ( 74.17419530692131957, 68.61376803465689989, 11.49684454571891479 ) ) ;
#71517=VERTEX_POINT ( 'NONE', #79442 ) ;
#71518=CARTESIAN_POINT ( 'NONE',  ( 74.44275639589338311, 58.61260243895608113, -15.83339419040879648 ) ) ;
#71519=CARTESIAN_POINT ( 'NONE',  ( 85.30525313256302411, 43.13218841966886430, -4.103031163142204285 ) ) ;
#71524=CARTESIAN_POINT ( 'NONE',  ( 69.09727653224064170, 69.59326890348451400, -5.001431338550271555 ) ) ;
#71530=CARTESIAN_POINT ( 'NONE',  ( 67.66641119600812715, 66.78092416874584103, 8.593359544578680342 ) ) ;
#71534=EDGE_LOOP ( 'NONE', ( #7520, #93669, #11856, #48182 ) ) ;
#71539=CARTESIAN_POINT ( 'NONE',  ( 83.63875120450398981, 51.47261955259384791, -14.38664681448914884 ) ) ;
#71552=CARTESIAN_POINT ( 'NONE',  ( 77.46790047979986582, 60.10606210004741712, -16.34033675906437111 ) ) ;
#71554=CARTESIAN_POINT ( 'NONE',  ( 88.00610859356287108, 44.56460208309338356, -4.030656215517964824 ) ) ;
#71555=B_SPLINE_SURFACE_WITH_KNOTS ( 'NONE', 3, 1, ( 
 ( #65186, #95136 ),
 ( #41374, #1899 ),
 ( #17080, #10001 ),
 ( #24683, #96134 ),
 ( #88549, #32779 ),
 ( #71811, #2407 ),
 ( #57576, #33811 ),
 ( #48996, #94625 ),
 ( #33286, #64695 ),
 ( #88054, #95648 ),
 ( #26195, #79932 ),
 ( #57074, #64187 ),
 ( #40368, #18603 ),
 ( #11011, #19115 ),
 ( #49991, #80946 ),
 ( #87569, #25182 ),
 ( #49482, #18096 ),
 ( #56062, #17590 ),
 ( #11514, #79437 ),
 ( #42368, #63185 ),
 ( #65676, #60056 ),
 ( #89066, #13982 ),
 ( #82444, #97611 ),
 ( #81429, #12000 ),
 ( #74317, #75299 ),
 ( #12501, #44857 ),
 ( #74809, #35282 ),
 ( #59050, #5880 ),
 ( #96630, #43370 ),
 ( #27197, #4899 ),
 ( #28179, #58086 ) ),
 .UNSPECIFIED., .F., .F., .F.,
 ( 4, 3, 3, 3, 3, 3, 3, 3, 3, 3, 4 ),
 ( 2, 2 ),
 ( 0.000000000000000000, 0.1333490885032416196, 0.3007194338854398130, 0.4699862290245220287, 0.5844252810809438259, 0.6686540514502733457, 0.7354980260655562541, 0.8028463152565635808, 0.8633854507757173780, 0.9437142632667323561, 1.000000000000000000 ),
 ( 0.000000000000000000, 1.000000000000000000 ),
 .UNSPECIFIED. ) ;
#71556=CARTESIAN_POINT ( 'NONE',  ( 71.69160970194380411, 71.06503076016720399, -5.341200118771810779 ) ) ;
#71563=CARTESIAN_POINT ( 'NONE',  ( 77.82435850266757882, 52.78930163363708061, -15.75762069573296387 ) ) ;
#71569=CARTESIAN_POINT ( 'NONE',  ( 12.54686387532899516, 29.01751292744055277, 6.180339887498949913 ) ) ;
#71570=FACE_OUTER_BOUND ( 'NONE', #50779, .T. ) ;
#71571=CARTESIAN_POINT ( 'NONE',  ( 80.75597752872654667, 49.71520906199375389, -14.73179648239882056 ) ) ;
#71572=CARTESIAN_POINT ( 'NONE',  ( 72.01517167333473424, 59.31195453282659003, -15.33353692504408272 ) ) ;
#71573=CARTESIAN_POINT ( 'NONE',  ( 72.25916493420206166, 71.97815949024219151, 3.567716402802650677 ) ) ;
#71582=EDGE_CURVE ( 'NONE', #38703, #14677, #52843, .T. ) ;
#71585=PLANE ( 'NONE',  #76531 ) ;
#71588=CARTESIAN_POINT ( 'NONE',  ( 35.77750112005064409, 38.84336893147759184, -7.433330006724137462 ) ) ;
#71591=DIRECTION ( 'NONE',  ( -0.8660254037844377084, -0.5000000000000014433, -0.000000000000000000 ) ) ;
#71592=CARTESIAN_POINT ( 'NONE',  ( 31.65185205300530313, 23.98920272979928114, 7.433330006724137462 ) ) ;
#71595=CARTESIAN_POINT ( 'NONE',  ( 66.05706222625097723, 68.55736014781324172, 2.107737461089805642 ) ) ;
#71599=CARTESIAN_POINT ( 'NONE',  ( 10.54248283575963008, 11.80170272979924206, 7.433330006724137462 ) ) ;
#71601=CARTESIAN_POINT ( 'NONE',  ( 13.67041502465407277, 29.93396525600389424, 2.839279412974139660 ) ) ;
#71607=CARTESIAN_POINT ( 'NONE',  ( 23.70688097944214334, 37.18528772668520332, -1.583844403245329602 ) ) ;
#71610=CARTESIAN_POINT ( 'NONE',  ( 66.26630907207875509, 68.23277418650276616, 4.087305060687866920 ) ) ;
#71617=CARTESIAN_POINT ( 'NONE',  ( 86.36983145024699127, 47.62973577336905606, 10.65328243325163804 ) ) ;
#71619=CARTESIAN_POINT ( 'NONE',  ( 77.63646380548019010, 56.82889395091936535, 16.18249514420208257 ) ) ;
#71624=EDGE_CURVE ( 'NONE', #37549, #85355, #3370, .T. ) ;
#71625=CARTESIAN_POINT ( 'NONE',  ( 15.92326719930538204, 21.14441083166260071, 10.00000000000000533 ) ) ;
#71632=ORIENTED_EDGE ( 'NONE', *, *, #34989, .T. ) ;
#71635=CARTESIAN_POINT ( 'NONE',  ( 41.56734871454121816, 26.12755873383629535, -6.180339887498949025 ) ) ;
#71639=CARTESIAN_POINT ( 'NONE',  ( 74.17829915416689346, 64.94294222156766239, 13.63034475538133350 ) ) ;
#71642=ORIENTED_EDGE ( 'NONE', *, *, #90130, .T. ) ;
#71643=CARTESIAN_POINT ( 'NONE',  ( 76.26946404230703536, 64.97317754398874001, 14.67006731301516176 ) ) ;
#71646=CARTESIAN_POINT ( 'NONE',  ( 70.74027447083685161, 68.01839942184822974, 9.368956669706040685 ) ) ;
#71648=B_SPLINE_CURVE_WITH_KNOTS ( 'NONE', 3,
 ( #1930, #46500, #94658, #77436, #8034, #38907, #23700, #38222, #68641, #99562, #68145, #14459, #92972, #83896, #29653, #99072, #92000, #69137, #75773, #22047, #15424, #23028, #76746, #83391 ),
 .UNSPECIFIED., .F., .F.,
 ( 4, 2, 2, 2, 2, 2, 2, 2, 2, 2, 2, 4 ),
 ( 0.000000000000000000, 0.1250000000000111300, 0.2500000000000222600, 0.3750000000000334177, 0.4375000000000321410, 0.5000000000000308642, 0.5625000000000295319, 0.6250000000000281997, 0.6875000000000268674, 0.7500000000000255351, 0.8750000000000128786, 1.000000000000000000 ),
 .UNSPECIFIED. ) ;
#71655=CARTESIAN_POINT ( 'NONE',  ( 22.06543860749898300, 21.24335787977763346, -9.188101187500008038 ) ) ;
#71669=DIRECTION ( 'NONE',  ( -0.8660254037844377084, -0.5000000000000014433, -0.000000000000000000 ) ) ;
#71670=CARTESIAN_POINT ( 'NONE',  ( 74.73078456835840200, 66.79972942087576371, -13.15602295301254543 ) ) ;
#71679=CARTESIAN_POINT ( 'NONE',  ( 75.55347530004152645, 65.47672821233528850, 13.82195870221527123 ) ) ;
#71684=CARTESIAN_POINT ( 'NONE',  ( 78.77678738312307871, 47.31940876559444575, -13.55958224463107165 ) ) ;
#71685=PLANE ( 'NONE',  #46701 ) ;
#71693=CARTESIAN_POINT ( 'NONE',  ( 84.24277800523259430, 48.02810533160893414, 12.01781408871613266 ) ) ;
#71714=CARTESIAN_POINT ( 'NONE',  ( 23.42942861845947178, 22.03085787977762777, 9.188101187500006262 ) ) ;
#71724=CARTESIAN_POINT ( 'NONE',  ( 86.41689343025348080, 47.58309788860988476, 10.57565383929702563 ) ) ;
#71730=CARTESIAN_POINT ( 'NONE',  ( 83.84059829558975707, 51.56187102439434256, -14.37481623513500040 ) ) ;
#71736=CARTESIAN_POINT ( 'NONE',  ( 37.18479240120036167, 39.65586893147759895, -7.433330006724137462 ) ) ;
#71739=CARTESIAN_POINT ( 'NONE',  ( 78.13090640523601849, 61.76054338150410672, 16.10053832301867516 ) ) ;
#71742=EDGE_LOOP ( 'NONE', ( #92813, #16508, #68620, #83586 ) ) ;
#71743=CARTESIAN_POINT ( 'NONE',  ( 79.49274628814450239, 59.57836040576013659, 16.53926144102299389 ) ) ;
#71746=CARTESIAN_POINT ( 'NONE',  ( 80.82219357636691370, 51.10915316415084675, -14.83884473207257670 ) ) ;
#71747=CARTESIAN_POINT ( 'NONE',  ( 80.47142419695269666, 44.41285142414567844, 11.35032686343901354 ) ) ;
#71749=ORIENTED_EDGE ( 'NONE', *, *, #22330, .F. ) ;
#71750=ORIENTED_EDGE ( 'NONE', *, *, #72194, .F. ) ;
#71753=CARTESIAN_POINT ( 'NONE',  ( 81.25645528111445515, 55.75359181263093689, 16.38715272843555226 ) ) ;
#71756=CARTESIAN_POINT ( 'NONE',  ( 79.50406474403273194, 54.96663328783942148, 16.02396390402955006 ) ) ;
#71759=CARTESIAN_POINT ( 'NONE',  ( 25.81463925578599117, 37.83705186507755514, 3.090169943749475401 ) ) ;
#71767=CARTESIAN_POINT ( 'NONE',  ( 70.79886843151163589, 61.41865354507500996, -14.84698767043841627 ) ) ;
#71768=CARTESIAN_POINT ( 'NONE',  ( 43.17480782474465428, 33.43085787977766898, -9.188101187500008038 ) ) ;
#71772=CARTESIAN_POINT ( 'NONE',  ( 85.68664465223866955, 48.45350732935998650, -12.23334744974731869 ) ) ;
#71778=CARTESIAN_POINT ( 'NONE',  ( 80.76436682390523458, 43.05937393749385222, 9.753329205520538281 ) ) ;
#71784=CARTESIAN_POINT ( 'NONE',  ( 65.82437617505169669, 69.12761414359022183, -0.3171011309739659167 ) ) ;
#71785=ORIENTED_EDGE ( 'NONE', *, *, #95640, .T. ) ;
#71801=CARTESIAN_POINT ( 'NONE',  ( 74.94581410820386225, 65.07354109301314793, -13.82487701360099486 ) ) ;
#71802=B_SPLINE_CURVE_WITH_KNOTS ( 'NONE', 3,
 ( #93883, #42976, #10245, #71556, #33032, #70530, #20217, #89179, #55803, #41115, #35401, #50593, #55317, #81543, #16831, #86796, #2152, #12114, #63931, #94870, #17331, #72049, #27807, #58682, #82050, #9241, #47718, #89655, #25432, #12623, #17850, #95398, #1147, #78655, #53582, #60670, #66797, #21701, #74923, #84536, #83541, #29798, #36389, #21215, #5504, #67804 ),
 .UNSPECIFIED., .F., .F.,
 ( 4, 1, 2, 2, 1, 2, 2, 1, 1, 2, 2, 1, 1, 2, 2, 1, 1, 2, 2, 1, 1, 1, 2, 2, 1, 1, 1, 2, 2, 4 ),
 ( 0.000000000000000000, 0.06250000000001508516, 0.09375000000002250977, 0.1250000000000299483, 0.1875000000000420775, 0.2187500000000465739, 0.2500000000000510703, 0.3125000000000602851, 0.3437500000000658362, 0.3593750000000670020, 0.3750000000000681122, 0.4375000000000753841, 0.4687500000000789924, 0.4843750000000808242, 0.5000000000000826006, 0.5625000000000942579, 0.5937500000000983658, 0.6093750000001009193, 0.6250000000001034728, 0.6875000000001139089, 0.7187500000001180167, 0.7343750000001182388, 0.7421875000001172396, 0.7500000000001161293, 0.8125000000000947020, 0.8437500000000832667, 0.8593750000000782707, 0.8671875000000739409, 0.8750000000000696110, 1.000000000000000000 ),
 .UNSPECIFIED. ) ;
#71804=CARTESIAN_POINT ( 'NONE',  ( 73.89028189157257032, 68.56231543382321547, 11.39439152759356944 ) ) ;
#71807=CARTESIAN_POINT ( 'NONE',  ( 67.68166703610724255, 69.53423434588013663, 2.055755005019128667 ) ) ;
#71811=CARTESIAN_POINT ( 'NONE',  ( 88.18429177444041045, 44.53138063026126048, -4.871266200417320391 ) ) ;
#71814=CARTESIAN_POINT ( 'NONE',  ( 77.77751611803083165, 53.46578304951030702, 15.90232757848929523 ) ) ;
#71820=CARTESIAN_POINT ( 'NONE',  ( 81.22424941298332612, 53.84597802519924414, -15.65359963525670217 ) ) ;
#71821=CARTESIAN_POINT ( 'NONE',  ( 79.47466498719533945, 53.91538503943934302, -16.25957047384575915 ) ) ;
#71823=CARTESIAN_POINT ( 'NONE',  ( 71.69164292429383067, 72.03424767056361588, -1.595364931656152674 ) ) ;
#71826=CARTESIAN_POINT ( 'NONE',  ( 76.74023481339004604, 63.31925950119924096, -15.43993991125870124 ) ) ;
#71831=CARTESIAN_POINT ( 'NONE',  ( 75.73407124508247534, 53.49751973368108082, -16.50271086146291211 ) ) ;
#71836=CARTESIAN_POINT ( 'NONE',  ( 28.70736568013821355, 22.28920272979928185, -7.433330006724141015 ) ) ;
#71839=ORIENTED_EDGE ( 'NONE', *, *, #72475, .T. ) ;
#71840=CARTESIAN_POINT ( 'NONE',  ( 22.99159801516092472, 18.98920272979926693, 7.433330006724137462 ) ) ;
#71842=CYLINDRICAL_SURFACE ( 'NONE', #96708, 15.60714546451156970 ) ;
#71850=LINE ( 'NONE', #94167, #8619 ) ;
#71851=CARTESIAN_POINT ( 'NONE',  ( 75.32116640173099142, 53.12209477811269664, 16.48561212775914697 ) ) ;
#71854=VERTEX_POINT ( 'NONE', #85942 ) ;
#71862=CARTESIAN_POINT ( 'NONE',  ( 79.11275361910446691, 46.11146926033848104, 13.27945046499836579 ) ) ;
#71866=CARTESIAN_POINT ( 'NONE',  ( 36.63328578856461348, 23.01110640527294748, 2.839279412974134775 ) ) ;
#71867=CARTESIAN_POINT ( 'NONE',  ( 79.75726243291551043, 44.80792267523282391, 11.39221341620031502 ) ) ;
#71868=CARTESIAN_POINT ( 'NONE',  ( 84.77725617564227889, 50.41784377465270950, -13.48640040656236927 ) ) ;
#71869=CARTESIAN_POINT ( 'NONE',  ( 78.06375342405178230, 49.62358045365419201, -14.80969209974775325 ) ) ;
#71875=CARTESIAN_POINT ( 'NONE',  ( 67.79725476218452229, 65.71048819351142356, 10.00598338191752390 ) ) ;
#71880=CARTESIAN_POINT ( 'NONE',  ( 78.28621045032348036, 60.56628696945801238, -16.35393821005401804 ) ) ;
#71883=B_SPLINE_CURVE_WITH_KNOTS ( 'NONE', 3,
 ( #19720, #67284, #20707, #65300, #42479, #89173, #28794, #65785, #59674, #51594, #73413, #82549, #35888, #66301, #97233, #96743, #66790, #4000, #58192, #96242, #4495, #89647, #74425, #27306, #12107, #98211, #26803, #35391, #20208, #90134, #5009, #50585, #52086, #27801, #90648, #97716, #13114, #81535, #28284, #58675, #51080, #82042, #57686, #74914, #5496, #12616 ),
 .UNSPECIFIED., .F., .F.,
 ( 4, 1, 2, 2, 1, 2, 2, 1, 1, 2, 2, 1, 1, 2, 2, 1, 1, 2, 2, 1, 1, 1, 2, 2, 1, 1, 1, 2, 2, 4 ),
 ( 0.000000000000000000, 0.06249999999999761302, 0.09374999999999655831, 0.1249999999999955036, 0.1874999999999933942, 0.2187499999999937550, 0.2499999999999941158, 0.3124999999999954481, 0.3437499999999967248, 0.3593749999999983347, 0.3749999999999998890, 0.4374999999999985012, 0.4687499999999967804, 0.4843749999999955591, 0.4999999999999943379, 0.5624999999999901190, 0.5937499999999876765, 0.6093749999999867883, 0.6249999999999860112, 0.6874999999999786837, 0.7187499999999742428, 0.7343749999999733546, 0.7421874999999722444, 0.7499999999999710232, 0.8124999999999769074, 0.8437499999999799050, 0.8593749999999821254, 0.8671874999999829026, 0.8749999999999835687, 1.000000000000000000 ),
 .UNSPECIFIED. ) ;
#71887=CARTESIAN_POINT ( 'NONE',  ( 78.16855185334185308, 61.58847221756811052, -16.14202726422458767 ) ) ;
#71889=EDGE_LOOP ( 'NONE', ( #11841, #24505, #90581, #73818 ) ) ;
#71890=CARTESIAN_POINT ( 'NONE',  ( 73.67824366217406862, 55.52431661998092238, 16.58293631993679540 ) ) ;
#71892=CARTESIAN_POINT ( 'NONE',  ( 80.42973500905783624, 44.73750331184790952, -11.66451360117097558 ) ) ;
#71894=PLANE ( 'NONE',  #74062 ) ;
#71895=CARTESIAN_POINT ( 'NONE',  ( 34.35958382788741261, 28.03677371833804344, 10.00000000000000533 ) ) ;
#71902=EDGE_CURVE ( 'NONE', #49096, #58645, #48383, .T. ) ;
#71903=CARTESIAN_POINT ( 'NONE',  ( 75.67384099942408682, 65.13299740138256766, -14.43017819244620803 ) ) ;
#71904=CARTESIAN_POINT ( 'NONE',  ( 71.69170005589681693, 69.37806338950922225, -8.395052771507090839 ) ) ;
#71906=CARTESIAN_POINT ( 'NONE',  ( 88.16762080519842470, 44.42520534355205797, 4.589585637743891056 ) ) ;
#71908=CARTESIAN_POINT ( 'NONE',  ( 87.42460433697408462, 44.12820928407189314, -3.507511662899541527 ) ) ;
#71919=CARTESIAN_POINT ( 'NONE',  ( 85.59540126815005578, 44.41612895177246401, 6.888311711144287308 ) ) ;
#71921=CARTESIAN_POINT ( 'NONE',  ( 77.99842658917772553, 61.99000515389445809, 15.67651427494045890 ) ) ;
#71927=CARTESIAN_POINT ( 'NONE',  ( 74.12482479103741184, 55.26569620697679852, 16.12359666345034626 ) ) ;
#71928=CARTESIAN_POINT ( 'NONE',  ( 69.59282007774174872, 62.40894646771045018, -13.45448169915730041 ) ) ;
#71929=CARTESIAN_POINT ( 'NONE',  ( 37.20204829050883433, 21.28848085856233752, 1.475505719884397138E-15 ) ) ;
#71933=CARTESIAN_POINT ( 'NONE',  ( 87.73298548431468191, 44.18903561216112763, 4.633618514853090176 ) ) ;
#71937=CARTESIAN_POINT ( 'NONE',  ( 82.04497822609438629, 47.34932639374565611, 12.42682962033639527 ) ) ;
#71943=CARTESIAN_POINT ( 'NONE',  ( 82.28113228126468925, 41.34250681205937639, 5.451554181100740415 ) ) ;
#71947=CARTESIAN_POINT ( 'NONE',  ( 34.38043361391329711, 31.80066082961424812, 10.00000000000000533 ) ) ;
#71956=CARTESIAN_POINT ( 'NONE',  ( 70.21489987089526608, 66.74148169577378553, -10.42873902553350085 ) ) ;
#71964=ORIENTED_EDGE ( 'NONE', *, *, #13908, .F. ) ;
#71967=CARTESIAN_POINT ( 'NONE',  ( 81.17232691891707930, 55.55242957854174080, 16.36487835605631602 ) ) ;
#71969=CARTESIAN_POINT ( 'NONE',  ( 29.15721111571870594, 19.76004757982090965, 5.678558825948272215 ) ) ;
#71974=CARTESIAN_POINT ( 'NONE',  ( 15.84867609773810138, 11.01110640527290840, 2.839279412974134775 ) ) ;
#71976=CARTESIAN_POINT ( 'NONE',  ( 71.63329245445480353, 72.42139875791372106, -1.350275132429440861 ) ) ;
#71979=CARTESIAN_POINT ( 'NONE',  ( 85.07250665400066225, 48.93453557688312117, 12.41781952940225153 ) ) ;
#71989=CARTESIAN_POINT ( 'NONE',  ( 71.98264401366868981, 72.39816763649429276, -2.869464145551836598 ) ) ;
#71990=CARTESIAN_POINT ( 'NONE',  ( 72.66110749420992931, 57.51441285064596087, -16.30982310438753657 ) ) ;
#71991=CARTESIAN_POINT ( 'NONE',  ( 77.33488381500329467, 63.19222936695796733, 15.59520410795408196 ) ) ;
#71996=EDGE_CURVE ( 'NONE', #82006, #25263, #11403, .T. ) ;
#72000=CARTESIAN_POINT ( 'NONE',  ( 31.43713336585798146, 20.01110640527293683, 2.839279412974134775 ) ) ;
#72002=CARTESIAN_POINT ( 'NONE',  ( 78.41593629422656875, 47.90319055863865572, -14.51313888544015995 ) ) ;
#72005=CARTESIAN_POINT ( 'NONE',  ( 74.28707621773548908, 68.55768173149772338, 11.10544092197707755 ) ) ;
#72010=EDGE_LOOP ( 'NONE', ( #33987, #60228, #64252, #83717 ) ) ;
#72017=EDGE_CURVE ( 'NONE', #19430, #54490, #98817, .T. ) ;
#72024=CARTESIAN_POINT ( 'NONE',  ( 68.91022223105564137, 64.71151235087043574, -12.22836756590942464 ) ) ;
#72029=CARTESIAN_POINT ( 'NONE',  ( 85.05810897262044534, 44.16933612965711831, -6.971008100970949251 ) ) ;
#72034=CARTESIAN_POINT ( 'NONE',  ( 83.46712633478475141, 51.63463124265641824, -14.88389777197023456 ) ) ;
#72035=CARTESIAN_POINT ( 'NONE',  ( 76.06472804764035800, 51.19927304191299555, -15.61780489609254197 ) ) ;
#72037=CARTESIAN_POINT ( 'NONE',  ( 80.46882139176624094, 57.60428850591405592, -16.59250918983046574 ) ) ;
#72048=EDGE_CURVE ( 'NONE', #95936, #94224, #38300, .T. ) ;
#72049=CARTESIAN_POINT ( 'NONE',  ( 69.19930876265073039, 70.42046229790001632, -2.224448151379176508 ) ) ;
#72058=CARTESIAN_POINT ( 'NONE',  ( 80.74219536503451877, 51.86096535971582000, -15.10915280358188895 ) ) ;
#72060=B_SPLINE_CURVE_WITH_KNOTS ( 'NONE', 3,
 ( #64634, #66120, #97069, #27640, #79375, #41811, #34227, #40801, #34715, #42796, #27137, #72759, #57010, #95586, #41304, #35218, #18039, #65615, #71746, #96570, #96070, #11940, #87989, #58022, #25635, #9938, #65123, #89004, #73730, #57512, #18538, #86990, #56517, #19554, #81372, #26628, #19050, #3351, #88488, #50414, #49421, #4314, #3830, #2339, #17520, #33222 ),
 .UNSPECIFIED., .F., .F.,
 ( 4, 1, 2, 2, 1, 2, 2, 1, 1, 2, 2, 1, 1, 2, 2, 1, 1, 2, 2, 1, 1, 1, 2, 2, 1, 1, 1, 2, 2, 4 ),
 ( 0.000000000000000000, 0.06249999999999249212, 0.09374999999998884226, 0.1249999999999852063, 0.1874999999999779066, 0.2187499999999762135, 0.2499999999999745204, 0.3124999999999669709, 0.3437499999999650280, 0.3593749999999655831, 0.3749999999999661382, 0.4374999999999704681, 0.4687499999999723554, 0.4843749999999731881, 0.4999999999999740208, 0.5624999999999785727, 0.5937499999999806821, 0.6093749999999837907, 0.6249999999999868994, 0.6874999999999896749, 0.7187499999999907851, 0.7343749999999892308, 0.7421874999999884537, 0.7499999999999876765, 0.8124999999999982236, 0.8437500000000037748, 0.8593750000000081046, 0.8671875000000084377, 0.8750000000000086597, 1.000000000000000000 ),
 .UNSPECIFIED. ) ;
#72063=CARTESIAN_POINT ( 'NONE',  ( 17.03907575219864867, 18.03677371833801146, 10.00000000000000533 ) ) ;
#72064=B_SPLINE_CURVE_WITH_KNOTS ( 'NONE', 3,
 ( #4666, #66458, #97383, #44628, #27950, #58832, #20372, #51243, #5163, #66943, #28446, #59326, #90306, #16242, #23330, #37531, #93788, #1050, #69930, #39022, #60819, #68436, #30940, #91781, #52730, #92291, #15731, #61331, #99365, #38021, #69439 ),
 .UNSPECIFIED., .F., .F.,
 ( 4, 3, 3, 3, 3, 3, 3, 3, 3, 3, 4 ),
 ( 0.000000000000000000, 0.1333490885032285189, 0.3007194338854188853, 0.4699862290244924967, 0.5844252810809184018, 0.6686540514502693489, 0.7354980260655538116, 0.8028463152565737948, 0.8633854507757268149, 0.9437142632667515629, 1.000000000000000000 ),
 .UNSPECIFIED. ) ;
#72066=CARTESIAN_POINT ( 'NONE',  ( 23.96727898247415212, 22.03677371833801857, 10.00000000000000533 ) ) ;
#72068=CARTESIAN_POINT ( 'NONE',  ( 82.63770679579928924, 49.15890594283347781, -13.91020417536396003 ) ) ;
#72070=CARTESIAN_POINT ( 'NONE',  ( 72.18677484676699407, 72.08588332058079118, 3.002544651710248758 ) ) ;
#72074=ADVANCED_FACE ( 'NONE', ( #19982 ), #65074, .T. ) ;
#72084=CARTESIAN_POINT ( 'NONE',  ( 34.12723495145388597, 35.10171378149922106, 9.188101187500008038 ) ) ;
#72088=CARTESIAN_POINT ( 'NONE',  ( 32.92443518896833154, 39.98502408145596121, -5.678558825948271327 ) ) ;
#72092=CARTESIAN_POINT ( 'NONE',  ( 43.32193544081557945, 25.41603393254330001, -1.583844403245396437 ) ) ;
#72095=CARTESIAN_POINT ( 'NONE',  ( 8.534987971495436199, 16.87878583063839599, -9.188101187500006262 ) ) ;
#72097=CARTESIAN_POINT ( 'NONE',  ( 19.63753723929501760, 13.19860640527291551, 2.839279412974134775 ) ) ;
#72099=VECTOR ( 'NONE', #2006, 1000.000000000000114 ) ;
#72100=CARTESIAN_POINT ( 'NONE',  ( 84.60739412327551179, 49.90025452092439906, -13.66407646797534703 ) ) ;
#72107=CARTESIAN_POINT ( 'NONE',  ( 66.05163167928934342, 68.53992083822487302, 4.515471496088387049 ) ) ;
#72108=CARTESIAN_POINT ( 'NONE',  ( 87.47489022187491514, 45.51477803643930287, 7.025279742117177761 ) ) ;
#72110=EDGE_LOOP ( 'NONE', ( #70345, #11872, #93563, #96298 ) ) ;
#72112=CARTESIAN_POINT ( 'NONE',  ( 85.90360539940944307, 47.54977701528212464, 10.84765075726303785 ) ) ;
#72114=CARTESIAN_POINT ( 'NONE',  ( 77.85016660199350724, 58.06595483709381256, 16.16712961033420015 ) ) ;
#72116=ORIENTED_EDGE ( 'NONE', *, *, #45370, .F. ) ;
#72118=CARTESIAN_POINT ( 'NONE',  ( 79.25252407528778065, 59.49743072449278714, -16.53464936128686347 ) ) ;
#72119=CARTESIAN_POINT ( 'NONE',  ( 82.85318063129575705, 47.73104734800577376, -12.93175278804887185 ) ) ;
#72120=CARTESIAN_POINT ( 'NONE',  ( 80.48263234248918252, 43.57791934932684796, 9.754260794015122471 ) ) ;
#72121=ORIENTED_EDGE ( 'NONE', *, *, #99957, .T. ) ;
#72136=DIRECTION ( 'NONE',  ( 0.4386133837897796539, 0.6599160945941811018, -0.6100238090894840592 ) ) ;
#72140=CARTESIAN_POINT ( 'NONE',  ( 69.50297104555633609, 65.22433265006822012, 11.43951683047897205 ) ) ;
#72147=CARTESIAN_POINT ( 'NONE',  ( 16.40018271037384068, 27.65586893147755987, -7.433330006724137462 ) ) ;
#72151=ORIENTED_EDGE ( 'NONE', *, *, #9491, .F. ) ;
#72155=CARTESIAN_POINT ( 'NONE',  ( 80.91225347342312091, 52.52757887018025684, -15.32176213838356738 ) ) ;
#72164=CYLINDRICAL_SURFACE ( 'NONE', #84046, 16.60714546451156792 ) ;
#72169=CARTESIAN_POINT ( 'NONE',  ( 82.65268600941737986, 40.56492479297515530, -1.423195747375628928 ) ) ;
#72175=ORIENTED_EDGE ( 'NONE', *, *, #36113, .F. ) ;
#72178=CARTESIAN_POINT ( 'NONE',  ( 69.25966472908447713, 70.58289072661317221, 0.9580429418411622322 ) ) ;
#72180=CARTESIAN_POINT ( 'NONE',  ( 33.43624804430746877, 19.70852965304480620, 1.583844403245330712 ) ) ;
#72183=CARTESIAN_POINT ( 'NONE',  ( 68.52907269813512414, 64.25491985315194654, 11.77327033154230840 ) ) ;
#72189=CARTESIAN_POINT ( 'NONE',  ( 79.31708208686120543, 59.64451620468175719, -16.52545681491535134 ) ) ;
#72190=EDGE_CURVE ( 'NONE', #10543, #39006, #39467, .T. ) ;
#72194=EDGE_CURVE ( 'NONE', #47356, #5374, #23437, .T. ) ;
#72195=CARTESIAN_POINT ( 'NONE',  ( 68.90356118335428448, 64.71243317138014106, -12.22457433626360945 ) ) ;
#72210=CARTESIAN_POINT ( 'NONE',  ( 18.45699304436188015, 28.84336893147756342, -7.433330006724137462 ) ) ;
#72211=CARTESIAN_POINT ( 'NONE',  ( 80.15404930735284950, 58.24487849859603017, -16.60713908503101877 ) ) ;
#72216=EDGE_LOOP ( 'NONE', ( #87402, #62478, #36057, #50297, #74881 ) ) ;
#72221=CARTESIAN_POINT ( 'NONE',  ( 81.55294353520883988, 55.93325196641738017, -16.02942048421892096 ) ) ;
#72223=CARTESIAN_POINT ( 'NONE',  ( 69.02380705549570905, 66.01831451487439040, -11.15343670725473402 ) ) ;
#72226=CARTESIAN_POINT ( 'NONE',  ( 71.95794525336513914, 72.58301972798901147, 1.600903759350535749 ) ) ;
#72227=CARTESIAN_POINT ( 'NONE',  ( 80.09789180664904507, 54.17278058467296376, 15.81966211497349484 ) ) ;
#72228=CARTESIAN_POINT ( 'NONE',  ( 83.91681368584680456, 51.76886007642450949, -14.44478906560582310 ) ) ;
#72229=CARTESIAN_POINT ( 'NONE',  ( 87.04122873496829982, 46.31593380912285340, -9.298662157179387933 ) ) ;
#72233=CARTESIAN_POINT ( 'NONE',  ( 83.10776606998568639, 40.75710275334526500, -2.573362665496658816E-06 ) ) ;
#72234=CARTESIAN_POINT ( 'NONE',  ( 13.50812563192542548, 9.927558733836244542, 6.180339887498953466 ) ) ;
#72238=EDGE_CURVE ( 'NONE', #40804, #77173, #9774, .T. ) ;
#72240=CARTESIAN_POINT ( 'NONE',  ( 86.47161471182764103, 44.02354154034633638, -6.066641966162809041 ) ) ;
#72241=ORIENTED_EDGE ( 'NONE', *, *, #65292, .T. ) ;
#72248=CARTESIAN_POINT ( 'NONE',  ( 80.55710883583050474, 44.52789654886623794, 11.41067263359725992 ) ) ;
#72249=CARTESIAN_POINT ( 'NONE',  ( 84.70579481679399692, 49.94286076369812832, -13.65556694543043825 ) ) ;
#72252=VERTEX_POINT ( 'NONE', #41130 ) ;
#72258=CARTESIAN_POINT ( 'NONE',  ( 88.35456099112356299, 44.18765297829227023, 0.2632442814954262245 ) ) ;
#72262=CARTESIAN_POINT ( 'NONE',  ( 82.24971233127639891, 41.19297818149956925, 3.242131167557051441 ) ) ;
#72263=CARTESIAN_POINT ( 'NONE',  ( 71.90400658755810070, 72.53437165389429708, 1.750395423964758557 ) ) ;
#72271=CARTESIAN_POINT ( 'NONE',  ( 70.43431413140284292, 61.24050369869113553, -14.83292379404218231 ) ) ;
#72273=CARTESIAN_POINT ( 'NONE',  ( 85.71030961992515529, 48.80922481583876049, -12.49884386288094440 ) ) ;
#72291=CARTESIAN_POINT ( 'NONE',  ( 66.21613658270437952, 69.35617794467320607, 0.1791810972791403056 ) ) ;
#72302=CARTESIAN_POINT ( 'NONE',  ( 75.54185705060035616, 61.33622908259397377, -15.40001492952482742 ) ) ;
#72304=CARTESIAN_POINT ( 'NONE',  ( 72.94657399261465969, 65.67239758029106156, -12.71627414374669307 ) ) ;
#72306=CARTESIAN_POINT ( 'NONE',  ( 80.76782053159526242, 43.13182372017047328, -9.836536121486679107 ) ) ;
#72307=CARTESIAN_POINT ( 'NONE',  ( 67.01113894376084090, 68.95971538285371594, 3.001280692439017184 ) ) ;
#72317=CARTESIAN_POINT ( 'NONE',  ( 74.77499314424673571, 55.31988034793729270, -16.13510914276501396 ) ) ;
#72321=FACE_OUTER_BOUND ( 'NONE', #9342, .T. ) ;
#72328=CARTESIAN_POINT ( 'NONE',  ( 76.77824862278549745, 55.54507606913799833, -16.16088072629311156 ) ) ;
#72329=DIRECTION ( 'NONE',  ( -0.8660254037844379305, -0.5000000000000014433, -0.000000000000000000 ) ) ;
#72331=CARTESIAN_POINT ( 'NONE',  ( 73.49483902118549850, 69.87589544865461733, 9.786909576851130055 ) ) ;
#72333=CARTESIAN_POINT ( 'NONE',  ( 76.88818783305237048, 63.31965297372375545, -15.46890590930648912 ) ) ;
#72336=CARTESIAN_POINT ( 'NONE',  ( 76.36065199378450075, 53.31052631447248302, -16.44376018799239958 ) ) ;
#72337=CYLINDRICAL_SURFACE ( 'NONE', #9344, 16.60714546451156792 ) ;
#72339=ADVANCED_FACE ( 'NONE', ( #74064 ), #91963, .T. ) ;
#72341=CARTESIAN_POINT ( 'NONE',  ( 35.70653501523218409, 32.56628583063843507, 9.188101187500006262 ) ) ;
#72342=AXIS2_PLACEMENT_3D ( 'NONE', #37744, #13973, #38234 ) ;
#72343=CARTESIAN_POINT ( 'NONE',  ( 79.17986403524099615, 49.31136220171410400, -14.94917676811451379 ) ) ;
#72344=CARTESIAN_POINT ( 'NONE',  ( 84.11950711319154550, 46.87244309510325024, -11.07336435221286131 ) ) ;
#72345=ORIENTED_EDGE ( 'NONE', *, *, #73279, .F. ) ;
#72346=CARTESIAN_POINT ( 'NONE',  ( 15.07467606819624173, 24.10171378149917842, 9.188101187500008038 ) ) ;
#72356=CARTESIAN_POINT ( 'NONE',  ( 87.44817167685637571, 45.02922442914869805, -6.108700660266276117 ) ) ;
#72359=EDGE_LOOP ( 'NONE', ( #33507, #33789, #87531, #91856 ) ) ;
#72367=CARTESIAN_POINT ( 'NONE',  ( 76.90746743093833970, 62.93938289886319382, -15.23233999435670150 ) ) ;
#72373=CARTESIAN_POINT ( 'NONE',  ( 27.20206195878591870, 37.74646525600392266, 2.839279412974139660 ) ) ;
#72374=CARTESIAN_POINT ( 'NONE',  ( 82.06425201348349674, 48.60968897072322648, -13.24680869277554862 ) ) ;
#72376=CARTESIAN_POINT ( 'NONE',  ( 82.41933087055697627, 40.38430946167127900, -0.8419157719606891188 ) ) ;
#72377=ORIENTED_EDGE ( 'NONE', *, *, #7138, .F. ) ;
#72382=CARTESIAN_POINT ( 'NONE',  ( 85.41398746878978443, 48.60267188261818916, 12.47190137721841019 ) ) ;
#72385=CARTESIAN_POINT ( 'NONE',  ( 70.72929604436274076, 60.91355080922355114, 15.04203567179363965 ) ) ;
#72398=CARTESIAN_POINT ( 'NONE',  ( 79.95370688104166845, 44.47433224906099980, -10.99098430061395604 ) ) ;
#72403=ADVANCED_FACE ( 'NONE', ( #82697 ), #16111, .T. ) ;
#72404=FACE_OUTER_BOUND ( 'NONE', #12591, .T. ) ;
#72413=ORIENTED_EDGE ( 'NONE', *, *, #17444, .T. ) ;
#72415=CARTESIAN_POINT ( 'NONE',  ( 25.64360150771697633, 30.50829794293882102, -10.00000000000000355 ) ) ;
#72416=CARTESIAN_POINT ( 'NONE',  ( 70.79495161673614234, 69.39911685413080988, -7.528900684444595370 ) ) ;
#72417=CARTESIAN_POINT ( 'NONE',  ( 87.38898754588738882, 44.84176836479306871, -6.666552467508535251 ) ) ;
#72419=CARTESIAN_POINT ( 'NONE',  ( 87.54784588100407916, 44.59992802364795494, 4.936297260842060552 ) ) ;
#72420=ORIENTED_EDGE ( 'NONE', *, *, #47156, .F. ) ;
#72423=CARTESIAN_POINT ( 'NONE',  ( 80.41304442479348324, 45.09799279809392658, 11.31444151523504260 ) ) ;
#72433=CARTESIAN_POINT ( 'NONE',  ( 84.54996403203030297, 43.01056371783313637, 5.045017719461522887 ) ) ;
#72434=CARTESIAN_POINT ( 'NONE',  ( 83.14271255481067158, 52.19653239224700059, 14.81391299184662813 ) ) ;
#72437=CARTESIAN_POINT ( 'NONE',  ( 29.01663622185449753, 35.49103043416550918, -8.090169943749479842 ) ) ;
#72442=CARTESIAN_POINT ( 'NONE',  ( 31.34407949807308569, 36.83478043621390441, -8.090169943749479842 ) ) ;
#72447=CARTESIAN_POINT ( 'NONE',  ( 82.93837572039436168, 43.22210157649355722, -7.357460665149816670 ) ) ;
#72449=CARTESIAN_POINT ( 'NONE',  ( 81.49265314619182732, 45.83748706731968525, 11.45477345881717213 ) ) ;
#72450=VERTEX_POINT ( 'NONE', #90295 ) ;
#72452=B_SPLINE_CURVE_WITH_KNOTS ( 'NONE', 3,
 ( #48118, #65320, #33944, #34419, #10128, #88183, #79061, #16719, #17211, #57206, #18234, #80568, #47613, #96258, #26330, #40506, #87202, #32425, #79570, #9647, #78540, #71439, #2028, #94755, #71937, #95281, #17734, #2542, #86680, #63320, #94260, #33424, #72449, #24815, #25843, #56718, #49129, #10633, #41509, #3056, #95776, #100104, #66317, #69172, #30688, #88680 ),
 .UNSPECIFIED., .F., .F.,
 ( 4, 1, 2, 2, 1, 2, 2, 1, 1, 2, 2, 1, 1, 2, 2, 1, 1, 2, 2, 1, 1, 1, 2, 2, 1, 1, 1, 2, 2, 4 ),
 ( 0.000000000000000000, 0.06250000000000034694, 0.09375000000000031919, 0.1250000000000003053, 0.1875000000000009159, 0.2187500000000013600, 0.2500000000000017764, 0.3125000000000036637, 0.3437500000000032752, 0.3593750000000032196, 0.3750000000000031641, 0.4375000000000084377, 0.4687500000000107137, 0.4843750000000112133, 0.5000000000000117684, 0.5625000000000167644, 0.5937500000000199840, 0.6093750000000217604, 0.6250000000000236478, 0.6875000000000259792, 0.7187500000000272005, 0.7343750000000270894, 0.7421875000000278666, 0.7500000000000287548, 0.8125000000000195399, 0.8437500000000142109, 0.8593750000000117684, 0.8671875000000103251, 0.8750000000000089928, 1.000000000000000000 ),
 .UNSPECIFIED. ) ;
#72453=CARTESIAN_POINT ( 'NONE',  ( 86.54933037531351658, 46.26600125392582186, 8.987360782618976529 ) ) ;
#72454=CARTESIAN_POINT ( 'NONE',  ( 13.69028360280385570, 30.83705186507753382, 3.090169943749475401 ) ) ;
#72461=CARTESIAN_POINT ( 'NONE',  ( 29.10553579016685077, 39.73705186507756082, -3.090169943749475845 ) ) ;
#72467=CARTESIAN_POINT ( 'NONE',  ( 87.15443966109820906, 46.07157893991718822, -8.233590127383161317 ) ) ;
#72468=CARTESIAN_POINT ( 'NONE',  ( 83.41128051646016672, 51.86661034151835992, 14.99497567496408301 ) ) ;
#72475=EDGE_CURVE ( 'NONE', #45639, #92014, #52230, .T. ) ;
#72479=CARTESIAN_POINT ( 'NONE',  ( 67.67290550563593854, 66.83298015526837332, -8.527019564984499311 ) ) ;
#72486=CARTESIAN_POINT ( 'NONE',  ( 24.44940106416278169, 29.51421378149920116, -9.188101187500004485 ) ) ;
#72490=ORIENTED_EDGE ( 'NONE', *, *, #36373, .T. ) ;
#72492=CARTESIAN_POINT ( 'NONE',  ( 11.20403028766721398, 24.65586893147754921, -7.433330006724137462 ) ) ;
#72500=ORIENTED_EDGE ( 'NONE', *, *, #15983, .F. ) ;
#72505=CARTESIAN_POINT ( 'NONE',  ( 34.73896580337741113, 43.55466486950702887, 7.012934429366973338E-14 ) ) ;
#72506=CARTESIAN_POINT ( 'NONE',  ( 72.01037534753049840, 72.25474680761037405, -3.568257732133948590 ) ) ;
#72507=CARTESIAN_POINT ( 'NONE',  ( 72.62323068768809264, 57.44918900967634556, -16.31697738479318716 ) ) ;
#72508=CARTESIAN_POINT ( 'NONE',  ( 78.16005489154372299, 61.02200473696554894, -15.90480247637162137 ) ) ;
#72516=CARTESIAN_POINT ( 'NONE',  ( 39.89592612264573290, 25.96004757982093025, -5.678558825948276656 ) ) ;
#72520=CARTESIAN_POINT ( 'NONE',  ( 73.81469611240122219, 68.48838210847161179, 10.92215486908102839 ) ) ;
#72525=CARTESIAN_POINT ( 'NONE',  ( 77.11906017550013814, 57.72506332681559371, -16.14635887841112094 ) ) ;
#72532=EDGE_CURVE ( 'NONE', #15648, #54612, #90215, .T. ) ;
#72533=CARTESIAN_POINT ( 'NONE',  ( 80.54443990458493374, 52.78455055202924484, -15.87853153993444622 ) ) ;
#72536=CARTESIAN_POINT ( 'NONE',  ( 82.57385212973971989, 41.04541115053230982, -1.138833187496899768 ) ) ;
#72537=CARTESIAN_POINT ( 'NONE',  ( 79.14312167556931854, 57.64441083166269664, 0.000000000000000000 ) ) ;
#72541=VECTOR ( 'NONE', #41194, 1000.000000000000000 ) ;
#72544=CARTESIAN_POINT ( 'NONE',  ( 84.31659741720631018, 44.16501652472276618, -7.663753778293648011 ) ) ;
#72546=CARTESIAN_POINT ( 'NONE',  ( 74.83655476910678317, 53.51806293180211327, 16.54630480343736210 ) ) ;
#72548=CARTESIAN_POINT ( 'NONE',  ( 74.95985714465535921, 62.05307465897563901, 15.09129879184485290 ) ) ;
#72550=ORIENTED_EDGE ( 'NONE', *, *, #93781, .T. ) ;
#72551=CARTESIAN_POINT ( 'NONE',  ( 80.64201675847387207, 57.55060183585958811, -16.24056620613974644 ) ) ;
#72555=CARTESIAN_POINT ( 'NONE',  ( 75.63268008801900066, 65.14737934564519151, -14.41129995628930516 ) ) ;
#72563=CARTESIAN_POINT ( 'NONE',  ( 20.76744934909352125, 17.15404122711133184, 8.090169943749479842 ) ) ;
#72571=CARTESIAN_POINT ( 'NONE',  ( 83.23897458906459690, 51.01732238469139702, -14.23410810326086740 ) ) ;
#72579=CARTESIAN_POINT ( 'NONE',  ( 20.54487693938818538, 27.56454794089042082, 10.00000000000000355 ) ) ;
#72580=CARTESIAN_POINT ( 'NONE',  ( 88.06269261788008862, 43.61796610520790551, 0.05835779599787207367 ) ) ;
#72582=CARTESIAN_POINT ( 'NONE',  ( 71.98264401366868981, 72.39816763649429276, -2.869464145551835710 ) ) ;
#72584=CARTESIAN_POINT ( 'NONE',  ( 73.95722056738210881, 55.62591273403975123, -16.58564036811612041 ) ) ;
#72596=CARTESIAN_POINT ( 'NONE',  ( 38.14222467998226307, 24.94754757982092386, 5.678558825948272215 ) ) ;
#72598=ADVANCED_FACE ( 'NONE', ( #9529 ), #63711, .T. ) ;
#72600=CARTESIAN_POINT ( 'NONE',  ( 28.71100085020356474, 39.68290643055189548, 3.479690158560446702E-15 ) ) ;
#72607=CARTESIAN_POINT ( 'NONE',  ( 7.668962567711002265, 16.37878583063838533, 9.188101187500006262 ) ) ;
#72609=CARTESIAN_POINT ( 'NONE',  ( 16.50122538818396478, 18.03085787977762777, 9.188101187500006262 ) ) ;
#72618=CARTESIAN_POINT ( 'NONE',  ( 66.29568901166975081, 68.16417104789285020, 4.350792714150624185 ) ) ;
#72624=CARTESIAN_POINT ( 'NONE',  ( 86.22252119400383208, 47.68394482253771116, 10.79685758221453007 ) ) ;
#72625=ORIENTED_EDGE ( 'NONE', *, *, #2938, .F. ) ;
#72629=CARTESIAN_POINT ( 'NONE',  ( 78.35930054750417639, 61.15116583347188595, -15.90188674197529473 ) ) ;
#72633=CARTESIAN_POINT ( 'NONE',  ( 80.51848489276528653, 43.48937927821671678, 9.625745649737424969 ) ) ;
#72636=CARTESIAN_POINT ( 'NONE',  ( 67.21491844529386128, 62.30466486950709992, 1.224646799147354045E-15 ) ) ;
#72641=EDGE_CURVE ( 'NONE', #95607, #21672, #17615, .T. ) ;
#72650=LINE ( 'NONE', #18435, #43150 ) ;
#72656=CARTESIAN_POINT ( 'NONE',  ( 86.51811418199767445, 43.18311598531779794, 0.5570016322997576319 ) ) ;
#72661=CARTESIAN_POINT ( 'NONE',  ( 19.79331822069313418, 23.37878583063840665, 9.188101187500006262 ) ) ;
#72663=CARTESIAN_POINT ( 'NONE',  ( 83.19608331955247138, 41.11598378048204694, -3.025298033747441107 ) ) ;
#72668=CARTESIAN_POINT ( 'NONE',  ( 84.06604358195920668, 51.46910565605918464, 14.65639964578790710 ) ) ;
#72671=CARTESIAN_POINT ( 'NONE',  ( 78.89368875498706757, 46.43720108942829228, 12.98266078055406680 ) ) ;
#72676=CARTESIAN_POINT ( 'NONE',  ( 72.04273812837080015, 59.28583566120335746, 15.84548535902080246 ) ) ;
#72681=CARTESIAN_POINT ( 'NONE',  ( 82.50844557763632281, 41.01330284059301334, -1.198675424783806287 ) ) ;
#72683=CARTESIAN_POINT ( 'NONE',  ( 17.65531800687426056, 22.14441083166260427, 10.00000000000000533 ) ) ;
#72692=CARTESIAN_POINT ( 'NONE',  ( 88.32078559155080200, 44.16791947909882765, 0.3596700509409204716 ) ) ;
#72693=CARTESIAN_POINT ( 'NONE',  ( 83.32940628703454422, 42.65613730677653592, 5.827714800416384122 ) ) ;
#72697=( BOUNDED_CURVE ( )  B_SPLINE_CURVE ( 2, ( #65554, #43238, #74181, #88937, #4771, #66554, #5258, #36140, #67043, #59424, #90403, #82800, #34169 ),
 .UNSPECIFIED., .F., .T. ) 
 B_SPLINE_CURVE_WITH_KNOTS ( ( 3, 2, 2, 2, 2, 2, 3 ),
 ( 0.06250000000000000000, 0.06500000000000000222, 0.07000000000000000666, 0.07499999999999999722, 0.08000000000000000167, 0.08500000000000000611, 0.08750000000000000833 ),
 .UNSPECIFIED. ) 
 CURVE ( )  GEOMETRIC_REPRESENTATION_ITEM ( )  RATIONAL_B_SPLINE_CURVE ( ( 0.9755282581475768211, 0.9755282581475768211, 1.000000000000000000, 0.9510565162951535312, 1.000000000000000000, 0.9510565162951535312, 1.000000000000000000, 0.9510565162951535312, 1.000000000000000000, 0.9510565162951535312, 1.000000000000000000, 0.9755282581475767101, 0.9755282581475768211 ) ) 
 REPRESENTATION_ITEM ( '' )  );
#72699=CARTESIAN_POINT ( 'NONE',  ( 73.82480279627529285, 68.30552952313148296, -11.59219441058860589 ) ) ;
#72703=CARTESIAN_POINT ( 'NONE',  ( 81.88992170983947005, 42.99646257747416200, 7.919497295398134185 ) ) ;
#72709=CARTESIAN_POINT ( 'NONE',  ( 68.75122914510536987, 64.15569240841469423, -11.94966557906562166 ) ) ;
#72711=DIRECTION ( 'NONE',  ( 0.9634819383873034493, -0.2491829092639731569, -0.09803281150812268030 ) ) ;
#72714=DIRECTION ( 'NONE',  ( 0.000000000000000000, 0.000000000000000000, -1.000000000000000000 ) ) ;
#72722=CARTESIAN_POINT ( 'NONE',  ( 26.01786902700012405, 17.94754757982089899, 5.678558825948272215 ) ) ;
#72723=CARTESIAN_POINT ( 'NONE',  ( 74.99160476570628475, 67.13646269190913074, 13.03024426091169197 ) ) ;
#72734=CARTESIAN_POINT ( 'NONE',  ( 81.73893769428700296, 55.29113635392555892, -15.92164997284989703 ) ) ;
#72742=CARTESIAN_POINT ( 'NONE',  ( 79.67407917426849906, 52.06013808976464929, 15.34621390177021283 ) ) ;
#72744=CARTESIAN_POINT ( 'NONE',  ( 72.31870688955723381, 71.66728745601001549, -5.813503713761849490 ) ) ;
#72747=CARTESIAN_POINT ( 'NONE',  ( 14.26996179277632848, 9.208019796199270246, -3.090169943749474069 ) ) ;
#72749=ORIENTED_EDGE ( 'NONE', *, *, #71902, .F. ) ;
#72752=CARTESIAN_POINT ( 'NONE',  ( 83.58619102057019745, 43.97462430113206011, -8.849062569972019787 ) ) ;
#72755=CARTESIAN_POINT ( 'NONE',  ( 79.33204938572286835, 59.85669560537334632, 16.15623921946350450 ) ) ;
#72757=CARTESIAN_POINT ( 'NONE',  ( 70.34454795188869980, 61.29844696716961749, 14.78467410895967760 ) ) ;
#72758=VECTOR ( 'NONE', #31907, 999.9999999999998863 ) ;
#72759=CARTESIAN_POINT ( 'NONE',  ( 82.22619446726943693, 50.63112855324299488, -14.32323471781884372 ) ) ;
#72767=CARTESIAN_POINT ( 'NONE',  ( 77.47491854863321237, 49.58014053284396283, 14.91146804420484528 ) ) ;
#72769=CARTESIAN_POINT ( 'NONE',  ( 74.54111643893327255, 56.67881626048158239, 16.07342755282378377 ) ) ;
#72770=VECTOR ( 'NONE', #87240, 1000.000000000000114 ) ;
#72772=ORIENTED_EDGE ( 'NONE', *, *, #66651, .T. ) ;
#72773=EDGE_CURVE ( 'NONE', #21377, #60539, #85138, .T. ) ;
#72774=CARTESIAN_POINT ( 'NONE',  ( 82.52834598917124254, 40.78028802545565412, 3.192646178055736694 ) ) ;
#72775=CARTESIAN_POINT ( 'NONE',  ( 85.04377965201177858, 48.84687674572034410, 12.36303725827022149 ) ) ;
#72780=CARTESIAN_POINT ( 'NONE',  ( 29.08982151148960682, 17.76426979415090912, 3.090169943749476733 ) ) ;
#72781=EDGE_CURVE ( 'NONE', #9880, #99877, #17809, .T. ) ;
#72783=CARTESIAN_POINT ( 'NONE',  ( 70.80606192109750907, 61.41720523217159666, -14.84941795604011539 ) ) ;
#72796=CARTESIAN_POINT ( 'NONE',  ( 70.99909089399695006, 61.09348569631758608, 14.50421621802051853 ) ) ;
#72798=CARTESIAN_POINT ( 'NONE',  ( 76.45572749639896415, 51.64231386251727685, -16.15369532822336751 ) ) ;
#72802=CARTESIAN_POINT ( 'NONE',  ( 75.64425446922575702, 62.03138304502632394, -15.24332385036787052 ) ) ;
#72803=ORIENTED_EDGE ( 'NONE', *, *, #10932, .T. ) ;
#72804=LINE ( 'NONE', #26668, #24108 ) ;
#72813=CARTESIAN_POINT ( 'NONE',  ( 72.20202516581701957, 62.31549783853672153, -14.29472092056413501 ) ) ;
#72817=CARTESIAN_POINT ( 'NONE',  ( 80.64028050891147359, 43.44267665222750452, -9.484970014585552889 ) ) ;
#72825=CARTESIAN_POINT ( 'NONE',  ( 81.49135018016791321, 59.57715975391656116, -0.01744974835125552223 ) ) ;
#72826=CARTESIAN_POINT ( 'NONE',  ( 75.70758752364832844, 55.03446575750268721, -16.13395138078375268 ) ) ;
#72835=CARTESIAN_POINT ( 'NONE',  ( 77.02263550477385934, 63.85671778288190836, -15.30752586418454086 ) ) ;
#72844=CARTESIAN_POINT ( 'NONE',  ( 33.10845880387886808, 31.06628583063843863, -9.188101187500006262 ) ) ;
#72847=EDGE_LOOP ( 'NONE', ( #68347, #34833, #64133, #92740 ) ) ;
#72848=CARTESIAN_POINT ( 'NONE',  ( 23.27484393518965788, 15.29860640527292226, -2.839279412974138328 ) ) ;
#72855=CARTESIAN_POINT ( 'NONE',  ( 70.33404001443909692, 61.26294760300035591, 14.79771436642047533 ) ) ;
#72857=CARTESIAN_POINT ( 'NONE',  ( 72.20842434904899676, 71.50474725277734933, 5.031331199130571363 ) ) ;
#72858=CARTESIAN_POINT ( 'NONE',  ( 87.32127743178345725, 44.99235608909022233, -6.181280657231217113 ) ) ;
#72869=CARTESIAN_POINT ( 'NONE',  ( 77.31286743954092344, 63.20723050550007827, -15.22062317857226965 ) ) ;
#72870=EDGE_LOOP ( 'NONE', ( #45375, #99038, #38192, #84775 ) ) ;
#72877=CARTESIAN_POINT ( 'NONE',  ( 27.74993340135630859, 36.99752408145592852, 5.678558825948276656 ) ) ;
#72878=CARTESIAN_POINT ( 'NONE',  ( 81.31198753610523511, 48.79742522285970807, -13.59794317573495981 ) ) ;
#72888=CARTESIAN_POINT ( 'NONE',  ( 85.75771426040881806, 48.69409737863756504, -11.92208042066353535 ) ) ;
#72891=DIRECTION ( 'NONE',  ( -0.8660254037844379305, -0.5000000000000014433, -0.000000000000000000 ) ) ;
#72905=CARTESIAN_POINT ( 'NONE',  ( 71.38860822316976851, 59.37102963310187675, 15.21422888946525731 ) ) ;
#72906=CARTESIAN_POINT ( 'NONE',  ( 85.19546613154977877, 42.46598081436301442, -0.1273095977939074364 ) ) ;
#72914=ORIENTED_EDGE ( 'NONE', *, *, #98351, .T. ) ;
#72915=CARTESIAN_POINT ( 'NONE',  ( 76.03425298724704362, 64.70400164203398674, -14.34693053486635606 ) ) ;
#72917=CARTESIAN_POINT ( 'NONE',  ( 72.94457269381892672, 69.24349002572374445, -9.567436796043198299 ) ) ;
#72921=DIRECTION ( 'NONE',  ( 0.8845109580947966288, -0.1124011590738275557, -0.4527762631246090574 ) ) ;
#72924=CARTESIAN_POINT ( 'NONE',  ( 80.65166287433959269, 45.65901089857030115, 11.68184599996163797 ) ) ;
#72926=CARTESIAN_POINT ( 'NONE',  ( 82.28003896804979433, 40.62557011389661454, -3.142018250930367795 ) ) ;
#72933=CARTESIAN_POINT ( 'NONE',  ( 85.70872427756812328, 44.59920998664200198, 7.110704347725950392 ) ) ;
#72935=CARTESIAN_POINT ( 'NONE',  ( 78.04004269445073305, 61.96668518898951561, 15.68684486111242293 ) ) ;
#72937=EDGE_CURVE ( 'NONE', #39006, #4740, #59455, .T. ) ;
#72940=CARTESIAN_POINT ( 'NONE',  ( 74.32104487728463482, 55.32907616431677411, 16.60218531702808065 ) ) ;
#72942=CARTESIAN_POINT ( 'NONE',  ( 34.10980067877857635, 31.64441083166263269, -10.00000000000000533 ) ) ;
#72947=CARTESIAN_POINT ( 'NONE',  ( 86.86181906774642414, 43.72161649829373431, -3.208833253784785011 ) ) ;
#72952=CARTESIAN_POINT ( 'NONE',  ( 86.78549426258132371, 45.83013854792883279, 8.849882187839877901 ) ) ;
#72953=CARTESIAN_POINT ( 'NONE',  ( 88.42017002704760387, 43.92753743058676719, 1.721442031696316377 ) ) ;
#72959=CARTESIAN_POINT ( 'NONE',  ( 32.74284248606149106, 41.83705186507756224, 3.090169943749475401 ) ) ;
#72965=CARTESIAN_POINT ( 'NONE',  ( 74.39841895140679640, 68.21392270468032848, 11.95628786500076934 ) ) ;
#72967=EDGE_CURVE ( 'NONE', #66065, #63171, #57500, .T. ) ;
#72975=CARTESIAN_POINT ( 'NONE',  ( 67.44824590140864018, 66.75839308862164501, -8.448268966284212311 ) ) ;
#72980=CARTESIAN_POINT ( 'NONE',  ( 30.88926192328758447, 20.76004757982090609, 5.678558825948272215 ) ) ;
#72982=CARTESIAN_POINT ( 'NONE',  ( 86.16184129357679922, 46.97112889942257397, -10.09731433673572276 ) ) ;
#72985=CARTESIAN_POINT ( 'NONE',  ( 15.78914702631840150, 24.51421378149918695, -9.188101187500004485 ) ) ;
#72990=CARTESIAN_POINT ( 'NONE',  ( 72.34188612886940462, 71.14473754787812254, -6.071946735866348810 ) ) ;
#73000=ORIENTED_EDGE ( 'NONE', *, *, #71996, .T. ) ;
#73001=CARTESIAN_POINT ( 'NONE',  ( 65.87995410094603699, 68.93345956842472333, -2.563197177700018425 ) ) ;
#73003=CARTESIAN_POINT ( 'NONE',  ( 72.59318330222436089, 57.33635058732104994, -16.33242561347062960 ) ) ;
#73004=CARTESIAN_POINT ( 'NONE',  ( 77.84440724905273612, 61.40677674231441330, -16.14086307328630809 ) ) ;
#73011=CARTESIAN_POINT ( 'NONE',  ( 29.13557404741141355, 37.79752408145594700, -5.678558825948271327 ) ) ;
#73013=CARTESIAN_POINT ( 'NONE',  ( 78.26893986734688724, 47.80136226004309208, -14.50496253017350767 ) ) ;
#73020=CARTESIAN_POINT ( 'NONE',  ( 78.00315723853645977, 57.40260998422804306, -16.18978363693141276 ) ) ;
#73022=CARTESIAN_POINT ( 'NONE',  ( 86.66305821822952282, 42.85738816998053835, 1.351321920865392823 ) ) ;
#73025=CARTESIAN_POINT ( 'NONE',  ( 70.64645261124985609, 69.81531829990819915, -6.590501872596628452 ) ) ;
#73027=CARTESIAN_POINT ( 'NONE',  ( 83.08469416262596496, 51.79154804246269350, -15.04490442047335641 ) ) ;
#73042=CARTESIAN_POINT ( 'NONE',  ( 75.18665594272103192, 63.32462222244616612, 14.68879760224534436 ) ) ;
#73045=CARTESIAN_POINT ( 'NONE',  ( 80.25178558894602077, 57.14685393251871659, -16.23521980932008546 ) ) ;
#73046=CARTESIAN_POINT ( 'NONE',  ( 71.65939579155516981, 72.09010134313686535, 0.6730539622211891837 ) ) ;
#73052=CARTESIAN_POINT ( 'NONE',  ( 68.33041130487251280, 69.19949468873031151, 4.826233711656780834 ) ) ;
#73054=CARTESIAN_POINT ( 'NONE',  ( 14.11247099069668742, 31.08080186712592052, -3.090169943749475845 ) ) ;
#73056=CARTESIAN_POINT ( 'NONE',  ( 41.76871284172324295, 36.06628583063844928, -9.188101187500006262 ) ) ;
#73057=B_SPLINE_CURVE_WITH_KNOTS ( 'NONE', 3,
 ( #81591, #11180, #42047, #12160, #3572, #34453, #29353, #60217, #67850, #68333, #30340, #92194, #39778, #94054, #60713, #91181, #9416, #76457, #59732, #98771, #86474, #70709, #84095, #37425 ),
 .UNSPECIFIED., .F., .F.,
 ( 4, 2, 2, 2, 2, 2, 2, 2, 2, 2, 2, 4 ),
 ( 0.000000000000000000, 0.1249999999999923395, 0.2499999999999846789, 0.3749999999999770184, 0.4374999999999794054, 0.4999999999999817923, 0.5624999999999841238, 0.6249999999999865663, 0.6874999999999888978, 0.7499999999999913403, 0.8749999999999956701, 1.000000000000000000 ),
 .UNSPECIFIED. ) ;
#73062=CARTESIAN_POINT ( 'NONE',  ( 83.41434387094278691, 50.95609258043517542, -14.15981904929085822 ) ) ;
#73063=ORIENTED_EDGE ( 'NONE', *, *, #25001, .F. ) ;
#73069=CARTESIAN_POINT ( 'NONE',  ( 13.69028360280385570, 30.83705186507753382, 3.090169943749475401 ) ) ;
#73070=CARTESIAN_POINT ( 'NONE',  ( 88.07426949318437437, 43.62472922332415237, 0.07787791115677776543 ) ) ;
#73072=CARTESIAN_POINT ( 'NONE',  ( 72.28747768279822594, 72.05077469953971558, -3.362523527234974718 ) ) ;
#73074=CARTESIAN_POINT ( 'NONE',  ( 73.78486849093569333, 55.14556177349142274, -16.59920503071222697 ) ) ;
#73077=CARTESIAN_POINT ( 'NONE',  ( 74.86380167504295002, 67.20554747851282684, 12.49214931513423466 ) ) ;
#73088=CARTESIAN_POINT ( 'NONE',  ( 37.43858582280105907, 33.56628583063844218, 9.188101187500006262 ) ) ;
#73090=EDGE_CURVE ( 'NONE', #82635, #35356, #99858, .T. ) ;
#73092=CARTESIAN_POINT ( 'NONE',  ( 35.70653501523218409, 32.56628583063843507, 9.188101187500006262 ) ) ;
#73096=CARTESIAN_POINT ( 'NONE',  ( 80.75837978203962564, 43.06974379819217091, -9.769810117882439471 ) ) ;
#73100=CARTESIAN_POINT ( 'NONE',  ( 7.739928672529463149, 22.65586893147754211, -7.433330006724137462 ) ) ;
#73102=CARTESIAN_POINT ( 'NONE',  ( 10.75418485208671804, 27.18502408145590366, 5.678558825948276656 ) ) ;
#73105=EDGE_LOOP ( 'NONE', ( #5212, #91829, #27016, #77832 ) ) ;
#73107=FACE_OUTER_BOUND ( 'NONE', #68346, .T. ) ;
#73108=ORIENTED_EDGE ( 'NONE', *, *, #15521, .F. ) ;
#73112=CARTESIAN_POINT ( 'NONE',  ( 87.42157367659969225, 45.50835484090782046, 7.071803456770564544 ) ) ;
#73118=CARTESIAN_POINT ( 'NONE',  ( 86.67919437798869353, 47.13106718819364716, 10.49222478779208068 ) ) ;
#73123=CARTESIAN_POINT ( 'NONE',  ( 33.24377527499414242, 31.14441083166263269, 10.00000000000000533 ) ) ;
#73124=CARTESIAN_POINT ( 'NONE',  ( 80.18890285298550680, 49.85588249849323716, -14.45051987738599486 ) ) ;
#73143=CARTESIAN_POINT ( 'NONE',  ( 86.99613933060332727, 43.49019189568694799, 1.303767148709912505 ) ) ;
#73148=CARTESIAN_POINT ( 'NONE',  ( 20.47532000956703513, 32.79752408145593279, -5.678558825948271327 ) ) ;
#73151=CARTESIAN_POINT ( 'NONE',  ( 77.41810753117228217, 49.76551275768444782, -14.98827377503008584 ) ) ;
#73157=CARTESIAN_POINT ( 'NONE',  ( 69.62506531815498079, 62.65334623341696840, 13.89417082518318836 ) ) ;
#73160=EDGE_CURVE ( 'NONE', #34200, #24743, #53899, .T. ) ;
#73168=EDGE_CURVE ( 'NONE', #12913, #57260, #8109, .T. ) ;
#73177=VERTEX_POINT ( 'NONE', #40657 ) ;
#73179=CARTESIAN_POINT ( 'NONE',  ( 67.71136690417436910, 69.33268738728419578, 3.139524805400198293 ) ) ;
#73186=ORIENTED_EDGE ( 'NONE', *, *, #60072, .T. ) ;
#73187=CARTESIAN_POINT ( 'NONE',  ( 83.75471768118535465, 46.64312366483261485, 11.04520889654889970 ) ) ;
#73189=CARTESIAN_POINT ( 'NONE',  ( 68.79385422379222348, 64.21269200074630135, -11.92370147360801980 ) ) ;
#73194=CARTESIAN_POINT ( 'NONE',  ( 68.71236162956441262, 68.31727361646146335, -8.171850045985486588 ) ) ;
#73200=FACE_OUTER_BOUND ( 'NONE', #83371, .T. ) ;
#73202=CARTESIAN_POINT ( 'NONE',  ( 20.98410315089673261, 24.06628583063841376, -9.188101187500006262 ) ) ;
#73203=CARTESIAN_POINT ( 'NONE',  ( 74.78129183281730263, 67.18734618188521779, 12.47178672914711584 ) ) ;
#73208=CARTESIAN_POINT ( 'NONE',  ( 81.63951372615375135, 59.32053296443953627, -0.4567727288213029868 ) ) ;
#73214=CARTESIAN_POINT ( 'NONE',  ( 81.63547489262985835, 55.73921394657421757, -16.35272683298455476 ) ) ;
#73220=CARTESIAN_POINT ( 'NONE',  ( 85.68836362758381142, 45.52427758709214345, 8.553938247697089992 ) ) ;
#73221=CARTESIAN_POINT ( 'NONE',  ( 80.20007227937493610, 54.77581058227145405, 15.92427733993149985 ) ) ;
#73223=CARTESIAN_POINT ( 'NONE',  ( 72.16236457449060993, 71.55515601828724925, -5.863900035885150075 ) ) ;
#73227=CARTESIAN_POINT ( 'NONE',  ( 7.263013161461002731, 16.14441083166258295, 10.00000000000000533 ) ) ;
#73234=CARTESIAN_POINT ( 'NONE',  ( 78.96241633089614709, 60.10021242361892035, 16.11556649788965601 ) ) ;
#73239=CARTESIAN_POINT ( 'NONE',  ( 84.46699969863880142, 49.90279977532637901, -13.71381277893580197 ) ) ;
#73246=ORIENTED_EDGE ( 'NONE', *, *, #30024, .T. ) ;
#73247=CARTESIAN_POINT ( 'NONE',  ( 75.22035300883564446, 59.77421810351211917, 15.71776402631701686 ) ) ;
#73251=CARTESIAN_POINT ( 'NONE',  ( 82.00610100450838047, 41.07700615983480930, 3.349603895260225173 ) ) ;
#73256=CARTESIAN_POINT ( 'NONE',  ( 23.98812876850004727, 25.80066082961422325, 10.00000000000000533 ) ) ;
#73258=CARTESIAN_POINT ( 'NONE',  ( 75.59476737973361082, 54.41781083123701279, 16.10556637520365442 ) ) ;
#73259=CARTESIAN_POINT ( 'NONE',  ( 15.84867609773810138, 11.01110640527290840, 2.839279412974134775 ) ) ;
#73262=CARTESIAN_POINT ( 'NONE',  ( 85.63146384662782395, 48.39429698310328121, -12.21155806772681629 ) ) ;
#73269=CARTESIAN_POINT ( 'NONE',  ( 70.67229411587209142, 60.84139834894546794, 14.53033638096200875 ) ) ;
#73271=CARTESIAN_POINT ( 'NONE',  ( 85.52015394113763591, 42.90618313698004727, 2.701328592287737251 ) ) ;
#73272=CARTESIAN_POINT ( 'NONE',  ( 88.39284856500222531, 43.98633817645592359, -2.257003550805378733 ) ) ;
#73276=CARTESIAN_POINT ( 'NONE',  ( 65.89235171844839556, 69.16849825365757454, 0.2321662580319230340 ) ) ;
#73279=EDGE_CURVE ( 'NONE', #90112, #95476, #72060, .T. ) ;
#73286=CARTESIAN_POINT ( 'NONE',  ( 88.23680129110753967, 43.93620611740950466, 2.496076054743389783 ) ) ;
#73289=DIRECTION ( 'NONE',  ( 0.03487823687205911238, -0.06041087834082882468, 0.9975640502598247528 ) ) ;
#73292=ADVANCED_FACE ( 'NONE', ( #48427 ), #80369, .T. ) ;
#73296=CARTESIAN_POINT ( 'NONE',  ( 80.77907182703577860, 43.03124623689828354, -9.709161605721851274 ) ) ;
#73311=FACE_OUTER_BOUND ( 'NONE', #84128, .T. ) ;
#73312=CARTESIAN_POINT ( 'NONE',  ( 74.25223132960039152, 56.37754847584465523, -16.09006086798675739 ) ) ;
#73313=FACE_OUTER_BOUND ( 'NONE', #12712, .T. ) ;
#73327=CARTESIAN_POINT ( 'NONE',  ( 35.22599450741489591, 22.19860640527294393, 2.839279412974134775 ) ) ;
#73328=CARTESIAN_POINT ( 'NONE',  ( 84.22812144220274888, 48.05245718175660130, -12.57432882457237966 ) ) ;
#73329=CARTESIAN_POINT ( 'NONE',  ( 74.81457254233032472, 57.45830024592526541, 16.48667394790776086 ) ) ;
#73331=CARTESIAN_POINT ( 'NONE',  ( 14.38185574516869458, 23.70171378149918695, -9.188101187500004485 ) ) ;
#73338=CARTESIAN_POINT ( 'NONE',  ( 86.54431918921495992, 47.23684621844409293, 10.68448168089783756 ) ) ;
#73339=CARTESIAN_POINT ( 'NONE',  ( 72.53811683814018352, 71.57833605577215508, 5.312062988065741287 ) ) ;
#73342=CARTESIAN_POINT ( 'NONE',  ( 28.32887064134541077, 16.75978393459165261, -1.583844403245362020 ) ) ;
#73344=CARTESIAN_POINT ( 'NONE',  ( 85.66375497126256278, 46.86456526682530210, 10.26853249941764012 ) ) ;
#73347=CARTESIAN_POINT ( 'NONE',  ( 72.26191451101281871, 71.91445694603925176, -5.118044210176698527 ) ) ;
#73354=CARTESIAN_POINT ( 'NONE',  ( 88.16744270275496831, 44.54586846255803323, -4.939063992914630497 ) ) ;
#73357=CARTESIAN_POINT ( 'NONE',  ( 37.04286019156342746, 27.10170272979929607, -7.433330006724141015 ) ) ;
#73358=CARTESIAN_POINT ( 'NONE',  ( 73.30726679204248342, 60.50815918352778766, -15.22201117688972971 ) ) ;
#73367=CARTESIAN_POINT ( 'NONE',  ( 85.93449727955278661, 48.41344338607260767, 12.08598331734388509 ) ) ;
#73369=AXIS2_PLACEMENT_3D ( 'NONE', #98124, #36299, #51505 ) ;
#73371=CARTESIAN_POINT ( 'NONE',  ( 70.32079880886523426, 61.21821433514125488, 14.81414658500229109 ) ) ;
#73377=EDGE_LOOP ( 'NONE', ( #23983, #47187, #48538, #88134 ) ) ;
#73379=FACE_OUTER_BOUND ( 'NONE', #22513, .T. ) ;
#73383=CARTESIAN_POINT ( 'NONE',  ( 87.15358044669149251, 46.07130289202554252, -8.233871337641097909 ) ) ;
#73386=CARTESIAN_POINT ( 'NONE',  ( 17.89217828605986327, 10.73415679381820986, 1.333680081654574804E-15 ) ) ;
#73387=CARTESIAN_POINT ( 'NONE',  ( 77.77867966053455007, 61.43039905302717330, -16.12786080876372807 ) ) ;
#73397=CARTESIAN_POINT ( 'NONE',  ( 71.17136799091453270, 69.39928743177321735, -7.895708389734693355 ) ) ;
#73399=CARTESIAN_POINT ( 'NONE',  ( 69.43848462473566485, 62.96533099991498261, -13.64912705282497818 ) ) ;
#73405=CARTESIAN_POINT ( 'NONE',  ( 81.12175378958070837, 46.86607467030008678, 12.41971840815434014 ) ) ;
#73412=CARTESIAN_POINT ( 'NONE',  ( 83.53204454370725784, 52.39401912150449903, -15.17729711222452238 ) ) ;
#73413=CARTESIAN_POINT ( 'NONE',  ( 80.69930153274798101, 53.64823478532364476, 15.66247753479108340 ) ) ;
#73416=CARTESIAN_POINT ( 'NONE',  ( 78.21665545015443399, 61.78861457223207054, 15.74551361518583548 ) ) ;
#73419=CONICAL_SURFACE ( 'NONE', #42654, 16.60714546451156082, 0.7853981633974407295 ) ;
#73420=CARTESIAN_POINT ( 'NONE',  ( 70.38699400097776504, 64.88736316116830949, -12.15252907320628672 ) ) ;
#73421=CARTESIAN_POINT ( 'NONE',  ( 73.51948839908330058, 69.73627507762923017, -9.361350578256050881 ) ) ;
#73424=CARTESIAN_POINT ( 'NONE',  ( 31.84840506572257723, 40.16126292948897003, -6.180339887498951690 ) ) ;
#73426=CARTESIAN_POINT ( 'NONE',  ( 71.64668629127858424, 59.15370159437364350, -15.31769636727452877 ) ) ;
#73427=CARTESIAN_POINT ( 'NONE',  ( 83.00116628026432863, 43.22466567352054767, -7.302193047968875028 ) ) ;
#73435=CARTESIAN_POINT ( 'NONE',  ( 86.99418556918212175, 46.03399372306155612, 8.963501050606421217 ) ) ;
#73437=B_SPLINE_CURVE_WITH_KNOTS ( 'NONE', 3,
 ( #64457, #71573, #17871, #93899, #17348, #48255, #86311, #16353, #93392, #95417, #32557, #72070, #18367, #16846, #1163, #55334, #39127, #48768, #79202, #25973, #2169, #24453, #8754, #63949 ),
 .UNSPECIFIED., .F., .F.,
 ( 4, 2, 2, 2, 2, 2, 2, 2, 2, 2, 2, 4 ),
 ( 0.000000000000000000, 0.1249999999999944211, 0.2499999999999888423, 0.3749999999999832356, 0.4374999999999849565, 0.4999999999999866773, 0.5624999999999884537, 0.6249999999999901190, 0.6874999999999917843, 0.7499999999999933387, 0.8749999999999966693, 1.000000000000000000 ),
 .UNSPECIFIED. ) ;
#73439=CARTESIAN_POINT ( 'NONE',  ( 81.81993950966820250, 41.65085046188367102, 5.428165815223279900 ) ) ;
#73443=CARTESIAN_POINT ( 'NONE',  ( 38.51650576605270260, 30.43677371833804202, -10.00000000000000355 ) ) ;
#73447=CARTESIAN_POINT ( 'NONE',  ( 68.84278490277841911, 67.88251720973005376, -8.019614188230095309 ) ) ;
#73451=CARTESIAN_POINT ( 'NONE',  ( 83.46272733064347449, 51.93221652752758644, 15.00972995268699961 ) ) ;
#73460=FACE_OUTER_BOUND ( 'NONE', #43718, .T. ) ;
#73465=CARTESIAN_POINT ( 'NONE',  ( 23.41017057962146097, 28.91421378149919619, 9.188101187500008038 ) ) ;
#73467=LINE ( 'NONE', #4050, #47292 ) ;
#73469=ORIENTED_EDGE ( 'NONE', *, *, #85523, .F. ) ;
#73470=CARTESIAN_POINT ( 'NONE',  ( 17.90851666933368236, 18.84335787977762067, 9.188101187500006262 ) ) ;
#73471=CARTESIAN_POINT ( 'NONE',  ( 75.98838095635207424, 59.87856586137668558, 15.81821194684219734 ) ) ;
#73476=CARTESIAN_POINT ( 'NONE',  ( 22.49293824011677856, 13.39040679176982707, 1.333680081654574804E-15 ) ) ;
#73477=CARTESIAN_POINT ( 'NONE',  ( 82.18753490691527475, 40.78579184768808830, -0.6546124752527386903 ) ) ;
#73484=CARTESIAN_POINT ( 'NONE',  ( 66.04626366651064018, 69.11317259379546840, -2.045714799961292574 ) ) ;
#73486=CARTESIAN_POINT ( 'NONE',  ( 81.46866702687000839, 55.81909161095428829, 16.37896761046575378 ) ) ;
#73487=CARTESIAN_POINT ( 'NONE',  ( 77.79976927246816842, 61.42068562798239384, -16.13251659512815550 ) ) ;
#73496=CARTESIAN_POINT ( 'NONE',  ( 36.52324494929276710, 26.80170272979929180, 7.433330006724137462 ) ) ;
#73507=CARTESIAN_POINT ( 'NONE',  ( 66.52392041426838887, 68.84470833973988135, -4.415679280545959706 ) ) ;
#73510=CARTESIAN_POINT ( 'NONE',  ( 70.86412831381173305, 69.83143264938641437, -6.808367436344060053 ) ) ;
#73515=CARTESIAN_POINT ( 'NONE',  ( 24.82038151633537026, 14.73415679381822230, 1.333680081654574804E-15 ) ) ;
#73529=CARTESIAN_POINT ( 'NONE',  ( 73.60933432321982650, 55.64367109616565443, 16.10230547196763595 ) ) ;
#73532=CARTESIAN_POINT ( 'NONE',  ( 80.64248598438099691, 57.30349260802955058, -16.23283928966112200 ) ) ;
#73533=EDGE_CURVE ( 'NONE', #2731, #29851, #9172, .T. ) ;
#73538=CARTESIAN_POINT ( 'NONE',  ( 69.22557465782018937, 70.15747877712618674, 3.469537545477277884 ) ) ;
#73541=CARTESIAN_POINT ( 'NONE',  ( 10.82157445631582249, 29.18080186712591839, 3.090169943749475401 ) ) ;
#73555=CARTESIAN_POINT ( 'NONE',  ( 84.36910100733514639, 42.65695583307471139, 5.752001605179764887 ) ) ;
#73556=CARTESIAN_POINT ( 'NONE',  ( 13.10165252270984304, 31.65659080271450421, -1.878358725466461243E-16 ) ) ;
#73559=CARTESIAN_POINT ( 'NONE',  ( 72.18990340680744566, 72.03918383723205920, -3.149060597287212104 ) ) ;
#73564=CARTESIAN_POINT ( 'NONE',  ( 76.96536368249300608, 60.63192262470904836, 16.19594659928378277 ) ) ;
#73573=B_SPLINE_CURVE_WITH_KNOTS ( 'NONE', 3,
 ( #84282, #45716, #76639, #51334, #7224, #38108, #99951, #82302, #12872, #74674 ),
 .UNSPECIFIED., .F., .F.,
 ( 4, 2, 2, 2, 4 ),
 ( 0.000000000000000000, 0.0002622400424272593612, 0.0005244800848545187223, 0.0007867201272817780835, 0.001048960169709037445 ),
 .UNSPECIFIED. ) ;
#73575=CARTESIAN_POINT ( 'NONE',  ( 35.63556891041371699, 26.28920272979929607, -7.433330006724141015 ) ) ;
#73580=CARTESIAN_POINT ( 'NONE',  ( 34.09918582485539673, 43.18528772668523175, -1.583844403245329602 ) ) ;
#73584=CARTESIAN_POINT ( 'NONE',  ( 10.26703877906431472, 17.87878583063839599, -9.188101187500006262 ) ) ;
#73585=CARTESIAN_POINT ( 'NONE',  ( 71.59874412008123556, 72.43189726433809028, 0.9745913883648391618 ) ) ;
#73586=CARTESIAN_POINT ( 'NONE',  ( 11.39049277451480080, 29.68290643055186706, 3.479690158560446702E-15 ) ) ;
#73588=LINE ( 'NONE', #80737, #100157 ) ;
#73590=CARTESIAN_POINT ( 'NONE',  ( 20.35638218401011912, 30.49103043416549497, -8.090169943749479842 ) ) ;
#73596=CARTESIAN_POINT ( 'NONE',  ( 66.36404765992830335, 68.16983728735020520, 4.450399946281168084 ) ) ;
#73597=CARTESIAN_POINT ( 'NONE',  ( 87.68151411726066158, 45.11153824597518280, 6.862463844403655422 ) ) ;
#73601=CARTESIAN_POINT ( 'NONE',  ( 17.29678581741014654, 10.39040679176981996, 1.333680081654574804E-15 ) ) ;
#73608=CARTESIAN_POINT ( 'NONE',  ( 88.48828274770076519, 43.87397573844135934, -0.5490789642627269540 ) ) ;
#73609=CARTESIAN_POINT ( 'NONE',  ( 81.05466020238847591, 43.66611230261246135, 9.465821864999529822 ) ) ;
#73618=VERTEX_POINT ( 'NONE', #43448 ) ;
#73625=CARTESIAN_POINT ( 'NONE',  ( 82.42561518943209364, 53.83419803862934572, 15.85509184085860390 ) ) ;
#73626=CARTESIAN_POINT ( 'NONE',  ( 10.44586698754085674, 29.52903772873355948, -1.583844403245363575 ) ) ;
#73628=CARTESIAN_POINT ( 'NONE',  ( 86.68115352851880573, 43.28345336846571456, 0.8059148367177517702 ) ) ;
#73632=CARTESIAN_POINT ( 'NONE',  ( 78.35675126109745747, 56.49915297402233705, -16.20020041168814018 ) ) ;
#73633=CARTESIAN_POINT ( 'NONE',  ( 21.59633513308047270, 30.65586893147756697, -7.433330006724137462 ) ) ;
#73636=CARTESIAN_POINT ( 'NONE',  ( 83.73300642799732429, 41.31124303260040875, -2.428015798050618734 ) ) ;
#73654=ADVANCED_FACE ( 'NONE', ( #28755 ), #39350, .T. ) ;
#73677=CARTESIAN_POINT ( 'NONE',  ( 79.25704083171595471, 59.98661423191555286, -16.48971415753125314 ) ) ;
#73680=CARTESIAN_POINT ( 'NONE',  ( 72.97045661744296297, 70.75163901906789476, -7.462049238873905033 ) ) ;
#73686=CARTESIAN_POINT ( 'NONE',  ( 69.80643203780810779, 69.29736018695484745, 6.650341497908645039 ) ) ;
#73692=CARTESIAN_POINT ( 'NONE',  ( 17.33597792084844258, 30.98502408145592213, -5.678558825948271327 ) ) ;
#73693=CARTESIAN_POINT ( 'NONE',  ( 74.70717368071740339, 67.14741735073857853, 12.46980216122492990 ) ) ;
#73697=CARTESIAN_POINT ( 'NONE',  ( 75.22447641198338886, 66.97122069168695191, 13.23119059164781852 ) ) ;
#73699=VERTEX_POINT ( 'NONE', #40817 ) ;
#73706=CARTESIAN_POINT ( 'NONE',  ( 81.53672410393728853, 56.04530558232496418, -16.40539795406885304 ) ) ;
#73708=CARTESIAN_POINT ( 'NONE',  ( 69.03448990137108865, 67.04097112400465619, 9.310083799442864461 ) ) ;
#73710=CARTESIAN_POINT ( 'NONE',  ( 82.90096945690618213, 41.76309762099524647, 4.006682518572778129 ) ) ;
#73711=CARTESIAN_POINT ( 'NONE',  ( 80.52421224103476050, 57.15337481666037434, 16.20884293195102899 ) ) ;
#73714=CARTESIAN_POINT ( 'NONE',  ( 70.52245475048280809, 71.40325566580152383, 0.2397668356339602846 ) ) ;
#73716=ORIENTED_EDGE ( 'NONE', *, *, #10976, .F. ) ;
#73717=CARTESIAN_POINT ( 'NONE',  ( 3.720166145283430925, 25.08080186712590276, -3.090169943749475845 ) ) ;
#73724=ORIENTED_EDGE ( 'NONE', *, *, #73279, .T. ) ;
#73725=CARTESIAN_POINT ( 'NONE',  ( 79.03265986744987970, 60.09179323390554117, 16.12040655615884077 ) ) ;
#73726=DIRECTION ( 'NONE',  ( 0.2347357813929421555, -0.4065742997269585213, 0.8829475928589297640 ) ) ;
#73727=CARTESIAN_POINT ( 'NONE',  ( 75.37843707191279918, 53.50823561223473490, 16.04097401286667335 ) ) ;
#73730=CARTESIAN_POINT ( 'NONE',  ( 78.99320801705290762, 51.70865386193722202, -15.35962929047159520 ) ) ;
#73739=CARTESIAN_POINT ( 'NONE',  ( 75.53649560587535916, 61.34551538626548250, 15.39653084909254233 ) ) ;
#73743=CARTESIAN_POINT ( 'NONE',  ( 82.20918741961230580, 40.63530303777752550, 3.361810051138397704 ) ) ;
#73744=CARTESIAN_POINT ( 'NONE',  ( 80.97755617445423582, 43.68821843711276642, -9.544220554497766074 ) ) ;
#73750=CARTESIAN_POINT ( 'NONE',  ( 70.96527508345572244, 61.11905909413832205, -14.48497578840443900 ) ) ;
#73752=CARTESIAN_POINT ( 'NONE',  ( 8.149503075528279794, 26.74646525600388358, 2.839279412974139660 ) ) ;
#73756=CARTESIAN_POINT ( 'NONE',  ( 85.53665298850141596, 48.34007191699684114, -12.21196891364052739 ) ) ;
#73761=CARTESIAN_POINT ( 'NONE',  ( 76.27279963928798168, 65.10967569403835853, -14.21370627898815542 ) ) ;
#73763=CARTESIAN_POINT ( 'NONE',  ( 84.18008060907449419, 49.39655662477972697, -13.52276195833983508 ) ) ;
#73766=CARTESIAN_POINT ( 'NONE',  ( 86.09437418083463456, 43.42260935030300573, 3.587124466458941008 ) ) ;
#73767=CARTESIAN_POINT ( 'NONE',  ( 88.26279489949382651, 43.89118386701247942, -2.126167786569203244 ) ) ;
#73768=ORIENTED_EDGE ( 'NONE', *, *, #15466, .T. ) ;
#73770=CARTESIAN_POINT ( 'NONE',  ( 65.75918626998540617, 69.09342105489017172, 0.05498200154574946208 ) ) ;
#73780=CARTESIAN_POINT ( 'NONE',  ( 87.96634291186354915, 44.23737611247270252, 2.817315086374476252 ) ) ;
#73783=CARTESIAN_POINT ( 'NONE',  ( 73.21090299573339166, 62.05059075953648318, -14.66927370496624228 ) ) ;
#73785=CARTESIAN_POINT ( 'NONE',  ( 73.90979809287503599, 65.40799970079461900, -13.26813225058578460 ) ) ;
#73786=CARTESIAN_POINT ( 'NONE',  ( 6.802937163926562114, 15.87878583063839066, -9.188101187500006262 ) ) ;
#73789=FACE_OUTER_BOUND ( 'NONE', #12827, .T. ) ;
#73800=CARTESIAN_POINT ( 'NONE',  ( 85.05760017557965114, 49.81609225799626017, 13.45342997944402796 ) ) ;
#73806=CARTESIAN_POINT ( 'NONE',  ( 72.64192451535615191, 57.19042016050428145, 15.87647339435071103 ) ) ;
#73815=CARTESIAN_POINT ( 'NONE',  ( 36.75658403392715456, 24.14754757982092315, -5.678558825948275768 ) ) ;
#73818=ORIENTED_EDGE ( 'NONE', *, *, #62888, .T. ) ;
#73819=CARTESIAN_POINT ( 'NONE',  ( 30.02984208470827454, 19.19860640527293327, 2.839279412974134775 ) ) ;
#73824=EDGE_CURVE ( 'NONE', #24668, #44579, #1854, .T. ) ;
#73827=CARTESIAN_POINT ( 'NONE',  ( 86.13530110067358692, 47.09369226531615737, 10.77952153921811096 ) ) ;
#73828=CARTESIAN_POINT ( 'NONE',  ( 74.80446345125277219, 64.37471161530348240, 14.55526155763435447 ) ) ;
#73830=CARTESIAN_POINT ( 'NONE',  ( 87.37434817825219113, 45.00237579746140426, -6.140289852623291189 ) ) ;
#73833=CARTESIAN_POINT ( 'NONE',  ( 74.92984376288937653, 53.18925172189641160, 16.51450970368439997 ) ) ;
#73836=ORIENTED_EDGE ( 'NONE', *, *, #1249, .T. ) ;
#73838=CARTESIAN_POINT ( 'NONE',  ( 66.04055754153552016, 68.56503372374930905, 4.418449956977249293 ) ) ;
#73840=ORIENTED_EDGE ( 'NONE', *, *, #351, .F. ) ;
#73841=CARTESIAN_POINT ( 'NONE',  ( 85.60299542505936188, 42.69774087082240754, 0.4164213344292336805 ) ) ;
#73846=CARTESIAN_POINT ( 'NONE',  ( 87.96405694255219032, 44.24133552746449283, -4.384643187820144838 ) ) ;
#73849=CARTESIAN_POINT ( 'NONE',  ( 38.53854167689037524, 24.11110640527295246, -2.839279412974138328 ) ) ;
#73851=CARTESIAN_POINT ( 'NONE',  ( 77.16999198201305887, 59.24405183509369266, -16.02415114386362305 ) ) ;
#73858=DIRECTION ( 'NONE',  ( -0.5000000000000014433, 0.8660254037844378194, 0.000000000000000000 ) ) ;
#73861=CARTESIAN_POINT ( 'NONE',  ( 85.70666193128211319, 48.42516261524464483, -11.73486726784230072 ) ) ;
#73862=CARTESIAN_POINT ( 'NONE',  ( 66.11687220234264828, 68.50194426514640611, -2.649008205479342237 ) ) ;
#73864=CARTESIAN_POINT ( 'NONE',  ( 81.88814419999580707, 58.88989235143515799, 0.4045084971874752799 ) ) ;
#73870=CARTESIAN_POINT ( 'NONE',  ( 73.97539535980833136, 55.64209510402770320, -16.58538844966203385 ) ) ;
#73875=CARTESIAN_POINT ( 'NONE',  ( 86.92624412656546440, 45.88388850009498299, -8.154586621708650895 ) ) ;
#73884=VERTEX_POINT ( 'NONE', #79392 ) ;
#73890=CARTESIAN_POINT ( 'NONE',  ( 30.01653393904200584, 17.73415679381823296, -6.890680421881970419E-14 ) ) ;
#73894=CARTESIAN_POINT ( 'NONE',  ( 69.61542750543651437, 62.56132062526208415, -13.94275833713536628 ) ) ;
#73899=ADVANCED_FACE ( 'NONE', ( #3371 ), #12454, .T. ) ;
#73901=CARTESIAN_POINT ( 'NONE',  ( 81.98093041017179416, 40.98279097121832137, -3.023795677445690000 ) ) ;
#73902=EDGE_CURVE ( 'NONE', #43596, #67223, #43325, .T. ) ;
#73910=CARTESIAN_POINT ( 'NONE',  ( 67.18400125431875836, 69.34949600813865800, -0.8641136148527382987 ) ) ;
#73915=AXIS2_PLACEMENT_3D ( 'NONE', #33006, #94845, #63907 ) ;
#73916=CARTESIAN_POINT ( 'NONE',  ( 73.68541970440786315, 69.64416370799906986, -9.598864117728750145 ) ) ;
#73919=CARTESIAN_POINT ( 'NONE',  ( 41.56734871454121816, 26.12755873383629535, -6.180339887498949025 ) ) ;
#73921=B_SPLINE_CURVE_WITH_KNOTS ( 'NONE', 3,
 ( #61627, #24634, #38826, #78358, #63638, #69234, #16038, #70738, #1349, #31715 ),
 .UNSPECIFIED., .F., .F.,
 ( 4, 2, 2, 2, 4 ),
 ( 0.000000000000000000, 0.2500000000000000000, 0.5000000000000000000, 0.7500000000000000000, 1.000000000000000000 ),
 .UNSPECIFIED. ) ;
#73924=CARTESIAN_POINT ( 'NONE',  ( 81.99434118348091260, 43.19859484614419642, -8.157555647291429679 ) ) ;
#73928=CARTESIAN_POINT ( 'NONE',  ( 86.95101435003084589, 46.48366829287757440, 8.967845595998873875 ) ) ;
#73930=CARTESIAN_POINT ( 'NONE',  ( 71.81881128194709163, 72.53313204687133009, -1.300380427722385823 ) ) ;
#73936=CARTESIAN_POINT ( 'NONE',  ( 4.836955906052805787, 24.83396525600387861, -2.839279412974133887 ) ) ;
#73942=EDGE_CURVE ( 'NONE', #59818, #50345, #4327, .T. ) ;
#73944=CARTESIAN_POINT ( 'NONE',  ( 81.95417956210631871, 41.06112128662814342, 3.409771386804488102 ) ) ;
#73945=CARTESIAN_POINT ( 'NONE',  ( 87.66109131259325693, 45.42289479680125908, -6.627856213955100273 ) ) ;
#73955=CARTESIAN_POINT ( 'NONE',  ( 67.33238274588912020, 67.23450051695161278, -8.593907957288223542 ) ) ;
#73960=CARTESIAN_POINT ( 'NONE',  ( 35.07444006175263240, 22.11110640527294535, -2.839279412974138328 ) ) ;
#73967=CARTESIAN_POINT ( 'NONE',  ( 9.333682440526761326, 28.49540643055185996, 3.479690158560446702E-15 ) ) ;
#73968=CARTESIAN_POINT ( 'NONE',  ( 21.97483017187327192, 36.18528772668518911, -1.583844403245363575 ) ) ;
#73973=CARTESIAN_POINT ( 'NONE',  ( 77.72205534048291042, 61.52847525230063042, 16.09962475150207339 ) ) ;
#73984=CARTESIAN_POINT ( 'NONE',  ( 66.13947098823611270, 69.16665220597090524, -2.048021925782174346 ) ) ;
#73987=CARTESIAN_POINT ( 'NONE',  ( 78.04817985968655591, 62.07294584189650521, -16.01854286150912898 ) ) ;
#73988=CARTESIAN_POINT ( 'NONE',  ( 72.10919973083444745, 72.28739807568710773, -1.448965806592429795 ) ) ;
#73993=EDGE_LOOP ( 'NONE', ( #92788, #1955, #76727, #11447 ) ) ;
#73997=CARTESIAN_POINT ( 'NONE',  ( 26.65419051621551461, 38.49540643055190259, 3.479690158560446702E-15 ) ) ;
#74000=CARTESIAN_POINT ( 'NONE',  ( 75.21170341390104852, 66.97160359861173617, -12.78114342037769013 ) ) ;
#74003=CARTESIAN_POINT ( 'NONE',  ( 81.62315923969183018, 55.76054528319124159, 16.35706999678057727 ) ) ;
#74007=ORIENTED_EDGE ( 'NONE', *, *, #87198, .F. ) ;
#74020=DIRECTION ( 'NONE',  ( 0.6355427771210591104, 0.000000000000000000, 0.7720656568254100627 ) ) ;
#74025=CARTESIAN_POINT ( 'NONE',  ( 85.24313230617720194, 44.17383514321656435, -6.788908311595864831 ) ) ;
#74029=CARTESIAN_POINT ( 'NONE',  ( 74.74991615466120720, 60.94473038293241274, 15.38198754237874688 ) ) ;
#74032=CARTESIAN_POINT ( 'NONE',  ( 76.94944781827869917, 56.99682769027370455, 16.18096124992289120 ) ) ;
#74044=CARTESIAN_POINT ( 'NONE',  ( 18.71539827744147999, 26.50829794293879615, -10.00000000000000355 ) ) ;
#74060=CARTESIAN_POINT ( 'NONE',  ( 17.15438521794160920, 32.83705186507754092, 3.090169943749475401 ) ) ;
#74061=CARTESIAN_POINT ( 'NONE',  ( 85.48911027617603509, 49.06452166842702667, 12.33247222509585228 ) ) ;
#74062=AXIS2_PLACEMENT_3D ( 'NONE', #64275, #25792, #56668 ) ;
#74064=FACE_OUTER_BOUND ( 'NONE', #99533, .T. ) ;
#74065=CARTESIAN_POINT ( 'NONE',  ( 73.75633218949143100, 55.22183339029175642, -16.59646955798544354 ) ) ;
#74068=CARTESIAN_POINT ( 'NONE',  ( 76.86551199909389709, 60.02806529646827016, 16.29612583600000875 ) ) ;
#74078=CARTESIAN_POINT ( 'NONE',  ( 31.70236382085744609, 33.70171378149921537, -9.188101187500004485 ) ) ;
#74079=B_SPLINE_CURVE_WITH_KNOTS ( 'NONE', 3,
 ( #47200, #15798, #85253, #53787, #69997, #47692, #23899, #63906, #46704, #77630, #612, #78124, #70502, #8214, #39084, #61891, #94349, #40592, #31494, #78627, #38600, #62386, #55287, #71031, #7707, #46185, #48210, #1633, #33005, #93343, #2123, #22901, #84748, #15288, #8712, #1117, #77104, #32517, #79156, #63410, #39581, #24903, #93856, #31994, #69504, #54801 ),
 .UNSPECIFIED., .F., .F.,
 ( 4, 1, 1, 1, 2, 2, 1, 1, 1, 2, 2, 1, 1, 2, 2, 1, 1, 2, 2, 1, 1, 2, 2, 1, 2, 2, 1, 2, 2, 4 ),
 ( 0.000000000000000000, 0.06249999999998294420, 0.09374999999997277178, 0.1093749999999694966, 0.1171874999999694411, 0.1249999999999693578, 0.1874999999999802103, 0.2187499999999858724, 0.2343749999999902023, 0.2421874999999925893, 0.2499999999999950040, 0.3125000000000006106, 0.3437500000000021094, 0.3593750000000013878, 0.3750000000000006661, 0.4374999999999905631, 0.4687499999999855671, 0.4843749999999844014, 0.4999999999999832356, 0.5624999999999895639, 0.5937499999999904521, 0.6093749999999907851, 0.6249999999999912292, 0.6874999999999906741, 0.7187499999999904521, 0.7499999999999902300, 0.8124999999999934497, 0.8437499999999931166, 0.8749999999999927836, 1.000000000000000000 ),
 .UNSPECIFIED. ) ;
#74080=CARTESIAN_POINT ( 'NONE',  ( 27.68909066282341058, 16.39040679176984128, 1.333680081654574804E-15 ) ) ;
#74086=CARTESIAN_POINT ( 'NONE',  ( 15.18774714507562962, 26.95586893147754992, 7.433330006724141015 ) ) ;
#74087=CARTESIAN_POINT ( 'NONE',  ( 82.20091667785729328, 54.22338727706198114, 15.63590626746406009 ) ) ;
#74092=CARTESIAN_POINT ( 'NONE',  ( 75.02147862394267008, 53.42613012923004590, -16.05124535999422974 ) ) ;
#74093=CARTESIAN_POINT ( 'NONE',  ( 81.36599162659588558, 42.15504690410337929, 8.050126262897936869 ) ) ;
#74094=EDGE_CURVE ( 'NONE', #65992, #70878, #33972, .T. ) ;
#74098=CARTESIAN_POINT ( 'NONE',  ( 66.49005502223729991, 68.69345493094031951, 4.810109871286462280 ) ) ;
#74107=CARTESIAN_POINT ( 'NONE',  ( 88.02868988710136477, 43.76708177457258842, -2.199075477856099692 ) ) ;
#74109=CARTESIAN_POINT ( 'NONE',  ( 80.21108484470566680, 57.40951183915923650, -16.59077246605596301 ) ) ;
#74113=CARTESIAN_POINT ( 'NONE',  ( 81.49213971395570866, 49.47327963668817574, -13.93402821202839625 ) ) ;
#74116=CARTESIAN_POINT ( 'NONE',  ( 80.94772830529335295, 43.03073618849790449, 9.590346675963626666 ) ) ;
#74127=B_SPLINE_CURVE_WITH_KNOTS ( 'NONE', 3,
 ( #23421, #58201, #86297, #87318, #79684, #97241, #1657, #63439, #71056, #40619 ),
 .UNSPECIFIED., .F., .F.,
 ( 4, 2, 2, 2, 4 ),
 ( 0.000000000000000000, 0.0002622400424272996935, 0.0005244800848545993870, 0.0007867201272818990804, 0.001048960169709198774 ),
 .UNSPECIFIED. ) ;
#74131=AXIS2_PLACEMENT_3D ( 'NONE', #78929, #41891, #9518 ) ;
#74134=CARTESIAN_POINT ( 'NONE',  ( 87.53138335513271784, 43.77696556206725376, 0.8862036439340156280 ) ) ;
#74139=CARTESIAN_POINT ( 'NONE',  ( 4.698709606056801213, 26.21091486745858390, -1.111400068045478839E-16 ) ) ;
#74143=CARTESIAN_POINT ( 'NONE',  ( 75.70440440058339959, 57.47974519366773194, -16.09699729114145939 ) ) ;
#74144=CARTESIAN_POINT ( 'NONE',  ( 39.81344631580554250, 23.39040679176985904, -6.890680421881970419E-14 ) ) ;
#74145=CARTESIAN_POINT ( 'NONE',  ( 77.48815792355858889, 49.76915981755508511, -14.97591747096309689 ) ) ;
#74151=CARTESIAN_POINT ( 'NONE',  ( 69.33329605705168319, 62.86184331883654153, 13.67499948212078564 ) ) ;
#74154=CARTESIAN_POINT ( 'NONE',  ( 19.02883662497902861, 11.39040679176981996, 1.333680081654574804E-15 ) ) ;
#74174=CARTESIAN_POINT ( 'NONE',  ( 74.10605571268695257, 68.62492193873490010, 11.45106078344675637 ) ) ;
#74175=CARTESIAN_POINT ( 'NONE',  ( 74.46402575432118454, 68.25533967602589769, -11.46783318448646050 ) ) ;
#74181=CARTESIAN_POINT ( 'NONE',  ( 3.893371226040319044, 25.18080186712590773, 3.090169943749475401 ) ) ;
#74188=CARTESIAN_POINT ( 'NONE',  ( 79.01889296114717354, 59.41967273037256092, -16.52995258344893159 ) ) ;
#74196=CARTESIAN_POINT ( 'NONE',  ( 79.16919300666631898, 46.29637006420016121, -12.78014982653817810 ) ) ;
#74198=CARTESIAN_POINT ( 'NONE',  ( 73.25535670630372920, 69.88482930906741331, 9.609716971570463784 ) ) ;
#74202=CARTESIAN_POINT ( 'NONE',  ( 69.70345325596831287, 69.13798228350341901, 6.832978093666964625 ) ) ;
#74207=PLANE ( 'NONE',  #12635 ) ;
#74209=CARTESIAN_POINT ( 'NONE',  ( 21.14648969749996610, 33.18502408145591431, 5.678558825948277544 ) ) ;
#74211=CARTESIAN_POINT ( 'NONE',  ( 83.82917762730355093, 51.97629592023758249, -14.94018958758825022 ) ) ;
#74216=CARTESIAN_POINT ( 'NONE',  ( 68.45344762038320141, 64.57392882354749020, 12.12708197217120798 ) ) ;
#74225=CARTESIAN_POINT ( 'NONE',  ( 69.39669185256211392, 67.72053295272533546, 8.719490259099096363 ) ) ;
#74228=CARTESIAN_POINT ( 'NONE',  ( 85.18722491056296064, 44.62996190128500018, 7.606051790527071255 ) ) ;
#74231=EDGE_CURVE ( 'NONE', #54612, #44705, #53902, .T. ) ;
#74232=CARTESIAN_POINT ( 'NONE',  ( 69.83738656355549779, 70.92545396396145918, 1.304034296880247412 ) ) ;
#74237=CARTESIAN_POINT ( 'NONE',  ( 10.89475974595093000, 11.45404122711131478, -8.090169943749478065 ) ) ;
#74238=CARTESIAN_POINT ( 'NONE',  ( 82.93658845200469898, 45.09976895464361490, 10.63726503173775484 ) ) ;
#74241=EDGE_CURVE ( 'NONE', #47030, #54902, #3250, .T. ) ;
#74242=CARTESIAN_POINT ( 'NONE',  ( 86.52685127962818967, 47.39493317473652212, -10.85533565734823824 ) ) ;
#74246=CARTESIAN_POINT ( 'NONE',  ( 67.15772368909350121, 67.74692886573922124, -6.548511843863573212 ) ) ;
#74253=CARTESIAN_POINT ( 'NONE',  ( 81.23970239364686563, 42.24692268292314168, -7.309682766412492150 ) ) ;
#74266=CARTESIAN_POINT ( 'NONE',  ( 82.15776938016838926, 40.64327202660170713, 3.515950796866609718 ) ) ;
#74267=CARTESIAN_POINT ( 'NONE',  ( 80.61131623575732874, 43.32435129898595960, -9.365491868763141881 ) ) ;
#74268=AXIS2_PLACEMENT_3D ( 'NONE', #72537, #77884, #23149 ) ;
#74276=CARTESIAN_POINT ( 'NONE',  ( 76.86366411620821282, 60.80910549659888886, 15.73837547318715480 ) ) ;
#74277=CARTESIAN_POINT ( 'NONE',  ( 15.64721481668148328, 11.96004757982088940, -5.678558825948276656 ) ) ;
#74283=EDGE_LOOP ( 'NONE', ( #42990, #61978, #67384, #93847 ) ) ;
#74287=CARTESIAN_POINT ( 'NONE',  ( 82.75883821533659557, 49.82052486449969564, -14.21782099992554116 ) ) ;
#74291=AXIS2_PLACEMENT_3D ( 'NONE', #4071, #34961, #66372 ) ;
#74294=CARTESIAN_POINT ( 'NONE',  ( 65.98410341620582642, 69.22083730553454473, 0.2678598787953536675 ) ) ;
#74299=CARTESIAN_POINT ( 'NONE',  ( 81.88567891057422798, 44.78205882872802590, -10.20763061476163536 ) ) ;
#74302=CARTESIAN_POINT ( 'NONE',  ( 79.14312167556931854, 57.64441083166269664, 0.000000000000000000 ) ) ;
#74303=CARTESIAN_POINT ( 'NONE',  ( 88.06349342987242323, 44.28914147295815695, 2.792731503129179504 ) ) ;
#74310=CARTESIAN_POINT ( 'NONE',  ( 80.31495243796621253, 58.05602015539035676, 16.26171843954676177 ) ) ;
#74311=CARTESIAN_POINT ( 'NONE',  ( 85.74709191876297609, 48.50741248266042049, -11.78150043536521174 ) ) ;
#74313=CARTESIAN_POINT ( 'NONE',  ( 80.82785412337717901, 42.97997768494945348, -9.612963753214643248 ) ) ;
#74317=CARTESIAN_POINT ( 'NONE',  ( 87.87366831029828518, 44.19753277059973584, -4.411077605820556968 ) ) ;
#74319=CARTESIAN_POINT ( 'NONE',  ( 78.14971419250070994, 52.01379824954777575, 15.54497553320235248 ) ) ;
#74320=CARTESIAN_POINT ( 'NONE',  ( 76.25499879835211914, 51.34390249587517019, 15.62284479604242549 ) ) ;
#74323=CARTESIAN_POINT ( 'NONE',  ( 84.46805331009542783, 50.67741563211675526, 13.74683494288181507 ) ) ;
#74329=CARTESIAN_POINT ( 'NONE',  ( 8.146472837920740062, 20.10171378149916777, 9.188101187500008038 ) ) ;
#74337=CARTESIAN_POINT ( 'NONE',  ( 80.46653820500203835, 44.39910589696482646, 11.34020455946100370 ) ) ;
#74338=CARTESIAN_POINT ( 'NONE',  ( 33.97448420766330202, 31.56628583063843152, 9.188101187500006262 ) ) ;
#74342=CARTESIAN_POINT ( 'NONE',  ( 20.59861825492957621, 33.93396525600390845, 2.839279412974139660 ) ) ;
#74349=CARTESIAN_POINT ( 'NONE',  ( 70.51412929403316809, 60.93737776118788929, 14.98137441988405705 ) ) ;
#74355=CARTESIAN_POINT ( 'NONE',  ( 87.40330451559304947, 45.01222676107010301, -6.126549417040136447 ) ) ;
#74358=CARTESIAN_POINT ( 'NONE',  ( 75.36158518500756998, 53.45249184671629905, 16.03634573857044288 ) ) ;
#74360=CARTESIAN_POINT ( 'NONE',  ( 72.00273082287530713, 68.45064935962042796, 10.42463711869592657 ) ) ;
#74366=ORIENTED_EDGE ( 'NONE', *, *, #2725, .F. ) ;
#74367=CARTESIAN_POINT ( 'NONE',  ( 77.31168512783449387, 63.18411157796573008, -15.22841949698756459 ) ) ;
#74373=CARTESIAN_POINT ( 'NONE',  ( 84.06604358195920668, 51.46910565605918464, 14.65639964578790710 ) ) ;
#74375=CARTESIAN_POINT ( 'NONE',  ( 38.84587710395076954, 34.37878583063844218, 9.188101187500006262 ) ) ;
#74377=CARTESIAN_POINT ( 'NONE',  ( 87.35606880162971777, 45.77061481740688009, 8.290963297571636303 ) ) ;
#74384=CARTESIAN_POINT ( 'NONE',  ( 85.59998877908455484, 48.66343243370425142, 12.43629469118824638 ) ) ;
#74387=CARTESIAN_POINT ( 'NONE',  ( 82.33791607580600669, 40.35809408978042967, 1.142683882547790519 ) ) ;
#74398=CARTESIAN_POINT ( 'NONE',  ( 71.96307967416730378, 59.12692550662651314, 15.37583765050489859 ) ) ;
#74403=ORIENTED_EDGE ( 'NONE', *, *, #46504, .F. ) ;
#74407=B_SPLINE_CURVE_WITH_KNOTS ( 'NONE', 3,
 ( #70273, #17076, #39853, #16081, #8489, #63181, #86054, #39359, #32277, #79928, #94124, #95133, #56578, #16579, #56058, #86545, #47477, #31763, #24678, #2916, #17586, #8982, #18094, #40860, #62667, #70788, #9498, #1397, #47966, #40364, #85539, #32775, #94620, #25178, #87051, #71807, #10488, #2403, #25698, #26191, #41369, #72307, #33808, #64692, #95644, #81922 ),
 .UNSPECIFIED., .F., .F.,
 ( 4, 1, 2, 2, 1, 2, 2, 1, 1, 2, 2, 1, 1, 2, 2, 1, 1, 2, 2, 1, 1, 1, 2, 2, 1, 1, 1, 2, 2, 4 ),
 ( 0.000000000000000000, 0.06250000000000142941, 0.09375000000000123512, 0.1250000000000010547, 0.1874999999999988898, 0.2187499999999966693, 0.2499999999999944489, 0.3124999999999933387, 0.3437499999999927836, 0.3593749999999907851, 0.3749999999999887867, 0.4374999999999796829, 0.4687499999999751310, 0.4843749999999724110, 0.4999999999999696354, 0.5624999999999605871, 0.5937499999999549249, 0.6093749999999518163, 0.6249999999999485967, 0.6874999999999394928, 0.7187499999999349409, 0.7343749999999334976, 0.7421874999999338307, 0.7499999999999340528, 0.8124999999999359401, 0.8437499999999379385, 0.8593749999999398259, 0.8671874999999427125, 0.8749999999999454880, 1.000000000000000000 ),
 .UNSPECIFIED. ) ;
#74411=CARTESIAN_POINT ( 'NONE',  ( 83.89386139451886493, 49.22207443597933008, 13.04948611042680540 ) ) ;
#74413=CARTESIAN_POINT ( 'NONE',  ( 69.41166179968418248, 62.72696118611258242, -13.78096777156330077 ) ) ;
#74421=FACE_OUTER_BOUND ( 'NONE', #97090, .T. ) ;
#74425=CARTESIAN_POINT ( 'NONE',  ( 80.25206473404905694, 51.20499363921007330, 14.98319710954680417 ) ) ;
#74429=CARTESIAN_POINT ( 'NONE',  ( 77.62454426129153262, 61.88953154547135682, 15.65088405748084988 ) ) ;
#74432=CARTESIAN_POINT ( 'NONE',  ( 66.64574440031255165, 67.65126300000102333, 6.155624976568763174 ) ) ;
#74435=CARTESIAN_POINT ( 'NONE',  ( 73.55996738445699634, 69.73057641899073644, -9.398744228737333728 ) ) ;
#74438=CARTESIAN_POINT ( 'NONE',  ( 37.37984742713354791, 29.78052372038643369, -10.00000000000000355 ) ) ;
#74439=CARTESIAN_POINT ( 'NONE',  ( 77.47571766935273274, 57.04508641376936851, -16.61716333516349664 ) ) ;
#74446=CARTESIAN_POINT ( 'NONE',  ( 86.80277191894818145, 46.47277518407399555, 9.069725256793763180 ) ) ;
#74449=CARTESIAN_POINT ( 'NONE',  ( 71.95078207959971905, 72.63412948483367870, -0.9918729297793668076 ) ) ;
#74451=CARTESIAN_POINT ( 'NONE',  ( 87.36774593059779193, 45.94567951850589083, 8.539250186115692642 ) ) ;
#74454=CARTESIAN_POINT ( 'NONE',  ( 41.28778705816291961, 32.03677371833806120, 10.00000000000000533 ) ) ;
#74459=CARTESIAN_POINT ( 'NONE',  ( 70.96446909585041851, 67.83507693878627265, -9.741514685561401876 ) ) ;
#74462=CARTESIAN_POINT ( 'NONE',  ( 74.19247292150758710, 57.10187714277506643, -16.01396260610887268 ) ) ;
#74465=DIRECTION ( 'NONE',  ( 0.5000000000000014433, -0.8660254037844378194, 0.000000000000000000 ) ) ;
#74479=CARTESIAN_POINT ( 'NONE',  ( 24.92213970864663963, 37.49540643055189548, 3.479690158560446702E-15 ) ) ;
#74481=CARTESIAN_POINT ( 'NONE',  ( 86.12135434523638366, 46.98046262810483142, -10.13131473785488090 ) ) ;
#74484=CARTESIAN_POINT ( 'NONE',  ( 21.59269996301512506, 13.26216523072493914, -2.296566073217252530E-15 ) ) ;
#74486=CARTESIAN_POINT ( 'NONE',  ( 67.70878694032322187, 69.48726129358172443, -2.441691297528492566 ) ) ;
#74498=CARTESIAN_POINT ( 'NONE',  ( 66.28959039141291498, 69.23996339252364862, -2.139077115682002983 ) ) ;
#74501=CARTESIAN_POINT ( 'NONE',  ( 78.32598375782600897, 61.10224562959768235, -15.90800848020992220 ) ) ;
#74504=LINE ( 'NONE', #42558, #86810 ) ;
#74508=ORIENTED_EDGE ( 'NONE', *, *, #99046, .T. ) ;
#74514=CARTESIAN_POINT ( 'NONE',  ( 80.55977923466276991, 44.53388773495298381, 11.41474457630165062 ) ) ;
#74516=CARTESIAN_POINT ( 'NONE',  ( 87.57478309584621456, 45.08285526713720515, 6.924932389716528469 ) ) ;
#74517=ORIENTED_EDGE ( 'NONE', *, *, #31039, .F. ) ;
#74518=CARTESIAN_POINT ( 'NONE',  ( 72.36414345318156904, 63.72805025348669972, -13.64787615739589555 ) ) ;
#74519=CARTESIAN_POINT ( 'NONE',  ( 86.82688353415350946, 43.55230325865861829, -2.297822768102545599 ) ) ;
#74523=CARTESIAN_POINT ( 'NONE',  ( 86.70911053808110580, 46.89117940024963360, 10.21290512048939547 ) ) ;
#74524=CARTESIAN_POINT ( 'NONE',  ( 76.10495001321383768, 51.13391335127094095, -16.08818559945424198 ) ) ;
#74539=CARTESIAN_POINT ( 'NONE',  ( 74.77989834281638082, 61.09922272559126100, 15.34499820422063010 ) ) ;
#74542=CARTESIAN_POINT ( 'NONE',  ( 77.37106971737360084, 59.79005663912887059, 15.99722322042923928 ) ) ;
#74555=CARTESIAN_POINT ( 'NONE',  ( 16.27523747222386774, 28.13478043621388025, 8.090169943749478065 ) ) ;
#74556=EDGE_CURVE ( 'NONE', #87380, #92014, #16298, .T. ) ;
#74559=CARTESIAN_POINT ( 'NONE',  ( 26.50804481403195467, 15.70852965304480087, 1.583844403245364907 ) ) ;
#74561=CARTESIAN_POINT ( 'NONE',  ( 72.13721715224981779, 71.83272178494776483, -3.912550702485382281 ) ) ;
#74564=ORIENTED_EDGE ( 'NONE', *, *, #6401, .F. ) ;
#74570=CARTESIAN_POINT ( 'NONE',  ( 19.47506710560450571, 33.01751292744055633, 6.180339887498949913 ) ) ;
#74571=LINE ( 'NONE', #5149, #75628 ) ;
#74577=CARTESIAN_POINT ( 'NONE',  ( 75.26053270681407525, 66.77963801587817727, 12.92466396265848871 ) ) ;
#74586=EDGE_CURVE ( 'NONE', #29855, #88281, #56160, .T. ) ;
#74587=CARTESIAN_POINT ( 'NONE',  ( 44.43411998782967487, 26.44966523072497822, -2.296566073217252530E-15 ) ) ;
#74591=CARTESIAN_POINT ( 'NONE',  ( 24.15577373785222193, 19.11029122506294797, -8.090169943749478065 ) ) ;
#74597=CARTESIAN_POINT ( 'NONE',  ( 11.61360469066603507, 28.74646525600389069, 2.839279412974139660 ) ) ;
#74598=CARTESIAN_POINT ( 'NONE',  ( 71.92952260767447115, 72.55458961131337503, 1.705568256100836066 ) ) ;
#74607=CARTESIAN_POINT ( 'NONE',  ( 81.10605299805037305, 42.47174888764966738, 7.802073681796036553 ) ) ;
#74612=CARTESIAN_POINT ( 'NONE',  ( 66.77373092297933965, 68.40140739384713697, 4.464727344145090981 ) ) ;
#74621=CARTESIAN_POINT ( 'NONE',  ( 80.19807517511665651, 58.11859141470634427, 16.26539701942824578 ) ) ;
#74625=CARTESIAN_POINT ( 'NONE',  ( 80.74266887835153739, 43.44699442419332769, 9.418154823084309513 ) ) ;
#74629=ORIENTED_EDGE ( 'NONE', *, *, #15630, .T. ) ;
#74639=CARTESIAN_POINT ( 'NONE',  ( 79.09745926769026880, 51.74933575859580515, -15.81631569581207941 ) ) ;
#74648=CARTESIAN_POINT ( 'NONE',  ( 78.69766452942040758, 56.36335943523778269, -16.19347606039230669 ) ) ;
#74649=CARTESIAN_POINT ( 'NONE',  ( 39.85783382567782951, 23.41603393254329291, -1.583844403245396437 ) ) ;
#74655=CARTESIAN_POINT ( 'NONE',  ( 71.88093039901364989, 69.29925688614676460, 8.664886389715691806 ) ) ;
#74661=ORIENTED_EDGE ( 'NONE', *, *, #12679, .T. ) ;
#74674=CARTESIAN_POINT ( 'NONE',  ( 82.66777534753497036, 40.88273136530058594, 3.288167606880417981 ) ) ;
#74678=CARTESIAN_POINT ( 'NONE',  ( 74.09798493915437234, 67.86634104065885253, -11.62737576625272418 ) ) ;
#74683=CARTESIAN_POINT ( 'NONE',  ( 81.65711888479437164, 41.53726941426280206, -5.387001511484587724 ) ) ;
#74693=CARTESIAN_POINT ( 'NONE',  ( 3.124773676633713748, 24.73705186507751463, -3.090169943749475845 ) ) ;
#74695=FACE_OUTER_BOUND ( 'NONE', #19928, .T. ) ;
#74696=CARTESIAN_POINT ( 'NONE',  ( 73.63435323750927353, 69.71791780730768551, 10.06421556446032461 ) ) ;
#74700=CARTESIAN_POINT ( 'NONE',  ( 68.57836030477737665, 67.22337045858328963, 8.752937159126823019 ) ) ;
#74701=CARTESIAN_POINT ( 'NONE',  ( 66.11933821713674320, 68.48733517449421981, -4.787403750998837637 ) ) ;
#74704=EDGE_CURVE ( 'NONE', #78719, #96205, #28385, .T. ) ;
#74707=CARTESIAN_POINT ( 'NONE',  ( 84.80475637890920382, 46.66516897523420937, 11.11621779752075945 ) ) ;
#74709=CARTESIAN_POINT ( 'NONE',  ( 32.30976433484754295, 19.44966523072496045, -2.296566073217252530E-15 ) ) ;
#74711=CARTESIAN_POINT ( 'NONE',  ( 83.42542119994750749, 51.64995580955420706, -14.90072893730332027 ) ) ;
#74714=CARTESIAN_POINT ( 'NONE',  ( 74.99160476570628475, 67.13646269190913074, 13.03024426091169019 ) ) ;
#74716=CARTESIAN_POINT ( 'NONE',  ( 68.43300413790026937, 64.44848761198993259, 12.21846621112735853 ) ) ;
#74721=DIRECTION ( 'NONE',  ( 0.5000000000000014433, -0.8660254037844378194, 0.000000000000000000 ) ) ;
#74722=CARTESIAN_POINT ( 'NONE',  ( 12.70933400901951416, 9.198606405272903075, 2.839279412974134775 ) ) ;
#74723=VERTEX_POINT ( 'NONE', #35492 ) ;
#74724=CARTESIAN_POINT ( 'NONE',  ( 70.64415969017909447, 69.81928975612606791, 6.580201901691414612 ) ) ;
#74725=CARTESIAN_POINT ( 'NONE',  ( 83.67528194178203194, 41.54745686406482008, -3.633279836990721989 ) ) ;
#74727=CARTESIAN_POINT ( 'NONE',  ( 84.53232711715837411, 43.64540581557137955, 6.477393172473421501 ) ) ;
#74730=CARTESIAN_POINT ( 'NONE',  ( 68.54312381459287451, 69.80873064283493079, 3.292911436909311096 ) ) ;
#74732=CARTESIAN_POINT ( 'NONE',  ( 72.58111491857235364, 57.29791513365444189, -16.33754921798919213 ) ) ;
#74734=CARTESIAN_POINT ( 'NONE',  ( 19.05068821614581864, 13.12755873383625449, -6.180339887498949025 ) ) ;
#74735=CARTESIAN_POINT ( 'NONE',  ( 82.09686517919956827, 43.36415878988843531, 9.196185934937616935 ) ) ;
#74737=CARTESIAN_POINT ( 'NONE',  ( 74.09260619880180343, 55.08812674012290245, 16.60422476838407846 ) ) ;
#74738=CARTESIAN_POINT ( 'NONE',  ( 86.30773806088525646, 46.95517243064260526, -10.53307507464018755 ) ) ;
#74754=CARTESIAN_POINT ( 'NONE',  ( 80.52412688334953828, 46.96905098241762744, 12.74129133586520091 ) ) ;
#74756=CARTESIAN_POINT ( 'NONE',  ( 75.08869305417201190, 59.14893459762363648, 15.81684554694788503 ) ) ;
#74760=CARTESIAN_POINT ( 'NONE',  ( 82.41914487369291464, 41.31337197830497132, 3.340431838514233753 ) ) ;
#74762=LINE ( 'NONE', #28130, #67301 ) ;
#74763=EDGE_CURVE ( 'NONE', #27651, #85116, #79184, .T. ) ;
#74765=CARTESIAN_POINT ( 'NONE',  ( 76.61888230025124358, 51.35972145274618583, 16.07233720520855158 ) ) ;
#74768=CARTESIAN_POINT ( 'NONE',  ( 76.07649505321222705, 56.58890100330362571, 16.14652101205965806 ) ) ;
#74769=CARTESIAN_POINT ( 'NONE',  ( 11.83670304002995266, 9.760047579820874120, 5.678558825948272215 ) ) ;
#74781=FACE_OUTER_BOUND ( 'NONE', #55391, .T. ) ;
#74784=CARTESIAN_POINT ( 'NONE',  ( 73.65583987803587718, 62.70152398185310716, -14.53858387021961107 ) ) ;
#74785=ORIENTED_EDGE ( 'NONE', *, *, #84398, .T. ) ;
#74791=CARTESIAN_POINT ( 'NONE',  ( 83.95136718548498322, 44.65165793737095612, -8.662646615273729367 ) ) ;
#74794=CARTESIAN_POINT ( 'NONE',  ( 88.25905654664580879, 44.35750191947202126, 2.523739344444579480 ) ) ;
#74799=CARTESIAN_POINT ( 'NONE',  ( 80.37423141194477694, 58.00578747994902074, 16.25890986437170938 ) ) ;
#74801=CARTESIAN_POINT ( 'NONE',  ( 85.55579313808955533, 48.95319673495580304, -12.20343581778852915 ) ) ;
#74805=CARTESIAN_POINT ( 'NONE',  ( 69.50667547386485978, 68.39943198049301998, 8.745776950494660085 ) ) ;
#74809=CARTESIAN_POINT ( 'NONE',  ( 87.81919554331292943, 44.17710153608190637, -4.445631852975253651 ) ) ;
#74811=CARTESIAN_POINT ( 'NONE',  ( 79.03035308903145051, 56.41680147193460471, 16.17228969028650454 ) ) ;
#74814=CARTESIAN_POINT ( 'NONE',  ( 79.11408761357685648, 53.92110988754666323, -15.85693396780485642 ) ) ;
#74815=DIRECTION ( 'NONE',  ( 0.3940053768033583426, -0.6824373310787393843, 0.6156614753256619554 ) ) ;
#74818=CARTESIAN_POINT ( 'NONE',  ( 84.73763152763326900, 50.49395269109753315, 13.54719052834833093 ) ) ;
#74826=CARTESIAN_POINT ( 'NONE',  ( 6.569006713621681648, 25.83396525600388216, -2.839279412974133887 ) ) ;
#74834=CARTESIAN_POINT ( 'NONE',  ( 34.65648599653719941, 40.98502408145595410, -5.678558825948271327 ) ) ;
#74838=CARTESIAN_POINT ( 'NONE',  ( 26.97531487256933858, 21.28920272979927830, -7.433330006724141015 ) ) ;
#74839=CARTESIAN_POINT ( 'NONE',  ( 6.475147923497964086, 27.23654200823201066, 1.583844403245363353 ) ) ;
#74843=CARTESIAN_POINT ( 'NONE',  ( 70.99909089399695006, 61.09348569631758608, 14.50421621802051675 ) ) ;
#74844=CARTESIAN_POINT ( 'NONE',  ( 75.75493378409400691, 65.86437009324527025, -14.07593894684413804 ) ) ;
#74853=CARTESIAN_POINT ( 'NONE',  ( 81.82036482989325066, 42.35048943672428834, -7.944650131338358179 ) ) ;
#74862=EDGE_CURVE ( 'NONE', #76483, #78218, #10534, .T. ) ;
#74863=CARTESIAN_POINT ( 'NONE',  ( 32.94608582406294062, 39.99752408145594984, 5.678558825948276656 ) ) ;
#74867=ORIENTED_EDGE ( 'NONE', *, *, #41670, .F. ) ;
#74869=CARTESIAN_POINT ( 'NONE',  ( 87.08174047714162214, 46.31017841404310786, -9.261312696178791271 ) ) ;
#74874=CARTESIAN_POINT ( 'NONE',  ( 71.06528275231133307, 61.93773232536235440, -14.16138117441405520 ) ) ;
#74875=CARTESIAN_POINT ( 'NONE',  ( 82.34797793138363886, 40.36079106117341553, 1.103604957399969111 ) ) ;
#74877=CARTESIAN_POINT ( 'NONE',  ( 77.06991968482392963, 62.91017430212377093, -15.27451705560989126 ) ) ;
#74881=ORIENTED_EDGE ( 'NONE', *, *, #24790, .T. ) ;
#74882=AXIS2_PLACEMENT_3D ( 'NONE', #42876, #25727, #42390 ) ;
#74885=CARTESIAN_POINT ( 'NONE',  ( 87.15344218626839279, 46.31686449193668409, -8.569727620351585529 ) ) ;
#74886=B_SPLINE_SURFACE_WITH_KNOTS ( 'NONE', 3, 1, ( 
 ( #25447, #87824 ),
 ( #18363, #49258 ),
 ( #80702, #19864 ),
 ( #63946, #80194 ),
 ( #10762, #21344 ),
 ( #52720, #90292 ),
 ( #37032, #76065 ),
 ( #12259, #43117 ),
 ( #51228, #13261 ),
 ( #81686, #98360 ),
 ( #20862, #74061 ),
 ( #21835, #67940 ),
 ( #13735, #29931 ),
 ( #60808, #44615 ),
 ( #59827, #4650 ),
 ( #58820, #6645 ),
 ( #83680, #66930 ),
 ( #60312, #75058 ),
 ( #12767, #35543 ),
 ( #75550, #51753 ),
 ( #43632, #27938 ),
 ( #97860, #45127 ),
 ( #89782, #28431 ),
 ( #20358, #14241 ),
 ( #82196, #59313 ),
 ( #98861, #66444 ),
 ( #37520, #29438 ),
 ( #82695, #91768 ),
 ( #97372, #91270 ),
 ( #90792, #68425 ),
 ( #50731, #99353 ) ),
 .UNSPECIFIED., .F., .F., .F.,
 ( 4, 3, 3, 3, 3, 3, 3, 3, 3, 3, 4 ),
 ( 2, 2 ),
 ( 0.000000000000000000, 0.1333490885032305451, 0.3007194338854253246, 0.4699862290244986029, 0.5844252810809236198, 0.6686540514502520294, 0.7354980260655306079, 0.8028463152565280536, 0.8633854507756927310, 0.9437142632666988273, 1.000000000000000000 ),
 ( 0.000000000000000000, 1.000000000000000000 ),
 .UNSPECIFIED. ) ;
#74898=CARTESIAN_POINT ( 'NONE',  ( 66.47089632795841396, 68.63383729509693865, -3.041274391255982756 ) ) ;
#74900=CARTESIAN_POINT ( 'NONE',  ( 69.40172078258943600, 62.86412582178058273, -13.69687571282228511 ) ) ;
#74904=CARTESIAN_POINT ( 'NONE',  ( 82.45205179438404741, 51.63644557190858819, 14.69498684280020662 ) ) ;
#74905=CARTESIAN_POINT ( 'NONE',  ( 82.13437940688061190, 41.17851433583147269, -3.455252894430590249 ) ) ;
#74910=CARTESIAN_POINT ( 'NONE',  ( 82.27124186229274017, 40.74952593748430019, -3.675396864436865307 ) ) ;
#74914=CARTESIAN_POINT ( 'NONE',  ( 79.17142675679626507, 47.23956432523275595, 13.38762579824775223 ) ) ;
#74915=CARTESIAN_POINT ( 'NONE',  ( 67.23123923419436210, 69.37383865658286197, -0.9211790948078316665 ) ) ;
#74916=ADVANCED_FACE ( 'NONE', ( #26232 ), #38523, .T. ) ;
#74921=EDGE_CURVE ( 'NONE', #14677, #19304, #5423, .T. ) ;
#74922=CARTESIAN_POINT ( 'NONE',  ( 66.47763888052396908, 67.99612994702233948, 6.463816604053789661 ) ) ;
#74923=CARTESIAN_POINT ( 'NONE',  ( 67.07005509396013565, 69.31304007049533311, 0.5152274618438157372 ) ) ;
#74924=CARTESIAN_POINT ( 'NONE',  ( 85.47913374364790684, 42.62622548008751266, 0.2499991700750583967 ) ) ;
#74926=CARTESIAN_POINT ( 'NONE',  ( 41.03800390905408335, 35.64441083166263979, -10.00000000000000533 ) ) ;
#74927=CARTESIAN_POINT ( 'NONE',  ( 79.21668578049593634, 56.34399116799300344, -16.56718607364530627 ) ) ;
#74929=CARTESIAN_POINT ( 'NONE',  ( 72.28225989300379695, 72.02129029449646680, 3.461803769446522239 ) ) ;
#74935=CARTESIAN_POINT ( 'NONE',  ( 78.23057914463134921, 51.11287733427894864, -15.28606483983534936 ) ) ;
#74936=CARTESIAN_POINT ( 'NONE',  ( 71.63329245445480353, 72.42139875791372106, -1.350275132429440861 ) ) ;
#74938=CARTESIAN_POINT ( 'NONE',  ( 27.11361191214091804, 16.44966523072495335, -2.296566073217252530E-15 ) ) ;
#74941=CARTESIAN_POINT ( 'NONE',  ( 3.104905098483929482, 23.83396525600387506, -2.839279412974133887 ) ) ;
#74946=CARTESIAN_POINT ( 'NONE',  ( 73.28832484065085850, 67.50848624533098530, -11.46336223192518844 ) ) ;
#74948=AXIS2_PLACEMENT_3D ( 'NONE', #58713, #49632, #97755 ) ;
#74956=LINE ( 'NONE', #67842, #82144 ) ;
#74962=CARTESIAN_POINT ( 'NONE',  ( 79.11321178432963563, 45.92345112123121709, -12.55202503363903155 ) ) ;
#74966=CARTESIAN_POINT ( 'NONE',  ( 86.53679916633876701, 47.27946550500259804, -10.19252361861625111 ) ) ;
#74970=CARTESIAN_POINT ( 'NONE',  ( 20.38389956778225809, 29.95586893147755703, 7.433330006724141015 ) ) ;
#74971=CARTESIAN_POINT ( 'NONE',  ( 76.39152921487998071, 62.56948907837542606, 15.23512175509495137 ) ) ;
#74981=CARTESIAN_POINT ( 'NONE',  ( 70.46175891972434613, 71.28076662974713429, -3.876972208410735199 ) ) ;
#74982=CARTESIAN_POINT ( 'NONE',  ( 65.88300657315410547, 69.00302489017140317, -2.153913200402058248 ) ) ;
#74992=VERTEX_POINT ( 'NONE', #33082 ) ;
#75003=B_SPLINE_CURVE_WITH_KNOTS ( 'NONE', 3,
 ( #86634, #33374, #16673, #23763, #17169, #32375, #64278, #48069, #31861, #15665, #56157, #94216, #79010, #87152, #55156, #62761, #980, #78495, #70370, #9081, #40459, #79525, #9597, #71395, #1985, #8584, #32870, #63776, #48584, #17684, #95229, #63274, #10086, #94708, #47567, #62253, #40949, #24280, #2492, #93719, #39951, #54151, #85113, #38961, #46559, #77494 ),
 .UNSPECIFIED., .F., .F.,
 ( 4, 1, 2, 2, 1, 2, 2, 1, 1, 2, 2, 1, 1, 2, 2, 1, 1, 2, 2, 1, 1, 1, 2, 2, 1, 1, 1, 2, 2, 4 ),
 ( 0.000000000000000000, 0.06250000000000068001, 0.09374999999999913958, 0.1249999999999976130, 0.1874999999999949485, 0.2187499999999950040, 0.2499999999999950318, 0.3124999999999953926, 0.3437499999999953371, 0.3593749999999956701, 0.3749999999999960032, 0.4374999999999978351, 0.4687499999999970024, 0.4843749999999983902, 0.4999999999999997780, 0.5624999999999968914, 0.5937499999999937828, 0.6093749999999906741, 0.6249999999999874545, 0.6874999999999754641, 0.7187499999999714673, 0.7343749999999694689, 0.7421874999999681366, 0.7499999999999666933, 0.8124999999999791278, 0.8437499999999833467, 0.8593749999999868994, 0.8671874999999871214, 0.8749999999999873435, 1.000000000000000000 ),
 .UNSPECIFIED. ) ;
#75016=CARTESIAN_POINT ( 'NONE',  ( 86.70911053808110580, 46.89117940024963360, 10.21290512048939902 ) ) ;
#75023=CARTESIAN_POINT ( 'NONE',  ( 85.34796002485173005, 43.47219069357272758, 5.045432809274035257 ) ) ;
#75024=EDGE_CURVE ( 'NONE', #31137, #40803, #44132, .T. ) ;
#75025=CARTESIAN_POINT ( 'NONE',  ( 80.32560484147226987, 44.93948968179056180, -11.21518412823304800 ) ) ;
#75026=B_SPLINE_CURVE_WITH_KNOTS ( 'NONE', 3,
 ( #86697, #93271, #24833, #31925, #87219, #70956, #63340, #94278, #62828, #56225, #87718, #10152, #41018, #17754, #79588, #55707, #71956, #2560, #63837, #17230, #56736, #9143, #39019, #24345, #69927, #2051, #93785, #1559, #544, #39511, #40525, #70436, #16239, #31426, #1046, #55219, #71460, #16739, #47628, #32933, #94775, #25335, #65339, #66336, #33964, #88702 ),
 .UNSPECIFIED., .F., .F.,
 ( 4, 1, 1, 1, 2, 2, 1, 1, 1, 2, 2, 1, 1, 2, 2, 1, 1, 2, 2, 1, 1, 2, 2, 1, 2, 2, 1, 2, 2, 4 ),
 ( 0.000000000000000000, 0.06250000000002643719, 0.09375000000003808065, 0.1093750000000423134, 0.1171875000000460465, 0.1250000000000497657, 0.1875000000000617562, 0.2187500000000678624, 0.2343750000000710543, 0.2421875000000724976, 0.2500000000000739409, 0.3125000000000892064, 0.3437500000000967004, 0.3593750000000985878, 0.3750000000001004752, 0.4375000000001050271, 0.4687500000001074141, 0.4843750000001070255, 0.5000000000001065814, 0.5625000000000948130, 0.5937500000000873746, 0.6093750000000841549, 0.6250000000000808242, 0.6875000000000719425, 0.7187500000000656142, 0.7500000000000592859, 0.8125000000000435207, 0.8437500000000360822, 0.8750000000000286438, 1.000000000000000000 ),
 .UNSPECIFIED. ) ;
#75027=CARTESIAN_POINT ( 'NONE',  ( 72.82976588666879536, 70.83552076258160923, 7.211487186626502677 ) ) ;
#75032=CARTESIAN_POINT ( 'NONE',  ( 76.16009226555104306, 53.07303640036436576, 15.95681292398955264 ) ) ;
#75036=CARTESIAN_POINT ( 'NONE',  ( 81.32851801649849222, 53.07575169590482744, 15.40321648735625004 ) ) ;
#75037=CARTESIAN_POINT ( 'NONE',  ( 73.64475323345853042, 69.68564092398970899, -9.517716319079164933 ) ) ;
#75043=CARTESIAN_POINT ( 'NONE',  ( 27.71094225399020061, 18.12755873383627403, -6.180339887498949025 ) ) ;
#75044=DIRECTION ( 'NONE',  ( -0.4972609476841356457, 0.8612812260087758798, 0.1045284632676436315 ) ) ;
#75046=CARTESIAN_POINT ( 'NONE',  ( 72.76074090227031377, 69.17543318582201550, -10.12738290133669850 ) ) ;
#75051=DIRECTION ( 'NONE',  ( -0.4635919272833941562, 0.8029647720336182681, 0.3746065934159032440 ) ) ;
#75053=CARTESIAN_POINT ( 'NONE',  ( 66.74093763034696281, 68.12488142277693726, -6.511293142817978996 ) ) ;
#75057=CARTESIAN_POINT ( 'NONE',  ( 25.88782454542109335, 20.11029122506295153, -8.090169943749478065 ) ) ;
#75058=CARTESIAN_POINT ( 'NONE',  ( 85.26413132878788304, 49.08502152628110338, 12.44825952561157578 ) ) ;
#75060=CARTESIAN_POINT ( 'NONE',  ( 71.73704408672971056, 72.08698097738312072, -3.607164568159269891 ) ) ;
#75064=CARTESIAN_POINT ( 'NONE',  ( 75.07870810345070822, 67.14405870075098903, 12.61863177765487620 ) ) ;
#75073=CARTESIAN_POINT ( 'NONE',  ( 38.63056705113294953, 37.70171378149921537, -9.188101187500004485 ) ) ;
#75080=CARTESIAN_POINT ( 'NONE',  ( 12.86511499041763074, 19.37878583063839244, 9.188101187500006262 ) ) ;
#75081=CARTESIAN_POINT ( 'NONE',  ( 71.85326037870231630, 72.57223462184857965, 1.067429543862033814 ) ) ;
#75086=EDGE_LOOP ( 'NONE', ( #55880, #78772, #54502, #11187 ) ) ;
#75089=CARTESIAN_POINT ( 'NONE',  ( 74.99952688636028597, 53.39440814940449798, -16.04976397322502990 ) ) ;
#75090=CARTESIAN_POINT ( 'NONE',  ( 81.12531108467926799, 42.43832548245816838, 7.730292043048938133 ) ) ;
#75094=CARTESIAN_POINT ( 'NONE',  ( 82.32736432458936804, 40.35218285420588558, 1.148310913625198104 ) ) ;
#75095=CYLINDRICAL_SURFACE ( 'NONE', #68746, 16.60714546451156792 ) ;
#75099=ORIENTED_EDGE ( 'NONE', *, *, #75481, .T. ) ;
#75105=CARTESIAN_POINT ( 'NONE',  ( 80.56183422562187957, 57.64990364647651688, 16.23776005631657426 ) ) ;
#75107=ORIENTED_EDGE ( 'NONE', *, *, #82056, .T. ) ;
#75109=CARTESIAN_POINT ( 'NONE',  ( 87.48484950937405813, 45.04520271710788393, -6.098260242492822059 ) ) ;
#75121=EDGE_CURVE ( 'NONE', #52122, #19903, #75359, .T. ) ;
#75122=LINE ( 'NONE', #5208, #40162 ) ;
#75126=CARTESIAN_POINT ( 'NONE',  ( 73.63577410123313882, 69.72805253716678919, 9.466241435726317377 ) ) ;
#75127=CARTESIAN_POINT ( 'NONE',  ( 87.24693701583447591, 43.60182921170479631, 0.4518306138544891382 ) ) ;
#75129=CARTESIAN_POINT ( 'NONE',  ( 82.62974588365311490, 53.86145749464596122, 15.83045060744369614 ) ) ;
#75134=ORIENTED_EDGE ( 'NONE', *, *, #14689, .T. ) ;
#75135=CARTESIAN_POINT ( 'NONE',  ( 75.96267333776768282, 57.39029935918532033, -16.11942128475391911 ) ) ;
#75137=CARTESIAN_POINT ( 'NONE',  ( 67.14419364460526651, 66.64754800388041645, 8.362635188899179894 ) ) ;
#75143=CARTESIAN_POINT ( 'NONE',  ( 71.02572423326354567, 67.25701790933874236, 10.42884077080723237 ) ) ;
#75145=CARTESIAN_POINT ( 'NONE',  ( 79.68566563166257311, 45.96296481709465809, 12.95737312212979297 ) ) ;
#75147=CARTESIAN_POINT ( 'NONE',  ( 80.91936912787150504, 54.12794304082212449, -16.13542988847117954 ) ) ;
#75158=CARTESIAN_POINT ( 'NONE',  ( 87.62133583293774564, 45.31115884160845297, -7.293173845241971875 ) ) ;
#75169=CARTESIAN_POINT ( 'NONE',  ( 69.42787255574388894, 70.69812650043003543, 0.7215327683271423043 ) ) ;
#75170=CARTESIAN_POINT ( 'NONE',  ( 81.66892272557473120, 41.49682992153503136, -5.273621467921760342 ) ) ;
#75178=CARTESIAN_POINT ( 'NONE',  ( 79.08643767721621032, 59.41746268492352101, -16.53334974603827945 ) ) ;
#75183=CARTESIAN_POINT ( 'NONE',  ( 72.24948267320672812, 68.65699682331809584, -10.35566155590062465 ) ) ;
#75185=CARTESIAN_POINT ( 'NONE',  ( 71.63279429240235174, 59.10062218824842972, -15.33079785499452896 ) ) ;
#75186=CARTESIAN_POINT ( 'NONE',  ( 71.99907712171530250, 72.20780430811404926, -1.638790099443578674 ) ) ;
#75189=CARTESIAN_POINT ( 'NONE',  ( 72.51691088610790814, 57.43791320888536234, 16.30873706240645049 ) ) ;
#75197=CARTESIAN_POINT ( 'NONE',  ( 22.00287929847174695, 28.10171378149919263, 9.188101187500008038 ) ) ;
#75199=CARTESIAN_POINT ( 'NONE',  ( 83.77593207218663451, 52.15966500954240104, -15.02877900679588130 ) ) ;
#75200=CARTESIAN_POINT ( 'NONE',  ( 81.80775818236242003, 41.72624112066809943, -5.623390783372381740 ) ) ;
#75202=CARTESIAN_POINT ( 'NONE',  ( 68.43883904695194076, 64.41866838014503571, 12.24487134208069783 ) ) ;
#75204=CARTESIAN_POINT ( 'NONE',  ( 79.84392966380758594, 46.37903614055092305, 13.18172969020267793 ) ) ;
#75210=FACE_OUTER_BOUND ( 'NONE', #93907, .T. ) ;
#75212=CARTESIAN_POINT ( 'NONE',  ( 79.14312167556931854, 57.64441083166269664, 0.000000000000000000 ) ) ;
#75215=CARTESIAN_POINT ( 'NONE',  ( 69.17578128875754828, 70.38967932611143397, 2.324284992333389699 ) ) ;
#75216=CARTESIAN_POINT ( 'NONE',  ( 73.93519270231455209, 68.56589142993286146, -10.88456953958179518 ) ) ;
#75218=CARTESIAN_POINT ( 'NONE',  ( 16.00201260034520345, 10.20801979619927380, -3.090169943749474069 ) ) ;
#75219=CARTESIAN_POINT ( 'NONE',  ( 73.00396795756827828, 57.62093675928252878, -16.32480838619500219 ) ) ;
#75222=CARTESIAN_POINT ( 'NONE',  ( 86.55235766077406367, 47.22292317728852140, -10.66532192617878749 ) ) ;
#75230=EDGE_LOOP ( 'NONE', ( #25771, #69545, #87532, #49546 ) ) ;
#75233=CARTESIAN_POINT ( 'NONE',  ( 73.14143739346300777, 69.59972439283021117, -9.872010100564622803 ) ) ;
#75235=CARTESIAN_POINT ( 'NONE',  ( 81.32406911314680542, 42.50972318262807192, -7.655652106578362037 ) ) ;
#75238=ORIENTED_EDGE ( 'NONE', *, *, #67122, .T. ) ;
#75244=EDGE_LOOP ( 'NONE', ( #15151, #87404, #62215, #25869 ) ) ;
#75245=CARTESIAN_POINT ( 'NONE',  ( 75.35497918779043403, 60.43207667070393541, 15.59439205038279574 ) ) ;
#75252=CARTESIAN_POINT ( 'NONE',  ( 82.61003618271377036, 54.05539744841610172, -15.51395791714448968 ) ) ;
#75255=FACE_OUTER_BOUND ( 'NONE', #87981, .T. ) ;
#75256=CARTESIAN_POINT ( 'NONE',  ( 2.953350652821653988, 23.74646525600387648, 2.839279412974139660 ) ) ;
#75259=DIRECTION ( 'NONE',  ( 0.5000000000000013323, -0.8660254037844378194, 0.000000000000000000 ) ) ;
#75270=EDGE_CURVE ( 'NONE', #18761, #31643, #93722, .T. ) ;
#75271=CARTESIAN_POINT ( 'NONE',  ( 74.74960108721565177, 62.34916436530387784, -14.94383104034243814 ) ) ;
#75282=CARTESIAN_POINT ( 'NONE',  ( 24.50477583610994259, 37.08080186712593473, -3.090169943749475845 ) ) ;
#75285=EDGE_LOOP ( 'NONE', ( #44787, #98798, #46003, #69485 ) ) ;
#75290=EDGE_CURVE ( 'NONE', #75472, #97425, #85758, .T. ) ;
#75293=CARTESIAN_POINT ( 'NONE',  ( 85.18020382826158254, 42.46978738886356552, 0.9382811178248954276 ) ) ;
#75295=CARTESIAN_POINT ( 'NONE',  ( 83.36075103893979588, 44.36208028417300397, 8.738630005962992442 ) ) ;
#75299=CARTESIAN_POINT ( 'NONE',  ( 87.75630041960181416, 44.40081992046322057, -3.969603809391093474 ) ) ;
#75301=CARTESIAN_POINT ( 'NONE',  ( 78.65335153445595040, 54.31254791370685098, 15.95818423819602216 ) ) ;
#75303=CARTESIAN_POINT ( 'NONE',  ( 83.61754957953866096, 52.24592005514148951, -14.70745080183156972 ) ) ;
#75307=CARTESIAN_POINT ( 'NONE',  ( 70.56051678902534263, 60.79552409407079949, -14.52389266189133998 ) ) ;
#75308=CARTESIAN_POINT ( 'NONE',  ( 84.64741752562134991, 50.25350151326510684, 13.85721388315136693 ) ) ;
#75316=CARTESIAN_POINT ( 'NONE',  ( 8.584303441219292452, 23.14336893147753571, 7.433330006724141015 ) ) ;
#75321=CARTESIAN_POINT ( 'NONE',  ( 84.43425781732527469, 42.39747773327804481, -3.149235988505898476 ) ) ;
#75325=CARTESIAN_POINT ( 'NONE',  ( 43.77620770598743150, 30.98920272979930601, 7.433330006724137462 ) ) ;
#75329=CARTESIAN_POINT ( 'NONE',  ( 20.05074681235918277, 34.68290643055188127, 3.479690158560446702E-15 ) ) ;
#75333=CARTESIAN_POINT ( 'NONE',  ( 70.47930578771455146, 60.95205399099343424, 14.96696578811553735 ) ) ;
#75335=CARTESIAN_POINT ( 'NONE',  ( 73.67706877977251168, 59.42851455646710690, 16.04744940023546818 ) ) ;
#75338=( BOUNDED_CURVE ( )  B_SPLINE_CURVE ( 2, ( #68469, #22870, #69471, #46151, #99397, #29975, #91816, #14775, #91315, #53755, #61857, #90838, #21389 ),
 .UNSPECIFIED., .F., .T. ) 
 B_SPLINE_CURVE_WITH_KNOTS ( ( 3, 2, 2, 2, 2, 2, 3 ),
 ( 0.5625000000000000000, 0.5649999999999999467, 0.5699999999999999512, 0.5749999999999999556, 0.5799999999999999600, 0.5849999999999999645, 0.5875000000000000222 ),
 .UNSPECIFIED. ) 
 CURVE ( )  GEOMETRIC_REPRESENTATION_ITEM ( )  RATIONAL_B_SPLINE_CURVE ( ( 0.9755282581475768211, 0.9755282581475768211, 1.000000000000000000, 0.9510565162951535312, 1.000000000000000000, 0.9510565162951535312, 1.000000000000000000, 0.9510565162951535312, 1.000000000000000000, 0.9510565162951535312, 1.000000000000000000, 0.9755282581475761550, 0.9755282581475767101 ) ) 
 REPRESENTATION_ITEM ( '' )  );
#75341=CARTESIAN_POINT ( 'NONE',  ( 70.98573842219099106, 65.83761980621460452, 12.30238249020369423 ) ) ;
#75344=CARTESIAN_POINT ( 'NONE',  ( 85.17037076274338858, 42.84250995736751833, 3.387596126962762355 ) ) ;
#75348=ADVANCED_FACE ( 'NONE', ( #63122 ), #54495, .T. ) ;
#75349=FACE_OUTER_BOUND ( 'NONE', #91184, .T. ) ;
#75355=CARTESIAN_POINT ( 'NONE',  ( 39.71190250773520347, 34.87878583063844928, -9.188101187500006262 ) ) ;
#75356=CARTESIAN_POINT ( 'NONE',  ( 78.31430634746025987, 58.80323091815131420, -16.15417916714726587 ) ) ;
#75359=( BOUNDED_CURVE ( )  B_SPLINE_CURVE ( 2, ( #89815, #20390, #51261, #82225, #26988, #96928, #19415, #41668, #73590, #95933, #12799, #12291, #4170 ),
 .UNSPECIFIED., .F., .T. ) 
 B_SPLINE_CURVE_WITH_KNOTS ( ( 3, 2, 2, 2, 2, 2, 3 ),
 ( 0.4375000000000000000, 0.4400000000000000022, 0.4450000000000000067, 0.4500000000000000111, 0.4550000000000000155, 0.4600000000000000200, 0.4625000000000000222 ),
 .UNSPECIFIED. ) 
 CURVE ( )  GEOMETRIC_REPRESENTATION_ITEM ( )  RATIONAL_B_SPLINE_CURVE ( ( 0.9755282581475768211, 0.9755282581475768211, 1.000000000000000000, 0.9510565162951535312, 1.000000000000000000, 0.9510565162951535312, 1.000000000000000000, 0.9510565162951535312, 1.000000000000000000, 0.9510565162951535312, 1.000000000000000000, 0.9755282581475768211, 0.9755282581475768211 ) ) 
 REPRESENTATION_ITEM ( '' )  );
#75362=EDGE_CURVE ( 'NONE', #1759, #35085, #32219, .T. ) ;
#75363=VERTEX_POINT ( 'NONE', #40303 ) ;
#75365=CARTESIAN_POINT ( 'NONE',  ( 87.22108034532067222, 46.19249316086605006, -9.000540691006557736 ) ) ;
#75370=CARTESIAN_POINT ( 'NONE',  ( 82.10283259859586735, 40.80311082331518691, 1.497507696010887512 ) ) ;
#75372=CARTESIAN_POINT ( 'NONE',  ( 77.00910850481052705, 63.69207575539577704, -14.97815254220546954 ) ) ;
#75375=ORIENTED_EDGE ( 'NONE', *, *, #16957, .T. ) ;
#75378=VERTEX_POINT ( 'NONE', #32718 ) ;
#75380=CARTESIAN_POINT ( 'NONE',  ( 74.06641568892433725, 68.90029856846140888, -11.17356148674937444 ) ) ;
#75383=CARTESIAN_POINT ( 'NONE',  ( 68.83415823943913381, 70.27335860090030906, 4.117195521840038452 ) ) ;
#75384=CARTESIAN_POINT ( 'NONE',  ( 74.24029763082349120, 55.47955095029949746, -16.12046342301015756 ) ) ;
#75387=ORIENTED_EDGE ( 'NONE', *, *, #15980, .F. ) ;
#75393=CARTESIAN_POINT ( 'NONE',  ( 83.70131808852121935, 48.44858958261185933, 12.58427742406832905 ) ) ;
#75399=CARTESIAN_POINT ( 'NONE',  ( 81.78459505290653908, 48.88907504212919974, 13.50450084590696953 ) ) ;
#75400=CARTESIAN_POINT ( 'NONE',  ( 82.40024631258233967, 41.31310794220259197, -3.382981533264477036 ) ) ;
#75401=EDGE_CURVE ( 'NONE', #7307, #37182, #88911, .T. ) ;
#75402=CARTESIAN_POINT ( 'NONE',  ( 73.27328646083023500, 70.16270934360544231, -9.274526489422585840 ) ) ;
#75405=CARTESIAN_POINT ( 'NONE',  ( 84.00948332465746660, 44.55099784152547215, 8.476636100854188172 ) ) ;
#75408=CARTESIAN_POINT ( 'NONE',  ( 66.79485077809044924, 69.14189238270698468, -0.3922495213730473607 ) ) ;
#75411=CARTESIAN_POINT ( 'NONE',  ( 77.84925963432132789, 61.76067837358136359, 16.06420508523131474 ) ) ;
#75414=VECTOR ( 'NONE', #100205, 999.9999999999998863 ) ;
#75419=CARTESIAN_POINT ( 'NONE',  ( 43.54162044069033755, 26.10801979619932567, 3.090169943749476733 ) ) ;
#75420=CARTESIAN_POINT ( 'NONE',  ( 73.38975662564067193, 58.44531319176417128, -16.23198634866734125 ) ) ;
#75423=CARTESIAN_POINT ( 'NONE',  ( 72.08446838866018425, 72.31872904169155447, 3.483634709754487080 ) ) ;
#75429=CARTESIAN_POINT ( 'NONE',  ( 71.81907866082414671, 72.09960760913652678, -1.684840435608867759 ) ) ;
#75431=CARTESIAN_POINT ( 'NONE',  ( 24.63222838094502265, 17.14754757982090538, -5.678558825948275768 ) ) ;
#75434=CARTESIAN_POINT ( 'NONE',  ( 36.46445469440066489, 39.79103043416552055, 8.090169943749478065 ) ) ;
#75436=CARTESIAN_POINT ( 'NONE',  ( 76.37262670668393127, 61.51550187027301320, 15.91785308945339494 ) ) ;
#75440=CARTESIAN_POINT ( 'NONE',  ( 68.30469270138026161, 67.85665571424478060, -7.560265020520116508 ) ) ;
#75442=CARTESIAN_POINT ( 'NONE',  ( 82.30057295520377636, 41.22186192095817603, 3.240003865797013383 ) ) ;
#75443=CARTESIAN_POINT ( 'NONE',  ( 87.76310869853918462, 45.07707962072153407, -6.704660406813174767 ) ) ;
#75452=PLANE ( 'NONE',  #54761 ) ;
#75455=CARTESIAN_POINT ( 'NONE',  ( 79.23893794663464973, 46.12127630347242757, -13.23827507291852434 ) ) ;
#75457=CARTESIAN_POINT ( 'NONE',  ( 23.75126848931443746, 37.21091486745861943, 7.012934429366973338E-14 ) ) ;
#75462=CARTESIAN_POINT ( 'NONE',  ( 17.35762855594305520, 30.99752408145591431, 5.678558825948276656 ) ) ;
#75463=CARTESIAN_POINT ( 'NONE',  ( 76.24236140527241901, 61.49608671980659835, 15.50578537986026539 ) ) ;
#75464=CARTESIAN_POINT ( 'NONE',  ( 68.55793687630249167, 69.78307366813099577, -3.432291385973068820 ) ) ;
#75465=CARTESIAN_POINT ( 'NONE',  ( 75.32733269473096982, 66.70192330152532634, -13.01492205759767629 ) ) ;
#75466=ORIENTED_EDGE ( 'NONE', *, *, #68274, .T. ) ;
#75471=ORIENTED_EDGE ( 'NONE', *, *, #85667, .T. ) ;
#75472=VERTEX_POINT ( 'NONE', #73786 ) ;
#75479=CARTESIAN_POINT ( 'NONE',  ( 81.89559477234445239, 55.33976261442212774, 16.26127046582525892 ) ) ;
#75481=EDGE_CURVE ( 'NONE', #77239, #68127, #77899, .T. ) ;
#75486=CARTESIAN_POINT ( 'NONE',  ( 79.70677143361787387, 46.01134058561531504, 12.98241517792750699 ) ) ;
#75490=VERTEX_POINT ( 'NONE', #76757 ) ;
#75492=CARTESIAN_POINT ( 'NONE',  ( 76.25214315863026115, 65.18377266038437767, 14.56725100193072109 ) ) ;
#75499=CARTESIAN_POINT ( 'NONE',  ( 71.91558025072355065, 67.94660262428635633, 10.25156427071338605 ) ) ;
#75500=CARTESIAN_POINT ( 'NONE',  ( 87.77058453035330388, 45.11289234403166404, 6.766180878992243741 ) ) ;
#75506=CARTESIAN_POINT ( 'NONE',  ( 76.06558573277115443, 51.36628043362249230, -15.65277118209960250 ) ) ;
#75514=CARTESIAN_POINT ( 'NONE',  ( 88.27143343078938642, 44.36575123808635368, 4.213746458969102271 ) ) ;
#75518=AXIS2_PLACEMENT_3D ( 'NONE', #68673, #99105, #99598 ) ;
#75520=CARTESIAN_POINT ( 'NONE',  ( 67.53205783091016201, 67.39954269358065631, -7.583584584872256507 ) ) ;
#75522=CARTESIAN_POINT ( 'NONE',  ( 76.24083095996626014, 53.42879034202049837, 15.99957989301804062 ) ) ;
#75525=CARTESIAN_POINT ( 'NONE',  ( 81.64670028806227720, 55.20916848805968158, 15.89581094406439554 ) ) ;
#75526=CARTESIAN_POINT ( 'NONE',  ( 73.61548149140467956, 69.27229284252211983, -9.996823136999276826 ) ) ;
#75533=CARTESIAN_POINT ( 'NONE',  ( 19.40821860046903069, 26.90829794293880539, 10.00000000000000355 ) ) ;
#75536=CARTESIAN_POINT ( 'NONE',  ( 21.11941962201201051, 24.14441083166261137, 10.00000000000000533 ) ) ;
#75543=CARTESIAN_POINT ( 'NONE',  ( 66.89753708227109996, 68.17595765912082584, -6.590651905259176324 ) ) ;
#75549=CARTESIAN_POINT ( 'NONE',  ( 24.85415417228448121, 26.30066082961422680, -10.00000000000000533 ) ) ;
#75550=CARTESIAN_POINT ( 'NONE',  ( 85.46201571263348740, 48.63304775035897620, 12.47391791266364791 ) ) ;
#75552=CARTESIAN_POINT ( 'NONE',  ( 72.01505508543084488, 71.76016648463198067, -3.920346449359661367 ) ) ;
#75559=DIRECTION ( 'NONE',  ( 0.1039558454088763267, -0.1800568059919503139, 0.9781476007338069101 ) ) ;
#75568=DIRECTION ( 'NONE',  ( 0.5000000000000013323, -0.8660254037844378194, 0.000000000000000000 ) ) ;
#75570=PRODUCT_CONTEXT ( 'NONE', #62128, 'mechanical' ) ;
#75571=CARTESIAN_POINT ( 'NONE',  ( 18.60133699236122595, 19.24335787977762990, -9.188101187500008038 ) ) ;
#75573=CARTESIAN_POINT ( 'NONE',  ( 82.70618072881376293, 53.83593579450208466, 15.81121719814038151 ) ) ;
#75574=CARTESIAN_POINT ( 'NONE',  ( 71.73982542038400823, 59.04037670598220444, 15.86454711389505334 ) ) ;
#75580=CARTESIAN_POINT ( 'NONE',  ( 81.48503363143359479, 41.97952132416679660, 7.656029848638611135 ) ) ;
#75581=CARTESIAN_POINT ( 'NONE',  ( 35.92001165216885994, 44.23654200823204974, 1.583844403245397769 ) ) ;
#75584=CARTESIAN_POINT ( 'NONE',  ( 67.78283758264466030, 69.71839983238106697, 0.6266629628056711310 ) ) ;
#75589=AXIS2_PLACEMENT_3D ( 'NONE', #69931, #70964, #85185 ) ;
#75593=CARTESIAN_POINT ( 'NONE',  ( 88.45040933577318754, 44.05593677119288287, -2.476488480078137933 ) ) ;
#75595=CARTESIAN_POINT ( 'NONE',  ( 80.44596413951620661, 57.92004253751065335, -16.60216415864725903 ) ) ;
#75599=ADVANCED_FACE ( 'NONE', ( #85927 ), #1265, .T. ) ;
#75600=EDGE_LOOP ( 'NONE', ( #38965, #49825, #11596, #17512 ) ) ;
#75608=CARTESIAN_POINT ( 'NONE',  ( 32.19481522723634725, 40.36126292948897287, 6.180339887498949913 ) ) ;
#75615=CARTESIAN_POINT ( 'NONE',  ( 82.38367100173057622, 53.80119691343342936, 15.85271891126490473 ) ) ;
#75620=CARTESIAN_POINT ( 'NONE',  ( 74.54785486515559967, 57.86623053792277460, -15.96777695429060806 ) ) ;
#75625=CARTESIAN_POINT ( 'NONE',  ( 71.22129689212546566, 72.22986999219065751, -0.8113714082787989446 ) ) ;
#75628=VECTOR ( 'NONE', #5635, 1000.000000000000227 ) ;
#75629=ORIENTED_EDGE ( 'NONE', *, *, #49148, .F. ) ;
#75631=CARTESIAN_POINT ( 'NONE',  ( 78.21076945151075677, 53.49648267122271506, -15.87264874329164677 ) ) ;
#75636=EDGE_LOOP ( 'NONE', ( #85227, #10693, #75375, #68207 ) ) ;
#75640=CARTESIAN_POINT ( 'NONE',  ( 85.93470712620026575, 48.23248545518190866, 11.93606436224419376 ) ) ;
#75648=B_SPLINE_CURVE_WITH_KNOTS ( 'NONE', 3,
 ( #548, #45140, #29944, #62321, #53243, #62832, #22346, #38533, #47133, #31430, #84198, #14253, #31928, #93274, #23831, #14745 ),
 .UNSPECIFIED., .F., .F.,
 ( 4, 1, 2, 2, 2, 1, 2, 2, 4 ),
 ( 0.000000000000000000, 0.1250000000000026368, 0.1875000000000034972, 0.2500000000000043854, 0.5000000000000066613, 0.6250000000000064393, 0.6875000000000063283, 0.7500000000000061062, 1.000000000000000000 ),
 .UNSPECIFIED. ) ;
#75652=AXIS2_PLACEMENT_3D ( 'NONE', #31598, #69615, #85888 ) ;
#75654=CARTESIAN_POINT ( 'NONE',  ( 72.93625488370378207, 69.25789689889019485, 9.544539825114355835 ) ) ;
#75656=CARTESIAN_POINT ( 'NONE',  ( 72.18990340680744566, 72.03918383723207342, -3.149060597287207219 ) ) ;
#75662=CARTESIAN_POINT ( 'NONE',  ( 68.91022223105564137, 64.71151235087043574, -12.22836756590942464 ) ) ;
#75667=CARTESIAN_POINT ( 'NONE',  ( 79.29973261757051262, 59.57579620614538385, -16.53044932756547425 ) ) ;
#75672=CARTESIAN_POINT ( 'NONE',  ( 4.441398484865463736, 26.65659080271448289, -1.878358725466461243E-16 ) ) ;
#75674=CARTESIAN_POINT ( 'NONE',  ( 71.50716427137886910, 59.09066120637785247, -15.81421025005064607 ) ) ;
#75679=CARTESIAN_POINT ( 'NONE',  ( 72.97550374175638410, 57.18490168260592554, 15.90463394248157947 ) ) ;
#75680=CARTESIAN_POINT ( 'NONE',  ( 70.37206268826852806, 70.13158196118115484, 5.629252521285986077 ) ) ;
#75688=CARTESIAN_POINT ( 'NONE',  ( 24.12224894148702248, 22.43085787977763701, -9.188101187500008038 ) ) ;
#75690=CARTESIAN_POINT ( 'NONE',  ( 83.68493280611274088, 51.65299594367198210, -14.83749715326822205 ) ) ;
#75692=CARTESIAN_POINT ( 'NONE',  ( 82.28003896795380001, 40.62557011406286733, -3.142018250819525793 ) ) ;
#75694=CARTESIAN_POINT ( 'NONE',  ( 68.62869117346340886, 64.12329276949824930, 11.92149815895183096 ) ) ;
#75699=CARTESIAN_POINT ( 'NONE',  ( 67.44257088943838596, 67.25355904234817217, -8.657396272410824878 ) ) ;
#75701=CARTESIAN_POINT ( 'NONE',  ( 5.721601707324311725, 18.70171378149916919, -9.188101187500004485 ) ) ;
#75702=ORIENTED_EDGE ( 'NONE', *, *, #3598, .F. ) ;
#75705=LINE ( 'NONE', #21497, #21517 ) ;
#75706=EDGE_CURVE ( 'NONE', #7688, #35964, #58485, .T. ) ;
#75708=CARTESIAN_POINT ( 'NONE',  ( 71.48480579176155914, 72.35852322450824659, 1.080755764661565754 ) ) ;
#75713=CARTESIAN_POINT ( 'NONE',  ( 67.36253031349440334, 68.54163467477879124, 5.081825066198372376 ) ) ;
#75717=CARTESIAN_POINT ( 'NONE',  ( 10.05514423959709447, 21.50829794293879260, -10.00000000000000355 ) ) ;
#75721=CARTESIAN_POINT ( 'NONE',  ( 86.42645758268480449, 47.01732744055364321, -10.52632212332717998 ) ) ;
#75722=CARTESIAN_POINT ( 'NONE',  ( 82.81350700933505493, 45.30993475200613574, -10.24506358842424270 ) ) ;
#75725=ADVANCED_FACE ( 'NONE', ( #96008 ), #47835, .T. ) ;
#75728=CARTESIAN_POINT ( 'NONE',  ( 69.42144788871627270, 62.89730317705431872, 13.10748580973936761 ) ) ;
#75729=ORIENTED_EDGE ( 'NONE', *, *, #30530, .T. ) ;
#75733=CARTESIAN_POINT ( 'NONE',  ( 81.38720151904264810, 42.05902438066944171, -7.878585452988780879 ) ) ;
#75734=EDGE_CURVE ( 'NONE', #73618, #69104, #80259, .T. ) ;
#75737=EDGE_CURVE ( 'NONE', #54050, #75363, #89938, .T. ) ;
#75740=CARTESIAN_POINT ( 'NONE',  ( 81.53437377926626084, 50.59759334475508297, 14.46997207384287343 ) ) ;
#75742=CARTESIAN_POINT ( 'NONE',  ( 69.41547982834435970, 69.97450927703960133, 4.531412641460686785 ) ) ;
#75749=CARTESIAN_POINT ( 'NONE',  ( 69.33709985148358612, 68.43352380735160523, -7.655773901753416766 ) ) ;
#75751=VERTEX_POINT ( 'NONE', #90401 ) ;
#75753=CARTESIAN_POINT ( 'NONE',  ( 9.708348802340269756, 27.64646525600388571, -2.839279412974133887 ) ) ;
#75756=CARTESIAN_POINT ( 'NONE',  ( 85.69780903665139249, 48.74868904809778059, 11.98201799417179991 ) ) ;
#75757=LINE ( 'NONE', #91984, #15318 ) ;
#75769=CARTESIAN_POINT ( 'NONE',  ( 71.40813930945712684, 63.30437739610238168, -13.57462368570346278 ) ) ;
#75773=CARTESIAN_POINT ( 'NONE',  ( 82.78552022943677002, 53.33943766691666610, -15.29229482101202109 ) ) ;
#75778=CARTESIAN_POINT ( 'NONE',  ( 72.08805153644932773, 72.27453658898816968, 1.326354783638816315 ) ) ;
#75782=CARTESIAN_POINT ( 'NONE',  ( 76.19586783375881112, 65.24272250020374031, 14.11841093771251643 ) ) ;
#75785=ORIENTED_EDGE ( 'NONE', *, *, #13908, .T. ) ;
#75793=CARTESIAN_POINT ( 'NONE',  ( 84.36168211171367659, 46.55299321218482334, 10.66842414931385541 ) ) ;
#75798=CARTESIAN_POINT ( 'NONE',  ( 65.83444237920811304, 68.98881161217069291, 2.061071955463292138 ) ) ;
#75803=CARTESIAN_POINT ( 'NONE',  ( 81.93876147804334664, 52.90231730716391922, -15.25894681625440974 ) ) ;
#75806=CARTESIAN_POINT ( 'NONE',  ( 83.07104351211755500, 49.91350363301629045, 14.17192785442602876 ) ) ;
#75808=CARTESIAN_POINT ( 'NONE',  ( 84.80230723680845983, 50.33593218185897911, 13.42795335988696870 ) ) ;
#75817=CARTESIAN_POINT ( 'NONE',  ( 12.50787272796288896, 10.14754757982087874, -5.678558825948276656 ) ) ;
#75820=CARTESIAN_POINT ( 'NONE',  ( 17.30334773395576775, 15.15404122711132651, 8.090169943749479842 ) ) ;
#75821=CARTESIAN_POINT ( 'NONE',  ( 83.12755468652130730, 42.05662557703112014, -4.534451112896598524 ) ) ;
#75826=CARTESIAN_POINT ( 'NONE',  ( 42.70206918026079990, 25.44966523072497822, -2.296566073217252530E-15 ) ) ;
#75829=EDGE_LOOP ( 'NONE', ( #99638, #56235 ) ) ;
#75830=CARTESIAN_POINT ( 'NONE',  ( 30.57771352727866443, 18.44966523072494979, -2.296566073217252530E-15 ) ) ;
#75837=CARTESIAN_POINT ( 'NONE',  ( 70.32997052007365824, 61.22580503597990287, 14.81304146787438114 ) ) ;
#75844=CARTESIAN_POINT ( 'NONE',  ( 73.59537120146498523, 69.79291368717997557, 9.952181187355030545 ) ) ;
#75846=VERTEX_POINT ( 'NONE', #42730 ) ;
#75848=CARTESIAN_POINT ( 'NONE',  ( 77.99518601148065500, 61.05539905302716619, -15.87786080876372274 ) ) ;
#75850=EDGE_CURVE ( 'NONE', #29132, #47356, #99600, .T. ) ;
#75862=CARTESIAN_POINT ( 'NONE',  ( 41.11799749075662191, 32.24335787977766898, -9.188101187500008038 ) ) ;
#75866=CARTESIAN_POINT ( 'NONE',  ( 87.65988181639181676, 45.35027930547009589, 6.479635358970763370 ) ) ;
#75867=ORIENTED_EDGE ( 'NONE', *, *, #20309, .F. ) ;
#75869=CARTESIAN_POINT ( 'NONE',  ( 72.04834849415195208, 72.28436413801230742, -0.8995985284803106330 ) ) ;
#75872=CARTESIAN_POINT ( 'NONE',  ( 79.73371708168252781, 56.78064988272082303, 16.21239358597816604 ) ) ;
#75877=CARTESIAN_POINT ( 'NONE',  ( 75.82000616564076267, 60.49516838392244011, -15.67118054971322572 ) ) ;
#75878=CARTESIAN_POINT ( 'NONE',  ( 82.08371825655493126, 40.78504432597228657, 1.422816544139647199 ) ) ;
#75880=CARTESIAN_POINT ( 'NONE',  ( 77.25314033157172844, 63.01322228697468830, -15.27545204580677485 ) ) ;
#75885=CARTESIAN_POINT ( 'NONE',  ( 43.73469409959700016, 27.11110640527295956, -2.839279412974138328 ) ) ;
#75889=CARTESIAN_POINT ( 'NONE',  ( 73.80638704669732419, 68.31061168272384521, -11.57820046455322149 ) ) ;
#75895=ORIENTED_EDGE ( 'NONE', *, *, #2786, .T. ) ;
#75903=CARTESIAN_POINT ( 'NONE',  ( 83.03413861592977696, 46.38630032584844542, 11.19405999254725437 ) ) ;
#75905=CARTESIAN_POINT ( 'NONE',  ( 69.79485179726921729, 63.14629169217509030, -13.66398113955644789 ) ) ;
#75909=CARTESIAN_POINT ( 'NONE',  ( 71.40961132680497769, 62.47877890195463380, 13.99073973727416842 ) ) ;
#75913=CARTESIAN_POINT ( 'NONE',  ( 71.76780065431621836, 72.18842372171909005, 3.264426277842164659 ) ) ;
#75914=CARTESIAN_POINT ( 'NONE',  ( 84.35478657919151146, 45.19241756715437930, 9.088159741279909554 ) ) ;
#75917=CARTESIAN_POINT ( 'NONE',  ( 70.63918758082388649, 61.42057648183527618, -14.80585868731052024 ) ) ;
#75930=CARTESIAN_POINT ( 'NONE',  ( 73.07600783879472317, 69.60248043393922046, -9.824339152688605026 ) ) ;
#75931=LINE ( 'NONE', #52588, #88513 ) ;
#75934=CARTESIAN_POINT ( 'NONE',  ( 38.43992769770077444, 34.14441083166263979, 10.00000000000000533 ) ) ;
#75936=CARTESIAN_POINT ( 'NONE',  ( 82.18797279649203347, 54.21966230526519581, 15.63691867135833036 ) ) ;
#75937=CARTESIAN_POINT ( 'NONE',  ( 72.27517474642483819, 72.00281888946810227, 3.513552353559626251 ) ) ;
#75944=CARTESIAN_POINT ( 'NONE',  ( 81.09727246379429744, 50.28454668112130577, -14.41009495042581712 ) ) ;
#75945=CARTESIAN_POINT ( 'NONE',  ( 71.72790558683757922, 72.47596629505412125, -1.350878852920679662 ) ) ;
#75948=CARTESIAN_POINT ( 'NONE',  ( 24.72364882272980324, 19.98920272979926693, 7.433330006724137462 ) ) ;
#75951=CARTESIAN_POINT ( 'NONE',  ( 5.721601707324312613, 18.70171378149916563, -9.188101187500004485 ) ) ;
#75956=CARTESIAN_POINT ( 'NONE',  ( 72.74023158506105347, 61.92935225774390773, 14.60112725577257820 ) ) ;
#75960=CARTESIAN_POINT ( 'NONE',  ( 87.69397940208136788, 45.37340796770510565, -6.500714127684745769 ) ) ;
#75973=CARTESIAN_POINT ( 'NONE',  ( 79.18282792688175675, 45.86070727306254469, -12.48096782606623734 ) ) ;
#75981=CARTESIAN_POINT ( 'NONE',  ( 19.25324864145614967, 26.51421378149919761, -9.188101187500004485 ) ) ;
#75982=CARTESIAN_POINT ( 'NONE',  ( 69.60857895278438434, 70.05621065339627762, -4.634882221859216500 ) ) ;
#75991=CARTESIAN_POINT ( 'NONE',  ( 67.78902524216930203, 70.26539227734573956, -0.4897883682968208752 ) ) ;
#75994=CARTESIAN_POINT ( 'NONE',  ( 81.17232691891706509, 55.55242957854174080, 16.36487835605630536 ) ) ;
#76006=VERTEX_POINT ( 'NONE', #39609 ) ;
#76009=CARTESIAN_POINT ( 'NONE',  ( 66.47155029869672660, 67.83944574720587184, 6.769174700624444263 ) ) ;
#76011=CARTESIAN_POINT ( 'NONE',  ( 82.84795146572012925, 42.04542452314480272, -6.343602513311916269 ) ) ;
#76012=CARTESIAN_POINT ( 'NONE',  ( 81.45345171730303946, 56.09117390121627977, 16.06974809975275420 ) ) ;
#76014=CARTESIAN_POINT ( 'NONE',  ( 71.93069005840953878, 67.98409351856226124, 10.22207861052760158 ) ) ;
#76019=ADVANCED_FACE ( 'NONE', ( #61919, #14833 ), #45721, .F. ) ;
#76020=CARTESIAN_POINT ( 'NONE',  ( 76.26909101152743631, 50.98313773053103404, -15.54286448327743742 ) ) ;
#76021=FACE_OUTER_BOUND ( 'NONE', #6473, .T. ) ;
#76023=VECTOR ( 'NONE', #16004, 1000.000000000000114 ) ;
#76029=CARTESIAN_POINT ( 'NONE',  ( 88.16762080519842470, 44.42520534355205797, 4.589585637743891944 ) ) ;
#76030=CARTESIAN_POINT ( 'NONE',  ( 85.75643568251058468, 43.97353779226914838, 5.730478947345492458 ) ) ;
#76033=CARTESIAN_POINT ( 'NONE',  ( 73.01638763941097920, 70.78844651441271196, 7.463027675286954654 ) ) ;
#76034=CARTESIAN_POINT ( 'NONE',  ( 68.96171688564015767, 67.43038479987662015, -8.781394817860746826 ) ) ;
#76042=CARTESIAN_POINT ( 'NONE',  ( 88.06269261788010283, 43.61796610520789841, 0.05835779599787610517 ) ) ;
#76047=CARTESIAN_POINT ( 'NONE',  ( 27.95316317257044858, 17.10801979619929725, 3.090169943749476733 ) ) ;
#76053=CARTESIAN_POINT ( 'NONE',  ( 71.91872812886755639, 71.71754829396212472, -3.869976083996915506 ) ) ;
#76058=VECTOR ( 'NONE', #70495, 1000.000000000000114 ) ;
#76060=CARTESIAN_POINT ( 'NONE',  ( 72.90882467353794993, 70.31776273714770298, -8.127408542227577470 ) ) ;
#76064=CARTESIAN_POINT ( 'NONE',  ( 32.55392312662736032, 19.76426979415091267, 3.090169943749476733 ) ) ;
#76065=CARTESIAN_POINT ( 'NONE',  ( 85.63659005182417161, 48.93691085330170409, 12.16422113781264969 ) ) ;
#76068=CARTESIAN_POINT ( 'NONE',  ( 81.53115339410011586, 41.92267797703283350, -7.515177224638169839 ) ) ;
#76077=EDGE_CURVE ( 'NONE', #44339, #78746, #74127, .T. ) ;
#76081=CARTESIAN_POINT ( 'NONE',  ( 79.20158430517960824, 60.00302764608026251, 16.13772425423236356 ) ) ;
#76082=CARTESIAN_POINT ( 'NONE',  ( 38.02916716989017942, 40.14336893147758900, 7.433330006724141015 ) ) ;
#76090=CARTESIAN_POINT ( 'NONE',  ( 10.42942532566755354, 26.99752408145590721, 5.678558825948277544 ) ) ;
#76091=CARTESIAN_POINT ( 'NONE',  ( 15.60912251971356213, 9.416033932543239615, -1.583844403245366905 ) ) ;
#76092=CARTESIAN_POINT ( 'NONE',  ( 71.96630278948212833, 59.14415382642645369, 15.87175206068406830 ) ) ;
#76097=CARTESIAN_POINT ( 'NONE',  ( 81.64979810624366507, 42.63530321562527803, 7.555915214504083544 ) ) ;
#76101=CARTESIAN_POINT ( 'NONE',  ( 82.35828269511283395, 40.36336379056105272, 1.060027914477761568 ) ) ;
#76102=CARTESIAN_POINT ( 'NONE',  ( 76.52571587298459121, 63.66138771598714641, 14.90242614926261311 ) ) ;
#76110=DIRECTION ( 'NONE',  ( -0.8660254037844379305, -0.5000000000000014433, -0.000000000000000000 ) ) ;
#76111=CARTESIAN_POINT ( 'NONE',  ( 80.29526846451028632, 57.41841621455482425, -16.58920233904881414 ) ) ;
#76113=B_SPLINE_CURVE_WITH_KNOTS ( 'NONE', 3,
 ( #34711, #96565, #58017, #99523, #53880, #91956, #91443, #45783, #53398, #23482 ),
 .UNSPECIFIED., .F., .F.,
 ( 4, 2, 2, 2, 4 ),
 ( 0.000000000000000000, 0.0002622400424272684142, 0.0005244800848545368285, 0.0007867201272818051885, 0.001048960169709073657 ),
 .UNSPECIFIED. ) ;
#76115=CARTESIAN_POINT ( 'NONE',  ( 87.56962886756771525, 45.10300061070547173, -6.116038350875187213 ) ) ;
#76116=EDGE_CURVE ( 'NONE', #23265, #9880, #71802, .T. ) ;
#76119=CARTESIAN_POINT ( 'NONE',  ( 74.52124453458169739, 63.30200860632920268, 14.49837560861971397 ) ) ;
#76122=CARTESIAN_POINT ( 'NONE',  ( 78.26215446592701142, 47.40418697570542861, -14.30981545185047565 ) ) ;
#76123=ORIENTED_EDGE ( 'NONE', *, *, #50822, .T. ) ;
#76131=CARTESIAN_POINT ( 'NONE',  ( 83.32561943262588500, 42.79751196862224560, -6.107886559562847317 ) ) ;
#76139=CARTESIAN_POINT ( 'NONE',  ( 70.39753563717141560, 68.48327457168743138, 8.534146841718333931 ) ) ;
#76142=CARTESIAN_POINT ( 'NONE',  ( 70.70420039156243774, 71.94848598797803163, 6.061257734329015641E-06 ) ) ;
#76144=CARTESIAN_POINT ( 'NONE',  ( 78.08372258140214228, 47.78081774239645796, 14.00095081412197473 ) ) ;
#76148=CARTESIAN_POINT ( 'NONE',  ( 79.26202630790012904, 53.12952634897852278, -15.69712025940643230 ) ) ;
#76149=CARTESIAN_POINT ( 'NONE',  ( 84.54826043205098074, 42.30827120018470566, 4.527376015812757615 ) ) ;
#76150=CARTESIAN_POINT ( 'NONE',  ( 79.26278427487086731, 46.15226300323974584, 12.64627858079322742 ) ) ;
#76152=CARTESIAN_POINT ( 'NONE',  ( 83.62455065227555906, 52.34512318633653649, -15.13772682721065621 ) ) ;
#76153=VECTOR ( 'NONE', #78517, 1000.000000000000000 ) ;
#76158=CARTESIAN_POINT ( 'NONE',  ( 72.60043212129588142, 71.47019982953712258, 5.638345928473151858 ) ) ;
#76162=DIRECTION ( 'NONE',  ( -0.8660254037844378194, -0.5000000000000014433, -0.000000000000000000 ) ) ;
#76168=CARTESIAN_POINT ( 'NONE',  ( 72.70715679364579387, 68.59801517648534741, 10.11885734070592413 ) ) ;
#76170=EDGE_CURVE ( 'NONE', #41092, #12902, #81513, .T. ) ;
#76178=EDGE_LOOP ( 'NONE', ( #65900, #81872, #78888, #69692 ) ) ;
#76184=CARTESIAN_POINT ( 'NONE',  ( 72.56357867676685203, 68.60059663970191934, -10.60869006465324205 ) ) ;
#76186=CARTESIAN_POINT ( 'NONE',  ( 71.51902242164648271, 59.42281871825910144, -15.72106062734085086 ) ) ;
#76187=DIRECTION ( 'NONE',  ( 0.5000000000000014433, -0.8660254037844378194, 0.000000000000000000 ) ) ;
#76191=CARTESIAN_POINT ( 'NONE',  ( 74.17656091806652796, 55.29306353059418910, 16.12363719729034983 ) ) ;
#76193=CARTESIAN_POINT ( 'NONE',  ( 66.36286506768924198, 68.17188559719302532, -4.442151567769474951 ) ) ;
#76194=VERTEX_POINT ( 'NONE', #28803 ) ;
#76198=CARTESIAN_POINT ( 'NONE',  ( 29.82838080365165112, 20.14754757982091249, -5.678558825948276656 ) ) ;
#76200=CARTESIAN_POINT ( 'NONE',  ( 83.70911819089758410, 52.26791303372475994, -15.08805761434582848 ) ) ;
#76201=FACE_OUTER_BOUND ( 'NONE', #63097, .T. ) ;
#76202=CARTESIAN_POINT ( 'NONE',  ( 88.03161368674544462, 43.80918251920727613, 2.446934266190726959 ) ) ;
#76204=CARTESIAN_POINT ( 'NONE',  ( 68.61953357195196190, 64.26322109196938470, 12.44723069995015408 ) ) ;
#76208=LINE ( 'NONE', #29102, #36163 ) ;
#76222=CARTESIAN_POINT ( 'NONE',  ( 14.17036660571061546, 16.38052372038639604, 10.00000000000000533 ) ) ;
#76228=B_SPLINE_CURVE_WITH_KNOTS ( 'NONE', 3,
 ( #63173, #70266, #69272, #93101, #8481, #62659, #93611, #86044, #47469, #1391, #38865, #32270, #94117, #57063, #65666, #25692 ),
 .UNSPECIFIED., .F., .F.,
 ( 4, 1, 2, 2, 2, 1, 2, 2, 4 ),
 ( 0.000000000000000000, 0.1250000000000010547, 0.1875000000000006384, 0.2500000000000002220, 0.4999999999999973355, 0.6249999999999953371, 0.6874999999999966693, 0.7499999999999980016, 1.000000000000000000 ),
 .UNSPECIFIED. ) ;
#76231=DIRECTION ( 'NONE',  ( -0.2702110370271922357, -0.9515975153008174869, 0.1464519181916024981 ) ) ;
#76234=CARTESIAN_POINT ( 'NONE',  ( 69.53918912477176661, 62.67033094902271984, 13.85614356406449943 ) ) ;
#76238=CARTESIAN_POINT ( 'NONE',  ( 73.34339640511194602, 69.67785411864186074, -9.916893174164222557 ) ) ;
#76240=CARTESIAN_POINT ( 'NONE',  ( 81.52667467699143344, 42.23108980399940293, -8.023880245682178725 ) ) ;
#76241=ORIENTED_EDGE ( 'NONE', *, *, #174, .T. ) ;
#76247=CARTESIAN_POINT ( 'NONE',  ( 68.87408322772347447, 69.31020849774787962, 5.424133776871966184 ) ) ;
#76253=CARTESIAN_POINT ( 'NONE',  ( 82.81311453349250939, 53.82731390497905721, -15.42448983893086734 ) ) ;
#76256=CARTESIAN_POINT ( 'NONE',  ( 14.74991654177707723, 23.91421378149918198, 9.188101187500008038 ) ) ;
#76258=CARTESIAN_POINT ( 'NONE',  ( 84.42663183290279960, 49.91580812419739743, -13.73522929182741059 ) ) ;
#76269=CARTESIAN_POINT ( 'NONE',  ( 70.75662654094317361, 63.45050265575406456, -13.26425860699792914 ) ) ;
#76275=CARTESIAN_POINT ( 'NONE',  ( 86.90280484423139740, 44.67138223063114566, -5.898473692909979249 ) ) ;
#76286=DIRECTION ( 'NONE',  ( 0.5000000000000013323, -0.8660254037844378194, 0.000000000000000000 ) ) ;
#76289=CARTESIAN_POINT ( 'NONE',  ( 83.98545619398112194, 45.63022158774919745, 9.896021495624898634 ) ) ;
#76296=FACE_OUTER_BOUND ( 'NONE', #53043, .T. ) ;
#76303=CARTESIAN_POINT ( 'NONE',  ( 70.57238475796081900, 60.71229067232671639, -14.56237343984944665 ) ) ;
#76306=CARTESIAN_POINT ( 'NONE',  ( 68.68578350440056113, 68.40580704404837320, 7.012371262790892956 ) ) ;
#76316=CARTESIAN_POINT ( 'NONE',  ( 83.76485939058579788, 42.20955296087365127, -3.876374748171139029 ) ) ;
#76319=FACE_OUTER_BOUND ( 'NONE', #36447, .T. ) ;
#76320=CARTESIAN_POINT ( 'NONE',  ( 44.43411998782967487, 26.44966523072498177, -2.296566073217252530E-15 ) ) ;
#76322=FACE_BOUND ( 'NONE', #13104, .T. ) ;
#76324=CARTESIAN_POINT ( 'NONE',  ( 22.15746398174156440, 34.83396525600390703, -2.839279412974133887 ) ) ;
#76330=B_SPLINE_CURVE_WITH_KNOTS ( 'NONE', 3,
 ( #71989, #55251, #64378, #56769, #54756, #85742, #1082, #47163, #87751, #80122, #32966, #10684, #41562, #72506, #63873, #9179, #93307, #8676, #24869, #23864, #16270, #39546, #1597, #70468, #31960, #86233, #16768, #47660, #78594, #32480, #63376 ),
 .UNSPECIFIED., .F., .F.,
 ( 4, 3, 3, 3, 3, 3, 3, 3, 3, 3, 4 ),
 ( 0.000000000000000000, 0.1333490885032340423, 0.3007194338854312643, 0.4699862290245129803, 0.5844252810809342780, 0.6686540514502644639, 0.7354980260655447077, 0.8028463152565625816, 0.8633854507757121599, 0.9437142632667110398, 1.000000000000000000 ),
 .UNSPECIFIED. ) ;
#76331=CARTESIAN_POINT ( 'NONE',  ( 70.85940962530331433, 60.99147867796299494, 15.04089833736761328 ) ) ;
#76332=CARTESIAN_POINT ( 'NONE',  ( 75.98901751930753790, 65.25029023645535631, -14.46192986472697584 ) ) ;
#76335=CARTESIAN_POINT ( 'NONE',  ( 75.13052455607011382, 52.91100154115419230, -15.99857184472472760 ) ) ;
#76339=CARTESIAN_POINT ( 'NONE',  ( 33.64972468124413751, 31.37878583063843152, 9.188101187500006262 ) ) ;
#76343=EDGE_LOOP ( 'NONE', ( #62106, #41677, #49932, #26259 ) ) ;
#76351=CARTESIAN_POINT ( 'NONE',  ( 34.33172647011804202, 40.79752408145594700, -5.678558825948271327 ) ) ;
#76352=CARTESIAN_POINT ( 'NONE',  ( 81.49529596843051138, 56.10236560196279498, -16.41626961062114631 ) ) ;
#76353=EDGE_CURVE ( 'NONE', #38635, #90112, #85086, .T. ) ;
#76354=CARTESIAN_POINT ( 'NONE',  ( 68.68909986782581711, 64.16576715805911135, -12.55144644517788421 ) ) ;
#76365=CARTESIAN_POINT ( 'NONE',  ( 78.21946184288361792, 59.52378438228485180, -16.11278392467423970 ) ) ;
#76373=CARTESIAN_POINT ( 'NONE',  ( 31.15319227796116053, 18.39040679176984128, -6.890680421881970419E-14 ) ) ;
#76374=CARTESIAN_POINT ( 'NONE',  ( 45.09207854535236493, 28.96004757982094446, -5.678558825948276656 ) ) ;
#76377=ORIENTED_EDGE ( 'NONE', *, *, #10755, .F. ) ;
#76378=CARTESIAN_POINT ( 'NONE',  ( 73.92441827737660276, 68.29833774401778612, -11.64939612493447996 ) ) ;
#76386=ORIENTED_EDGE ( 'NONE', *, *, #74231, .F. ) ;
#76398=VERTEX_POINT ( 'NONE', #45970 ) ;
#76400=CARTESIAN_POINT ( 'NONE',  ( 72.44101633376520510, 65.82767294218574250, 12.36625408228399259 ) ) ;
#76402=CARTESIAN_POINT ( 'NONE',  ( 82.41127205671455158, 40.84167155264970006, -3.717692515266792341 ) ) ;
#76406=CARTESIAN_POINT ( 'NONE',  ( 82.70173776682830180, 42.57814917962534196, 6.376911687432284204 ) ) ;
#76410=CARTESIAN_POINT ( 'NONE',  ( 71.65769282842789778, 70.70965056591087716, -6.033769676015556804 ) ) ;
#76420=CARTESIAN_POINT ( 'NONE',  ( 76.54298794630824432, 51.21710260455724040, 16.04984378097219633 ) ) ;
#76423=CARTESIAN_POINT ( 'NONE',  ( 44.68504016816519453, 27.92755873383629606, 6.180339887498953466 ) ) ;
#76426=CARTESIAN_POINT ( 'NONE',  ( 72.14611019483686505, 72.30310738408833515, 3.684292749196578232 ) ) ;
#76433=CARTESIAN_POINT ( 'NONE',  ( 20.70865909420142259, 30.14336893147755703, 7.433330006724141015 ) ) ;
#76436=CARTESIAN_POINT ( 'NONE',  ( 16.06339478488542127, 14.98920272979925272, 7.433330006724137462 ) ) ;
#76438=CARTESIAN_POINT ( 'NONE',  ( 77.24238159045749796, 63.47610639771342278, 15.48509222746617553 ) ) ;
#76441=CARTESIAN_POINT ( 'NONE',  ( 72.18153366120698422, 59.81188395286972082, 15.22051537925258202 ) ) ;
#76443=CARTESIAN_POINT ( 'NONE',  ( 81.30930031418027681, 54.60213497152520290, -15.79650731256931273 ) ) ;
#76448=CARTESIAN_POINT ( 'NONE',  ( 77.52100321733644250, 49.65180640845364479, 14.92792641300140843 ) ) ;
#76455=CARTESIAN_POINT ( 'NONE',  ( 79.21048608390624679, 45.84430088201565212, -12.45846168025711798 ) ) ;
#76457=CARTESIAN_POINT ( 'NONE',  ( 72.98228618152094782, 70.36901929029048119, -8.113406466234710734 ) ) ;
#76460=CARTESIAN_POINT ( 'NONE',  ( 18.92729281690869314, 22.87878583063841020, -9.188101187500006262 ) ) ;
#76461=CARTESIAN_POINT ( 'NONE',  ( 67.72713518178136383, 69.49437377556795070, -2.463275011707438900 ) ) ;
#76465=CYLINDRICAL_SURFACE ( 'NONE', #15817, 16.60714546451156792 ) ;
#76471=CARTESIAN_POINT ( 'NONE',  ( 67.92772920839225037, 65.41715411821847681, -10.39043899096739665 ) ) ;
#76483=VERTEX_POINT ( 'NONE', #80602 ) ;
#76485=CARTESIAN_POINT ( 'NONE',  ( 72.82159975088246995, 72.59360798638101642, 0.000000000000000000 ) ) ;
#76489=CARTESIAN_POINT ( 'NONE',  ( 66.92706188925286881, 68.00105104109823628, 6.962559168495445761 ) ) ;
#76491=EDGE_CURVE ( 'NONE', #50515, #96813, #73057, .T. ) ;
#76492=LINE ( 'NONE', #92231, #33647 ) ;
#76493=CARTESIAN_POINT ( 'NONE',  ( 80.96506752577832344, 55.91141337780396725, 16.08528190432093297 ) ) ;
#76500=CARTESIAN_POINT ( 'NONE',  ( 73.00396795756827828, 57.62093675928252878, -16.32480838619500219 ) ) ;
#76501=CARTESIAN_POINT ( 'NONE',  ( 76.04450315243209957, 65.42723423563565177, -13.97889933544638019 ) ) ;
#76507=CARTESIAN_POINT ( 'NONE',  ( 87.93413682123004094, 44.35120838780621000, 4.768703809423660012 ) ) ;
#76508=CARTESIAN_POINT ( 'NONE',  ( 42.35759689194659927, 26.58380873178790793, 6.180339887498953466 ) ) ;
#76511=CARTESIAN_POINT ( 'NONE',  ( 72.77087662098560372, 70.82427377826435588, 7.173618689453861386 ) ) ;
#76512=CARTESIAN_POINT ( 'NONE',  ( 71.00707024578083804, 67.28932756229654899, -10.38437885875134192 ) ) ;
#76520=CARTESIAN_POINT ( 'NONE',  ( 83.37362496471422446, 52.41223193542727898, 14.84798797970331563 ) ) ;
#76521=EDGE_CURVE ( 'NONE', #30181, #87380, #45212, .T. ) ;
#76525=CARTESIAN_POINT ( 'NONE',  ( 71.84797400569436832, 72.18106025956552685, -0.5846029390931422043 ) ) ;
#76529=FACE_BOUND ( 'NONE', #8696, .T. ) ;
#76531=AXIS2_PLACEMENT_3D ( 'NONE', #86826, #63957, #79213 ) ;
#76533=CARTESIAN_POINT ( 'NONE',  ( 26.98754258172029452, 23.78052372038640883, -10.00000000000000355 ) ) ;
#76534=CARTESIAN_POINT ( 'NONE',  ( 80.56202954020663753, 57.53823600680942718, 16.23110421993949259 ) ) ;
#76539=ORIENTED_EDGE ( 'NONE', *, *, #46245, .T. ) ;
#76540=CARTESIAN_POINT ( 'NONE',  ( 66.56294892191600354, 68.00698982583806185, -6.541986041792972273 ) ) ;
#76541=CARTESIAN_POINT ( 'NONE',  ( 72.74024025722110309, 70.77703717069300637, -7.960999691682589585 ) ) ;
#76544=CARTESIAN_POINT ( 'NONE',  ( 28.50119043139558883, 18.58380873178787951, 6.180339887498953466 ) ) ;
#76545=CARTESIAN_POINT ( 'NONE',  ( 77.12554246003209357, 53.45558293378064718, 16.40013681541701018 ) ) ;
#76548=B_SPLINE_SURFACE_WITH_KNOTS ( 'NONE', 3, 1, ( 
 ( #50780, #13310 ),
 ( #4702, #35592 ),
 ( #91316, #75105 ),
 ( #81730, #67479 ),
 ( #58861, #12307 ),
 ( #21390, #28999 ),
 ( #83217, #44660 ),
 ( #28479, #6181 ),
 ( #12817, #37078 ),
 ( #20406, #67982 ),
 ( #21876, #43167 ),
 ( #36076, #66487 ),
 ( #43679, #74621 ),
 ( #66977, #97904 ),
 ( #59360, #16271 ),
 ( #69963, #93821 ),
 ( #84229, #47164 ),
 ( #7167, #22871 ),
 ( #53756, #15255 ),
 ( #38054, #68967 ),
 ( #84715, #70995 ),
 ( #24380, #31961 ),
 ( #69472, #77069 ),
 ( #55252, #30475 ),
 ( #91817, #86234 ),
 ( #86, #45658 ),
 ( #46152, #22377 ),
 ( #78088, #8182 ),
 ( #8677, #99890 ),
 ( #9180, #7677 ),
 ( #93308, #39547 ) ),
 .UNSPECIFIED., .F., .F., .F.,
 ( 4, 3, 3, 3, 3, 3, 3, 3, 3, 3, 4 ),
 ( 2, 2 ),
 ( 0.000000000000000000, 0.1333490885032399820, 0.3007194338854488058, 0.4699862290245400698, 0.5844252810809538179, 0.6686540514502882226, 0.7354980260655652469, 0.8028463152565959993, 0.8633854507757408037, 0.9437142632667595565, 1.000000000000000000 ),
 ( 0.000000000000000000, 1.000000000000000000 ),
 .UNSPECIFIED. ) ;
#76550=DIRECTION ( 'NONE',  ( -0.2938926261462390666, 0.5090369604551334692, 0.8090169943749425663 ) ) ;
#76552=CARTESIAN_POINT ( 'NONE',  ( 81.83268240801082527, 41.27904705060213075, 5.916546515311264187 ) ) ;
#76557=CARTESIAN_POINT ( 'NONE',  ( 45.41683807177152232, 29.14754757982093736, -5.678558825948276656 ) ) ;
#76563=CARTESIAN_POINT ( 'NONE',  ( 26.13094010387951371, 20.80170272979927049, 7.433330006724137462 ) ) ;
#76565=CARTESIAN_POINT ( 'NONE',  ( 71.62614020371384527, 59.05562564738432485, 15.34271347411686115 ) ) ;
#76567=EDGE_LOOP ( 'NONE', ( #13680, #89519, #38303, #96837, #21996, #84461 ) ) ;
#76569=CARTESIAN_POINT ( 'NONE',  ( 86.51254904731311512, 45.35660278255235056, -8.424040530456800013 ) ) ;
#76570=DIRECTION ( 'NONE',  ( 0.5000000000000013323, -0.8660254037844378194, 0.000000000000000000 ) ) ;
#76571=CARTESIAN_POINT ( 'NONE',  ( 81.49684083197098516, 42.49698986986711446, 7.471786974450515650 ) ) ;
#76572=DIRECTION ( 'NONE',  ( -0.8503781557569336513, 0.05328141121994486862, 0.5234673661555679924 ) ) ;
#76573=EDGE_LOOP ( 'NONE', ( #37365, #20317, #60133, #25030 ) ) ;
#76575=CARTESIAN_POINT ( 'NONE',  ( 70.21041392557471283, 70.96369918409062905, -2.494471698684542105 ) ) ;
#76576=CARTESIAN_POINT ( 'NONE',  ( 76.73487078864175714, 63.86935209113470080, 14.87109117981107076 ) ) ;
#76582=CARTESIAN_POINT ( 'NONE',  ( 72.11639660595672296, 70.09681734935580266, 8.459716556816276878 ) ) ;
#76595=EDGE_CURVE ( 'NONE', #35211, #16493, #12422, .T. ) ;
#76599=CARTESIAN_POINT ( 'NONE',  ( 36.11248442148217919, 32.80066082961424456, 10.00000000000000533 ) ) ;
#76601=EDGE_CURVE ( 'NONE', #64000, #62590, #11141, .T. ) ;
#76603=CARTESIAN_POINT ( 'NONE',  ( 73.08787508166213343, 59.01509672055304634, -15.57900745017619393 ) ) ;
#76605=CARTESIAN_POINT ( 'NONE',  ( 82.29734961797252879, 53.60383310410945512, 15.81226994477779790 ) ) ;
#76615=CARTESIAN_POINT ( 'NONE',  ( 66.98597148399355206, 67.06197240495457379, 8.554490737669659950 ) ) ;
#76617=CARTESIAN_POINT ( 'NONE',  ( 78.22548900086377444, 47.74579297413086465, 13.94123525276128994 ) ) ;
#76621=CARTESIAN_POINT ( 'NONE',  ( 71.22012620979680264, 67.74042170150684683, 10.05071617227448044 ) ) ;
#76623=CARTESIAN_POINT ( 'NONE',  ( 79.14837792229336344, 45.86247416287834966, 13.10094053291496508 ) ) ;
#76627=ORIENTED_EDGE ( 'NONE', *, *, #26577, .T. ) ;
#76631=CARTESIAN_POINT ( 'NONE',  ( 72.21801880702699350, 71.73430858976985292, 5.514776891874405784 ) ) ;
#76635=CARTESIAN_POINT ( 'NONE',  ( 66.70421483277053198, 67.41215751505673381, -6.693045608280014491 ) ) ;
#76639=CARTESIAN_POINT ( 'NONE',  ( 82.14960936660257573, 40.66333750097311395, 3.614425481505477489 ) ) ;
#76653=CARTESIAN_POINT ( 'NONE',  ( 83.52484103943936589, 46.90027433733275330, -11.98971445564651717 ) ) ;
#76656=CARTESIAN_POINT ( 'NONE',  ( 10.99774771173347432, 18.30066082961419838, -10.00000000000000533 ) ) ;
#76658=CARTESIAN_POINT ( 'NONE',  ( 71.72487096640281834, 58.74680701327284993, -15.44539912601161546 ) ) ;
#76663=CARTESIAN_POINT ( 'NONE',  ( 72.97677987389820942, 57.10916639992058208, 16.39923404589487177 ) ) ;
#76664=CARTESIAN_POINT ( 'NONE',  ( 69.39148564807371145, 65.38147651185532538, 11.91492136379578426 ) ) ;
#76665=CARTESIAN_POINT ( 'NONE',  ( 66.73167312141883656, 68.39993800570366034, -4.394447365586645837 ) ) ;
#76670=B_SPLINE_CURVE_WITH_KNOTS ( 'NONE', 3,
 ( #43095, #33023, #44591, #75037, #43609, #13716, #29906, #82674, #82170, #5614, #6618, #36506, #51731, #37492, #45106, #59800, #12745, #75526, #14214, #36005, #98334, #97349, #14707, #6111 ),
 .UNSPECIFIED., .F., .F.,
 ( 4, 2, 2, 2, 2, 2, 2, 2, 2, 2, 2, 4 ),
 ( 0.000000000000000000, 0.1250000000000001110, 0.2500000000000002220, 0.3750000000000003331, 0.4375000000000003886, 0.5000000000000004441, 0.5625000000000004441, 0.6250000000000005551, 0.6875000000000006661, 0.7500000000000006661, 0.8750000000000003331, 1.000000000000000000 ),
 .UNSPECIFIED. ) ;
#76673=CARTESIAN_POINT ( 'NONE',  ( 26.34264212020660167, 36.18502408145594273, 5.678558825948277544 ) ) ;
#76676=CARTESIAN_POINT ( 'NONE',  ( 75.36487073175837281, 53.53173320265494084, -16.04382577248123809 ) ) ;
#76680=CARTESIAN_POINT ( 'NONE',  ( 68.65765088900910484, 64.10725282940799730, 11.94679850282813938 ) ) ;
#76685=CARTESIAN_POINT ( 'NONE',  ( 11.38685760444945672, 12.28920272979924988, -7.433330006724141015 ) ) ;
#76692=CARTESIAN_POINT ( 'NONE',  ( 67.63503648096795473, 68.85725524262423392, 4.671258359888055267 ) ) ;
#76698=CARTESIAN_POINT ( 'NONE',  ( 70.80888052646473341, 69.64703403501997059, 8.011688916067704724 ) ) ;
#76699=CARTESIAN_POINT ( 'NONE',  ( 84.26010284367181669, 45.15451964197480095, -9.139984135955533162 ) ) ;
#76705=CARTESIAN_POINT ( 'NONE',  ( 69.75493487105953250, 62.68956563894904832, 13.91594397096109503 ) ) ;
#76715=CARTESIAN_POINT ( 'NONE',  ( 81.33756375948632922, 49.74101304335109575, 14.11251714982108574 ) ) ;
#76718=CARTESIAN_POINT ( 'NONE',  ( 68.03534369547149652, 68.16390280863178930, 6.778061388490955075 ) ) ;
#76721=LINE ( 'NONE', #44316, #12605 ) ;
#76726=CARTESIAN_POINT ( 'NONE',  ( 67.40003082602686391, 68.24590789163552529, -5.841565263471736991 ) ) ;
#76727=ORIENTED_EDGE ( 'NONE', *, *, #55904, .T. ) ;
#76729=CARTESIAN_POINT ( 'NONE',  ( 12.32504541118064978, 22.51421378149917985, -9.188101187500004485 ) ) ;
#76737=CARTESIAN_POINT ( 'NONE',  ( 67.79478323710348775, 65.59340164614276603, -10.86706726790307798 ) ) ;
#76739=CARTESIAN_POINT ( 'NONE',  ( 70.62955678152277983, 60.80479719363770386, -15.06269029744276899 ) ) ;
#76743=CARTESIAN_POINT ( 'NONE',  ( 75.07870222088889989, 67.13256391452972593, -13.06718628923150405 ) ) ;
#76746=CARTESIAN_POINT ( 'NONE',  ( 82.51756260356231110, 53.28320474767543402, -15.32090594621901758 ) ) ;
#76749=CARTESIAN_POINT ( 'NONE',  ( 83.23625814710678128, 44.68616627695709553, -9.226232325800772571 ) ) ;
#76752=CARTESIAN_POINT ( 'NONE',  ( 31.67936943677743855, 23.45404122711135386, -8.090169943749478065 ) ) ;
#76757=CARTESIAN_POINT ( 'NONE',  ( 64.41134571303810219, 67.16059528448873550, 0.000000000000000000 ) ) ;
#76758=CARTESIAN_POINT ( 'NONE',  ( 84.71689455500938948, 42.18615029519279602, 0.2983201894514607710 ) ) ;
#76760=CARTESIAN_POINT ( 'NONE',  ( 71.06207387823002364, 70.85672049742558443, 6.009000135645388596 ) ) ;
#76774=CARTESIAN_POINT ( 'NONE',  ( 80.74974841587442143, 43.27611110060701805, 10.01619596027649095 ) ) ;
#76779=CARTESIAN_POINT ( 'NONE',  ( 70.51171994387159714, 70.77651729788739488, 4.033880998964182396 ) ) ;
#76780=CARTESIAN_POINT ( 'NONE',  ( 71.47384123275857348, 72.35069954344788812, 1.100233114707620530 ) ) ;
#76785=ADVANCED_FACE ( 'NONE', ( #692 ), #53387, .T. ) ;
#76787=CARTESIAN_POINT ( 'NONE',  ( 12.64980493759981250, 22.70171378149918340, -9.188101187500004485 ) ) ;
#76788=CARTESIAN_POINT ( 'NONE',  ( 72.42824182984617210, 61.00551489497025415, -15.37960674554226159 ) ) ;
#76789=FACE_OUTER_BOUND ( 'NONE', #83968, .T. ) ;
#76790=CARTESIAN_POINT ( 'NONE',  ( 8.758203689844268780, 28.55466486950697913, -1.111400068045478839E-16 ) ) ;
#76795=CARTESIAN_POINT ( 'NONE',  ( 39.71070620960689723, 31.43085787977766543, -9.188101187500008038 ) ) ;
#76799=CARTESIAN_POINT ( 'NONE',  ( 31.93509797303403630, 20.29860640527293825, -2.839279412974138328 ) ) ;
#76800=CARTESIAN_POINT ( 'NONE',  ( 71.71174882302005926, 58.93038559421764688, -15.88944412480316259 ) ) ;
#76801=CARTESIAN_POINT ( 'NONE',  ( 82.25857016995360027, 53.22243677109732118, 15.71245593812844632 ) ) ;
#76804=CARTESIAN_POINT ( 'NONE',  ( 84.78734842081532008, 50.40784050611168965, -13.89907628984690113 ) ) ;
#76806=CARTESIAN_POINT ( 'NONE',  ( 75.00216722520403323, 65.29316891282158508, 14.16376155384191904 ) ) ;
#76810=CARTESIAN_POINT ( 'NONE',  ( 73.25535670630372920, 69.88482930906741331, 9.609716971570463784 ) ) ;
#76811=B_SPLINE_SURFACE_WITH_KNOTS ( 'NONE', 3, 1, ( 
 ( #99264, #38933 ),
 ( #46527, #22753 ),
 ( #68340, #98273 ),
 ( #30847, #91187 ),
 ( #28861, #59739 ),
 ( #85081, #61733 ),
 ( #92682, #90707 ),
 ( #45040, #52142 ),
 ( #37431, #83091 ),
 ( #13662, #75465 ),
 ( #450, #78465 ),
 ( #69838, #94187 ),
 ( #85606, #62225 ),
 ( #16146, #79493 ),
 ( #10055, #9049 ),
 ( #23729, #86605 ),
 ( #48553, #1463 ),
 ( #24740, #39919 ),
 ( #70339, #55622 ),
 ( #16641, #47045 ),
 ( #17139, #31341 ),
 ( #9566, #48036 ),
 ( #93687, #32839 ),
 ( #55127, #70854 ),
 ( #32343, #77960 ),
 ( #8552, #39421 ),
 ( #63246, #952 ),
 ( #47536, #31828 ),
 ( #40920, #2466 ),
 ( #93177, #78980 ),
 ( #94682, #17656 ) ),
 .UNSPECIFIED., .F., .F., .F.,
 ( 4, 3, 3, 3, 3, 3, 3, 3, 3, 3, 4 ),
 ( 2, 2 ),
 ( 0.000000000000000000, 0.1333490885032361239, 0.3007194338854258242, 0.4699862290245113705, 0.5844252810809250631, 0.6686540514502664623, 0.7354980260655568092, 0.8028463152565741279, 0.8633854507757309227, 0.9437142632667492315, 1.000000000000000000 ),
 ( 0.000000000000000000, 1.000000000000000000 ),
 .UNSPECIFIED. ) ;
#76812=CARTESIAN_POINT ( 'NONE',  ( 38.53854167689037524, 24.11110640527295246, -2.839279412974138328 ) ) ;
#76818=LINE ( 'NONE', #59101, #60306 ) ;
#76820=CARTESIAN_POINT ( 'NONE',  ( 85.05760017557965114, 49.81609225799626017, 13.45342997944402796 ) ) ;
#76826=ORIENTED_EDGE ( 'NONE', *, *, #47844, .T. ) ;
#76835=CARTESIAN_POINT ( 'NONE',  ( 72.39542100948224856, 61.59435533500952431, -14.66294840908354402 ) ) ;
#76836=CARTESIAN_POINT ( 'NONE',  ( 82.64100954815702949, 40.51523152100199354, 0.8905920172003339852 ) ) ;
#76838=EDGE_CURVE ( 'NONE', #79014, #82804, #22060, .T. ) ;
#76839=CARTESIAN_POINT ( 'NONE',  ( 77.18662672379076639, 63.56519964668829203, -15.06539499090657763 ) ) ;
#76842=CARTESIAN_POINT ( 'NONE',  ( 70.41572640437576069, 60.98787027670521610, -14.93661785217966198 ) ) ;
#76843=CARTESIAN_POINT ( 'NONE',  ( 43.36002773778349706, 27.96004757982094446, -5.678558825948276656 ) ) ;
#76849=CARTESIAN_POINT ( 'NONE',  ( 69.60926776342978428, 64.26717917311120232, -12.25031856425473364 ) ) ;
#76854=CARTESIAN_POINT ( 'NONE',  ( 73.85566786302621267, 55.32763327914238261, -16.11774481835226069 ) ) ;
#76855=ORIENTED_EDGE ( 'NONE', *, *, #95548, .F. ) ;
#76857=ORIENTED_EDGE ( 'NONE', *, *, #22340, .T. ) ;
#76861=CYLINDRICAL_SURFACE ( 'NONE', #67795, 16.60714546451156792 ) ;
#76870=CARTESIAN_POINT ( 'NONE',  ( 73.65729962767424865, 69.49757902785616182, 9.740712345197151123 ) ) ;
#76871=CARTESIAN_POINT ( 'NONE',  ( 82.50439176478489856, 40.89164830652052274, -3.703415047413355143 ) ) ;
#76875=VECTOR ( 'NONE', #62482, 1000.000000000000114 ) ;
#76877=CARTESIAN_POINT ( 'NONE',  ( 23.08833070876649529, 13.73415679381821874, 1.333680081654574804E-15 ) ) ;
#76888=CARTESIAN_POINT ( 'NONE',  ( 75.84856439504059722, 51.76521084193598199, 15.76359423700354689 ) ) ;
#76890=CARTESIAN_POINT ( 'NONE',  ( 45.03145032967896100, 28.12755873383630600, -6.180339887498949025 ) ) ;
#76893=CARTESIAN_POINT ( 'NONE',  ( 71.68255973785201718, 72.12657461437540007, 3.318624374305799041 ) ) ;
#76898=CARTESIAN_POINT ( 'NONE',  ( 81.24166145016371843, 42.23607023897516655, -7.290125548428411761 ) ) ;
#76903=AXIS2_PLACEMENT_3D ( 'NONE', #87429, #71669, #64547 ) ;
#76904=CARTESIAN_POINT ( 'NONE',  ( 15.40246583222295129, 30.93396525600389424, 2.839279412974139660 ) ) ;
#76906=CARTESIAN_POINT ( 'NONE',  ( 82.10990542498430500, 41.84899041517284957, 5.504228460268151046 ) ) ;
#76907=CARTESIAN_POINT ( 'NONE',  ( 17.90548643172614263, 12.19860640527291373, 2.839279412974134775 ) ) ;
#76911=CARTESIAN_POINT ( 'NONE',  ( 78.61941745410977944, 58.11157619480126613, -16.59458311719091128 ) ) ;
#76913=CARTESIAN_POINT ( 'NONE',  ( 82.09480132358520166, 40.75487975465649271, -0.9815627762904419740 ) ) ;
#76915=ADVANCED_FACE ( 'NONE', ( #22981 ), #61982, .T. ) ;
#76917=CARTESIAN_POINT ( 'NONE',  ( 76.73822351447255130, 56.29186403409720185, -16.16359082176946416 ) ) ;
#76922=CARTESIAN_POINT ( 'NONE',  ( 77.08242418523479955, 49.46725263400162476, 15.46546490473176938 ) ) ;
#76929=CARTESIAN_POINT ( 'NONE',  ( 79.21534038901880592, 46.09240496756496697, -13.22827714657437781 ) ) ;
#76932=CARTESIAN_POINT ( 'NONE',  ( 20.76088743254790359, 12.39040679176982529, 1.333680081654574804E-15 ) ) ;
#76934=CARTESIAN_POINT ( 'NONE',  ( 18.21401815691482895, 25.91421378149918553, 9.188101187500008038 ) ) ;
#76943=ORIENTED_EDGE ( 'NONE', *, *, #4642, .T. ) ;
#76946=CARTESIAN_POINT ( 'NONE',  ( 72.61942445857775397, 68.50386890797452111, 10.74179888713238107 ) ) ;
#76947=CARTESIAN_POINT ( 'NONE',  ( 67.71824482912023768, 65.66011283822241751, -10.75488218253084582 ) ) ;
#76950=DIRECTION ( 'NONE',  ( -0.8660254037844379305, -0.5000000000000014433, -0.000000000000000000 ) ) ;
#76959=CARTESIAN_POINT ( 'NONE',  ( 73.50309919034782524, 60.00084379880728847, -15.88072908836307029 ) ) ;
#76966=CARTESIAN_POINT ( 'NONE',  ( 66.94906710382659298, 68.02340058291366631, 6.944469598640234942 ) ) ;
#76972=CARTESIAN_POINT ( 'NONE',  ( 70.47523177494278457, 64.09717175604362183, 12.73376050057014197 ) ) ;
#76984=EDGE_LOOP ( 'NONE', ( #68402, #27780, #27511, #44654 ) ) ;
#76989=CARTESIAN_POINT ( 'NONE',  ( 72.72146555473813123, 70.80955590929056598, 7.150549449074294905 ) ) ;
#76995=CARTESIAN_POINT ( 'NONE',  ( 80.22871040234743134, 48.51986718445390778, 13.76706510026316899 ) ) ;
#76996=CARTESIAN_POINT ( 'NONE',  ( 83.46914375417860299, 52.40757773513071527, 14.82330941673155245 ) ) ;
#77005=CARTESIAN_POINT ( 'NONE',  ( 73.99094044066663400, 55.21107462180383862, 16.12321973269548536 ) ) ;
#77006=EDGE_CURVE ( 'NONE', #71517, #76398, #18497, .T. ) ;
#77007=CARTESIAN_POINT ( 'NONE',  ( 21.45610022030931674, 34.16126292948896293, -6.180339887498951690 ) ) ;
#77017=CARTESIAN_POINT ( 'NONE',  ( 67.02157033833375976, 67.70868166164997604, -6.467237866492896892 ) ) ;
#77019=CARTESIAN_POINT ( 'NONE',  ( 81.57634712059733317, 41.66383691174480930, 5.797449893469142523 ) ) ;
#77021=CARTESIAN_POINT ( 'NONE',  ( 76.77173841120222164, 63.31185858333683569, -15.44871830894366838 ) ) ;
#77022=CARTESIAN_POINT ( 'NONE',  ( 25.55253460671674759, 33.49103043416550918, -8.090169943749479842 ) ) ;
#77032=CARTESIAN_POINT ( 'NONE',  ( 44.96521122863986619, 26.36477965099644649, 1.583844403245364907 ) ) ;
#77035=CARTESIAN_POINT ( 'NONE',  ( 67.41248320326423027, 66.37693208286884783, -8.946798147498746800 ) ) ;
#77043=CARTESIAN_POINT ( 'NONE',  ( 19.08967936351193373, 31.99752408145592497, 5.678558825948277544 ) ) ;
#77045=CARTESIAN_POINT ( 'NONE',  ( 71.81391265307100014, 59.05408711125518550, 15.87230141160151575 ) ) ;
#77047=ORIENTED_EDGE ( 'NONE', *, *, #14843, .T. ) ;
#77049=CARTESIAN_POINT ( 'NONE',  ( 5.396842180905147224, 18.51421378149916208, -9.188101187500004485 ) ) ;
#77051=CARTESIAN_POINT ( 'NONE',  ( 80.25178558894602077, 57.14685393251872370, -16.23521980932009612 ) ) ;
#77059=CARTESIAN_POINT ( 'NONE',  ( 72.84393339948680079, 57.07810317368846142, 16.39299656256352833 ) ) ;
#77060=CARTESIAN_POINT ( 'NONE',  ( 87.35606880162971777, 45.77061481740688009, 8.290963297571636303 ) ) ;
#77062=VERTEX_POINT ( 'NONE', #60675 ) ;
#77063=EDGE_CURVE ( 'NONE', #56753, #315, #43759, .T. ) ;
#77065=CARTESIAN_POINT ( 'NONE',  ( 86.27418400483192329, 43.17587234054840195, -1.979591663834713966 ) ) ;
#77068=DIRECTION ( 'NONE',  ( 0.5000000000000014433, -0.8660254037844378194, 0.000000000000000000 ) ) ;
#77069=CARTESIAN_POINT ( 'NONE',  ( 79.91723393423865218, 58.07319122800065259, 16.26806395467770727 ) ) ;
#77070=CARTESIAN_POINT ( 'NONE',  ( 71.44486053167919692, 69.80518736647204037, -8.307854525019157776 ) ) ;
#77083=CARTESIAN_POINT ( 'NONE',  ( 78.17014198728131191, 47.55004527273559489, -13.86079054836211810 ) ) ;
#77088=CARTESIAN_POINT ( 'NONE',  ( 83.66769832939698404, 52.30133544591161865, 14.73017738415024169 ) ) ;
#77090=ORIENTED_EDGE ( 'NONE', *, *, #13148, .F. ) ;
#77101=CARTESIAN_POINT ( 'NONE',  ( 71.69982436666802528, 70.81612773607918143, 5.925385826462316707 ) ) ;
#77103=CARTESIAN_POINT ( 'NONE',  ( 67.03549487444914234, 66.88278970582167915, 8.847049729461536671 ) ) ;
#77104=CARTESIAN_POINT ( 'NONE',  ( 74.73315994561023956, 64.49924696742777996, -14.01681635444520957 ) ) ;
#77105=CARTESIAN_POINT ( 'NONE',  ( 78.15103970674991274, 47.75416819384486899, 13.96761498558048231 ) ) ;
#77109=CARTESIAN_POINT ( 'NONE',  ( 87.71125355519491507, 45.00661457325054471, -6.624481356856373182 ) ) ;
#77110=CARTESIAN_POINT ( 'NONE',  ( 79.08373359491760368, 46.13869499162948529, 12.70867304314121604 ) ) ;
#77112=CARTESIAN_POINT ( 'NONE',  ( 82.35285118013293015, 53.50770157854819331, -15.77620284334257938 ) ) ;
#77117=CARTESIAN_POINT ( 'NONE',  ( 72.14394712234364704, 71.70061920742823247, 5.492383471420795082 ) ) ;
#77123=FACE_OUTER_BOUND ( 'NONE', #42687, .T. ) ;
#77128=LINE ( 'NONE', #81918, #100146 ) ;
#77129=VERTEX_POINT ( 'NONE', #13127 ) ;
#77130=CARTESIAN_POINT ( 'NONE',  ( 70.37934122712871954, 61.23818324669216651, 14.28954007458889386 ) ) ;
#77131=CARTESIAN_POINT ( 'NONE',  ( 87.63170318219837895, 44.36446170533411504, -4.079950490519347106 ) ) ;
#77141=ORIENTED_EDGE ( 'NONE', *, *, #53901, .T. ) ;
#77148=CARTESIAN_POINT ( 'NONE',  ( 18.69751666607634988, 11.76426979415088958, 3.090169943749476733 ) ) ;
#77152=B_SPLINE_CURVE_WITH_KNOTS ( 'NONE', 3,
 ( #15820, #633, #1139, #48747 ),
 .UNSPECIFIED., .F., .F.,
 ( 4, 4 ),
 ( 0.000000000000000000, 0.1732562812666568475 ),
 .UNSPECIFIED. ) ;
#77153=FACE_OUTER_BOUND ( 'NONE', #813, .T. ) ;
#77157=CARTESIAN_POINT ( 'NONE',  ( 72.61990804881321537, 57.19017774089424222, 16.35758357749855207 ) ) ;
#77160=CARTESIAN_POINT ( 'NONE',  ( 66.51309011095609947, 68.84183934625441736, -4.405043755099953273 ) ) ;
#77161=ORIENTED_EDGE ( 'NONE', *, *, #8362, .T. ) ;
#77167=CARTESIAN_POINT ( 'NONE',  ( 25.99623195869281744, 35.98502408145594700, -5.678558825948271327 ) ) ;
#77170=CARTESIAN_POINT ( 'NONE',  ( 67.66477494612622934, 65.93994996590180335, 10.43000742999573838 ) ) ;
#77172=CARTESIAN_POINT ( 'NONE',  ( 66.21400821115226165, 68.61137286571008076, 2.321765048532279163 ) ) ;
#77173=VERTEX_POINT ( 'NONE', #14109 ) ;
#77177=CARTESIAN_POINT ( 'NONE',  ( 13.03712377304622194, 16.03085787977761356, 9.188101187500006262 ) ) ;
#77178=ORIENTED_EDGE ( 'NONE', *, *, #66634, .F. ) ;
#77180=CARTESIAN_POINT ( 'NONE',  ( 75.58214075417596689, 65.23491603964200181, 14.35294216029142333 ) ) ;
#77188=ORIENTED_EDGE ( 'NONE', *, *, #56694, .T. ) ;
#77191=CARTESIAN_POINT ( 'NONE',  ( 72.63381747954645107, 70.76794473758097581, 7.135479174949443504 ) ) ;
#77194=CARTESIAN_POINT ( 'NONE',  ( 68.74550570596571220, 65.29344765021964747, 11.68071900121614526 ) ) ;
#77195=CARTESIAN_POINT ( 'NONE',  ( 83.96921505230092464, 45.18285929837890080, -9.373418216583857543 ) ) ;
#77198=CARTESIAN_POINT ( 'NONE',  ( 79.52267089340274708, 59.39869781967021112, -16.20969956878131413 ) ) ;
#77200=CARTESIAN_POINT ( 'NONE',  ( 8.162811221194553823, 28.21091486745858745, -1.111400068045478839E-16 ) ) ;
#77203=CARTESIAN_POINT ( 'NONE',  ( 69.68191272334148323, 62.54370116513975830, 13.40392498406904842 ) ) ;
#77208=CARTESIAN_POINT ( 'NONE',  ( 73.20181606317161993, 69.60992630376679813, -9.900803345273253342 ) ) ;
#77215=CARTESIAN_POINT ( 'NONE',  ( 73.39810145532288743, 61.39966270044930496, 14.96885843746143152 ) ) ;
#77221=CARTESIAN_POINT ( 'NONE',  ( 82.84292370591116139, 47.81104087607728559, 12.42676687899641230 ) ) ;
#77224=CARTESIAN_POINT ( 'NONE',  ( 82.72605847261863232, 53.97080330652735825, -15.84526420522619894 ) ) ;
#77226=CARTESIAN_POINT ( 'NONE',  ( 11.72364552993787967, 24.95586893147754282, 7.433330006724141015 ) ) ;
#77228=CARTESIAN_POINT ( 'NONE',  ( 80.10302014060799536, 57.75140007922346541, 16.60262925785714216 ) ) ;
#77234=CARTESIAN_POINT ( 'NONE',  ( 77.30113122908805678, 49.12792392959498500, -15.30166374384701911 ) ) ;
#77235=CARTESIAN_POINT ( 'NONE',  ( 80.61151161062586823, 46.19852708120087215, -12.13081066922774731 ) ) ;
#77239=VERTEX_POINT ( 'NONE', #4505 ) ;
#77250=CARTESIAN_POINT ( 'NONE',  ( 72.41389820116259557, 70.72247311216293042, 7.745007521649655224 ) ) ;
#77252=CARTESIAN_POINT ( 'NONE',  ( 26.14792707536646432, 33.83478043621389020, -8.090169943749479842 ) ) ;
#77258=CARTESIAN_POINT ( 'NONE',  ( 83.11954624601993658, 46.44810582658406872, -11.20842123171843596 ) ) ;
#77260=CARTESIAN_POINT ( 'NONE',  ( 80.74781574657598071, 57.21644485803223290, 16.56566952311892749 ) ) ;
#77281=CARTESIAN_POINT ( 'NONE',  ( 69.15337702377902929, 69.07843188401378143, 6.265891433177522174 ) ) ;
#77290=ADVANCED_FACE ( 'NONE', ( #73311 ), #80447, .T. ) ;
#77292=CARTESIAN_POINT ( 'NONE',  ( 19.52749640002317122, 16.98920272979925628, 7.433330006724137462 ) ) ;
#77294=CARTESIAN_POINT ( 'NONE',  ( 80.59739948449713154, 56.56319013636019832, -16.53599074302314165 ) ) ;
#77299=CARTESIAN_POINT ( 'NONE',  ( 74.14312167556930433, 66.30466486950707861, 1.224646799147354045E-15 ) ) ;
#77306=CARTESIAN_POINT ( 'NONE',  ( 33.66714878060290772, 21.29860640527294180, -2.839279412974138328 ) ) ;
#77307=CARTESIAN_POINT ( 'NONE',  ( 69.85984440804038798, 64.57025534319816984, -12.75834560728216616 ) ) ;
#77308=CARTESIAN_POINT ( 'NONE',  ( 82.10359218643519341, 52.07680853587788050, 15.36587509554532538 ) ) ;
#77309=LINE ( 'NONE', #5912, #20213 ) ;
#77313=CARTESIAN_POINT ( 'NONE',  ( 72.37415438388894984, 71.90064624941815907, -5.324036893254605829 ) ) ;
#77314=CARTESIAN_POINT ( 'NONE',  ( 74.90236252610125689, 53.33673484778374529, -16.52890225279428549 ) ) ;
#77316=VECTOR ( 'NONE', #88175, 1000.000000000000114 ) ;
#77319=CARTESIAN_POINT ( 'NONE',  ( 73.63435323750927353, 69.71791780730768551, 10.06421556446032461 ) ) ;
#77320=CARTESIAN_POINT ( 'NONE',  ( 34.33172647011804912, 40.79752408145593989, -5.678558825948271327 ) ) ;
#77323=CARTESIAN_POINT ( 'NONE',  ( 85.04793144752866851, 49.76842598555752772, 13.42690168825988550 ) ) ;
#77325=CARTESIAN_POINT ( 'NONE',  ( 86.25376498619890242, 46.94328282020536136, -10.55339115541321604 ) ) ;
#77327=CARTESIAN_POINT ( 'NONE',  ( 84.49275162666286576, 50.19829916693547744, 13.87667126673719231 ) ) ;
#77331=CARTESIAN_POINT ( 'NONE',  ( 80.02357168100483875, 44.69250730557818940, 11.14898322769941608 ) ) ;
#77332=CARTESIAN_POINT ( 'NONE',  ( 81.25101512611533394, 55.44295246005403754, -16.34115372143416778 ) ) ;
#77338=CARTESIAN_POINT ( 'NONE',  ( 87.22262286821016630, 46.01322853962243897, -8.753954545221112937 ) ) ;
#77340=FACE_OUTER_BOUND ( 'NONE', #56111, .T. ) ;
#77341=CARTESIAN_POINT ( 'NONE',  ( 30.91633199877554716, 29.80066082961423746, 10.00000000000000533 ) ) ;
#77344=CARTESIAN_POINT ( 'NONE',  ( 82.33563566117209120, 40.89915267565207557, 1.012059201927479224 ) ) ;
#77352=CARTESIAN_POINT ( 'NONE',  ( 36.41018743920069056, 41.99752408145594273, 5.678558825948277544 ) ) ;
#77359=CARTESIAN_POINT ( 'NONE',  ( 73.89337880468768560, 68.29732366427398915, -11.63451623248603006 ) ) ;
#77360=CARTESIAN_POINT ( 'NONE',  ( 75.83733595332329003, 62.71011828194265547, -15.04395063225968165 ) ) ;
#77363=CARTESIAN_POINT ( 'NONE',  ( 73.34094528678892289, 66.77043691544750459, 12.11220508038992172 ) ) ;
#77370=ORIENTED_EDGE ( 'NONE', *, *, #50822, .F. ) ;
#77376=AXIS2_PLACEMENT_3D ( 'NONE', #79773, #64024, #55397 ) ;
#77380=CARTESIAN_POINT ( 'NONE',  ( 70.81620453278789284, 71.83147976216292818, -2.355153135381267582 ) ) ;
#77390=CARTESIAN_POINT ( 'NONE',  ( 87.83899792242847582, 44.00541668311378629, -1.848955303085625390 ) ) ;
#77393=CARTESIAN_POINT ( 'NONE',  ( 83.65644665907211674, 43.95837842834492903, 7.881347961145165115 ) ) ;
#77397=CARTESIAN_POINT ( 'NONE',  ( 82.41797270617800564, 53.48512899883142779, -15.75897339677477582 ) ) ;
#77399=CARTESIAN_POINT ( 'NONE',  ( 67.12731856515000572, 66.75179982629357767, 8.201365336552942864 ) ) ;
#77403=B_SPLINE_CURVE_WITH_KNOTS ( 'NONE', 3,
 ( #9405, #76801, #16497, #77308, #54992, #38790, #69696, #85971, #301, #23582, #54474, #16000, #46899, #57997, #96542, #87485 ),
 .UNSPECIFIED., .F., .F.,
 ( 4, 1, 2, 2, 2, 1, 2, 2, 4 ),
 ( 0.000000000000000000, 0.1250000000000010547, 0.1875000000000025258, 0.2500000000000039968, 0.5000000000000062172, 0.6250000000000067724, 0.6875000000000056621, 0.7500000000000046629, 1.000000000000000000 ),
 .UNSPECIFIED. ) ;
#77406=CARTESIAN_POINT ( 'NONE',  ( 84.86723485156080926, 50.00129088274004374, -13.21731324173513400 ) ) ;
#77408=CARTESIAN_POINT ( 'NONE',  ( 73.66743201189373735, 69.33122701867863213, -9.963040539579864685 ) ) ;
#77409=CARTESIAN_POINT ( 'NONE',  ( 76.07050809621944154, 51.21356314218704142, 16.11001018009165620 ) ) ;
#77415=CARTESIAN_POINT ( 'NONE',  ( 71.76351473723396168, 71.84897031608997509, 2.971691788643022303 ) ) ;
#77416=LINE ( 'NONE', #39873, #52972 ) ;
#77417=ADVANCED_FACE ( 'NONE', ( #82454 ), #15900, .T. ) ;
#77419=CIRCLE ( 'NONE', #27238, 0.5000000000000004441 ) ;
#77423=CARTESIAN_POINT ( 'NONE',  ( 88.08725135673812190, 43.63233996731285202, 0.09640656973314606915 ) ) ;
#77430=CARTESIAN_POINT ( 'NONE',  ( 29.82838080365165112, 20.14754757982091249, -5.678558825948275768 ) ) ;
#77432=CARTESIAN_POINT ( 'NONE',  ( 80.87570718637368827, 47.50421068166237859, -12.95331308923947056 ) ) ;
#77433=CARTESIAN_POINT ( 'NONE',  ( 14.33134397731654630, 13.98920272979924917, 7.433330006724137462 ) ) ;
#77435=CARTESIAN_POINT ( 'NONE',  ( 77.20655462988578677, 63.53086439471233859, 15.45977356242439349 ) ) ;
#77436=CARTESIAN_POINT ( 'NONE',  ( 82.72330532876915754, 53.96112743574217774, -15.47339361700331928 ) ) ;
#77441=CARTESIAN_POINT ( 'NONE',  ( 75.56006359584802112, 56.67736960126342183, -16.12308054916178079 ) ) ;
#77443=CARTESIAN_POINT ( 'NONE',  ( 87.72955037964742075, 45.02833699891566255, -6.646681420800613971 ) ) ;
#77448=CARTESIAN_POINT ( 'NONE',  ( 77.36024730155139650, 49.51677810190187756, 14.91251237265224638 ) ) ;
#77449=CARTESIAN_POINT ( 'NONE',  ( 82.88482919494256862, 53.69580434870785979, 15.74208873548984755 ) ) ;
#77453=CARTESIAN_POINT ( 'NONE',  ( 71.84509507049874344, 68.86203342550538764, -9.163320704559227536 ) ) ;
#77457=CARTESIAN_POINT ( 'NONE',  ( 79.56744450085628273, 46.24204545948038714, -13.19286817301344250 ) ) ;
#77462=PRODUCT_DEFINITION ( 'UNKNOWN', '', #99610, #39228 ) ;
#77463=CARTESIAN_POINT ( 'NONE',  ( 23.19008890107776821, 36.49540643055188838, 3.479690158560446702E-15 ) ) ;
#77464=CARTESIAN_POINT ( 'NONE',  ( 75.57971908217777468, 57.62099012794157460, 16.07717357865400842 ) ) ;
#77468=DIRECTION ( 'NONE',  ( 0.5000000000000014433, -0.8660254037844378194, 0.000000000000000000 ) ) ;
#77470=VERTEX_POINT ( 'NONE', #15972 ) ;
#77472=CARTESIAN_POINT ( 'NONE',  ( 67.75500653864465050, 65.62281390131039416, -10.81429207771451573 ) ) ;
#77486=ORIENTED_EDGE ( 'NONE', *, *, #10130, .T. ) ;
#77490=CARTESIAN_POINT ( 'NONE',  ( 66.43357910826331647, 67.89188047633619760, 6.623141227690268806 ) ) ;
#77492=CARTESIAN_POINT ( 'NONE',  ( 83.76824508872513775, 42.19076294718777831, -5.428203380119669852 ) ) ;
#77494=CARTESIAN_POINT ( 'NONE',  ( 77.36600796148924530, 49.13692148722834929, -14.77749963168140113 ) ) ;
#77495=CARTESIAN_POINT ( 'NONE',  ( 70.40095915148631889, 63.88372271459088836, 12.84393136659105572 ) ) ;
#77497=EDGE_LOOP ( 'NONE', ( #22986, #99911, #74629, #54041 ) ) ;
#77499=EDGE_LOOP ( 'NONE', ( #58542, #38742, #11756, #18470 ) ) ;
#77500=CARTESIAN_POINT ( 'NONE',  ( 15.68640692011977222, 32.55466486950700045, -1.111400068045478839E-16 ) ) ;
#77502=EDGE_LOOP ( 'NONE', ( #23471, #33390, #79789, #45406 ) ) ;
#77504=CARTESIAN_POINT ( 'NONE',  ( 76.39943616605862076, 51.65488121685059042, -16.16297552989059128 ) ) ;
#77513=CARTESIAN_POINT ( 'NONE',  ( 81.95226675463217703, 43.66151996434197713, -8.822569420014042763 ) ) ;
#77515=CARTESIAN_POINT ( 'NONE',  ( 28.94742091202107304, 40.21091486745862653, 7.012934429366973338E-14 ) ) ;
#77517=CARTESIAN_POINT ( 'NONE',  ( 72.44020731426283533, 70.76712560363094440, 7.696415609646560796 ) ) ;
#77518=CARTESIAN_POINT ( 'NONE',  ( 69.47694127934478558, 67.41711995099386456, -9.198496735959366788 ) ) ;
#77525=CARTESIAN_POINT ( 'NONE',  ( 83.61973431552902980, 52.33906237753651425, 14.75805511933742054 ) ) ;
#77531=CARTESIAN_POINT ( 'NONE',  ( 74.06178371959768469, 55.22988461276135297, 16.12358979270296189 ) ) ;
#77534=CARTESIAN_POINT ( 'NONE',  ( 29.94731862920856358, 22.45404122711134676, -8.090169943749478065 ) ) ;
#77545=CARTESIAN_POINT ( 'NONE',  ( 72.82956929615316710, 70.88121797294115822, -7.877017184599600874 ) ) ;
#77549=CARTESIAN_POINT ( 'NONE',  ( 36.01802474176511026, 21.76426979415091978, 3.090169943749476733 ) ) ;
#77550=CARTESIAN_POINT ( 'NONE',  ( 77.80683632129496630, 56.80414902711877545, 16.61016218681300316 ) ) ;
#77552=CARTESIAN_POINT ( 'NONE',  ( 80.96958682834429055, 55.96437743930621878, 16.09281336319931199 ) ) ;
#77554=CARTESIAN_POINT ( 'NONE',  ( 84.15650392679282277, 46.61449241044970648, 11.42639398603495948 ) ) ;
#77557=CARTESIAN_POINT ( 'NONE',  ( 37.86538501507694576, 37.56454794089044213, 10.00000000000000355 ) ) ;
#77560=CARTESIAN_POINT ( 'NONE',  ( 66.47763888060634940, 67.99612994687967671, 6.463816603905435443 ) ) ;
#77561=CARTESIAN_POINT ( 'NONE',  ( 28.38430345058481663, 38.16126292948897003, -6.180339887498951690 ) ) ;
#77564=VECTOR ( 'NONE', #97509, 1000.000000000000000 ) ;
#77570=CARTESIAN_POINT ( 'NONE',  ( 24.39888929631063519, 19.80170272979926693, 7.433330006724137462 ) ) ;
#77572=CARTESIAN_POINT ( 'NONE',  ( 71.73982542038400823, 59.04037670598220444, 15.36454711367335513 ) ) ;
#77577=CARTESIAN_POINT ( 'NONE',  ( 12.55777956335723644, 9.111106405272902720, -2.839279412974138328 ) ) ;
#77578=CARTESIAN_POINT ( 'NONE',  ( 75.29803635635754233, 53.62586610745756843, -16.53393874230848581 ) ) ;
#77580=CARTESIAN_POINT ( 'NONE',  ( 88.28488596560143264, 44.32818720243073329, 2.217326208295938628 ) ) ;
#77582=DIRECTION ( 'NONE',  ( -0.7691052716734824157, -0.08748735329025024432, -0.6331058711608398282 ) ) ;
#77583=FACE_OUTER_BOUND ( 'NONE', #55998, .T. ) ;
#77585=CARTESIAN_POINT ( 'NONE',  ( 77.05460391109571106, 63.75555097366715529, 14.97632912148298168 ) ) ;
#77591=CARTESIAN_POINT ( 'NONE',  ( 87.61103589779790468, 43.76214543387700218, -0.04131823639585689711 ) ) ;
#77596=CARTESIAN_POINT ( 'NONE',  ( 77.10733807873376122, 63.61886353868632682, 15.40965320646045100 ) ) ;
#77606=CARTESIAN_POINT ( 'NONE',  ( 31.76492312988469280, 26.84335787977765264, 9.188101187500006262 ) ) ;
#77609=ADVANCED_FACE ( 'NONE', ( #5764 ), #100030, .T. ) ;
#77623=EDGE_CURVE ( 'NONE', #47892, #89224, #52191, .T. ) ;
#77627=CARTESIAN_POINT ( 'NONE',  ( 69.03049085021430642, 65.53841201702186936, 10.92225791274772106 ) ) ;
#77629=CARTESIAN_POINT ( 'NONE',  ( 75.88013953913147702, 65.59923957098945380, 13.85558759313056143 ) ) ;
#77630=CARTESIAN_POINT ( 'NONE',  ( 69.90077517449054767, 65.54052102004983738, -11.37488096913896030 ) ) ;
#77631=CARTESIAN_POINT ( 'NONE',  ( 78.55989720566141443, 47.96478771419136677, 13.95455569139155827 ) ) ;
#77635=CARTESIAN_POINT ( 'NONE',  ( 70.22598590769381133, 65.16623735881336188, 11.86258439676588061 ) ) ;
#77636=CARTESIAN_POINT ( 'NONE',  ( 87.79271458260285499, 45.16522989489592987, -6.842624051142037089 ) ) ;
#77637=EDGE_CURVE ( 'NONE', #32407, #69987, #37746, .T. ) ;
#77641=CARTESIAN_POINT ( 'NONE',  ( 83.55324616867257248, 51.62071861895685743, -14.85649312488210860 ) ) ;
#77644=CARTESIAN_POINT ( 'NONE',  ( 80.32771389996757705, 57.94408260071152483, -16.24746918486167857 ) ) ;
#77645=CARTESIAN_POINT ( 'NONE',  ( 72.07419404290544662, 71.65773480557935216, 5.498832909113074763 ) ) ;
#77646=CARTESIAN_POINT ( 'NONE',  ( 74.60675634627781960, 67.01455260309188589, 12.52145295594442942 ) ) ;
#77654=CARTESIAN_POINT ( 'NONE',  ( 85.61207876059154387, 48.93336676014416753, -12.63415981529851884 ) ) ;
#77655=ORIENTED_EDGE ( 'NONE', *, *, #69283, .F. ) ;
#77656=CARTESIAN_POINT ( 'NONE',  ( 71.10485482541737667, 63.64399173889170669, 13.27423776213106876 ) ) ;
#77657=CARTESIAN_POINT ( 'NONE',  ( 87.66405103922522812, 44.36922529636178325, -4.037368063366974624 ) ) ;
#77659=CARTESIAN_POINT ( 'NONE',  ( 73.23245250435016374, 60.46961760979917244, 15.70485221038128287 ) ) ;
#77668=VERTEX_POINT ( 'NONE', #48258 ) ;
#77671=CARTESIAN_POINT ( 'NONE',  ( 19.84093639355121397, 13.58380873178786530, 6.180339887498953466 ) ) ;
#77672=VECTOR ( 'NONE', #74815, 1000.000000000000000 ) ;
#77675=CARTESIAN_POINT ( 'NONE',  ( 21.01819855373923929, 11.94473085651391564, 1.475505719884397138E-15 ) ) ;
#77685=CARTESIAN_POINT ( 'NONE',  ( 69.60656329481270177, 65.89280548041654129, 11.57311433810471435 ) ) ;
#77686=CARTESIAN_POINT ( 'NONE',  ( 66.52392041415761526, 68.84470833993178474, -4.415679280538202356 ) ) ;
#77691=CARTESIAN_POINT ( 'NONE',  ( 24.61059131263772670, 35.18502408145592852, 5.678558825948277544 ) ) ;
#77695=CARTESIAN_POINT ( 'NONE',  ( 71.47018505618770234, 71.90846791982409059, 3.715355237622318896 ) ) ;
#77696=CARTESIAN_POINT ( 'NONE',  ( 66.04017617576342047, 68.56661300442509344, 1.988326559363849055 ) ) ;
#77698=CARTESIAN_POINT ( 'NONE',  ( 7.127696690345725727, 16.06628583063839244, -9.188101187500006262 ) ) ;
#77701=CARTESIAN_POINT ( 'NONE',  ( 15.46199490364264406, 17.43085787977761925, -9.188101187500008038 ) ) ;
#77703=FACE_OUTER_BOUND ( 'NONE', #44806, .T. ) ;
#77705=CARTESIAN_POINT ( 'NONE',  ( 71.74013172673453198, 72.14163783910345273, 0.6028694846914187666 ) ) ;
#77709=CARTESIAN_POINT ( 'NONE',  ( 87.86298961015023679, 44.89260222163543546, 6.207647304897663254 ) ) ;
#77711=VERTEX_POINT ( 'NONE', #44503 ) ;
#77717=CARTESIAN_POINT ( 'NONE',  ( 69.62991599110473828, 67.28754920473278389, 10.19854214946012938 ) ) ;
#77721=CARTESIAN_POINT ( 'NONE',  ( 79.45404352011763649, 59.64539556637617324, -16.18188341986842005 ) ) ;
#77723=CARTESIAN_POINT ( 'NONE',  ( 69.41727946307592845, 62.73729316916369925, 13.77678217037445840 ) ) ;
#77733=CARTESIAN_POINT ( 'NONE',  ( 72.89193669360001593, 59.22924534911017957, 15.51103768891951695 ) ) ;
#77735=CARTESIAN_POINT ( 'NONE',  ( 71.40725718522095633, 71.90619859764527178, 1.119957492137431343 ) ) ;
#77739=CARTESIAN_POINT ( 'NONE',  ( 81.50752084980894097, 44.54043232651186912, 10.17210088699022918 ) ) ;
#77746=CARTESIAN_POINT ( 'NONE',  ( 81.73998748822677385, 54.58416966175224161, -16.14354867815247729 ) ) ;
#77747=CARTESIAN_POINT ( 'NONE',  ( 18.76490627030545610, 13.76004757982088655, 5.678558825948272215 ) ) ;
#77749=CARTESIAN_POINT ( 'NONE',  ( 80.01979875032591849, 57.54866692369599690, 16.59896302490740538 ) ) ;
#77757=ADVANCED_FACE ( 'NONE', ( #38400 ), #70821, .T. ) ;
#77759=CARTESIAN_POINT ( 'NONE',  ( 71.41016749218992743, 59.45273978182970609, 15.69346469599747174 ) ) ;
#77766=CARTESIAN_POINT ( 'NONE',  ( 82.42089004567290544, 40.96640717916999108, -1.235892450584623381 ) ) ;
#77767=CARTESIAN_POINT ( 'NONE',  ( 7.599693759758307188, 26.16126292948893806, -6.180339887498951690 ) ) ;
#77771=CARTESIAN_POINT ( 'NONE',  ( 75.84828732440915644, 65.60728826867935481, 13.84218333541264556 ) ) ;
#77782=EDGE_CURVE ( 'NONE', #48220, #96813, #85572, .T. ) ;
#77792=CARTESIAN_POINT ( 'NONE',  ( 80.50903874866318688, 57.12766137858866244, -16.22900141427163945 ) ) ;
#77801=CARTESIAN_POINT ( 'NONE',  ( 68.45082498735337140, 68.05190841428618853, 7.383510520589708470 ) ) ;
#77809=CARTESIAN_POINT ( 'NONE',  ( 14.38185574516869458, 23.70171378149918695, -9.188101187500004485 ) ) ;
#77812=CARTESIAN_POINT ( 'NONE',  ( 66.19292216254950745, 68.59989815790002865, 2.318610380053390596 ) ) ;
#77813=CARTESIAN_POINT ( 'NONE',  ( 86.53906990778989439, 43.21878081143324835, -0.5596625769422287622 ) ) ;
#77817=CARTESIAN_POINT ( 'NONE',  ( 45.41683807177152943, 29.14754757982093736, -5.678558825948275768 ) ) ;
#77818=CARTESIAN_POINT ( 'NONE',  ( 40.15112871924374360, 31.38052372038644577, 10.00000000000000533 ) ) ;
#77819=CARTESIAN_POINT ( 'NONE',  ( 81.50691414224651510, 55.96606086945440950, -16.03680236514553314 ) ) ;
#77822=LINE ( 'NONE', #32193, #50689 ) ;
#77825=CARTESIAN_POINT ( 'NONE',  ( 75.14966582671556239, 65.99894161753822175, 13.81944563728900377 ) ) ;
#77830=CARTESIAN_POINT ( 'NONE',  ( 73.20446552614963309, 69.86374744967437778, 9.599577609524185817 ) ) ;
#77831=CARTESIAN_POINT ( 'NONE',  ( 36.06377727768691699, 41.79752408145595410, -5.678558825948271327 ) ) ;
#77832=ORIENTED_EDGE ( 'NONE', *, *, #74704, .T. ) ;
#77838=CARTESIAN_POINT ( 'NONE',  ( 86.46583077919046900, 47.10391736892673009, -10.05241405704699353 ) ) ;
#77841=CARTESIAN_POINT ( 'NONE',  ( 85.42383634753986144, 44.41940826771883621, -7.937727123839215082 ) ) ;
#77843=DIRECTION ( 'NONE',  ( -0.8660254037844377084, -0.5000000000000014433, -0.000000000000000000 ) ) ;
#77847=CARTESIAN_POINT ( 'NONE',  ( 81.18434463996317163, 55.62183548715842107, 16.37412944077603782 ) ) ;
#77850=CARTESIAN_POINT ( 'NONE',  ( 78.31144745436395738, 49.34677990821563753, 14.65856222115218443 ) ) ;
#77853=CARTESIAN_POINT ( 'NONE',  ( 34.02846334099481140, 24.81029122506296503, 8.090169943749479842 ) ) ;
#77856=CARTESIAN_POINT ( 'NONE',  ( 75.51323141522172477, 65.35427051582675517, 13.87231131232226744 ) ) ;
#77859=B_SPLINE_CURVE_WITH_KNOTS ( 'NONE', 3,
 ( #99534, #51931, #60496, #53408, #30116, #43816, #60998, #5334, #21050, #82872, #36215, #36711, #67618, #29136, #60004, #21531, #75740, #37213, #30621, #76715, #68114, #91969, #91453, #99039, #52912, #22515, #14905, #83864, #82384, #12953, #7309, #14429, #45309, #38191, #20543, #100034, #74754, #89964, #23000, #85882, #78229, #47793, #38702, #24508, #40697, #46810 ),
 .UNSPECIFIED., .F., .F.,
 ( 4, 1, 2, 2, 1, 2, 2, 1, 1, 2, 2, 1, 1, 2, 2, 1, 1, 2, 2, 1, 1, 1, 2, 2, 1, 1, 1, 2, 2, 4 ),
 ( 0.000000000000000000, 0.06250000000000975608, 0.09375000000001376677, 0.1250000000000177913, 0.1875000000000250910, 0.2187500000000290601, 0.2500000000000330291, 0.3125000000000403011, 0.3437500000000449085, 0.3593750000000467959, 0.3750000000000486278, 0.4375000000000480727, 0.4687500000000481282, 0.4843750000000476286, 0.5000000000000470735, 0.5625000000000482947, 0.5937500000000489608, 0.6093750000000479616, 0.6250000000000469624, 0.6875000000000460743, 0.7187500000000449640, 0.7343750000000438538, 0.7421875000000432987, 0.7500000000000426326, 0.8125000000000284217, 0.8437500000000207612, 0.8593750000000167644, 0.8671875000000155431, 0.8750000000000143219, 1.000000000000000000 ),
 .UNSPECIFIED. ) ;
#77864=CARTESIAN_POINT ( 'NONE',  ( 42.15722797529793553, 32.84335787977767041, 9.188101187500006262 ) ) ;
#77866=ORIENTED_EDGE ( 'NONE', *, *, #21264, .T. ) ;
#77869=CARTESIAN_POINT ( 'NONE',  ( 81.74119788692269140, 59.14441083166271085, 0.000000000000000000 ) ) ;
#77872=CARTESIAN_POINT ( 'NONE',  ( 72.55405144367838943, 63.78809379931346513, 13.69945044486563468 ) ) ;
#77873=EDGE_CURVE ( 'NONE', #99249, #48842, #23114, .T. ) ;
#77874=CARTESIAN_POINT ( 'NONE',  ( 66.66373457531125268, 68.30566046464788599, 4.557399502277720060 ) ) ;
#77875=CARTESIAN_POINT ( 'NONE',  ( 77.99681166185179393, 50.47661464015640576, 15.62787934327010397 ) ) ;
#77878=AXIS2_PLACEMENT_3D ( 'NONE', #31956, #16764, #47655 ) ;
#77880=ORIENTED_EDGE ( 'NONE', *, *, #77063, .F. ) ;
#77882=CARTESIAN_POINT ( 'NONE',  ( 65.74496443904322973, 69.08459607026262006, -0.1437899284560469337 ) ) ;
#77884=DIRECTION ( 'NONE',  ( -0.8660254037844377084, -0.5000000000000014433, -0.000000000000000000 ) ) ;
#77899=B_SPLINE_CURVE_WITH_KNOTS ( 'NONE', 3,
 ( #97127, #89535, #90527, #20096, #21098, #36759, #62032, #78271, #14944, #45834 ),
 .UNSPECIFIED., .F., .F.,
 ( 4, 2, 2, 2, 4 ),
 ( 0.000000000000000000, 0.0002622400424272595238, 0.0005244800848545190476, 0.0007867201272817785172, 0.001048960169709038095 ),
 .UNSPECIFIED. ) ;
#77909=CARTESIAN_POINT ( 'NONE',  ( 78.27615213422006946, 56.24099877768735922, 16.18748323720173943 ) ) ;
#77911=CARTESIAN_POINT ( 'NONE',  ( 73.61134034488466682, 69.26824756038205066, -9.998744155463656469 ) ) ;
#77912=CARTESIAN_POINT ( 'NONE',  ( 75.99893621847269287, 51.39177364591706265, 15.66710071473398358 ) ) ;
#77914=CARTESIAN_POINT ( 'NONE',  ( 73.76584831522595209, 68.38082682530665579, 11.49424229391075514 ) ) ;
#77921=CARTESIAN_POINT ( 'NONE',  ( 88.01740701321664062, 43.99393894108155934, 0.5439121987275350456 ) ) ;
#77922=CARTESIAN_POINT ( 'NONE',  ( 10.80369284495069238, 14.43677371833799583, -10.00000000000000355 ) ) ;
#77928=CARTESIAN_POINT ( 'NONE',  ( 27.58635055662477598, 24.43085787977765122, -9.188101187500008038 ) ) ;
#77930=CARTESIAN_POINT ( 'NONE',  ( 80.23656086893576855, 47.63841505922916753, -13.26053850169819803 ) ) ;
#77931=CARTESIAN_POINT ( 'NONE',  ( 10.40777469057294091, 26.98502408145591502, -5.678558825948271327 ) ) ;
#77933=CARTESIAN_POINT ( 'NONE',  ( 77.14069742968855792, 63.65222853049024110, 15.02831949864487271 ) ) ;
#77936=CARTESIAN_POINT ( 'NONE',  ( 74.12249027442281601, 67.16814668724251192, 12.15174938425090012 ) ) ;
#77939=CARTESIAN_POINT ( 'NONE',  ( 74.89708722414906106, 56.88665470694825643, -16.07962807653123605 ) ) ;
#77940=CARTESIAN_POINT ( 'NONE',  ( 87.68902078672120126, 44.98529012857299136, -6.607530655827392074 ) ) ;
#77944=VERTEX_POINT ( 'NONE', #27224 ) ;
#77945=CARTESIAN_POINT ( 'NONE',  ( 77.37658274812778814, 49.21614173473252407, 15.31778251827114623 ) ) ;
#77947=ORIENTED_EDGE ( 'NONE', *, *, #9427, .F. ) ;
#77950=CARTESIAN_POINT ( 'NONE',  ( 69.95819854987405506, 68.88853697437434676, -7.495272743277247685 ) ) ;
#77954=CARTESIAN_POINT ( 'NONE',  ( 65.92723761088207368, 68.94945291059251247, -2.624861928015910895 ) ) ;
#77957=ORIENTED_EDGE ( 'NONE', *, *, #84044, .F. ) ;
#77958=CARTESIAN_POINT ( 'NONE',  ( 23.41017057962146097, 28.91421378149919619, 9.188101187500008038 ) ) ;
#77960=CARTESIAN_POINT ( 'NONE',  ( 75.07321287302792712, 66.36857194797330806, -13.14009733065324070 ) ) ;
#77967=CARTESIAN_POINT ( 'NONE',  ( 67.98680250238912492, 65.22133151511555127, -10.62698878092350085 ) ) ;
#77980=CARTESIAN_POINT ( 'NONE',  ( 77.84440724905273612, 61.40677674231441330, -16.14086307328630809 ) ) ;
#77985=CARTESIAN_POINT ( 'NONE',  ( 80.02753730852559499, 44.42912664858859273, -10.91029207558068670 ) ) ;
#77988=B_SPLINE_SURFACE_WITH_KNOTS ( 'NONE', 3, 1, ( 
 ( #45082, #28386 ),
 ( #98314, #76020 ),
 ( #66887, #35983 ),
 ( #6597, #99306 ),
 ( #44073, #5592 ),
 ( #5104, #36482 ),
 ( #74524, #60267 ),
 ( #59266, #6091 ),
 ( #97819, #20815 ),
 ( #13214, #67386 ),
 ( #68872, #83128 ),
 ( #52673, #29886 ),
 ( #83633, #28903 ),
 ( #59780, #75506 ),
 ( #90747, #7078 ),
 ( #53186, #61272 ),
 ( #15166, #60760 ),
 ( #21303, #52179 ),
 ( #91722, #22286 ),
 ( #13699, #37965 ),
 ( #44571, #84142 ),
 ( #14690, #45571 ),
 ( #30386, #22790 ),
 ( #8096, #10981 ),
 ( #2890, #69876 ),
 ( #46567, #7581 ),
 ( #77504, #38971 ),
 ( #18577, #85641 ),
 ( #88524, #16188 ),
 ( #489, #33786 ),
 ( #72798, #49455 ) ),
 .UNSPECIFIED., .F., .F., .F.,
 ( 4, 3, 3, 3, 3, 3, 3, 3, 3, 3, 4 ),
 ( 2, 2 ),
 ( 0.000000000000000000, 0.1122669598086537268, 0.2243161639709344568, 0.3396355846218790386, 0.4553962076584738838, 0.5677860799921967683, 0.6749047109689209067, 0.7773884377078009722, 0.8775581155833749314, 0.9782364162377522598, 1.000000000000000000 ),
 ( 0.000000000000000000, 1.000000000000000000 ),
 .UNSPECIFIED. ) ;
#77991=EDGE_CURVE ( 'NONE', #79111, #34466, #17017, .T. ) ;
#77996=ORIENTED_EDGE ( 'NONE', *, *, #27655, .T. ) ;
#77999=CARTESIAN_POINT ( 'NONE',  ( 24.22498904768565353, 14.39040679176983062, 1.333680081654574804E-15 ) ) ;
#78001=CARTESIAN_POINT ( 'NONE',  ( 75.92541454099094267, 65.74968322642241958, -14.18997729123868901 ) ) ;
#78004=CARTESIAN_POINT ( 'NONE',  ( 87.66889377758084834, 44.69705958948441094, 5.015779035299128275 ) ) ;
#78026=CARTESIAN_POINT ( 'NONE',  ( 73.59812156768246894, 55.56520137471197529, 16.10559722777662373 ) ) ;
#78028=CARTESIAN_POINT ( 'NONE',  ( 25.64360150771698343, 30.50829794293882102, -10.00000000000000355 ) ) ;
#78036=EDGE_CURVE ( 'NONE', #20756, #14203, #92252, .T. ) ;
#78043=AXIS2_PLACEMENT_3D ( 'NONE', #19570, #64649, #50430 ) ;
#78044=CARTESIAN_POINT ( 'NONE',  ( 29.16343140518078414, 25.03677371833803278, 10.00000000000000533 ) ) ;
#78045=CARTESIAN_POINT ( 'NONE',  ( 29.01663622185449753, 35.49103043416550918, -8.090169943749479842 ) ) ;
#78057=ADVANCED_FACE ( 'NONE', ( #46894 ), #69190, .T. ) ;
#78061=CARTESIAN_POINT ( 'NONE',  ( 74.14312167556930433, 66.30466486950707861, 1.224646799147354045E-15 ) ) ;
#78066=CARTESIAN_POINT ( 'NONE',  ( 24.68213521633936836, 16.11110640527292759, -2.839279412974138328 ) ) ;
#78071=CARTESIAN_POINT ( 'NONE',  ( 43.29939952211008602, 27.12755873383629890, -6.180339887498949025 ) ) ;
#78072=CARTESIAN_POINT ( 'NONE',  ( 12.38457448260035143, 9.011106405272903075, 2.839279412974134775 ) ) ;
#78073=DIRECTION ( 'NONE',  ( 0.8660254037844475894, 0.4999999999999846789, -0.000000000000000000 ) ) ;
#78074=CARTESIAN_POINT ( 'NONE',  ( 71.95199650962558735, 72.63932214931871556, -0.9219114722910072279 ) ) ;
#78075=CARTESIAN_POINT ( 'NONE',  ( 43.01983786573178037, 33.03677371833806120, 10.00000000000000533 ) ) ;
#78078=CARTESIAN_POINT ( 'NONE',  ( 72.24303396261568366, 71.49679634179437926, -5.037392375358459518 ) ) ;
#78080=CARTESIAN_POINT ( 'NONE',  ( 83.43773055803072225, 41.05266667205868458, 1.786701415307724750 ) ) ;
#78084=CARTESIAN_POINT ( 'NONE',  ( 84.90289089734821459, 42.76399680830722616, -3.660411970491889377 ) ) ;
#78088=CARTESIAN_POINT ( 'NONE',  ( 80.03143596134809457, 57.61873189500683878, 16.60059503390609592 ) ) ;
#78089=CARTESIAN_POINT ( 'NONE',  ( 77.27782791576461818, 63.42193016440150899, 15.51014190020122641 ) ) ;
#78096=CARTESIAN_POINT ( 'NONE',  ( 23.93942162470478863, 34.79752408145593989, -5.678558825948271327 ) ) ;
#78099=CYLINDRICAL_SURFACE ( 'NONE', #56291, 16.60714546451156792 ) ;
#78103=CARTESIAN_POINT ( 'NONE',  ( 24.67798091686682938, 37.18080186712595037, 3.090169943749475401 ) ) ;
#78106=B_SPLINE_CURVE_WITH_KNOTS ( 'NONE', 3,
 ( #11302, #10283, #18386, #73096, #49281, #95439, #58837, #96410, #26485, #42160 ),
 .UNSPECIFIED., .F., .F.,
 ( 4, 2, 2, 2, 4 ),
 ( 0.000000000000000000, 0.0002622400424272597406, 0.0005244800848545194813, 0.0007867201272817791677, 0.001048960169709038963 ),
 .UNSPECIFIED. ) ;
#78120=CARTESIAN_POINT ( 'NONE',  ( 69.45390216962655927, 66.50352562030866466, 10.22003932022287032 ) ) ;
#78122=CARTESIAN_POINT ( 'NONE',  ( 88.45958475239287111, 43.85926912372239883, -0.5941283661710258235 ) ) ;
#78124=CARTESIAN_POINT ( 'NONE',  ( 70.37752084497869021, 65.47563201637457553, -11.66932464330069230 ) ) ;
#78125=CARTESIAN_POINT ( 'NONE',  ( 77.94338102238666011, 47.97603164893081384, 14.13821563815946725 ) ) ;
#78127=ORIENTED_EDGE ( 'NONE', *, *, #84369, .T. ) ;
#78129=CARTESIAN_POINT ( 'NONE',  ( 78.92023586790456591, 59.45316570216661489, -16.52216786098997403 ) ) ;
#78134=CARTESIAN_POINT ( 'NONE',  ( 83.86143710801805184, 52.01156594317939152, -14.55893269640292154 ) ) ;
#78135=CARTESIAN_POINT ( 'NONE',  ( 69.31152416607949363, 65.05164803522899319, -11.50429494836084565 ) ) ;
#78137=FACE_OUTER_BOUND ( 'NONE', #60344, .T. ) ;
#78138=CARTESIAN_POINT ( 'NONE',  ( 71.94643353573425770, 71.53214566342799685, 5.625104812542582877 ) ) ;
#78147=CARTESIAN_POINT ( 'NONE',  ( 85.65277752055500571, 48.41186657597218357, -12.21575983946770450 ) ) ;
#78149=CARTESIAN_POINT ( 'NONE',  ( 71.98134248244618050, 66.42195643918441306, 11.72108357238321652 ) ) ;
#78154=B_SPLINE_CURVE_WITH_KNOTS ( 'NONE', 3,
 ( #38844, #39825, #77875, #63153, #23636, #9972, #16056, #70756, #55533, #25672, #86518, #62636, #86025, #17049, #1369, #33257 ),
 .UNSPECIFIED., .F., .F.,
 ( 4, 1, 2, 2, 2, 1, 2, 2, 4 ),
 ( 0.000000000000000000, 0.1250000000000033307, 0.1875000000000040523, 0.2500000000000047740, 0.5000000000000016653, 0.6250000000000000000, 0.6875000000000001110, 0.7500000000000002220, 1.000000000000000000 ),
 .UNSPECIFIED. ) ;
#78161=CARTESIAN_POINT ( 'NONE',  ( 87.87676930530868447, 44.78862430170916298, 4.932775619378069187 ) ) ;
#78164=CARTESIAN_POINT ( 'NONE',  ( 12.92385338608513301, 23.16454794089040092, -10.00000000000000355 ) ) ;
#78165=CARTESIAN_POINT ( 'NONE',  ( 83.51796290786062116, 48.89396064590803093, -13.43348588850899183 ) ) ;
#78167=CARTESIAN_POINT ( 'NONE',  ( 66.49317117068670768, 67.78108392186146602, -6.905541408637477119 ) ) ;
#78168=DIRECTION ( 'NONE',  ( 0.6793907169778423683, 0.000000000000000000, 0.7337767056021424761 ) ) ;
#78180=CARTESIAN_POINT ( 'NONE',  ( 28.84929788977513709, 34.84336893147758474, -7.433330006724137462 ) ) ;
#78187=CARTESIAN_POINT ( 'NONE',  ( 65.93175743083646978, 68.97510768830362338, 2.497091622996998161 ) ) ;
#78192=CARTESIAN_POINT ( 'NONE',  ( 13.72994409607376731, 16.43085787977761569, -9.188101187500008038 ) ) ;
#78194=B_SPLINE_CURVE_WITH_KNOTS ( 'NONE', 3,
 ( #47867, #71207, #7381, #76788, #32683, #63583, #94525, #53480, #84431, #100111, #14976, #30695, #19013, #27099, #64088, #72211 ),
 .UNSPECIFIED., .F., .F.,
 ( 4, 1, 2, 2, 2, 1, 2, 2, 4 ),
 ( 0.000000000000000000, 0.1249999999999962808, 0.1874999999999963363, 0.2499999999999963918, 0.4999999999999973355, 0.6249999999999973355, 0.6874999999999972244, 0.7499999999999970024, 1.000000000000000000 ),
 .UNSPECIFIED. ) ;
#78195=CARTESIAN_POINT ( 'NONE',  ( 69.47336484112540234, 62.61584900673512522, 13.29333455021356158 ) ) ;
#78200=DIRECTION ( 'NONE',  ( -0.8660254037844378194, -0.5000000000000014433, -0.000000000000000000 ) ) ;
#78207=CARTESIAN_POINT ( 'NONE',  ( 72.89440483270105631, 70.83506548046183582, 7.273745411891205492 ) ) ;
#78208=ORIENTED_EDGE ( 'NONE', *, *, #22608, .T. ) ;
#78214=VECTOR ( 'NONE', #47247, 1000.000000000000000 ) ;
#78215=CARTESIAN_POINT ( 'NONE',  ( 17.34117332728243355, 10.41603393254323962, -1.583844403245362020 ) ) ;
#78216=CARTESIAN_POINT ( 'NONE',  ( 81.17880017041383667, 48.14434756715330366, -13.80270438712140013 ) ) ;
#78217=CARTESIAN_POINT ( 'NONE',  ( 69.64850847652870414, 62.66264390746926694, 13.89643941053915022 ) ) ;
#78218=VERTEX_POINT ( 'NONE', #56982 ) ;
#78224=ORIENTED_EDGE ( 'NONE', *, *, #3840, .T. ) ;
#78229=CARTESIAN_POINT ( 'NONE',  ( 80.22712853404131295, 46.14526667274431304, 12.26665755571171701 ) ) ;
#78241=CARTESIAN_POINT ( 'NONE',  ( 19.86428432551159418, 29.65586893147756342, -7.433330006724137462 ) ) ;
#78244=FACE_OUTER_BOUND ( 'NONE', #67563, .T. ) ;
#78246=ADVANCED_FACE ( 'NONE', ( #29103 ), #36672, .T. ) ;
#78252=CARTESIAN_POINT ( 'NONE',  ( 84.30423139501758101, 45.69133797766890837, -9.735438995952875985 ) ) ;
#78255=ORIENTED_EDGE ( 'NONE', *, *, #41738, .T. ) ;
#78271=CARTESIAN_POINT ( 'NONE',  ( 67.28774071949871427, 67.22545272451772291, -8.569909696590800152 ) ) ;
#78275=CARTESIAN_POINT ( 'NONE',  ( 74.36956061611711277, 67.95497152727877221, -11.68736594047405930 ) ) ;
#78278=ORIENTED_EDGE ( 'NONE', *, *, #37953, .F. ) ;
#78285=CARTESIAN_POINT ( 'NONE',  ( 68.68909986772983700, 64.16576715822536414, -12.55144644528872533 ) ) ;
#78297=CARTESIAN_POINT ( 'NONE',  ( 74.35158511417792226, 58.53122306914246309, 16.30383169004117150 ) ) ;
#78302=CARTESIAN_POINT ( 'NONE',  ( 19.08966579672462061, 13.94754757982089188, 5.678558825948272215 ) ) ;
#78321=CARTESIAN_POINT ( 'NONE',  ( 85.19931647622364324, 44.72206782681810466, 8.604955222596291975 ) ) ;
#78324=CARTESIAN_POINT ( 'NONE',  ( 74.92485320761846879, 53.17783355571813075, -16.51377003329815096 ) ) ;
#78328=DIRECTION ( 'NONE',  ( -0.6758705274779434058, -0.2489746672676118044, 0.6936934806855752367 ) ) ;
#78329=CARTESIAN_POINT ( 'NONE',  ( 40.64525884627276042, 24.26216523072497466, -2.296566073217252530E-15 ) ) ;
#78331=CARTESIAN_POINT ( 'NONE',  ( 78.43012671350176390, 61.37287260322700888, 16.21548333613125337 ) ) ;
#78334=VERTEX_POINT ( 'NONE', #31065 ) ;
#78335=CARTESIAN_POINT ( 'NONE',  ( 86.17560058389634037, 46.94341623220315540, -10.60084123426474179 ) ) ;
#78338=CARTESIAN_POINT ( 'NONE',  ( 87.56148871955852542, 44.50103375289268826, -5.753754189115007023 ) ) ;
#78339=CARTESIAN_POINT ( 'NONE',  ( 37.70440764347101492, 39.95586893147758900, 7.433330006724141015 ) ) ;
#78340=CARTESIAN_POINT ( 'NONE',  ( 80.38494540807658950, 44.35137226082142803, 11.33962482632668944 ) ) ;
#78341=CARTESIAN_POINT ( 'NONE',  ( 84.83590989842353736, 50.19589791021755332, -13.76099895038702847 ) ) ;
#78347=CARTESIAN_POINT ( 'NONE',  ( 77.30283862971377573, 49.68973779529829216, -15.49743936997366411 ) ) ;
#78350=CARTESIAN_POINT ( 'NONE',  ( 86.92574391271591594, 45.77938117786232652, -8.666101563913320760 ) ) ;
#78358=CARTESIAN_POINT ( 'NONE',  ( 78.95260674202536677, 46.19732041717283977, 12.80077979390832610 ) ) ;
#78365=CARTESIAN_POINT ( 'NONE',  ( 70.62955678144575700, 60.80479719377109404, -15.06269029760223077 ) ) ;
#78367=EDGE_CURVE ( 'NONE', #32340, #25515, #60967, .T. ) ;
#78368=CARTESIAN_POINT ( 'NONE',  ( 85.74702290878657607, 48.70847181056628727, -12.40582123554878358 ) ) ;
#78375=CARTESIAN_POINT ( 'NONE',  ( 81.19662769710231487, 43.13455380257515515, 9.541327768654262798 ) ) ;
#78377=CARTESIAN_POINT ( 'NONE',  ( 26.41003172443570790, 38.18080186712595037, 3.090169943749475401 ) ) ;
#78396=B_SPLINE_CURVE_WITH_KNOTS ( 'NONE', 3,
 ( #49067, #73371, #10570, #3958, #34841, #87639, #72385, #25779, #33359, #10068 ),
 .UNSPECIFIED., .F., .F.,
 ( 4, 2, 2, 2, 4 ),
 ( 0.000000000000000000, 0.0002622400424272591985, 0.0005244800848545183971, 0.0007867201272817776498, 0.001048960169709036794 ),
 .UNSPECIFIED. ) ;
#78399=CARTESIAN_POINT ( 'NONE',  ( 73.78595477147815984, 68.43622263357737268, 11.45456581244436123 ) ) ;
#78410=CARTESIAN_POINT ( 'NONE',  ( 84.65037625111526154, 50.51595192201220641, -13.58046508661252894 ) ) ;
#78411=CARTESIAN_POINT ( 'NONE',  ( 78.12758897056819762, 61.89708633492155343, 15.71247334545933505 ) ) ;
#78412=DIRECTION ( 'NONE',  ( -0.5000000000000014433, 0.8660254037844379305, 0.000000000000000000 ) ) ;
#78425=VECTOR ( 'NONE', #50755, 1000.000000000000114 ) ;
#78426=CARTESIAN_POINT ( 'NONE',  ( 88.14558033319170249, 43.66656252067526367, 0.1579512601322911325 ) ) ;
#78428=CARTESIAN_POINT ( 'NONE',  ( 9.265696904164599346, 17.30066082961419838, -10.00000000000000533 ) ) ;
#78429=DIRECTION ( 'NONE',  ( 0.000000000000000000, 0.5247752241695049502, 0.8512408378936280329 ) ) ;
#78432=CARTESIAN_POINT ( 'NONE',  ( 33.29248241878940462, 22.14754757982091604, -5.678558825948275768 ) ) ;
#78435=CARTESIAN_POINT ( 'NONE',  ( 14.92192532440567199, 20.56628583063839955, 9.188101187500006262 ) ) ;
#78437=CARTESIAN_POINT ( 'NONE',  ( 76.92045831404706746, 63.69682018499118925, 15.34400990693822564 ) ) ;
#78444=CARTESIAN_POINT ( 'NONE',  ( 78.54737301421290852, 55.66250919272829378, -16.12479227928217540 ) ) ;
#78449=CARTESIAN_POINT ( 'NONE',  ( 77.47838539169265459, 49.59694670388121551, 14.91689290702275983 ) ) ;
#78451=ORIENTED_EDGE ( 'NONE', *, *, #57248, .T. ) ;
#78458=CARTESIAN_POINT ( 'NONE',  ( 72.46567298678348834, 71.74231227323613780, 5.836615459846345999 ) ) ;
#78462=CARTESIAN_POINT ( 'NONE',  ( 25.06043674821822265, 32.65586893147757053, -7.433330006724137462 ) ) ;
#78463=CARTESIAN_POINT ( 'NONE',  ( 79.99303828038561903, 44.39269627614997660, 11.58267821196168157 ) ) ;
#78465=CARTESIAN_POINT ( 'NONE',  ( 75.32876355654416045, 66.66275840934527253, -13.04208647660080089 ) ) ;
#78466=CARTESIAN_POINT ( 'NONE',  ( 78.41488460546182182, 49.53322450150187706, -14.69929798244788266 ) ) ;
#78473=CARTESIAN_POINT ( 'NONE',  ( 68.26378387136982440, 65.68578065247751852, -10.31175839017903328 ) ) ;
#78476=CARTESIAN_POINT ( 'NONE',  ( 19.62422909362874535, 11.73415679381821342, 1.333680081654574804E-15 ) ) ;
#78479=CARTESIAN_POINT ( 'NONE',  ( 70.20948996332299430, 63.06637520435538846, -13.85461378616484041 ) ) ;
#78490=CARTESIAN_POINT ( 'NONE',  ( 80.11111641639102743, 44.89713496294027095, -11.28635903916993932 ) ) ;
#78491=EDGE_CURVE ( 'NONE', #64537, #16291, #89570, .T. ) ;
#78494=CARTESIAN_POINT ( 'NONE',  ( 81.37739665788856769, 55.81704345181816507, 16.38624498997419110 ) ) ;
#78495=CARTESIAN_POINT ( 'NONE',  ( 83.00813062480057170, 47.72000278234192194, -12.31777161607909044 ) ) ;
#78504=AXIS2_PLACEMENT_3D ( 'NONE', #91787, #58838, #75568 ) ;
#78505=CARTESIAN_POINT ( 'NONE',  ( 76.08373593127036827, 64.71300453985560353, -14.35646715271085405 ) ) ;
#78508=CARTESIAN_POINT ( 'NONE',  ( 87.80215979260032100, 44.26138434534234278, 4.729176973005307261 ) ) ;
#78511=CARTESIAN_POINT ( 'NONE',  ( 40.95666657127031840, 28.81029122506297924, 8.090169943749479842 ) ) ;
#78517=DIRECTION ( 'NONE',  ( -0.2649596321165964552, 0.4589235447807054058, -0.8480480961564325071 ) ) ;
#78523=CARTESIAN_POINT ( 'NONE',  ( 84.07138645536940658, 51.57118087273711637, 14.70185406139691153 ) ) ;
#78524=EDGE_CURVE ( 'NONE', #59341, #25263, #58461, .T. ) ;
#78526=ORIENTED_EDGE ( 'NONE', *, *, #86296, .T. ) ;
#78531=CARTESIAN_POINT ( 'NONE',  ( 73.66928586354876529, 55.48613233660923072, 16.58448172204914783 ) ) ;
#78533=CARTESIAN_POINT ( 'NONE',  ( 23.53456118939196529, 35.36126292948896577, 6.180339887498949913 ) ) ;
#78540=CARTESIAN_POINT ( 'NONE',  ( 82.24012673451345279, 47.97130509467530857, 12.79208699616589229 ) ) ;
#78544=CARTESIAN_POINT ( 'NONE',  ( 81.59255471807858839, 41.71843698051294780, 5.901189277464562011 ) ) ;
#78547=CARTESIAN_POINT ( 'NONE',  ( 37.16144446923997435, 23.58380873178789727, 6.180339887498953466 ) ) ;
#78550=CARTESIAN_POINT ( 'NONE',  ( 80.98395585398840524, 56.01611329191965893, 16.09912269941438723 ) ) ;
#78552=CARTESIAN_POINT ( 'NONE',  ( 85.04793144752866851, 49.76842598555752772, 13.42690168825988550 ) ) ;
#78567=CARTESIAN_POINT ( 'NONE',  ( 67.01770718203071908, 66.86662898352919626, -8.855153707138468278 ) ) ;
#78569=CARTESIAN_POINT ( 'NONE',  ( 17.89217828605986327, 10.73415679381820986, 1.333680081654574804E-15 ) ) ;
#78572=CARTESIAN_POINT ( 'NONE',  ( 27.97303175072023151, 18.01110640527293327, 2.839279412974134775 ) ) ;
#78576=EDGE_LOOP ( 'NONE', ( #5480, #60651, #96722, #51016 ) ) ;
#78578=CARTESIAN_POINT ( 'NONE',  ( 16.39654754030849659, 10.26216523072493203, -2.296566073217252530E-15 ) ) ;
#78580=CARTESIAN_POINT ( 'NONE',  ( 75.74547564527691179, 59.01063491041397668, -15.93052030936962460 ) ) ;
#78584=CARTESIAN_POINT ( 'NONE',  ( 72.34691042023506213, 71.90931229659582868, -5.260778230539377098 ) ) ;
#78586=CARTESIAN_POINT ( 'NONE',  ( 85.13065436355927318, 49.01193835628323114, 12.45131667738069225 ) ) ;
#78591=CARTESIAN_POINT ( 'NONE',  ( 82.36190372195099485, 42.31745646093239088, -6.261288449950242807 ) ) ;
#78592=ORIENTED_EDGE ( 'NONE', *, *, #87623, .T. ) ;
#78593=CARTESIAN_POINT ( 'NONE',  ( 66.14792423582534298, 68.51351281792520354, -2.683414512432761079 ) ) ;
#78594=CARTESIAN_POINT ( 'NONE',  ( 71.67184923690800247, 72.06465046553262255, -3.547063142499712551 ) ) ;
#78595=CARTESIAN_POINT ( 'NONE',  ( 72.95830788359974406, 56.77128196665827176, -15.96545419981961267 ) ) ;
#78599=ORIENTED_EDGE ( 'NONE', *, *, #49987, .T. ) ;
#78603=CARTESIAN_POINT ( 'NONE',  ( 28.52453836335597614, 34.65586893147758474, -7.433330006724137462 ) ) ;
#78605=CARTESIAN_POINT ( 'NONE',  ( 78.26988008674611308, 47.94124790171424877, -14.02519726671745737 ) ) ;
#78607=CARTESIAN_POINT ( 'NONE',  ( 74.32474745866193189, 68.52230083288840490, 11.15590001247776364 ) ) ;
#78623=ADVANCED_FACE ( 'NONE', ( #28752 ), #69270, .T. ) ;
#78627=CARTESIAN_POINT ( 'NONE',  ( 71.54698464547352899, 65.28335351056534819, -12.36203232579594236 ) ) ;
#78630=ORIENTED_EDGE ( 'NONE', *, *, #84131, .F. ) ;
#78638=CARTESIAN_POINT ( 'NONE',  ( 83.79506744998815293, 51.52028683484932259, -14.36816095265300319 ) ) ;
#78644=CARTESIAN_POINT ( 'NONE',  ( 74.58922631747107346, 66.95469429158355013, 12.55546573254312470 ) ) ;
#78651=CARTESIAN_POINT ( 'NONE',  ( 85.39636071719610300, 48.32640963909398124, -12.26545443191637297 ) ) ;
#78652=EDGE_LOOP ( 'NONE', ( #91882, #61313, #435, #66758 ) ) ;
#78653=CARTESIAN_POINT ( 'NONE',  ( 72.13197559556067517, 66.88302471189031451, 11.41260966439740798 ) ) ;
#78655=CARTESIAN_POINT ( 'NONE',  ( 67.66566145506487828, 69.67521865087169886, -0.2583700242925219270 ) ) ;
#78664=CARTESIAN_POINT ( 'NONE',  ( 87.96858562469613219, 44.79953861350612954, 4.806926248663378587 ) ) ;
#78667=CARTESIAN_POINT ( 'NONE',  ( 19.84093639355121397, 13.58380873178786707, 6.180339887498953466 ) ) ;
#78670=CARTESIAN_POINT ( 'NONE',  ( 72.02976470237955198, 59.30830629416841759, -15.33705471575644808 ) ) ;
#78672=CARTESIAN_POINT ( 'NONE',  ( 12.69602586335324190, 7.734156793818200981, -2.889640176918245968E-15 ) ) ;
#78685=CARTESIAN_POINT ( 'NONE',  ( 24.26418115112394247, 34.98502408145593279, -5.678558825948271327 ) ) ;
#78688=EDGE_CURVE ( 'NONE', #71267, #57136, #73921, .T. ) ;
#78692=CARTESIAN_POINT ( 'NONE',  ( 65.81576594865798313, 68.96196425835729826, 2.168796872202445769 ) ) ;
#78698=CARTESIAN_POINT ( 'NONE',  ( 8.146472837920740062, 20.10171378149916777, 9.188101187500008038 ) ) ;
#78700=AXIS2_PLACEMENT_3D ( 'NONE', #27808, #58683, #43982 ) ;
#78706=CARTESIAN_POINT ( 'NONE',  ( 87.89611104468033886, 44.97730679797473385, 6.346758332113883405 ) ) ;
#78711=CARTESIAN_POINT ( 'NONE',  ( 85.97987434235641047, 47.62252706626447463, 10.87664434560344340 ) ) ;
#78714=CARTESIAN_POINT ( 'NONE',  ( 73.75461245277466560, 71.97758258259658248, 0.000000000000000000 ) ) ;
#78716=CARTESIAN_POINT ( 'NONE',  ( 68.90560621877192204, 63.79076715805910425, -12.30144644517788421 ) ) ;
#78718=CARTESIAN_POINT ( 'NONE',  ( 12.17791779510973171, 30.52903772873356658, -1.583844403245363575 ) ) ;
#78719=VERTEX_POINT ( 'NONE', #63136 ) ;
#78723=CARTESIAN_POINT ( 'NONE',  ( 38.08795742478228163, 27.15404122711136381, 8.090169943749479842 ) ) ;
#78728=CARTESIAN_POINT ( 'NONE',  ( 73.68192328755300480, 62.65634618987721183, 14.56402732850078152 ) ) ;
#78731=EDGE_LOOP ( 'NONE', ( #12549, #35490, #33369, #89001 ) ) ;
#78732=CARTESIAN_POINT ( 'NONE',  ( 81.96249893094650929, 45.51685736730845377, 10.90602769004302530 ) ) ;
#78733=CARTESIAN_POINT ( 'NONE',  ( 71.28049052964838950, 69.11027213759044230, 8.374494312738244517 ) ) ;
#78740=B_SPLINE_CURVE_WITH_KNOTS ( 'NONE', 3,
 ( #86445, #46880, #9385, #54974, #38262, #69175, #53962, #85951, #84919, #55459, #47374, #78297, #15463, #46360, #8881, #39749 ),
 .UNSPECIFIED., .F., .F.,
 ( 4, 1, 2, 2, 2, 1, 2, 2, 4 ),
 ( 0.000000000000000000, 0.1250000000000003053, 0.1875000000000004441, 0.2500000000000006106, 0.4999999999999976130, 0.6249999999999962252, 0.6874999999999963363, 0.7499999999999964473, 1.000000000000000000 ),
 .UNSPECIFIED. ) ;
#78741=CARTESIAN_POINT ( 'NONE',  ( 23.25741983583088413, 25.37878583063841376, 9.188101187500006262 ) ) ;
#78743=EDGE_CURVE ( 'NONE', #65907, #96690, #94081, .T. ) ;
#78744=DIRECTION ( 'NONE',  ( 0.1378186779084994706, -0.2387089523694924387, -0.9612616959383186721 ) ) ;
#78746=VERTEX_POINT ( 'NONE', #78862 ) ;
#78747=VECTOR ( 'NONE', #92592, 1000.000000000000114 ) ;
#78755=VERTEX_POINT ( 'NONE', #77856 ) ;
#78757=CARTESIAN_POINT ( 'NONE',  ( 75.00762831775021766, 66.90256318391983825, -13.19391308334217605 ) ) ;
#78762=CARTESIAN_POINT ( 'NONE',  ( 82.34414259798680291, 40.36743405348067881, -1.213300603182490001 ) ) ;
#78766=CARTESIAN_POINT ( 'NONE',  ( 75.88363445057348144, 65.49265179502715739, 14.31053417012051554 ) ) ;
#78768=VECTOR ( 'NONE', #9758, 1000.000000000000114 ) ;
#78770=AXIS2_PLACEMENT_3D ( 'NONE', #2741, #72136, #94958 ) ;
#78772=ORIENTED_EDGE ( 'NONE', *, *, #89022, .T. ) ;
#78774=CARTESIAN_POINT ( 'NONE',  ( 81.50940192328098988, 59.54589321767952725, 0.1873032967079516220 ) ) ;
#78776=CARTESIAN_POINT ( 'NONE',  ( 84.12407613425114050, 43.74822318919484587, 7.135943603182840711 ) ) ;
#78778=CARTESIAN_POINT ( 'NONE',  ( 82.30424563670493399, 42.66182458811155698, 6.991864634221377273 ) ) ;
#78787=CARTESIAN_POINT ( 'NONE',  ( 66.50871531961365690, 67.78145361369897159, -6.921353532618302218 ) ) ;
#78802=CARTESIAN_POINT ( 'NONE',  ( 9.796739006517501736, 23.84336893147754566, -7.433330006724137462 ) ) ;
#78810=CARTESIAN_POINT ( 'NONE',  ( 29.85841906089621389, 18.20801979619929867, -3.090169943749474069 ) ) ;
#78815=CARTESIAN_POINT ( 'NONE',  ( 67.41069134358542669, 70.04696837240071261, -4.305487806446024446E-08 ) ) ;
#78818=CARTESIAN_POINT ( 'NONE',  ( 25.95703985525452850, 15.39040679176983240, 1.333680081654574804E-15 ) ) ;
#78823=CARTESIAN_POINT ( 'NONE',  ( 72.13210804887378913, 72.31988279945024090, 1.151498749227306995 ) ) ;
#78825=CARTESIAN_POINT ( 'NONE',  ( 78.91779975210128839, 49.13212207373893392, 14.41565681662890341 ) ) ;
#78832=CARTESIAN_POINT ( 'NONE',  ( 39.89592612264573290, 25.96004757982093025, -5.678558825948276656 ) ) ;
#78839=CARTESIAN_POINT ( 'NONE',  ( 86.44990779080247023, 47.08395378219080385, -10.04107686951885192 ) ) ;
#78842=CARTESIAN_POINT ( 'NONE',  ( 17.74977768659132593, 33.18080186712593616, 3.090169943749475401 ) ) ;
#78844=CARTESIAN_POINT ( 'NONE',  ( 85.82777105212227298, 44.89325558436473784, -8.300099996375795541 ) ) ;
#78846=CARTESIAN_POINT ( 'NONE',  ( 80.16024689640217105, 44.74056149942663296, 11.12043925283496115 ) ) ;
#78847=CARTESIAN_POINT ( 'NONE',  ( 84.86414386349152039, 49.99136666923657657, -13.21250203946878621 ) ) ;
#78853=CARTESIAN_POINT ( 'NONE',  ( 77.15726504878196579, 49.33124488487003845, -15.40379270228043573 ) ) ;
#78860=CARTESIAN_POINT ( 'NONE',  ( 71.54202820451581601, 72.24755327463289234, 2.386327895633298279 ) ) ;
#78862=CARTESIAN_POINT ( 'NONE',  ( 80.44297273216874089, 44.73620253192707708, -11.65665792466250039 ) ) ;
#78870=CARTESIAN_POINT ( 'NONE',  ( 40.74993669414823927, 32.03085787977766330, 9.188101187500006262 ) ) ;
#78873=CARTESIAN_POINT ( 'NONE',  ( 85.46624767806203238, 43.53765940098641352, -6.277485798516380555 ) ) ;
#78874=EDGE_LOOP ( 'NONE', ( #81119, #8316, #72121, #86877 ) ) ;
#78887=CARTESIAN_POINT ( 'NONE',  ( 65.75369581714585365, 69.08918575267863105, -0.1828176307183302651 ) ) ;
#78888=ORIENTED_EDGE ( 'NONE', *, *, #75850, .T. ) ;
#78899=ORIENTED_EDGE ( 'NONE', *, *, #14534, .T. ) ;
#78907=CARTESIAN_POINT ( 'NONE',  ( 85.02612526452620045, 46.67130807634502077, 10.38696136103375878 ) ) ;
#78911=CARTESIAN_POINT ( 'NONE',  ( 74.39841895140679640, 68.21392270468032848, 11.45628786500076579 ) ) ;
#78915=CARTESIAN_POINT ( 'NONE',  ( 70.00074031614300907, 71.54231853062985635, 1.101452585462014300 ) ) ;
#78920=CARTESIAN_POINT ( 'NONE',  ( 78.09662876767376360, 55.14805409318260843, 16.10810231782577873 ) ) ;
#78929=CARTESIAN_POINT ( 'NONE',  ( 80.74974841587442143, 43.27611110060701805, 10.01619596027649806 ) ) ;
#78930=CARTESIAN_POINT ( 'NONE',  ( 80.38505107983586129, 54.19253253477483412, -15.81918041010719023 ) ) ;
#78931=CARTESIAN_POINT ( 'NONE',  ( 27.81076257310190769, 39.55466486950702176, 7.012934429366973338E-14 ) ) ;
#78935=CARTESIAN_POINT ( 'NONE',  ( 77.05176924353446566, 63.79896054814203410, -15.33469885150045542 ) ) ;
#78938=CARTESIAN_POINT ( 'NONE',  ( 88.48828274770076519, 43.87397573844135934, -0.5490789642627272871 ) ) ;
#78944=EDGE_CURVE ( 'NONE', #16883, #57886, #95502, .T. ) ;
#78945=CARTESIAN_POINT ( 'NONE',  ( 31.05045217176252237, 26.43085787977764767, -9.188101187500008038 ) ) ;
#78949=CARTESIAN_POINT ( 'NONE',  ( 13.12254358208367400, 30.68290643055187061, 3.479690158560446702E-15 ) ) ;
#78958=CARTESIAN_POINT ( 'NONE',  ( 87.47063030522556915, 45.04046199688875163, -6.105227862096588964 ) ) ;
#78963=CARTESIAN_POINT ( 'NONE',  ( 77.55626133878480744, 49.73613333205595666, 14.95107568548285215 ) ) ;
#78969=CARTESIAN_POINT ( 'NONE',  ( 71.29390400445934972, 68.89192637807246911, -8.686554677171336891 ) ) ;
#78973=CARTESIAN_POINT ( 'NONE',  ( 65.83400234654939709, 68.92279781603272681, -2.474918377774905753 ) ) ;
#78979=CARTESIAN_POINT ( 'NONE',  ( 25.14222138719033595, 29.91421378149919619, 9.188101187500008038 ) ) ;
#78980=CARTESIAN_POINT ( 'NONE',  ( 74.93795995569031732, 66.37748476621555938, -13.08215655857838655 ) ) ;
#78981=CARTESIAN_POINT ( 'NONE',  ( 80.44963597398161426, 49.01439875558640580, -13.96582802915731492 ) ) ;
#78989=CARTESIAN_POINT ( 'NONE',  ( 67.65051319695646725, 65.91095239435391306, 10.45228776382301383 ) ) ;
#78999=ORIENTED_EDGE ( 'NONE', *, *, #53625, .T. ) ;
#79005=ORIENTED_EDGE ( 'NONE', *, *, #5707, .F. ) ;
#79006=CARTESIAN_POINT ( 'NONE',  ( 80.31904029099077036, 44.94024336421264820, -11.21917720938367324 ) ) ;
#79010=CARTESIAN_POINT ( 'NONE',  ( 83.79842386373591978, 47.52858511108933470, -11.83496612566354855 ) ) ;
#79014=VERTEX_POINT ( 'NONE', #80139 ) ;
#79019=CARTESIAN_POINT ( 'NONE',  ( 76.21739704791244208, 64.80718227787073715, -14.34818600867717464 ) ) ;
#79025=CARTESIAN_POINT ( 'NONE',  ( 80.73870607681467959, 45.87205857520788044, 11.81702607854560050 ) ) ;
#79036=DIRECTION ( 'NONE',  ( -0.5000000000000016653, 0.8660254037844375974, 0.000000000000000000 ) ) ;
#79039=CARTESIAN_POINT ( 'NONE',  ( 77.88662807442577218, 62.02336507127854759, 15.65480789639172876 ) ) ;
#79046=CARTESIAN_POINT ( 'NONE',  ( 72.63029380029557558, 64.40628814066955954, -13.38103629891480217 ) ) ;
#79048=CARTESIAN_POINT ( 'NONE',  ( 73.94500316957324060, 55.09575893527664192, 16.60253717196292200 ) ) ;
#79050=CARTESIAN_POINT ( 'NONE',  ( 28.39959312520600676, 35.13478043621390157, 8.090169943749478065 ) ) ;
#79058=VECTOR ( 'NONE', #8779, 1000.000000000000114 ) ;
#79061=CARTESIAN_POINT ( 'NONE',  ( 82.93874205646059750, 50.87638965249802681, 14.26819964912884231 ) ) ;
#79065=CARTESIAN_POINT ( 'NONE',  ( 34.63914548426571116, 22.12755873383627758, -6.180339887498949025 ) ) ;
#79066=CARTESIAN_POINT ( 'NONE',  ( 82.32963097709573219, 41.38348250535303663, 5.483832747226924376 ) ) ;
#79069=CARTESIAN_POINT ( 'NONE',  ( 81.50343375784891009, 59.55623038343588149, -0.1545084971874786939 ) ) ;
#79070=CARTESIAN_POINT ( 'NONE',  ( 35.05240415091495976, 28.43677371833803846, -10.00000000000000355 ) ) ;
#79079=CARTESIAN_POINT ( 'NONE',  ( 83.82185059330514321, 51.95230014857059331, 14.93193377595571825 ) ) ;
#79089=CARTESIAN_POINT ( 'NONE',  ( 67.13884004924136661, 66.79719628306519041, -9.043772424411733013 ) ) ;
#79091=FACE_OUTER_BOUND ( 'NONE', #59984, .T. ) ;
#79092=CARTESIAN_POINT ( 'NONE',  ( 69.12672858200174630, 64.33651235087042153, -11.97836756590942997 ) ) ;
#79094=CARTESIAN_POINT ( 'NONE',  ( 23.56475526289127842, 35.64646525600391413, -2.839279412974133887 ) ) ;
#79099=CARTESIAN_POINT ( 'NONE',  ( 6.007877864960585512, 21.65586893147753855, -7.433330006724137462 ) ) ;
#79101=CARTESIAN_POINT ( 'NONE',  ( 77.22652224754085637, 58.45676704727122797, -16.12585536898887284 ) ) ;
#79105=CARTESIAN_POINT ( 'NONE',  ( 72.48187990437281769, 71.22453042848766813, -6.074313086633869929 ) ) ;
#79106=DIRECTION ( 'NONE',  ( 0.5000000000000014433, -0.8660254037844378194, 0.000000000000000000 ) ) ;
#79111=VERTEX_POINT ( 'NONE', #74514 ) ;
#79114=CARTESIAN_POINT ( 'NONE',  ( 82.48583416037470784, 42.33184412569765698, -6.146425681634053895 ) ) ;
#79116=CARTESIAN_POINT ( 'NONE',  ( 38.46077748372667315, 37.90829794293884447, 10.00000000000000355 ) ) ;
#79119=CARTESIAN_POINT ( 'NONE',  ( 72.70720764797087554, 57.09321477475226914, -15.89700010401374364 ) ) ;
#79131=CARTESIAN_POINT ( 'NONE',  ( 34.90123498099573851, 22.01110640527294393, 2.839279412974134775 ) ) ;
#79133=CARTESIAN_POINT ( 'NONE',  ( 78.30023004233427741, 47.96220519360661427, -14.02684811912188323 ) ) ;
#79136=CARTESIAN_POINT ( 'NONE',  ( 73.81469611240122219, 68.48838210847161179, 11.42215486908103728 ) ) ;
#79142=CARTESIAN_POINT ( 'NONE',  ( 74.14148900092213523, 58.70489250135918979, -15.78255431708223888 ) ) ;
#79147=CARTESIAN_POINT ( 'NONE',  ( 71.27247878601987452, 69.85383392380222745, -7.214268055942345548 ) ) ;
#79155=CARTESIAN_POINT ( 'NONE',  ( 67.31665553791867751, 66.91278932699420068, 9.026460761065990823 ) ) ;
#79156=CARTESIAN_POINT ( 'NONE',  ( 75.09035324708760584, 64.38728148916531779, -14.18083448766436128 ) ) ;
#79161=LINE ( 'NONE', #48216, #49750 ) ;
#79166=CARTESIAN_POINT ( 'NONE',  ( 83.75130605492059033, 51.70531176359354220, -14.84358514963803977 ) ) ;
#79167=PLANE ( 'NONE',  #14659 ) ;
#79168=ORIENTED_EDGE ( 'NONE', *, *, #44925, .F. ) ;
#79169=CARTESIAN_POINT ( 'NONE',  ( 80.38256674825400694, 58.04436476229781761, -16.60504034864360179 ) ) ;
#79172=CARTESIAN_POINT ( 'NONE',  ( 78.30955769916531040, 61.43963167811126169, 15.82323565659766373 ) ) ;
#79176=CARTESIAN_POINT ( 'NONE',  ( 81.74119788692269140, 59.14441083166271085, 0.000000000000000000 ) ) ;
#79178=CARTESIAN_POINT ( 'NONE',  ( 85.57719226846251104, 48.31999287754577210, -11.71062333427767044 ) ) ;
#79180=LINE ( 'NONE', #8737, #78768 ) ;
#79184=B_SPLINE_CURVE_WITH_KNOTS ( 'NONE', 3,
 ( #74523, #79472, #87094, #11544, #42402, #88588, #33325, #19647, #3445, #96661, #73338, #2445, #25742, #4417, #27231, #80978, #19150, #3923, #34324, #10036, #26725, #56622, #65708, #57609, #58115, #66225, #73827, #35312, #34806, #87605, #65221 ),
 .UNSPECIFIED., .F., .F.,
 ( 4, 3, 3, 3, 3, 3, 3, 3, 3, 3, 4 ),
 ( 0.000000000000000000, 0.1333490885032306283, 0.3007194338854234927, 0.4699862290244963270, 0.5844252810809187348, 0.6686540514502645749, 0.7354980260655307189, 0.8028463152565288308, 0.8633854507756889562, 0.9437142632666959408, 1.000000000000000000 ),
 .UNSPECIFIED. ) ;
#79191=CARTESIAN_POINT ( 'NONE',  ( 75.58055549604159751, 53.46810915028748212, -16.02836618447256001 ) ) ;
#79193=EDGE_CURVE ( 'NONE', #98946, #53182, #37464, .T. ) ;
#79196=CARTESIAN_POINT ( 'NONE',  ( 87.53662896702414287, 44.58992679936064008, 4.926115213305346074 ) ) ;
#79199=CARTESIAN_POINT ( 'NONE',  ( 11.78502771447809394, 29.73705186507753240, -3.090169943749475845 ) ) ;
#79202=CARTESIAN_POINT ( 'NONE',  ( 72.00170078070283353, 72.01756085178577393, 2.840212697767991568 ) ) ;
#79203=CARTESIAN_POINT ( 'NONE',  ( 84.06604358195920668, 51.46910565605918464, 14.65639964578790533 ) ) ;
#79209=ORIENTED_EDGE ( 'NONE', *, *, #66448, .F. ) ;
#79213=DIRECTION ( 'NONE',  ( 0.2503889871761765251, 0.9681453171404014180, 0.000000000000000000 ) ) ;
#79216=CARTESIAN_POINT ( 'NONE',  ( 39.01788588657935719, 31.03085787977765975, 9.188101187500006262 ) ) ;
#79220=CARTESIAN_POINT ( 'NONE',  ( 35.77386594998528579, 21.44966523072496756, -2.296566073217252530E-15 ) ) ;
#79227=PLANE ( 'NONE',  #69752 ) ;
#79229=CARTESIAN_POINT ( 'NONE',  ( 15.64721481668148328, 11.96004757982088940, -5.678558825948276656 ) ) ;
#79231=CARTESIAN_POINT ( 'NONE',  ( 21.16812676580726915, 15.14754757982089650, -5.678558825948275768 ) ) ;
#79238=CARTESIAN_POINT ( 'NONE',  ( 24.32480936679734640, 35.81751292744058190, -6.180339887498951690 ) ) ;
#79246=CARTESIAN_POINT ( 'NONE',  ( 86.05378759701316937, 47.66281079019294964, 10.87423542265411136 ) ) ;
#79248=CARTESIAN_POINT ( 'NONE',  ( 76.92291097195925431, 53.37782505870914918, 15.93814142932378353 ) ) ;
#79251=CARTESIAN_POINT ( 'NONE',  ( 34.95497629653712579, 28.38052372038643156, 10.00000000000000533 ) ) ;
#79253=CARTESIAN_POINT ( 'NONE',  ( 10.49025449741314375, 29.55466486950698624, -1.111400068045478839E-16 ) ) ;
#79256=CARTESIAN_POINT ( 'NONE',  ( 74.86688500840476479, 62.61836409510868151, -15.31937621055942067 ) ) ;
#79269=CARTESIAN_POINT ( 'NONE',  ( 83.37517334370022581, 49.65420094554470865, 13.45943336448511296 ) ) ;
#79272=CARTESIAN_POINT ( 'NONE',  ( 70.41189838529163580, 67.31627706263940070, 9.946319558533476268 ) ) ;
#79275=CARTESIAN_POINT ( 'NONE',  ( 82.35285118013293015, 53.50770157854819331, -15.77620284334259360 ) ) ;
#79278=DIRECTION ( 'NONE',  ( -0.2649596321165964552, 0.4589235447807054058, -0.8480480961564325071 ) ) ;
#79279=CARTESIAN_POINT ( 'NONE',  ( 24.83671989960918935, 22.84335787977763488, 9.188101187500006262 ) ) ;
#79281=VECTOR ( 'NONE', #54947, 1000.000000000000114 ) ;
#79289=EDGE_CURVE ( 'NONE', #58918, #90569, #75003, .T. ) ;
#79292=CARTESIAN_POINT ( 'NONE',  ( 71.55257436342132848, 59.07939963282102269, 15.82466129307116098 ) ) ;
#79296=CARTESIAN_POINT ( 'NONE',  ( 11.39908531360040911, 14.78052372038638573, -10.00000000000000355 ) ) ;
#79298=EDGE_CURVE ( 'NONE', #82006, #749, #33323, .T. ) ;
#79307=CARTESIAN_POINT ( 'NONE',  ( 74.15479259499207387, 55.62765001666249276, -16.59030973340311022 ) ) ;
#79311=ORIENTED_EDGE ( 'NONE', *, *, #7138, .T. ) ;
#79314=CARTESIAN_POINT ( 'NONE',  ( 81.06156068051836883, 46.84227557089664629, -12.44431404537389696 ) ) ;
#79318=CARTESIAN_POINT ( 'NONE',  ( 74.38843302549192060, 67.97504088991867377, -11.67932444824502802 ) ) ;
#79321=ORIENTED_EDGE ( 'NONE', *, *, #8925, .T. ) ;
#79322=CARTESIAN_POINT ( 'NONE',  ( 84.73412771832131796, 49.86158731552951195, 13.15459715302734978 ) ) ;
#79324=CARTESIAN_POINT ( 'NONE',  ( 36.87552185948406702, 26.45404122711136097, -8.090169943749478065 ) ) ;
#79329=CARTESIAN_POINT ( 'NONE',  ( 71.21424051265081800, 68.22285992147928368, -10.17931454856913120 ) ) ;
#79335=CARTESIAN_POINT ( 'NONE',  ( 22.99159801516092472, 18.98920272979926693, 7.433330006724137462 ) ) ;
#79336=CARTESIAN_POINT ( 'NONE',  ( 74.68831750804957892, 67.03523027571368686, 12.97943796060243216 ) ) ;
#79338=CARTESIAN_POINT ( 'NONE',  ( 72.91440843804703320, 59.27959524831282323, -15.98284220614978501 ) ) ;
#79347=CARTESIAN_POINT ( 'NONE',  ( 46.16617079539854274, 27.44966523072498177, -2.296566073217252530E-15 ) ) ;
#79349=FACE_OUTER_BOUND ( 'NONE', #66576, .T. ) ;
#79351=CARTESIAN_POINT ( 'NONE',  ( 69.57147599204645871, 65.95357847136563123, -11.50044640693676001 ) ) ;
#79356=CARTESIAN_POINT ( 'NONE',  ( 85.69613440654960357, 45.85434288225457777, 9.691492161565614438 ) ) ;
#79357=CARTESIAN_POINT ( 'NONE',  ( 83.90135245898494532, 51.67424826075555444, -14.40821023666590150 ) ) ;
#79364=CARTESIAN_POINT ( 'NONE',  ( 35.53452623260358223, 35.91421378149921395, 9.188101187500008038 ) ) ;
#79367=CARTESIAN_POINT ( 'NONE',  ( 77.87494449001893315, 61.77424058857110367, 16.06449337301375735 ) ) ;
#79372=CARTESIAN_POINT ( 'NONE',  ( 86.19539083654223077, 46.94244887560866886, -10.58787169974292297 ) ) ;
#79374=CARTESIAN_POINT ( 'NONE',  ( 27.36453209247643770, 17.92755873383626408, 6.180339887498953466 ) ) ;
#79375=CARTESIAN_POINT ( 'NONE',  ( 83.64242591893872714, 50.13093507612888544, -13.68615876095049266 ) ) ;
#79376=CARTESIAN_POINT ( 'NONE',  ( 84.81815374307583966, 49.91023469830950177, -13.17998982162479571 ) ) ;
#79382=CARTESIAN_POINT ( 'NONE',  ( 77.15327844083580544, 49.48234140023242134, -15.45668963368342119 ) ) ;
#79384=CARTESIAN_POINT ( 'NONE',  ( 88.37114838251338256, 44.19826770168089780, 0.1617965445409229042 ) ) ;
#79385=CARTESIAN_POINT ( 'NONE',  ( 79.42409360036769783, 54.45300451108273876, 15.94632819799358892 ) ) ;
#79392=CARTESIAN_POINT ( 'NONE',  ( 23.08833070876649529, 13.73415679381821874, 1.333680081654574804E-15 ) ) ;
#79395=CARTESIAN_POINT ( 'NONE',  ( 70.59038599826907046, 60.90612631591859127, -14.48346838026379579 ) ) ;
#79396=CARTESIAN_POINT ( 'NONE',  ( 45.61829935282815995, 28.19860640527296525, 2.839279412974134775 ) ) ;
#79397=ORIENTED_EDGE ( 'NONE', *, *, #74862, .F. ) ;
#79398=CARTESIAN_POINT ( 'NONE',  ( 85.49318370521093868, 48.99722645306706426, -12.73116331006621316 ) ) ;
#79404=CARTESIAN_POINT ( 'NONE',  ( 73.40795240808809297, 67.02439710917190041, 11.95168579066343995 ) ) ;
#79405=CARTESIAN_POINT ( 'NONE',  ( 76.45572749640669485, 51.64231386250387601, -16.15369532800221108 ) ) ;
#79415=EDGE_CURVE ( 'NONE', #79774, #91452, #5510, .T. ) ;
#79430=CARTESIAN_POINT ( 'NONE',  ( 73.91288345017510153, 68.57868192222672121, 11.39134523673511623 ) ) ;
#79437=CARTESIAN_POINT ( 'NONE',  ( 87.89455619572203204, 44.47450605225177611, -3.950270982313550672 ) ) ;
#79440=CARTESIAN_POINT ( 'NONE',  ( 78.28440716897011953, 56.29478510322071827, 16.19025749928794156 ) ) ;
#79441=DIRECTION ( 'NONE',  ( -0.5000000000000014433, 0.8660254037844378194, 0.000000000000000000 ) ) ;
#79442=CARTESIAN_POINT ( 'NONE',  ( 77.95436975687957215, 48.11784896437987413, 14.20357318872345331 ) ) ;
#79449=CARTESIAN_POINT ( 'NONE',  ( 72.80224333330460240, 56.85357120363885031, -15.94159948215087219 ) ) ;
#79452=CARTESIAN_POINT ( 'NONE',  ( 76.82578666445662918, 64.07401149769333415, -15.18382690731647600 ) ) ;
#79455=CARTESIAN_POINT ( 'NONE',  ( 88.15693819664804209, 44.07453305466302140, 0.5464416844217639957 ) ) ;
#79456=CARTESIAN_POINT ( 'NONE',  ( 13.67456932412660997, 8.864269794150878568, -3.090169943749474069 ) ) ;
#79461=CARTESIAN_POINT ( 'NONE',  ( 27.63686232447692603, 34.14336893147756768, 7.433330006724141015 ) ) ;
#79465=CARTESIAN_POINT ( 'NONE',  ( 13.87187630571069263, 28.98502408145591502, -5.678558825948271327 ) ) ;
#79471=EDGE_CURVE ( 'NONE', #32340, #18263, #64037, .T. ) ;
#79472=CARTESIAN_POINT ( 'NONE',  ( 86.72314128514305764, 46.93129043413777168, 10.24845158530357558 ) ) ;
#79476=CARTESIAN_POINT ( 'NONE',  ( 75.14123710989004223, 53.08787395263782827, 16.49283882849012173 ) ) ;
#79478=CARTESIAN_POINT ( 'NONE',  ( 82.33309958831539177, 53.73407448881686577, 15.84243556053685786 ) ) ;
#79483=CARTESIAN_POINT ( 'NONE',  ( 68.35293204362942276, 68.73096724137640479, -5.990830183022922029 ) ) ;
#79486=ORIENTED_EDGE ( 'NONE', *, *, #48612, .T. ) ;
#79487=CARTESIAN_POINT ( 'NONE',  ( 72.29720748969889144, 71.75793896413090067, 5.568862843245712568 ) ) ;
#79491=B_SPLINE_CURVE_WITH_KNOTS ( 'NONE', 3,
 ( #30960, #37552, #52268, #30465, #22862, #77059, #7667, #92797, #38553, #69463 ),
 .UNSPECIFIED., .F., .F.,
 ( 4, 2, 2, 2, 4 ),
 ( 0.000000000000000000, 0.0002622400424273620893, 0.0005244800848547241786, 0.0007867201272820862137, 0.001048960169709448357 ),
 .UNSPECIFIED. ) ;
#79492=CARTESIAN_POINT ( 'NONE',  ( 31.43713336585798146, 20.01110640527293683, 2.839279412974134775 ) ) ;
#79493=CARTESIAN_POINT ( 'NONE',  ( 75.30311887994048448, 66.55154771318241558, -13.10674181759690704 ) ) ;
#79494=CARTESIAN_POINT ( 'NONE',  ( 82.15597685699214026, 48.58689493459846176, -13.20209974158375488 ) ) ;
#79495=DIRECTION ( 'NONE',  ( 0.5000000000000014433, -0.8660254037844378194, 0.000000000000000000 ) ) ;
#79506=CARTESIAN_POINT ( 'NONE',  ( 32.36713501728652176, 42.18528772668521043, -1.583844403245329602 ) ) ;
#79509=CARTESIAN_POINT ( 'NONE',  ( 71.38852909611460973, 62.80635017521332486, -14.35756287307077805 ) ) ;
#79512=ORIENTED_EDGE ( 'NONE', *, *, #67003, .T. ) ;
#79516=ORIENTED_EDGE ( 'NONE', *, *, #97429, .T. ) ;
#79519=EDGE_CURVE ( 'NONE', #41986, #39534, #22928, .T. ) ;
#79521=CARTESIAN_POINT ( 'NONE',  ( 66.64560853618554859, 67.51366659840367390, 6.429781813620476072 ) ) ;
#79525=CARTESIAN_POINT ( 'NONE',  ( 82.18974175748606115, 47.92037233983167965, -12.77561182005171858 ) ) ;
#79539=CARTESIAN_POINT ( 'NONE',  ( 87.71763047028392180, 44.72620838780621000, 5.018703809423653794 ) ) ;
#79547=CARTESIAN_POINT ( 'NONE',  ( 71.55773796007210308, 59.00899692431989507, -15.84486509706986190 ) ) ;
#79555=CARTESIAN_POINT ( 'NONE',  ( 78.25353035412973668, 61.73196396808427266, 15.76132319596081111 ) ) ;
#79559=CARTESIAN_POINT ( 'NONE',  ( 75.68675361614918984, 63.43720209078236394, -14.77468968376273395 ) ) ;
#79561=CARTESIAN_POINT ( 'NONE',  ( 79.78867003348828746, 55.35328538066816861, 16.44695013865527855 ) ) ;
#79562=CARTESIAN_POINT ( 'NONE',  ( 36.61341721041482344, 22.10801979619931501, 3.090169943749476733 ) ) ;
#79565=CARTESIAN_POINT ( 'NONE',  ( 86.96434452339640586, 43.30424524822677768, 3.123802667395221722 ) ) ;
#79570=CARTESIAN_POINT ( 'NONE',  ( 82.37317549191088517, 48.42277367534339305, 13.04792507358340359 ) ) ;
#79575=CARTESIAN_POINT ( 'NONE',  ( 42.17466224797323804, 36.30066082961425877, -10.00000000000000533 ) ) ;
#79579=CARTESIAN_POINT ( 'NONE',  ( 31.59942275858663407, 40.01751292744058475, 6.180339887498949913 ) ) ;
#79583=CARTESIAN_POINT ( 'NONE',  ( 81.40062866174868361, 56.12702037940537991, 16.07990521299680609 ) ) ;
#79584=CARTESIAN_POINT ( 'NONE',  ( 13.24385365016830107, 12.81029122506292772, 8.090169943749479842 ) ) ;
#79586=CARTESIAN_POINT ( 'NONE',  ( 66.47763888060634940, 67.99612994687967671, 6.463816603905435443 ) ) ;
#79588=CARTESIAN_POINT ( 'NONE',  ( 69.74736874176301171, 66.77905827124916982, -10.09415051326821811 ) ) ;
#79592=VERTEX_POINT ( 'NONE', #58844 ) ;
#79598=CARTESIAN_POINT ( 'NONE',  ( 72.97386446981147401, 70.68132344495336383, 8.316175787459508584 ) ) ;
#79602=CARTESIAN_POINT ( 'NONE',  ( 25.06043674821822265, 32.65586893147757053, -7.433330006724137462 ) ) ;
#79606=EDGE_LOOP ( 'NONE', ( #67979, #96978, #60612, #36726 ) ) ;
#79607=CARTESIAN_POINT ( 'NONE',  ( 6.417452267959404821, 25.74646525600388003, 2.839279412974139660 ) ) ;
#79609=CARTESIAN_POINT ( 'NONE',  ( 71.95078207959971905, 72.63412948483367870, -0.9918729297793668076 ) ) ;
#79612=CARTESIAN_POINT ( 'NONE',  ( 72.26425284656475867, 71.11905259567225812, -6.027786176564315035 ) ) ;
#79614=EDGE_CURVE ( 'NONE', #56696, #66291, #73588, .T. ) ;
#79625=CARTESIAN_POINT ( 'NONE',  ( 73.10654890674743456, 57.42163371433187535, -15.88130622537231673 ) ) ;
#79626=CARTESIAN_POINT ( 'NONE',  ( 76.98684284838461167, 63.68060895951392553, 15.36346902396294745 ) ) ;
#79633=CARTESIAN_POINT ( 'NONE',  ( 34.35336353842534152, 22.76004757982091320, 5.678558825948272215 ) ) ;
#79635=CARTESIAN_POINT ( 'NONE',  ( 78.24597377814070853, 47.77139718876669860, -14.49689961856089759 ) ) ;
#79637=CARTESIAN_POINT ( 'NONE',  ( 73.86986929274216607, 68.54753403896816621, 11.39714278534123437 ) ) ;
#79643=CARTESIAN_POINT ( 'NONE',  ( 81.45669997382150029, 55.98862135975878118, -16.04303691645969820 ) ) ;
#79645=CARTESIAN_POINT ( 'NONE',  ( 78.49844431995686023, 56.32831885670888994, 16.60005998789102577 ) ) ;
#79648=CARTESIAN_POINT ( 'NONE',  ( 67.75753012590708124, 69.25273034730335553, -3.573886548774661165 ) ) ;
#79652=ADVANCED_FACE ( 'NONE', ( #64988 ), #11311, .T. ) ;
#79663=FACE_OUTER_BOUND ( 'NONE', #4180, .T. ) ;
#79667=CARTESIAN_POINT ( 'NONE',  ( 83.91646131505093820, 51.73966832772509861, -14.43249324666324895 ) ) ;
#79670=CARTESIAN_POINT ( 'NONE',  ( 80.61962873213096259, 57.61924663962614090, -16.24249425847791173 ) ) ;
#79672=CARTESIAN_POINT ( 'NONE',  ( 72.44020731426283533, 70.76712560363094440, 7.696415609646552802 ) ) ;
#79673=CARTESIAN_POINT ( 'NONE',  ( 71.96464922262767061, 71.55750601381073750, 5.589292941210060484 ) ) ;
#79684=CARTESIAN_POINT ( 'NONE',  ( 80.01034338638787347, 44.43011396636085664, -11.60714397506079720 ) ) ;
#79691=CARTESIAN_POINT ( 'NONE',  ( 81.21734643817387678, 51.70401989366683893, -14.96604167157805598 ) ) ;
#79697=CARTESIAN_POINT ( 'NONE',  ( 15.66455532895297331, 30.81751292744056059, -6.180339887498951690 ) ) ;
#79699=CARTESIAN_POINT ( 'NONE',  ( 85.33699565288863198, 48.33901173460944278, -12.30238903177781395 ) ) ;
#79701=CARTESIAN_POINT ( 'NONE',  ( 45.60499120716188060, 26.73415679381826138, -6.890680421881970419E-14 ) ) ;
#79704=CARTESIAN_POINT ( 'NONE',  ( 9.667034506031535912, 13.78052372038638396, -10.00000000000000355 ) ) ;
#79713=CARTESIAN_POINT ( 'NONE',  ( 36.84800447571193160, 26.98920272979929180, 7.433330006724137462 ) ) ;
#79717=CARTESIAN_POINT ( 'NONE',  ( 27.04628097738780212, 27.56628583063842086, 9.188101187500006262 ) ) ;
#79722=CARTESIAN_POINT ( 'NONE',  ( 43.27754793094329244, 25.39040679176986970, -6.890680421881970419E-14 ) ) ;
#79724=CARTESIAN_POINT ( 'NONE',  ( 12.38457448260035143, 9.011106405272903075, 2.839279412974134775 ) ) ;
#79726=CARTESIAN_POINT ( 'NONE',  ( 18.23327619575285041, 19.03085787977761711, 9.188101187500006262 ) ) ;
#79729=CARTESIAN_POINT ( 'NONE',  ( 87.86832398745416128, 44.01541417138756884, -1.805110452858952552 ) ) ;
#79737=CARTESIAN_POINT ( 'NONE',  ( 87.39182636385071135, 45.50004596871073659, 7.088608641304300129 ) ) ;
#79742=CARTESIAN_POINT ( 'NONE',  ( 86.37991722458738764, 47.25272401055813276, 10.79753792097408116 ) ) ;
#79744=CARTESIAN_POINT ( 'NONE',  ( 76.48640248419295062, 51.58918322513654431, 15.64831315713033355 ) ) ;
#79747=CARTESIAN_POINT ( 'NONE',  ( 78.39991307920188035, 61.32441222751918986, -15.87033061864282324 ) ) ;
#79748=CARTESIAN_POINT ( 'NONE',  ( 79.26974131400611157, 59.52036692680491115, -16.53359576550787224 ) ) ;
#79749=CARTESIAN_POINT ( 'NONE',  ( 12.79584618246493477, 29.16126292948894516, -6.180339887498951690 ) ) ;
#79755=CARTESIAN_POINT ( 'NONE',  ( 29.87413333957346140, 40.18080186712595747, 3.090169943749475401 ) ) ;
#79758=CARTESIAN_POINT ( 'NONE',  ( 32.96252748593624915, 42.52903772873360566, -1.583844403245329602 ) ) ;
#79762=LINE ( 'NONE', #10327, #72541 ) ;
#79764=DIRECTION ( 'NONE',  ( -0.3978777116982094575, -0.7304723483372487225, 0.5550706935593536784 ) ) ;
#79770=CARTESIAN_POINT ( 'NONE',  ( 69.20971128213882650, 64.50273501078117988, 11.88834065357228731 ) ) ;
#79773=CARTESIAN_POINT ( 'NONE',  ( 79.14312167556931854, 57.64441083166269664, 0.000000000000000000 ) ) ;
#79774=VERTEX_POINT ( 'NONE', #66351 ) ;
#79776=CARTESIAN_POINT ( 'NONE',  ( 17.01121839442928163, 30.79752408145592568, -5.678558825948271327 ) ) ;
#79783=CARTESIAN_POINT ( 'NONE',  ( 81.19243458941035385, 52.42165318742301139, -15.24367534770689225 ) ) ;
#79785=CARTESIAN_POINT ( 'NONE',  ( 36.44916501977947831, 42.81751292744058901, -6.180339887498951690 ) ) ;
#79789=ORIENTED_EDGE ( 'NONE', *, *, #44241, .T. ) ;
#79791=FACE_OUTER_BOUND ( 'NONE', #83574, .T. ) ;
#79792=DIRECTION ( 'NONE',  ( -0.8660254037844378194, -0.5000000000000013323, -0.000000000000000000 ) ) ;
#79803=UNCERTAINTY_MEASURE_WITH_UNIT (LENGTH_MEASURE( 1.000000000000000082E-05 ), #80219, 'distance_accuracy_value', 'NONE');
#79806=CARTESIAN_POINT ( 'NONE',  ( 68.57836289805518959, 70.07438557745322782, 1.916984831344509699 ) ) ;
#79807=CARTESIAN_POINT ( 'NONE',  ( 81.96547941067910870, 41.17040324926905015, 3.814626384468428721 ) ) ;
#79812=CARTESIAN_POINT ( 'NONE',  ( 74.31626339567910122, 68.46754964620755857, -11.19101123510062301 ) ) ;
#79815=CARTESIAN_POINT ( 'NONE',  ( 79.18418104304701899, 60.10533407485776536, -16.47260471942688653 ) ) ;
#79818=CARTESIAN_POINT ( 'NONE',  ( 68.49197605392033950, 64.33996568623787482, -12.33092966291259174 ) ) ;
#79822=CARTESIAN_POINT ( 'NONE',  ( 66.90909321525144549, 68.17756947874360662, -6.600776075497404527 ) ) ;
#79830=CARTESIAN_POINT ( 'NONE',  ( 13.87187630571069263, 28.98502408145591502, -5.678558825948271327 ) ) ;
#79831=B_SPLINE_CURVE_WITH_KNOTS ( 'NONE', 3,
 ( #76780, #4510, #51614, #35905, #92036, #59180, #97733, #20728, #58692, #82065, #81072, #12124, #5024, #66805, #50603, #6879 ),
 .UNSPECIFIED., .F., .F.,
 ( 4, 1, 2, 2, 2, 1, 2, 2, 4 ),
 ( 0.000000000000000000, 0.1250000000000001388, 0.1875000000000002220, 0.2500000000000002776, 0.5000000000000001110, 0.6249999999999991118, 0.6874999999999985567, 0.7499999999999978906, 1.000000000000000000 ),
 .UNSPECIFIED. ) ;
#79832=CARTESIAN_POINT ( 'NONE',  ( 75.22447641198338886, 66.97122069168695191, 13.23119059164782030 ) ) ;
#79834=VECTOR ( 'NONE', #84093, 1000.000000000000227 ) ;
#79843=CARTESIAN_POINT ( 'NONE',  ( 81.57862098688173091, 55.52127002482139062, -16.32346926850663493 ) ) ;
#79845=CARTESIAN_POINT ( 'NONE',  ( 71.77426126090318803, 65.60551381397631587, -12.81782449613754515 ) ) ;
#79848=CARTESIAN_POINT ( 'NONE',  ( 71.96242732416023102, 72.61395932958829746, 1.324942441655030834 ) ) ;
#79850=CARTESIAN_POINT ( 'NONE',  ( 80.23209172613701412, 54.97481774069060378, 15.95603643075370748 ) ) ;
#79851=CARTESIAN_POINT ( 'NONE',  ( 83.55710330194072810, 51.48266744151908370, -14.41134322998550310 ) ) ;
#79852=EDGE_CURVE ( 'NONE', #67548, #44339, #24203, .T. ) ;
#79853=CARTESIAN_POINT ( 'NONE',  ( 71.96639307748559133, 71.49757472301890004, -5.734781593071435424 ) ) ;
#79856=CARTESIAN_POINT ( 'NONE',  ( 86.46048006423905008, 47.32182001325401188, 10.26516935212321968 ) ) ;
#79858=CARTESIAN_POINT ( 'NONE',  ( 40.57792791151964451, 35.37878583063844218, 9.188101187500006262 ) ) ;
#79861=CARTESIAN_POINT ( 'NONE',  ( 77.74340892523753155, 61.62887588481113710, 16.08014808546132102 ) ) ;
#79866=CARTESIAN_POINT ( 'NONE',  ( 78.90607854399013377, 60.09749198675558546, 16.11258120454802523 ) ) ;
#79869=DIRECTION ( 'NONE',  ( 0.5000000000000014433, -0.8660254037844378194, 0.000000000000000000 ) ) ;
#79870=B_SPLINE_CURVE_WITH_KNOTS ( 'NONE', 3,
 ( #33349, #19670, #41435, #72376 ),
 .UNSPECIFIED., .F., .F.,
 ( 4, 4 ),
 ( 0.8924449491999673079, 1.000000000000000000 ),
 .UNSPECIFIED. ) ;
#79871=CARTESIAN_POINT ( 'NONE',  ( 80.53677833458100110, 44.48879437267268599, 11.38558430043868697 ) ) ;
#79872=CARTESIAN_POINT ( 'NONE',  ( 84.79995857201339504, 49.88899232450376786, -13.17356253177934455 ) ) ;
#79874=VERTEX_POINT ( 'NONE', #80362 ) ;
#79878=DIRECTION ( 'NONE',  ( 0.000000000000000000, -0.6050222638427448230, 0.7962085532412974676 ) ) ;
#79881=CARTESIAN_POINT ( 'NONE',  ( 79.58877750526134776, 55.57171882432602672, 16.09998944077883110 ) ) ;
#79903=CARTESIAN_POINT ( 'NONE',  ( 82.28003896795380001, 40.62557011406286733, -3.142018250819525793 ) ) ;
#79923=CARTESIAN_POINT ( 'NONE',  ( 71.14215440105562038, 62.56599120317326879, -13.86464812710125294 ) ) ;
#79925=CARTESIAN_POINT ( 'NONE',  ( 78.41477381122238910, 47.32040575024741713, -14.22103711499937262 ) ) ;
#79927=CARTESIAN_POINT ( 'NONE',  ( 80.66106005736661189, 43.24916060877089308, -9.240259099883365579 ) ) ;
#79928=CARTESIAN_POINT ( 'NONE',  ( 70.58472459542726085, 71.29540112946914121, -2.020767390530186614 ) ) ;
#79932=CARTESIAN_POINT ( 'NONE',  ( 88.05369993652286098, 44.62252207614050548, -4.124069452546489600 ) ) ;
#79942=CARTESIAN_POINT ( 'NONE',  ( 77.44921057498504524, 55.30942947506500218, -16.14045094355945054 ) ) ;
#79943=CARTESIAN_POINT ( 'NONE',  ( 79.15179632339811633, 45.85242797515901714, -13.09306047831970510 ) ) ;
#79945=CARTESIAN_POINT ( 'NONE',  ( 73.61926920126447271, 69.75873974038962899, 10.00767910897496193 ) ) ;
#79947=CARTESIAN_POINT ( 'NONE',  ( 76.86986466358051473, 64.04458250793000218, -15.20481942635857742 ) ) ;
#79950=CARTESIAN_POINT ( 'NONE',  ( 87.90060490056963260, 43.92552512120865771, 0.4375478113261034308 ) ) ;
#79952=CARTESIAN_POINT ( 'NONE',  ( 84.14312167556933275, 48.98415679381830756, 0.000000000000000000 ) ) ;
#79955=CARTESIAN_POINT ( 'NONE',  ( 31.53879454291322304, 39.18502408145594273, 5.678558825948276656 ) ) ;
#79956=CARTESIAN_POINT ( 'NONE',  ( 82.47767859619965236, 50.30750760982864733, 14.54247616347400296 ) ) ;
#79959=CARTESIAN_POINT ( 'NONE',  ( 19.43607595823839418, 14.14754757982089473, -5.678558825948276656 ) ) ;
#79961=CARTESIAN_POINT ( 'NONE',  ( 74.23555041547365363, 68.49601928387087924, -11.11897725275786719 ) ) ;
#79971=CARTESIAN_POINT ( 'NONE',  ( 74.73487060833782891, 53.69418506457893159, 16.08953207461605217 ) ) ;
#79987=CARTESIAN_POINT ( 'NONE',  ( 30.49295849316677831, 39.64646525600392835, -2.839279412974133887 ) ) ;
#79988=CARTESIAN_POINT ( 'NONE',  ( 79.91974514325150381, 44.69068051420087073, 11.20237123581853744 ) ) ;
#79989=CARTESIAN_POINT ( 'NONE',  ( 84.83352707183692587, 50.23671165375215253, -13.78554283518410095 ) ) ;
#79990=CARTESIAN_POINT ( 'NONE',  ( 78.73344330045726736, 49.45143681483339293, -14.59549011545008490 ) ) ;
#79998=CARTESIAN_POINT ( 'NONE',  ( 81.71134522782797660, 55.74075304576283685, -15.99172648312053369 ) ) ;
#80013=CARTESIAN_POINT ( 'NONE',  ( 79.96962623824013860, 44.78594355328343823, -11.26070751024680661 ) ) ;
#80014=CARTESIAN_POINT ( 'NONE',  ( 66.66342508697567837, 67.67433879810248243, 6.129251300726011209 ) ) ;
#80016=CARTESIAN_POINT ( 'NONE',  ( 85.47913374364790684, 42.62622548008751266, 0.2499991700750583967 ) ) ;
#80020=EDGE_LOOP ( 'NONE', ( #80754, #62483, #46915, #7794 ) ) ;
#80025=CARTESIAN_POINT ( 'NONE',  ( 75.91502559367474134, 65.16891969575354437, -14.48077610374784996 ) ) ;
#80028=CARTESIAN_POINT ( 'NONE',  ( 87.68902078672120126, 44.98529012857299136, -6.607530655827392074 ) ) ;
#80030=CARTESIAN_POINT ( 'NONE',  ( 87.62752662085767952, 44.66923158952226203, 5.004374079557546651 ) ) ;
#80034=CARTESIAN_POINT ( 'NONE',  ( 67.44257088943838596, 67.25355904234817217, -8.657396272410824878 ) ) ;
#80037=CARTESIAN_POINT ( 'NONE',  ( 76.20493386330700503, 51.02659346225095049, -16.05104161519640371 ) ) ;
#80044=CARTESIAN_POINT ( 'NONE',  ( 84.09950503289748269, 42.51577704912055111, 4.332266723902765904 ) ) ;
#80046=CARTESIAN_POINT ( 'NONE',  ( 77.90166149968712261, 61.78270738046986565, 16.06607043079731767 ) ) ;
#80050=VERTEX_POINT ( 'NONE', #11446 ) ;
#80051=AXIS2_PLACEMENT_3D ( 'NONE', #17412, #79764, #24510 ) ;
#80052=CARTESIAN_POINT ( 'NONE',  ( 74.61052374806135390, 63.82185717549396031, -14.32275223664241715 ) ) ;
#80056=CARTESIAN_POINT ( 'NONE',  ( 40.25072390630947439, 24.20801979619931998, -3.090169943749474069 ) ) ;
#80057=CARTESIAN_POINT ( 'NONE',  ( 78.56719005003022005, 47.98515344134877836, 13.96283253221395704 ) ) ;
#80058=CARTESIAN_POINT ( 'NONE',  ( 81.19656099875513178, 43.43094936621162105, -9.896970666190503252 ) ) ;
#80061=CARTESIAN_POINT ( 'NONE',  ( 83.14648767797254436, 43.23107607431138177, -7.173306651377752807 ) ) ;
#80066=CARTESIAN_POINT ( 'NONE',  ( 86.79190430688251467, 45.84585087985657736, 8.866399834819148396 ) ) ;
#80067=CARTESIAN_POINT ( 'NONE',  ( 29.10770312285472983, 32.50829794293882458, -10.00000000000000355 ) ) ;
#80068=CARTESIAN_POINT ( 'NONE',  ( 81.67161923058380069, 41.61203830614370247, 5.543601729363009767 ) ) ;
#80072=CARTESIAN_POINT ( 'NONE',  ( 33.70846307691164156, 35.16454794089043645, -10.00000000000000355 ) ) ;
#80080=CARTESIAN_POINT ( 'NONE',  ( 87.18760076931933156, 46.20468558230229661, -8.391508599297639037 ) ) ;
#80081=CARTESIAN_POINT ( 'NONE',  ( 83.50487366122874278, 51.96486753097845224, 15.01313857892666626 ) ) ;
#80086=CARTESIAN_POINT ( 'NONE',  ( 29.27874087092374111, 39.83705186507756224, 3.090169943749475401 ) ) ;
#80092=CARTESIAN_POINT ( 'NONE',  ( 67.51094951715245429, 66.79118171239792900, -8.453174244170460483 ) ) ;
#80098=CARTESIAN_POINT ( 'NONE',  ( 72.19011348444853127, 68.90289858658827882, 10.04383758347407074 ) ) ;
#80099=CARTESIAN_POINT ( 'NONE',  ( 22.55378097864968012, 33.99752408145592852, 5.678558825948277544 ) ) ;
#80104=CARTESIAN_POINT ( 'NONE',  ( 21.21803360120161486, 14.11110640527291871, -2.839279412974138328 ) ) ;
#80105=EDGE_CURVE ( 'NONE', #75846, #19430, #65104, .T. ) ;
#80107=CARTESIAN_POINT ( 'NONE',  ( 71.89122079532039322, 72.62093029633255981, -0.6100853850958146696 ) ) ;
#80118=CARTESIAN_POINT ( 'NONE',  ( 88.67874521539408761, 45.12822637883663646, 1.911324073694122932E-15 ) ) ;
#80119=CARTESIAN_POINT ( 'NONE',  ( 9.964077338596862177, 24.49103043416547365, -8.090169943749479842 ) ) ;
#80122=CARTESIAN_POINT ( 'NONE',  ( 72.07791713363762653, 72.33007614824393272, -3.421992246486540434 ) ) ;
#80123=CARTESIAN_POINT ( 'NONE',  ( 72.83035752141398689, 57.36277735378698850, -15.86473357501050074 ) ) ;
#80124=CARTESIAN_POINT ( 'NONE',  ( 78.11917150362724271, 61.95746172053952705, -16.05486485196055568 ) ) ;
#80133=CARTESIAN_POINT ( 'NONE',  ( 28.76090768559789979, 38.64646525600391413, -2.839279412974133887 ) ) ;
#80135=CARTESIAN_POINT ( 'NONE',  ( 78.21114047790953805, 47.70659236517302304, -14.47520218207839982 ) ) ;
#80137=CARTESIAN_POINT ( 'NONE',  ( 74.24116255903008721, 68.58322516222325760, 11.55893809163645614 ) ) ;
#80139=CARTESIAN_POINT ( 'NONE',  ( 73.04277380876573034, 70.56196896876862468, 7.835544939490341143 ) ) ;
#80142=CARTESIAN_POINT ( 'NONE',  ( 75.91858796819732902, 58.13906729783923311, -16.03854386934378695 ) ) ;
#80147=CARTESIAN_POINT ( 'NONE',  ( 69.06272728912895786, 69.58621347229239973, -4.965237653724661193 ) ) ;
#80153=CARTESIAN_POINT ( 'NONE',  ( 87.00029699285249762, 43.25090828054809577, -2.658650631722468294 ) ) ;
#80159=CARTESIAN_POINT ( 'NONE',  ( 84.83104025798097325, 44.16562702927063100, -7.189586749132937271 ) ) ;
#80160=DIRECTION ( 'NONE',  ( -0.8660254037844379305, -0.5000000000000014433, -0.000000000000000000 ) ) ;
#80163=CARTESIAN_POINT ( 'NONE',  ( 79.47299837911636189, 59.61027691956581975, -16.18668525952085346 ) ) ;
#80164=CARTESIAN_POINT ( 'NONE',  ( 75.26800218211973004, 63.80269639718548547, 14.51819789563784546 ) ) ;
#80167=CARTESIAN_POINT ( 'NONE',  ( 80.38474943732042277, 57.10871594127473116, -16.23110256588661571 ) ) ;
#80172=EDGE_CURVE ( 'NONE', #70878, #7719, #50027, .T. ) ;
#80175=CARTESIAN_POINT ( 'NONE',  ( 68.93992071117129683, 69.86581718082992154, 3.903901410921837289 ) ) ;
#80187=CARTESIAN_POINT ( 'NONE',  ( 81.72375876848666110, 59.17461627083314113, 0.4987820251299118213 ) ) ;
#80193=CARTESIAN_POINT ( 'NONE',  ( 21.57298720112009249, 14.58380873178786885, 6.180339887498953466 ) ) ;
#80194=CARTESIAN_POINT ( 'NONE',  ( 85.69214519656509310, 48.79468762505698720, 12.02259801017994789 ) ) ;
#80195=CARTESIAN_POINT ( 'NONE',  ( 66.18996477082612273, 69.34069001910528129, 0.2116841265692433471 ) ) ;
#80198=CARTESIAN_POINT ( 'NONE',  ( 73.87037352680503943, 54.99746270706273776, -16.12935872011092897 ) ) ;
#80202=CARTESIAN_POINT ( 'NONE',  ( 3.517663757265353741, 25.52903772873354171, -1.583844403245363575 ) ) ;
#80211=CARTESIAN_POINT ( 'NONE',  ( 32.31339950491288704, 36.84336893147758474, -7.433330006724137462 ) ) ;
#80214=CARTESIAN_POINT ( 'NONE',  ( 26.97895004263468266, 38.68290643055188127, 3.479690158560446702E-15 ) ) ;
#80216=EDGE_CURVE ( 'NONE', #68463, #41583, #25497, .T. ) ;
#80219=( LENGTH_UNIT ( ) NAMED_UNIT ( * ) SI_UNIT ( .MILLI., .METRE. ) );
#80220=CARTESIAN_POINT ( 'NONE',  ( 8.149503075528279794, 26.74646525600388358, 2.839279412974139660 ) ) ;
#80222=CARTESIAN_POINT ( 'NONE',  ( 13.26084062165525523, 25.84336893147755276, -7.433330006724137462 ) ) ;
#80227=CARTESIAN_POINT ( 'NONE',  ( 84.83229447964083647, 50.15339875539878989, -13.73726727158769023 ) ) ;
#80229=CARTESIAN_POINT ( 'NONE',  ( 88.16031874257379286, 44.17530435389893739, -1.747866100070386564 ) ) ;
#80234=CARTESIAN_POINT ( 'NONE',  ( 66.08842961843907915, 68.52315484731427375, 4.630389166009985402 ) ) ;
#80235=CARTESIAN_POINT ( 'NONE',  ( 87.36818918644996756, 45.49344374928407575, 7.101962019857444020 ) ) ;
#80237=ORIENTED_EDGE ( 'NONE', *, *, #13159, .F. ) ;
#80239=CARTESIAN_POINT ( 'NONE',  ( 86.72415995732357885, 47.00718562526229505, 10.33097223407348686 ) ) ;
#80241=CARTESIAN_POINT ( 'NONE',  ( 78.30955769916531040, 61.43963167811126169, 15.82323565659766373 ) ) ;
#80245=CARTESIAN_POINT ( 'NONE',  ( 79.11171798038402869, 59.41904482235665341, -16.53441574648433487 ) ) ;
#80246=CARTESIAN_POINT ( 'NONE',  ( 79.02426040586578893, 48.68606636885871808, -14.72935746379201838 ) ) ;
#80247=CARTESIAN_POINT ( 'NONE',  ( 15.25129666230372827, 24.50829794293881037, -10.00000000000000355 ) ) ;
#80252=CARTESIAN_POINT ( 'NONE',  ( 74.25791966876403194, 62.13065321042455480, 14.88776587584266942 ) ) ;
#80253=ORIENTED_EDGE ( 'NONE', *, *, #25109, .T. ) ;
#80259=B_SPLINE_CURVE_WITH_KNOTS ( 'NONE', 3,
 ( #72692, #3286, #18473, #63553, #80821, #33672, #26568, #34166, #32655, #55927, #65551, #88423 ),
 .UNSPECIFIED., .F., .F.,
 ( 4, 2, 2, 2, 2, 4 ),
 ( 0.4976197654691878469, 0.6232148241018862223, 0.6860123534182385185, 0.7488098827345908148, 0.8744049413672954074, 1.000000000000000000 ),
 .UNSPECIFIED. ) ;
#80262=CARTESIAN_POINT ( 'NONE',  ( 67.53009088161343243, 67.40294954277804607, 7.576186009010610789 ) ) ;
#80264=CARTESIAN_POINT ( 'NONE',  ( 83.06694468350191585, 50.40823306540413995, -14.42615828136741918 ) ) ;
#80267=CARTESIAN_POINT ( 'NONE',  ( 70.35913297700497537, 67.20083026265126591, 10.03723707890633321 ) ) ;
#80273=CARTESIAN_POINT ( 'NONE',  ( 19.64056747690256088, 19.84335787977763133, 9.188101187500006262 ) ) ;
#80275=CARTESIAN_POINT ( 'NONE',  ( 77.54361356138011274, 49.75803992512373952, -14.96129575302289716 ) ) ;
#80277=CARTESIAN_POINT ( 'NONE',  ( 84.74965453446901620, 41.75349613245864333, -1.218611519740888882 ) ) ;
#80283=CARTESIAN_POINT ( 'NONE',  ( 9.894862028763428796, 29.21091486745858745, -1.111400068045478839E-16 ) ) ;
#80300=CARTESIAN_POINT ( 'NONE',  ( 74.46167478334288603, 68.12047429673633303, -11.58806946105432978 ) ) ;
#80302=CARTESIAN_POINT ( 'NONE',  ( 80.77153619337677526, 46.90080847010725051, -12.59910185819319217 ) ) ;
#80305=CARTESIAN_POINT ( 'NONE',  ( 82.41840067511127188, 41.61564054470166241, 4.454349221539423809 ) ) ;
#80313=CARTESIAN_POINT ( 'NONE',  ( 83.86212765327434226, 46.92509768004335058, 11.25106203221198875 ) ) ;
#80316=CARTESIAN_POINT ( 'NONE',  ( 68.51532939750342166, 64.50022977702580818, -12.21507596867179046 ) ) ;
#80327=B_SPLINE_CURVE_WITH_KNOTS ( 'NONE', 3,
 ( #49064, #63255, #17150, #56651, #87636, #79998, #39928, #94691, #94196, #10567, #25252, #47547, #56135, #70865, #40440, #62740, #48048, #24750, #69847, #31350, #85613, #93696, #16156, #47054 ),
 .UNSPECIFIED., .F., .F.,
 ( 4, 2, 2, 2, 2, 2, 2, 2, 2, 2, 2, 4 ),
 ( 0.000000000000000000, 0.1249999999999813483, 0.2499999999999626965, 0.3749999999999440448, 0.4374999999999475975, 0.4999999999999511502, 0.5624999999999547029, 0.6249999999999582556, 0.6874999999999618083, 0.7499999999999653610, 0.8749999999999826805, 1.000000000000000000 ),
 .UNSPECIFIED. ) ;
#80332=CARTESIAN_POINT ( 'NONE',  ( 23.10163885443276754, 15.19860640527292261, 2.839279412974134775 ) ) ;
#80333=CARTESIAN_POINT ( 'NONE',  ( 75.10353227920388974, 67.08955699197328215, 13.10598502456514680 ) ) ;
#80345=CARTESIAN_POINT ( 'NONE',  ( 81.29586503113306151, 55.42867650357229081, -16.33480133305122450 ) ) ;
#80347=CARTESIAN_POINT ( 'NONE',  ( 68.11396990072299218, 66.09066184265174115, -10.54551009852403709 ) ) ;
#80352=CARTESIAN_POINT ( 'NONE',  ( 83.70511640034648337, 52.20013393807822411, -14.67019430348358888 ) ) ;
#80353=CARTESIAN_POINT ( 'NONE',  ( 72.13998692144450331, 71.54377819717346654, -5.860361805407116265 ) ) ;
#80357=CARTESIAN_POINT ( 'NONE',  ( 45.84141126897937824, 27.26216523072498887, -2.296566073217252530E-15 ) ) ;
#80360=CARTESIAN_POINT ( 'NONE',  ( 77.82724693974202523, 61.74329194277088106, 16.06526602017299510 ) ) ;
#80362=CARTESIAN_POINT ( 'NONE',  ( 76.62156306105930526, 63.43458379359962152, 15.37592086074861619 ) ) ;
#80364=CARTESIAN_POINT ( 'NONE',  ( 78.87398835131222086, 59.62348996268822532, 16.50394892759813814 ) ) ;
#80367=CARTESIAN_POINT ( 'NONE',  ( 84.37825102736907468, 49.99960613749293969, 13.80049582259582763 ) ) ;
#80369=CYLINDRICAL_SURFACE ( 'NONE', #38711, 16.60714546451156792 ) ;
#80371=CARTESIAN_POINT ( 'NONE',  ( 73.45606387015448036, 70.03420106287664737, -9.568701002945239509 ) ) ;
#80372=CARTESIAN_POINT ( 'NONE',  ( 84.58308955143566266, 49.89698236725671165, -13.67050406800346707 ) ) ;
#80374=ORIENTED_EDGE ( 'NONE', *, *, #67003, .F. ) ;
#80379=FACE_OUTER_BOUND ( 'NONE', #15375, .T. ) ;
#80386=CARTESIAN_POINT ( 'NONE',  ( 82.28206475745885484, 40.65554467922788007, 3.268909026120783157 ) ) ;
#80388=CARTESIAN_POINT ( 'NONE',  ( 6.396987757676594555, 15.64441083166260427, 0.000000000000000000 ) ) ;
#80392=CARTESIAN_POINT ( 'NONE',  ( 82.79552190425015112, 41.59957507336271476, -5.373932124834087887 ) ) ;
#80395=VERTEX_POINT ( 'NONE', #44170 ) ;
#80396=CARTESIAN_POINT ( 'NONE',  ( 70.60797872409460751, 60.93970780067326132, -14.47325389371336790 ) ) ;
#80397=CARTESIAN_POINT ( 'NONE',  ( 35.63920408047906818, 43.68290643055190969, 3.479690158560446702E-15 ) ) ;
#80399=CARTESIAN_POINT ( 'NONE',  ( 85.73351810911900373, 48.76173041439603395, -12.45270611261530469 ) ) ;
#80407=CARTESIAN_POINT ( 'NONE',  ( 87.38036106307322370, 44.18516793481750682, 5.218929132667811110 ) ) ;
#80410=CARTESIAN_POINT ( 'NONE',  ( 22.42372293028334340, 18.11029122506294442, -8.090169943749478065 ) ) ;
#80415=CARTESIAN_POINT ( 'NONE',  ( 65.81325020318384134, 69.12384646711140590, 0.1587991348731422614 ) ) ;
#80417=CARTESIAN_POINT ( 'NONE',  ( 13.95435611255089725, 31.55466486950698268, -1.111400068045478839E-16 ) ) ;
#80423=CARTESIAN_POINT ( 'NONE',  ( 87.99973427719299934, 43.78392399561505499, 2.406698522940694307 ) ) ;
#80429=DIRECTION ( 'NONE',  ( -0.9619696745371177915, 0.2731562652969021787, 0.000000000000000000 ) ) ;
#80431=EDGE_CURVE ( 'NONE', #65130, #93491, #42122, .T. ) ;
#80432=CARTESIAN_POINT ( 'NONE',  ( 80.98736875202749275, 43.37942139736701108, -9.977273511710089693 ) ) ;
#80442=CARTESIAN_POINT ( 'NONE',  ( 77.34348292206982478, 51.51894111865114212, 15.53773553076495162 ) ) ;
#80445=DIRECTION ( 'NONE',  ( -0.8660254037844379305, -0.5000000000000014433, -0.000000000000000000 ) ) ;
#80447=PLANE ( 'NONE',  #74131 ) ;
#80456=CARTESIAN_POINT ( 'NONE',  ( 81.72770187496514893, 51.60650539560465688, -15.27405233875389179 ) ) ;
#80458=CARTESIAN_POINT ( 'NONE',  ( 87.98594423550160570, 43.75089820288621212, -2.253463800273092676 ) ) ;
#80461=CARTESIAN_POINT ( 'NONE',  ( 29.97031301328857467, 32.70171378149920827, -9.188101187500004485 ) ) ;
#80462=CARTESIAN_POINT ( 'NONE',  ( 83.17871495584169850, 48.30807258732734510, -13.18720427395424011 ) ) ;
#80463=CARTESIAN_POINT ( 'NONE',  ( 86.98925081226386169, 46.40596221211884398, -8.809588356812493970 ) ) ;
#80464=VERTEX_POINT ( 'NONE', #36573 ) ;
#80465=CARTESIAN_POINT ( 'NONE',  ( 18.23327619575285041, 19.03085787977762067, 9.188101187500006262 ) ) ;
#80467=CARTESIAN_POINT ( 'NONE',  ( 76.52691452431521668, 63.65543071367928007, 14.90473833858518127 ) ) ;
#80472=CARTESIAN_POINT ( 'NONE',  ( 70.37934122712871954, 61.23818324669216651, 14.28954007458889031 ) ) ;
#80477=CARTESIAN_POINT ( 'NONE',  ( 27.71094225399020416, 18.12755873383627048, -6.180339887498949025 ) ) ;
#80479=CARTESIAN_POINT ( 'NONE',  ( 85.23727002651352791, 45.78824278971900696, 9.273454399903927836 ) ) ;
#80480=ORIENTED_EDGE ( 'NONE', *, *, #50873, .F. ) ;
#80494=CARTESIAN_POINT ( 'NONE',  ( 29.13557404741141355, 37.79752408145594700, -5.678558825948271327 ) ) ;
#80496=DIRECTION ( 'NONE',  ( 0.5000000000000013323, -0.8660254037844378194, 0.000000000000000000 ) ) ;
#80503=CARTESIAN_POINT ( 'NONE',  ( 85.59143893114691082, 48.93292747530462350, -12.17357014060645604 ) ) ;
#80516=CARTESIAN_POINT ( 'NONE',  ( 80.17579727260986999, 44.92489227719274680, -11.27803833280161072 ) ) ;
#80520=CARTESIAN_POINT ( 'NONE',  ( 12.45916558416763209, 19.14441083166259361, 10.00000000000000533 ) ) ;
#80521=CARTESIAN_POINT ( 'NONE',  ( 75.15191903148871688, 52.97183600646508239, -16.48001256418180915 ) ) ;
#80529=CARTESIAN_POINT ( 'NONE',  ( 31.59046986846508887, 19.20801979619930222, -3.090169943749474069 ) ) ;
#80531=CARTESIAN_POINT ( 'NONE',  ( 69.10341330002957250, 69.27088624711088016, -5.834800079929739702 ) ) ;
#80538=CARTESIAN_POINT ( 'NONE',  ( 87.05064968419601712, 44.04826721231160747, -3.969180055969657950 ) ) ;
#80540=CARTESIAN_POINT ( 'NONE',  ( 82.25407785542023476, 40.61683643427734580, -3.170132542450867508 ) ) ;
#80545=CARTESIAN_POINT ( 'NONE',  ( 82.18398586331583999, 40.60379566207949154, -3.290968078514205253 ) ) ;
#80549=AXIS2_PLACEMENT_3D ( 'NONE', #73208, #65585, #96533 ) ;
#80550=CARTESIAN_POINT ( 'NONE',  ( 84.82914023846464602, 43.34880007081749653, 5.509971121964090557 ) ) ;
#80552=CARTESIAN_POINT ( 'NONE',  ( 78.29764689744347095, 61.60233437561736736, 15.79145928805303711 ) ) ;
#80556=CARTESIAN_POINT ( 'NONE',  ( 73.23875918664506912, 64.24404681984078991, -13.68588676845166674 ) ) ;
#80559=CARTESIAN_POINT ( 'NONE',  ( 31.43297906638544603, 41.08080186712595605, -3.090169943749475845 ) ) ;
#80568=CARTESIAN_POINT ( 'NONE',  ( 82.71692427225742961, 49.78115959597967333, 13.75658874660800102 ) ) ;
#80571=CARTESIAN_POINT ( 'NONE',  ( 86.88058850597731464, 45.96296635460476665, 8.956153083123110648 ) ) ;
#80572=CARTESIAN_POINT ( 'NONE',  ( 20.50317736733639506, 20.03677371833801502, 10.00000000000000533 ) ) ;
#80573=CARTESIAN_POINT ( 'NONE',  ( 81.91674078166553841, 41.69822484696639719, 5.406868786614782429 ) ) ;
#80578=CARTESIAN_POINT ( 'NONE',  ( 42.94622797204061726, 25.76426979415093044, 3.090169943749476733 ) ) ;
#80589=CARTESIAN_POINT ( 'NONE',  ( 74.83067777111257612, 53.34009888148298728, 16.53286476888989043 ) ) ;
#80592=ORIENTED_EDGE ( 'NONE', *, *, #59323, .F. ) ;
#80595=CARTESIAN_POINT ( 'NONE',  ( 67.09245893241136116, 67.08985158454382258, -8.602705837570949754 ) ) ;
#80598=DIRECTION ( 'NONE',  ( 0.4996954135095463823, -0.8654978445076774163, -0.03489949670249753444 ) ) ;
#80601=CARTESIAN_POINT ( 'NONE',  ( 23.93942162470478863, 34.79752408145593989, -5.678558825948271327 ) ) ;
#80602=CARTESIAN_POINT ( 'NONE',  ( 33.48063555417975579, 19.73415679381824006, -6.890680421881970419E-14 ) ) ;
#80604=EDGE_CURVE ( 'NONE', #96468, #79874, #57929, .T. ) ;
#80607=CARTESIAN_POINT ( 'NONE',  ( 19.72235211587467063, 17.10170272979926764, -7.433330006724141015 ) ) ;
#80614=CARTESIAN_POINT ( 'NONE',  ( 75.80568730619351925, 63.70677841270451580, -15.10342109092735363 ) ) ;
#80625=CARTESIAN_POINT ( 'NONE',  ( 71.59249531027893454, 71.81680186753220596, -4.291330315329808798 ) ) ;
#80626=CARTESIAN_POINT ( 'NONE',  ( 77.87641386972968860, 61.39850456329286743, -16.14647179981831115 ) ) ;
#80630=DIRECTION ( 'NONE',  ( -0.8660254037844379305, -0.5000000000000014433, -0.000000000000000000 ) ) ;
#80635=CARTESIAN_POINT ( 'NONE',  ( 32.22500930073565684, 40.64646525600392835, -2.839279412974133887 ) ) ;
#80637=CARTESIAN_POINT ( 'NONE',  ( 78.60031580754363745, 47.91716149375564981, -14.46830116769540275 ) ) ;
#80644=CARTESIAN_POINT ( 'NONE',  ( 80.19198528322290542, 56.53738137329634839, -16.16019141255892677 ) ) ;
#80649=CARTESIAN_POINT ( 'NONE',  ( 69.28395859784794197, 69.63058245955254222, -5.196709074601549183 ) ) ;
#80664=CARTESIAN_POINT ( 'NONE',  ( 83.97456745667967937, 42.10302139383830422, 2.974818707872815882 ) ) ;
#80665=EDGE_CURVE ( 'NONE', #58510, #52122, #2090, .T. ) ;
#80666=LINE ( 'NONE', #11243, #94287 ) ;
#80671=CARTESIAN_POINT ( 'NONE',  ( 80.14460775109067470, 57.42271260518928244, -16.59269094194095473 ) ) ;
#80675=DIRECTION ( 'NONE',  ( 0.5000000000000013323, -0.8660254037844378194, 0.000000000000000000 ) ) ;
#80679=EDGE_CURVE ( 'NONE', #35085, #54157, #18542, .T. ) ;
#80685=CARTESIAN_POINT ( 'NONE',  ( 14.21206617776240044, 23.90829794293879118, 10.00000000000000355 ) ) ;
#80693=CARTESIAN_POINT ( 'NONE',  ( 82.70224374152380165, 51.20310041363545395, -14.45093331327230146 ) ) ;
#80701=CARTESIAN_POINT ( 'NONE',  ( 25.36820930315042943, 19.81029122506294726, 8.090169943749479842 ) ) ;
#80702=CARTESIAN_POINT ( 'NONE',  ( 85.94797495143531307, 48.32083425265168586, 12.00338787116683470 ) ) ;
#80704=CARTESIAN_POINT ( 'NONE',  ( 72.07791713363762653, 72.33007614824393272, -3.421992246486540434 ) ) ;
#80706=CARTESIAN_POINT ( 'NONE',  ( 73.76715751097611928, 55.18302132200656018, -16.59786953572997348 ) ) ;
#80709=CARTESIAN_POINT ( 'NONE',  ( 74.78830374546942039, 67.19102293627160805, 12.47204474763305093 ) ) ;
#80712=( BOUNDED_CURVE ( )  B_SPLINE_CURVE ( 2, ( #94728, #7593, #38481, #69395, #999, #11, #46578, #30895, #8106, #23280, #93226, #54169, #77515 ),
 .UNSPECIFIED., .F., .T. ) 
 B_SPLINE_CURVE_WITH_KNOTS ( ( 3, 2, 2, 2, 2, 2, 3 ),
 ( 0.7375000000000000444, 0.7399999999999999911, 0.7449999999999999956, 0.7500000000000000000, 0.7550000000000000044, 0.7600000000000000089, 0.7625000000000000666 ),
 .UNSPECIFIED. ) 
 CURVE ( )  GEOMETRIC_REPRESENTATION_ITEM ( )  RATIONAL_B_SPLINE_CURVE ( ( 0.9755282581475767101, 0.9755282581475772652, 1.000000000000000000, 0.9510565162951535312, 1.000000000000000000, 0.9510565162951535312, 1.000000000000000000, 0.9510565162951535312, 1.000000000000000000, 0.9510565162951535312, 1.000000000000000000, 0.9755282581475761550, 0.9755282581475767101 ) ) 
 REPRESENTATION_ITEM ( '' )  );
#80713=B_SPLINE_CURVE_WITH_KNOTS ( 'NONE', 3,
 ( #84501, #98187, #61647, #83008, #36861, #76854, #5474, #7450, #13580, #75384 ),
 .UNSPECIFIED., .F., .F.,
 ( 4, 2, 2, 2, 4 ),
 ( 0.000000000000000000, 0.2500000000000000000, 0.5000000000000000000, 0.7500000000000000000, 1.000000000000000000 ),
 .UNSPECIFIED. ) ;
#80720=CARTESIAN_POINT ( 'NONE',  ( 36.89851624356406745, 36.70171378149922248, -9.188101187500004485 ) ) ;
#80724=CARTESIAN_POINT ( 'NONE',  ( 33.97448420766330202, 31.56628583063843152, 9.188101187500006262 ) ) ;
#80732=CARTESIAN_POINT ( 'NONE',  ( 2.405479210251257438, 24.49540643055184930, 3.479690158560446702E-15 ) ) ;
#80734=CARTESIAN_POINT ( 'NONE',  ( 11.76515913632831101, 28.83396525600389282, -2.839279412974133887 ) ) ;
#80737=CARTESIAN_POINT ( 'NONE',  ( 84.14312167556933275, 48.98415679381830756, 0.000000000000000000 ) ) ;
#80746=CARTESIAN_POINT ( 'NONE',  ( 66.13301673674520487, 68.52568730408864894, 4.698905408680452922 ) ) ;
#80747=CARTESIAN_POINT ( 'NONE',  ( 87.59998515009166908, 45.09196136326725224, 6.914658723149486264 ) ) ;
#80753=CARTESIAN_POINT ( 'NONE',  ( 85.92471682701912528, 47.57321576112601491, 10.85901928151990958 ) ) ;
#80754=ORIENTED_EDGE ( 'NONE', *, *, #2178, .T. ) ;
#80755=CARTESIAN_POINT ( 'NONE',  ( 78.26871893555610882, 61.06000381536296118, 15.88849461485118297 ) ) ;
#80758=ADVANCED_FACE ( 'NONE', ( #1599 ), #56265, .T. ) ;
#80760=CARTESIAN_POINT ( 'NONE',  ( 77.15553965011207538, 50.73118323507032557, -15.35405348121969560 ) ) ;
#80761=CARTESIAN_POINT ( 'NONE',  ( 80.81174745787325264, 43.46938007122601277, 9.396612886052723823 ) ) ;
#80769=ADVANCED_FACE ( 'NONE', ( #65861 ), #29619, .T. ) ;
#80778=CARTESIAN_POINT ( 'NONE',  ( 69.96053279364318200, 66.30487250405448663, 10.70721000888415020 ) ) ;
#80784=CARTESIAN_POINT ( 'NONE',  ( 30.25295400085950703, 18.26216523072495690, -2.296566073217252530E-15 ) ) ;
#80786=CARTESIAN_POINT ( 'NONE',  ( 77.43554664961604317, 49.73530731850063802, -15.48705580038115848 ) ) ;
#80800=CARTESIAN_POINT ( 'NONE',  ( 14.47246418079440389, 8.759783934591627741, -1.583844403245366905 ) ) ;
#80814=CARTESIAN_POINT ( 'NONE',  ( 25.95703985525452850, 15.39040679176983240, 1.333680081654574804E-15 ) ) ;
#80820=EDGE_CURVE ( 'NONE', #5854, #59206, #78396, .T. ) ;
#80821=CARTESIAN_POINT ( 'NONE',  ( 88.20356954673827943, 44.10112916931887383, 0.5196327138970232573 ) ) ;
#80833=CARTESIAN_POINT ( 'NONE',  ( 68.48614760541654789, 64.37018547164757365, -12.30469093693554150 ) ) ;
#80841=ORIENTED_EDGE ( 'NONE', *, *, #41016, .T. ) ;
#80843=CARTESIAN_POINT ( 'NONE',  ( 83.36691583440136810, 43.49436753249096910, 8.332904630864705453 ) ) ;
#80845=CARTESIAN_POINT ( 'NONE',  ( 25.00689474275853286, 16.29860640527292759, -2.839279412974138328 ) ) ;
#80846=CARTESIAN_POINT ( 'NONE',  ( 74.83456390391278035, 67.20231954166843025, 12.48272054267759046 ) ) ;
#80850=CYLINDRICAL_SURFACE ( 'NONE', #80549, 16.60714546451156792 ) ;
#80856=CARTESIAN_POINT ( 'NONE',  ( 81.71476302640699885, 55.72971451982099467, -15.98982683184117448 ) ) ;
#80860=CARTESIAN_POINT ( 'NONE',  ( 71.87514149713709344, 72.22094621771665857, 0.5828543197166242695 ) ) ;
#80861=CARTESIAN_POINT ( 'NONE',  ( 84.75074989694867611, 43.95653813994506720, 6.843521681741808749 ) ) ;
#80864=CARTESIAN_POINT ( 'NONE',  ( 71.98137461515177904, 71.49844079294172161, -5.753101040561137580 ) ) ;
#80868=CARTESIAN_POINT ( 'NONE',  ( 8.974214183003983436, 13.38052372038638538, 10.00000000000000533 ) ) ;
#80870=EDGE_LOOP ( 'NONE', ( #68467, #77880, #65277, #51449 ) ) ;
#80877=CARTESIAN_POINT ( 'NONE',  ( 79.27109561811333549, 59.78567773455861811, 16.51039248270449633 ) ) ;
#80882=CARTESIAN_POINT ( 'NONE',  ( 73.47333430897622009, 69.87645613598228067, -9.771583980831868743 ) ) ;
#80883=CARTESIAN_POINT ( 'NONE',  ( 84.68112478133504339, 49.92754082849447883, -13.65492077727069820 ) ) ;
#80885=ORIENTED_EDGE ( 'NONE', *, *, #69723, .F. ) ;
#80890=EDGE_LOOP ( 'NONE', ( #29958, #55245, #55726, #56094 ) ) ;
#80891=CARTESIAN_POINT ( 'NONE',  ( 81.53393849378393554, 59.50339463092494441, -0.2795964517353782819 ) ) ;
#80897=CARTESIAN_POINT ( 'NONE',  ( 82.16505394594395284, 40.63743801994069571, 3.475557980665269664 ) ) ;
#80905=CARTESIAN_POINT ( 'NONE',  ( 70.40520854310760512, 61.17034131612381032, -14.85613665266377836 ) ) ;
#80906=CARTESIAN_POINT ( 'NONE',  ( 6.965323710529800927, 24.99752408145590366, 5.678558825948277544 ) ) ;
#80909=CARTESIAN_POINT ( 'NONE',  ( 85.61005001132002690, 48.37664482377094544, -12.20733655019925479 ) ) ;
#80920=ORIENTED_EDGE ( 'NONE', *, *, #15071, .F. ) ;
#80922=ADVANCED_FACE ( 'NONE', ( #27266 ), #58634, .T. ) ;
#80923=CARTESIAN_POINT ( 'NONE',  ( 66.13011622596867767, 68.75667804639587644, 0.07765751491501762804 ) ) ;
#80929=CARTESIAN_POINT ( 'NONE',  ( 87.04122873496829982, 46.31593380912286761, -9.298662157179395038 ) ) ;
#80933=CARTESIAN_POINT ( 'NONE',  ( 88.35595341439740480, 43.98873182231152157, 2.401576318819961919 ) ) ;
#80936=CARTESIAN_POINT ( 'NONE',  ( 73.35598197599438208, 62.01013554246837600, -14.72002716710399817 ) ) ;
#80938=CARTESIAN_POINT ( 'NONE',  ( 80.09759165418883242, 58.14035731840515098, 16.26729025684296204 ) ) ;
#80939=CARTESIAN_POINT ( 'NONE',  ( 72.81152980648018058, 65.70600229248903190, -12.63635638373012782 ) ) ;
#80941=CARTESIAN_POINT ( 'NONE',  ( 81.08346246620165232, 43.41693178244018014, -9.956532816971719768 ) ) ;
#80946=CARTESIAN_POINT ( 'NONE',  ( 87.98075804981249348, 44.53981909570472908, -3.999110579342586291 ) ) ;
#80949=CYLINDRICAL_SURFACE ( 'NONE', #33460, 10.00000000000001066 ) ;
#80950=CARTESIAN_POINT ( 'NONE',  ( 76.48640248419295062, 51.58918322513654431, 15.64831315713033355 ) ) ;
#80956=CARTESIAN_POINT ( 'NONE',  ( 81.49432349081075699, 53.73119012861440780, -15.59150876117132256 ) ) ;
#80968=CARTESIAN_POINT ( 'NONE',  ( 29.46033357383057449, 37.98502408145594700, -5.678558825948271327 ) ) ;
#80970=CARTESIAN_POINT ( 'NONE',  ( 43.87294039959300562, 25.73415679381825427, 1.333680081654574804E-15 ) ) ;
#80972=CARTESIAN_POINT ( 'NONE',  ( 17.24455747906367264, 28.14336893147755347, 7.433330006724141015 ) ) ;
#80978=CARTESIAN_POINT ( 'NONE',  ( 86.37991722458738764, 47.25272401055813276, 10.79753792097408116 ) ) ;
#80980=CARTESIAN_POINT ( 'NONE',  ( 72.47349332888545348, 71.58927234190268507, 5.197985995894253364 ) ) ;
#80983=CARTESIAN_POINT ( 'NONE',  ( 74.73210197474243444, 53.53813011673200606, 16.07754455680917616 ) ) ;
#80989=CARTESIAN_POINT ( 'NONE',  ( 72.61953979799211822, 57.46676429237049177, -16.31386327007983539 ) ) ;
#80998=CARTESIAN_POINT ( 'NONE',  ( 82.78738711968594544, 46.53022027656172099, 12.04865083719906593 ) ) ;
#81000=CARTESIAN_POINT ( 'NONE',  ( 37.18115723113500337, 22.26216523072496756, -2.296566073217252530E-15 ) ) ;
#81001=CARTESIAN_POINT ( 'NONE',  ( 74.41277528214355641, 60.17971584258503270, -15.50566959064950190 ) ) ;
#81009=ADVANCED_FACE ( 'NONE', ( #29288 ), #60153, .T. ) ;
#81013=CARTESIAN_POINT ( 'NONE',  ( 85.74798619856123594, 48.50762779557322801, -11.78128263942436327 ) ) ;
#81017=CARTESIAN_POINT ( 'NONE',  ( 87.51647913336857698, 44.56403561216112053, 4.883618514853080406 ) ) ;
#81022=EDGE_LOOP ( 'NONE', ( #150, #26002, #52876, #73063 ) ) ;
#81041=CARTESIAN_POINT ( 'NONE',  ( 69.77718044168689460, 69.34802543791555252, -6.518941176212923239 ) ) ;
#81043=CARTESIAN_POINT ( 'NONE',  ( 69.53286917118612109, 63.07419471374822706, -13.61637355923466686 ) ) ;
#81048=CARTESIAN_POINT ( 'NONE',  ( 80.71282890952170419, 45.80828928750833029, 11.77677843188879869 ) ) ;
#81049=CARTESIAN_POINT ( 'NONE',  ( 82.06353261700769508, 41.00057011406288154, -2.892018250819526237 ) ) ;
#81056=CARTESIAN_POINT ( 'NONE',  ( 67.21612508256824015, 69.36607345415896475, -0.9029263575005446185 ) ) ;
#81058=CARTESIAN_POINT ( 'NONE',  ( 83.38731009417298878, 51.80618739314797239, 14.97569794390972575 ) ) ;
#81063=CARTESIAN_POINT ( 'NONE',  ( 71.50988583758216066, 64.67014808439049034, -12.78853484773171978 ) ) ;
#81066=CARTESIAN_POINT ( 'NONE',  ( 34.99667586858890189, 35.90829794293883737, 10.00000000000000355 ) ) ;
#81070=CARTESIAN_POINT ( 'NONE',  ( 84.78050178888084076, 43.36151058244004020, -5.604529421430612501 ) ) ;
#81072=CARTESIAN_POINT ( 'NONE',  ( 68.47825347583855660, 69.28228719442910233, 6.190467033948801046 ) ) ;
#81074=CARTESIAN_POINT ( 'NONE',  ( 87.37996854902368682, 45.84054858551529321, 8.374939902689632731 ) ) ;
#81077=CARTESIAN_POINT ( 'NONE',  ( 82.35222073790458808, 41.40766035265922795, 5.511273014246758528 ) ) ;
#81081=CARTESIAN_POINT ( 'NONE',  ( 36.97850982526662023, 33.30066082961424456, -10.00000000000000533 ) ) ;
#81085=CARTESIAN_POINT ( 'NONE',  ( 69.10630519318601728, 67.88941290928615047, -8.241121219118390684 ) ) ;
#81086=CARTESIAN_POINT ( 'NONE',  ( 87.17079100176395912, 46.10763928714972337, -8.270830193046910139 ) ) ;
#81087=CARTESIAN_POINT ( 'NONE',  ( 83.95452371275135306, 51.84303909528518517, 14.85259985614519884 ) ) ;
#81089=CARTESIAN_POINT ( 'NONE',  ( 87.57362070123205910, 45.45821687468009742, -6.782828800802978897 ) ) ;
#81091=CARTESIAN_POINT ( 'NONE',  ( 74.81623774949822803, 53.43188568764122692, 16.54077080093535557 ) ) ;
#81098=CARTESIAN_POINT ( 'NONE',  ( 67.43651257506147090, 67.25343589811649281, -8.652612161161503224 ) ) ;
#81099=EDGE_LOOP ( 'NONE', ( #99760, #89190, #54139, #51928 ) ) ;
#81103=CARTESIAN_POINT ( 'NONE',  ( 26.87427219475921092, 30.91421378149919974, 9.188101187500008038 ) ) ;
#81105=CARTESIAN_POINT ( 'NONE',  ( 86.46843151262319793, 47.10573899677975618, -10.05275782589266065 ) ) ;
#81108=CARTESIAN_POINT ( 'NONE',  ( 15.18774714507562962, 26.95586893147754992, 7.433330006724141015 ) ) ;
#81111=CARTESIAN_POINT ( 'NONE',  ( 20.80527494242019060, 12.41603393254324494, -1.583844403245362020 ) ) ;
#81118=EDGE_LOOP ( 'NONE', ( #93173, #25531, #66717, #29634 ) ) ;
#81119=ORIENTED_EDGE ( 'NONE', *, *, #92211, .F. ) ;
#81124=CARTESIAN_POINT ( 'NONE',  ( 65.82416590051595051, 68.93390312404366682, -2.375186792701355021 ) ) ;
#81125=EDGE_CURVE ( 'NONE', #41317, #99059, #50462, .T. ) ;
#81127=CARTESIAN_POINT ( 'NONE',  ( 72.77243010704501103, 56.90600714599002430, -15.93123261131951196 ) ) ;
#81128=CARTESIAN_POINT ( 'NONE',  ( 78.17919853682799669, 61.76234676664309120, -16.10619035535653509 ) ) ;
#81136=CARTESIAN_POINT ( 'NONE',  ( 34.79119414172389213, 25.80170272979928470, 7.433330006724137462 ) ) ;
#81138=CARTESIAN_POINT ( 'NONE',  ( 75.22346589584923038, 66.43729998232824130, -13.15201661418532098 ) ) ;
#81149=CARTESIAN_POINT ( 'NONE',  ( 70.75593123090459358, 69.82372255332346356, -6.700183475668088917 ) ) ;
#81162=CARTESIAN_POINT ( 'NONE',  ( 82.89276890572784851, 41.25948029148610630, 1.516552898798564364 ) ) ;
#81164=B_SPLINE_CURVE_WITH_KNOTS ( 'NONE', 3,
 ( #45623, #76552, #98868, #13745, #69436, #30438, #92772, #37039, #61327, #61821 ),
 .UNSPECIFIED., .F., .F.,
 ( 4, 2, 2, 2, 4 ),
 ( 0.000000000000000000, 0.0002622400424273282080, 0.0005244800848546564160, 0.0007867201272819846240, 0.001048960169709312832 ),
 .UNSPECIFIED. ) ;
#81166=CARTESIAN_POINT ( 'NONE',  ( 75.40315211601793521, 64.63645072480072429, 14.18768813069354273 ) ) ;
#81170=CARTESIAN_POINT ( 'NONE',  ( 80.17693862949111860, 57.41387879531588112, -16.59169664258510224 ) ) ;
#81174=B_SPLINE_CURVE_WITH_KNOTS ( 'NONE', 3,
 ( #597, #68001, #15278, #92829, #46173, #98925, #62374, #30992, #60379, #52785, #76131, #68492, #41074, #2109, #87774, #64905, #49691, #39567, #95363, #2616, #86253, #94831, #63397, #9724, #1105, #71519, #86758, #17292, #33504, #64399, #71019, #9201, #32505, #42089, #65885, #20304, #74519, #27406, #20809, #5098, #65394, #96335, #82145, #82650, #11712, #58285 ),
 .UNSPECIFIED., .F., .F.,
 ( 4, 1, 1, 1, 2, 2, 1, 1, 1, 2, 2, 1, 1, 2, 2, 1, 1, 2, 2, 1, 1, 2, 2, 1, 2, 2, 1, 2, 2, 4 ),
 ( 0.000000000000000000, 0.06250000000001434963, 0.09375000000002152445, 0.1093750000000235229, 0.1171875000000245359, 0.1250000000000255351, 0.1875000000000333344, 0.2187500000000385247, 0.2343750000000410505, 0.2421875000000424660, 0.2500000000000439093, 0.3125000000000414113, 0.3437500000000416334, 0.3593750000000416889, 0.3750000000000417999, 0.4375000000000413558, 0.4687500000000399125, 0.4843750000000404676, 0.5000000000000410783, 0.5625000000000393019, 0.5937500000000383027, 0.6093750000000375255, 0.6250000000000367484, 0.6875000000000319744, 0.7187500000000293099, 0.7500000000000267564, 0.8125000000000188738, 0.8437500000000152101, 0.8750000000000114353, 1.000000000000000000 ),
 .UNSPECIFIED. ) ;
#81176=CARTESIAN_POINT ( 'NONE',  ( 68.86548415544730517, 69.78790591026515244, 4.016893358874391140 ) ) ;
#81180=CARTESIAN_POINT ( 'NONE',  ( 17.65531800687426056, 22.14441083166260427, 10.00000000000000533 ) ) ;
#81187=CARTESIAN_POINT ( 'NONE',  ( 80.05875441287906824, 52.08331270771197552, -15.29290510163803418 ) ) ;
#81194=CARTESIAN_POINT ( 'NONE',  ( 86.27526515939862861, 45.76759053229242369, 9.183507728554419103 ) ) ;
#81195=CARTESIAN_POINT ( 'NONE',  ( 22.33482336197099016, 13.86426979415089455, -3.090169943749474069 ) ) ;
#81200=CARTESIAN_POINT ( 'NONE',  ( 73.99193044287086707, 55.63566381354063139, -16.58609767700729165 ) ) ;
#81203=CARTESIAN_POINT ( 'NONE',  ( 76.41665957711717283, 57.56464406158257674, 16.56912583713305764 ) ) ;
#81204=CARTESIAN_POINT ( 'NONE',  ( 34.28597393419622819, 20.76426979415091978, 3.090169943749476733 ) ) ;
#81213=CARTESIAN_POINT ( 'NONE',  ( 32.39518414388500389, 34.10171378149920685, 9.188101187500008038 ) ) ;
#81214=CARTESIAN_POINT ( 'NONE',  ( 19.14394661871191161, 29.79103043416549212, 8.090169943749478065 ) ) ;
#81219=CARTESIAN_POINT ( 'NONE',  ( 2.953350652821653988, 23.74646525600387648, 2.839279412974139660 ) ) ;
#81220=CARTESIAN_POINT ( 'NONE',  ( 71.80888402837305762, 72.55032655444114198, 1.016447747306844285 ) ) ;
#81221=CARTESIAN_POINT ( 'NONE',  ( 15.07467606819624173, 24.10171378149917842, 9.188101187500008038 ) ) ;
#81231=CARTESIAN_POINT ( 'NONE',  ( 66.53923092494953551, 68.73325766750851074, 4.777391229452033095 ) ) ;
#81232=CARTESIAN_POINT ( 'NONE',  ( 87.10876144644647923, 45.29703821539081332, 7.013113301196394644 ) ) ;
#81240=CARTESIAN_POINT ( 'NONE',  ( 77.31184969415271269, 55.15837166631282429, 16.11507958877023583 ) ) ;
#81243=CARTESIAN_POINT ( 'NONE',  ( 30.13164393277487818, 36.13478043621390157, 8.090169943749478065 ) ) ;
#81245=CARTESIAN_POINT ( 'NONE',  ( 77.92555521731604529, 50.51076232770562058, -15.15948202354326568 ) ) ;
#81254=VERTEX_POINT ( 'NONE', #12487 ) ;
#81260=CARTESIAN_POINT ( 'NONE',  ( 88.01831552501732858, 44.11100423982306751, 1.674833614738614695 ) ) ;
#81262=CARTESIAN_POINT ( 'NONE',  ( 82.88482919494256862, 53.69580434870786689, 15.74208873548984400 ) ) ;
#81269=CARTESIAN_POINT ( 'NONE',  ( 19.72598728594001116, 34.49540643055188127, 3.479690158560446702E-15 ) ) ;
#81296=ADVANCED_FACE ( 'NONE', ( #19602 ), #64682, .T. ) ;
#81297=CARTESIAN_POINT ( 'NONE',  ( 73.65729962767424865, 69.49757902785616182, 9.740712345197151123 ) ) ;
#81298=ORIENTED_EDGE ( 'NONE', *, *, #6493, .T. ) ;
#81314=CARTESIAN_POINT ( 'NONE',  ( 83.90681972514065023, 47.04571552257464617, 11.33789640138802035 ) ) ;
#81317=CARTESIAN_POINT ( 'NONE',  ( 68.72553068027684731, 64.68746542795034316, -12.16225929270542494 ) ) ;
#81319=CARTESIAN_POINT ( 'NONE',  ( 80.22169496146727852, 49.80210241725078646, 14.90787428718167185 ) ) ;
#81323=CARTESIAN_POINT ( 'NONE',  ( 69.36807548234968124, 68.59810528570370991, 7.418719991931705948 ) ) ;
#81326=VERTEX_POINT ( 'NONE', #88535 ) ;
#81331=CARTESIAN_POINT ( 'NONE',  ( 16.58664519722142927, 32.68290643055186706, 3.479690158560446702E-15 ) ) ;
#81332=CARTESIAN_POINT ( 'NONE',  ( 74.72957723844164946, 67.16412678672320169, 12.46718536312577719 ) ) ;
#81335=CARTESIAN_POINT ( 'NONE',  ( 75.28739987566954994, 66.81623516066271407, 13.35525127813182067 ) ) ;
#81342=CARTESIAN_POINT ( 'NONE',  ( 81.25101512611533394, 55.44295246005403754, -16.34115372143417133 ) ) ;
#81344=CARTESIAN_POINT ( 'NONE',  ( 70.15248158267399958, 69.03648656905426151, 7.442703178729979996 ) ) ;
#81345=AXIS2_PLACEMENT_3D ( 'NONE', #13888, #36675, #37183 ) ;
#81350=CARTESIAN_POINT ( 'NONE',  ( 85.72180487497212198, 45.58971590517442252, 8.620633354355701883 ) ) ;
#81353=CARTESIAN_POINT ( 'NONE',  ( 71.56199657794928726, 71.97676475843201160, -1.390604029342513925 ) ) ;
#81357=CARTESIAN_POINT ( 'NONE',  ( 4.858991816890471327, 18.50829794293877839, -10.00000000000000355 ) ) ;
#81360=FACE_OUTER_BOUND ( 'NONE', #48594, .T. ) ;
#81365=CARTESIAN_POINT ( 'NONE',  ( 78.96564777457507489, 59.77152385746119023, 16.49451479044647328 ) ) ;
#81369=CARTESIAN_POINT ( 'NONE',  ( 75.05438881318511335, 53.25138768964912828, 16.03402430238056908 ) ) ;
#81372=CARTESIAN_POINT ( 'NONE',  ( 77.77188545216394289, 52.09635595759155535, -15.62539252360470954 ) ) ;
#81377=CARTESIAN_POINT ( 'NONE',  ( 88.48047015690482908, 43.85905421517757929, 0.03257650617625663936 ) ) ;
#81378=ORIENTED_EDGE ( 'NONE', *, *, #3657, .F. ) ;
#81379=CARTESIAN_POINT ( 'NONE',  ( 76.91786011064853312, 49.72511384082106645, 15.07646197409581390 ) ) ;
#81381=CARTESIAN_POINT ( 'NONE',  ( 75.34515349063467227, 60.38358704892218043, 15.60396358203763967 ) ) ;
#81389=CARTESIAN_POINT ( 'NONE',  ( 73.44130805767331083, 68.03446431250019089, -11.12216700113787127 ) ) ;
#81391=VERTEX_POINT ( 'NONE', #39283 ) ;
#81392=CARTESIAN_POINT ( 'NONE',  ( 75.72846040655473132, 54.99831286504160488, 16.13249358657354193 ) ) ;
#81393=CARTESIAN_POINT ( 'NONE',  ( 6.618913549016022912, 24.79752408145590081, -5.678558825948271327 ) ) ;
#81401=CARTESIAN_POINT ( 'NONE',  ( 87.11157952361327261, 44.55241027477293869, 5.348311053102904999 ) ) ;
#81402=CARTESIAN_POINT ( 'NONE',  ( 88.04428041263226135, 44.10238440132638971, -1.708206819958570044 ) ) ;
#81405=CARTESIAN_POINT ( 'NONE',  ( 66.18888642898470209, 69.34007213467177166, 0.2082648703207360674 ) ) ;
#81414=CARTESIAN_POINT ( 'NONE',  ( 88.28948486398485329, 44.33448523864236535, 2.244918718876048214 ) ) ;
#81417=EDGE_LOOP ( 'NONE', ( #65346, #60009, #63235, #67106 ) ) ;
#81418=CARTESIAN_POINT ( 'NONE',  ( 78.84444043921700995, 60.06282491878221919, -16.09152508400769932 ) ) ;
#81420=AXIS2_PLACEMENT_3D ( 'NONE', #21378, #99878, #37066 ) ;
#81422=PLANE ( 'NONE',  #6338 ) ;
#81424=CARTESIAN_POINT ( 'NONE',  ( 80.84042243888920609, 43.63393987770743365, -9.572765014343259438 ) ) ;
#81429=CARTESIAN_POINT ( 'NONE',  ( 87.89481703180801730, 44.20627101738029552, -4.400163950806250668 ) ) ;
#81432=CARTESIAN_POINT ( 'NONE',  ( 77.70006599894800559, 50.25350553986154978, 15.10357061109865917 ) ) ;
#81438=CARTESIAN_POINT ( 'NONE',  ( 84.24654968840980018, 50.62473343291171801, 13.78984717790371661 ) ) ;
#81445=CARTESIAN_POINT ( 'NONE',  ( 83.19206654810436419, 51.10784717693168488, -14.73575672656897240 ) ) ;
#81450=CARTESIAN_POINT ( 'NONE',  ( 79.98829826350832661, 44.59498145193617802, 11.76229303994366049 ) ) ;
#81451=CARTESIAN_POINT ( 'NONE',  ( 38.48863484149603664, 25.14754757982092670, -5.678558825948275768 ) ) ;
#81453=CARTESIAN_POINT ( 'NONE',  ( 76.26946404230704957, 64.97317754398874001, 14.67006731301515998 ) ) ;
#81455=CARTESIAN_POINT ( 'NONE',  ( 22.71615395846560759, 25.06628583063842086, -9.188101187500006262 ) ) ;
#81461=CARTESIAN_POINT ( 'NONE',  ( 74.68164300898216368, 63.81063734443356594, 14.78194474382439694 ) ) ;
#81462=DIRECTION ( 'NONE',  ( 0.4851478631379963491, -0.8403007481384849875, 0.2419218955996714493 ) ) ;
#81466=CARTESIAN_POINT ( 'NONE',  ( 75.11518065281146050, 53.26383345445703554, 16.03154839982004631 ) ) ;
#81471=CARTESIAN_POINT ( 'NONE',  ( 83.08202181667390107, 41.27958953865602609, 0.4477113809661833477 ) ) ;
#81474=B_SPLINE_CURVE_WITH_KNOTS ( 'NONE', 3,
 ( #9080, #70887, #84134, #14683, #45564, #7071, #37956, #41458, #41969, #88637 ),
 .UNSPECIFIED., .F., .F.,
 ( 4, 2, 2, 2, 4 ),
 ( 0.000000000000000000, 0.2500000000000000000, 0.5000000000000000000, 0.7500000000000000000, 1.000000000000000000 ),
 .UNSPECIFIED. ) ;
#81478=CARTESIAN_POINT ( 'NONE',  ( 6.688470478837180266, 19.56454794089038884, 10.00000000000000355 ) ) ;
#81480=CARTESIAN_POINT ( 'NONE',  ( 88.01192408641850307, 44.27121890238829138, -4.391744778743009725 ) ) ;
#81482=VECTOR ( 'NONE', #31187, 1000.000000000000114 ) ;
#81485=CARTESIAN_POINT ( 'NONE',  ( 37.81746515356308436, 24.76004757982092386, 5.678558825948272215 ) ) ;
#81486=CARTESIAN_POINT ( 'NONE',  ( 73.91582071829171241, 60.33129874575597995, -15.38455064745800449 ) ) ;
#81492=CARTESIAN_POINT ( 'NONE',  ( 87.11651898459504650, 46.29685661633757832, -9.218154771921559743 ) ) ;
#81496=CARTESIAN_POINT ( 'NONE',  ( 66.06609959339904492, 68.51740553072025364, -2.387806098926052556 ) ) ;
#81504=ORIENTED_EDGE ( 'NONE', *, *, #82054, .T. ) ;
#81508=CARTESIAN_POINT ( 'NONE',  ( 87.02238245971742003, 45.93041326596856777, -8.141809006855861952 ) ) ;
#81511=CARTESIAN_POINT ( 'NONE',  ( 9.347034241948367850, 24.13478043621386604, 8.090169943749478065 ) ) ;
#81513=B_SPLINE_CURVE_WITH_KNOTS ( 'NONE', 3,
 ( #99709, #36893, #14605, #98730 ),
 .UNSPECIFIED., .F., .F.,
 ( 4, 4 ),
 ( 0.000000000000000000, 0.0003401861652890088511 ),
 .UNSPECIFIED. ) ;
#81521=CARTESIAN_POINT ( 'NONE',  ( 71.84099058795369785, 69.36843466522826418, -8.537052276230351566 ) ) ;
#81528=CARTESIAN_POINT ( 'NONE',  ( 82.50650581714903353, 51.91895525678945233, 14.80017960748231154 ) ) ;
#81529=CARTESIAN_POINT ( 'NONE',  ( 82.41933087055697627, 40.38430946167127900, -0.8419157719606891188 ) ) ;
#81533=CARTESIAN_POINT ( 'NONE',  ( 82.22136387774217781, 40.60583099706693133, -3.205559772122553497 ) ) ;
#81535=CARTESIAN_POINT ( 'NONE',  ( 79.50423164993438263, 48.29920615383874605, 13.87520480776860055 ) ) ;
#81543=CARTESIAN_POINT ( 'NONE',  ( 70.13236730935095409, 70.74420383565504267, -3.402677824215883717 ) ) ;
#81544=FACE_OUTER_BOUND ( 'NONE', #14354, .T. ) ;
#81546=DIRECTION ( 'NONE',  ( -0.8660254037844378194, -0.5000000000000014433, -0.000000000000000000 ) ) ;
#81548=CARTESIAN_POINT ( 'NONE',  ( 32.57180473799248688, 34.50829794293882458, -10.00000000000000355 ) ) ;
#81551=CARTESIAN_POINT ( 'NONE',  ( 86.01409551425155087, 42.49941138162544263, 1.569904702652799910 ) ) ;
#81557=VERTEX_POINT ( 'NONE', #66602 ) ;
#81559=CARTESIAN_POINT ( 'NONE',  ( 86.98337649904340196, 46.47637665038675436, 8.932041053647461482 ) ) ;
#81561=CARTESIAN_POINT ( 'NONE',  ( 38.60757266705294910, 27.45404122711136452, -8.090169943749478065 ) ) ;
#81563=CARTESIAN_POINT ( 'NONE',  ( 87.32537421964468649, 46.00455475262659633, 8.658505635391252397 ) ) ;
#81565=CARTESIAN_POINT ( 'NONE',  ( 39.23990543832260869, 24.78380873178790011, -6.180339887498949025 ) ) ;
#81568=CARTESIAN_POINT ( 'NONE',  ( 87.35606880162970356, 45.77061481740687299, 8.290963297571641633 ) ) ;
#81569=CARTESIAN_POINT ( 'NONE',  ( 70.54949879551072911, 67.86437491032424418, -9.416702132505674783 ) ) ;
#81574=CARTESIAN_POINT ( 'NONE',  ( 87.62133583293774564, 45.31115884160844587, -7.293173845241980757 ) ) ;
#81578=ADVANCED_FACE ( 'NONE', ( #98015 ), #59474, .T. ) ;
#81579=DIRECTION ( 'NONE',  ( -0.8660254037844378194, -0.5000000000000014433, -0.000000000000000000 ) ) ;
#81585=CARTESIAN_POINT ( 'NONE',  ( 67.68514482100738405, 66.83340866827893478, -8.536435324610973652 ) ) ;
#81590=CARTESIAN_POINT ( 'NONE',  ( 29.04415360562664361, 34.95586893147757479, 7.433330006724141015 ) ) ;
#81591=CARTESIAN_POINT ( 'NONE',  ( 72.93270222632347100, 70.75261854202813083, -7.421515863126944446 ) ) ;
#81594=EDGE_LOOP ( 'NONE', ( #67148, #53269, #319, #40051 ) ) ;
#81595=CARTESIAN_POINT ( 'NONE',  ( 16.32921660555538423, 21.37878583063840310, 9.188101187500006262 ) ) ;
#81599=EDGE_CURVE ( 'NONE', #6177, #73699, #82014, .T. ) ;
#81609=CARTESIAN_POINT ( 'NONE',  ( 65.84838944952173279, 68.97303637434430357, -2.219146741909078457 ) ) ;
#81612=CARTESIAN_POINT ( 'NONE',  ( 78.17116731237634042, 61.83023861435394508, -16.09040300007290725 ) ) ;
#81613=CARTESIAN_POINT ( 'NONE',  ( 72.12219891194473576, 72.29872703567703240, -1.398582990988473718 ) ) ;
#81620=CARTESIAN_POINT ( 'NONE',  ( 32.07042461746584650, 33.91421378149919974, 9.188101187500008038 ) ) ;
#81622=CARTESIAN_POINT ( 'NONE',  ( 75.28408590364399799, 66.87309274870622744, -12.87999511164833244 ) ) ;
#81629=ORIENTED_EDGE ( 'NONE', *, *, #23271, .T. ) ;
#81631=EDGE_CURVE ( 'NONE', #315, #20041, #56248, .T. ) ;
#81636=VERTEX_POINT ( 'NONE', #72 ) ;
#81641=CARTESIAN_POINT ( 'NONE',  ( 83.42542119994750749, 51.64995580955420706, -14.90072893730332027 ) ) ;
#81650=CARTESIAN_POINT ( 'NONE',  ( 82.31194215350321031, 44.23274708058759330, -9.322014020231229381 ) ) ;
#81654=CARTESIAN_POINT ( 'NONE',  ( 74.41657139711887226, 59.28711007250513632, 15.72167588865270105 ) ) ;
#81657=CARTESIAN_POINT ( 'NONE',  ( 77.57184175184252695, 61.56740756872861198, 15.71511318425823589 ) ) ;
#81665=CARTESIAN_POINT ( 'NONE',  ( 70.02381739212118816, 70.89375414050529400, 2.247727738370168371 ) ) ;
#81668=EDGE_CURVE ( 'NONE', #84261, #4682, #92791, .T. ) ;
#81669=CARTESIAN_POINT ( 'NONE',  ( 23.90043047733868420, 15.92755873383626408, 6.180339887498953466 ) ) ;
#81673=EDGE_CURVE ( 'NONE', #97425, #7077, #16755, .T. ) ;
#81685=CARTESIAN_POINT ( 'NONE',  ( 19.46394688279507079, 19.43677371833800649, -10.00000000000000355 ) ) ;
#81686=CARTESIAN_POINT ( 'NONE',  ( 85.77117071415351290, 48.61266522586591776, 12.32040783412941920 ) ) ;
#81688=CARTESIAN_POINT ( 'NONE',  ( 72.25715799891941060, 71.93417405212122162, -3.785998945288025830 ) ) ;
#81693=CARTESIAN_POINT ( 'NONE',  ( 75.24745298538975646, 66.90968352439989530, 12.83700467311895999 ) ) ;
#81702=CARTESIAN_POINT ( 'NONE',  ( 79.33995266210858688, 59.84812545430209951, 16.15734818946814144 ) ) ;
#81703=CARTESIAN_POINT ( 'NONE',  ( 38.58005528328081368, 27.98920272979929535, 7.433330006724137462 ) ) ;
#81711=CARTESIAN_POINT ( 'NONE',  ( 21.04482852044473162, 14.01110640527291906, 2.839279412974134775 ) ) ;
#81712=CARTESIAN_POINT ( 'NONE',  ( 71.88106639363310535, 72.58558382077730187, 1.103795272596830968 ) ) ;
#81721=CARTESIAN_POINT ( 'NONE',  ( 68.30695491555283638, 70.04613929395418381, -0.05533233183379759196 ) ) ;
#81722=CARTESIAN_POINT ( 'NONE',  ( 66.37497810201837467, 68.61734744729311331, 4.837691964654595722 ) ) ;
#81723=CARTESIAN_POINT ( 'NONE',  ( 87.22363864817131685, 45.41812704280852131, 7.117319539031738529 ) ) ;
#81730=CARTESIAN_POINT ( 'NONE',  ( 80.73437012277888414, 57.38180594535328538, 16.57560423861647791 ) ) ;
#81732=ORIENTED_EDGE ( 'NONE', *, *, #11590, .T. ) ;
#81733=CARTESIAN_POINT ( 'NONE',  ( 87.64894182299636327, 45.42967476813434757, -6.652927784817597612 ) ) ;
#81734=CARTESIAN_POINT ( 'NONE',  ( 77.58272377184611912, 50.60896635146917077, -15.24740917957588060 ) ) ;
#81735=B_SPLINE_CURVE_WITH_KNOTS ( 'NONE', 3,
 ( #50321, #72663, #73636, #35118, #80277, #58412, #57416, #10842 ),
 .UNSPECIFIED., .F., .F.,
 ( 4, 2, 2, 4 ),
 ( 0.000000000000000000, 0.2371517132195850586, 0.3557275698293775879, 0.4743034264391701171 ),
 .UNSPECIFIED. ) ;
#81737=CARTESIAN_POINT ( 'NONE',  ( 80.64280233791232888, 43.43830871627009316, 9.478028014899054554 ) ) ;
#81752=CARTESIAN_POINT ( 'NONE',  ( 87.14941533941508567, 43.54552546780055877, 0.3078308432578384934 ) ) ;
#81760=LINE ( 'NONE', #43198, #82037 ) ;
#81765=ORIENTED_EDGE ( 'NONE', *, *, #80431, .F. ) ;
#81768=CARTESIAN_POINT ( 'NONE',  ( 82.29245928123272336, 51.99578426057395575, -14.89862599341149263 ) ) ;
#81772=B_SPLINE_CURVE_WITH_KNOTS ( 'NONE', 3,
 ( #90859, #44681, #53294, #6202, #90355, #75126, #68000, #21411, #22399, #37582, #59378, #68491, #29503, #52294, #60378, #20935, #5702, #84247, #36592, #91336, #99417, #29994, #20426, #43190 ),
 .UNSPECIFIED., .F., .F.,
 ( 4, 2, 2, 2, 2, 2, 2, 2, 2, 2, 2, 4 ),
 ( 0.000000000000000000, 0.1249999999999881206, 0.2499999999999762412, 0.3749999999999643618, 0.4374999999999651390, 0.4999999999999659162, 0.5624999999999665823, 0.6249999999999673594, 0.6874999999999680256, 0.7499999999999688027, 0.8749999999999843459, 1.000000000000000000 ),
 .UNSPECIFIED. ) ;
#81778=CARTESIAN_POINT ( 'NONE',  ( 82.39721099668476256, 40.42262220707492304, 1.474573639734339192 ) ) ;
#81783=PLANE ( 'NONE',  #85088 ) ;
#81785=CARTESIAN_POINT ( 'NONE',  ( 84.21326495356250064, 50.60090342464640401, 13.78724288159853728 ) ) ;
#81792=CARTESIAN_POINT ( 'NONE',  ( 74.31200754921134433, 68.46947570921950899, -11.18681609572362134 ) ) ;
#81794=CARTESIAN_POINT ( 'NONE',  ( 74.27061467689566143, 65.15629350404239517, 13.99533241632264158 ) ) ;
#81798=CARTESIAN_POINT ( 'NONE',  ( 68.65239601531978053, 64.10048622081454539, 11.94980523598330358 ) ) ;
#81812=CARTESIAN_POINT ( 'NONE',  ( 73.57209063514699210, 69.79607308722023618, 9.344099467940562675 ) ) ;
#81816=CARTESIAN_POINT ( 'NONE',  ( 71.19846455806460028, 71.21114677313781272, 4.076820472404566686 ) ) ;
#81819=AXIS2_PLACEMENT_3D ( 'NONE', #85628, #17681, #32372 ) ;
#81821=CARTESIAN_POINT ( 'NONE',  ( 83.11015170815555564, 43.06723244532030748, 7.901789092622347965 ) ) ;
#81823=CARTESIAN_POINT ( 'NONE',  ( 31.76189289227714951, 20.19860640527293683, 2.839279412974134775 ) ) ;
#81827=CARTESIAN_POINT ( 'NONE',  ( 75.29548954665729354, 66.77148020061324019, 13.38688763123640690 ) ) ;
#81834=CARTESIAN_POINT ( 'NONE',  ( 81.59199138121388728, 55.54565483415311888, -16.32615847003737741 ) ) ;
#81835=EDGE_LOOP ( 'NONE', ( #17912, #22970, #38051, #92205 ) ) ;
#81836=CARTESIAN_POINT ( 'NONE',  ( 71.92247502996752928, 71.58450950858453155, 4.220300433249585481 ) ) ;
#81838=VECTOR ( 'NONE', #57009, 999.9999999999998863 ) ;
#81839=CARTESIAN_POINT ( 'NONE',  ( 83.62813027309111646, 42.52490326476596039, 5.061828679325668823 ) ) ;
#81840=CARTESIAN_POINT ( 'NONE',  ( 79.81418777460577019, 52.70850083650530848, 15.50782481748570341 ) ) ;
#81843=CARTESIAN_POINT ( 'NONE',  ( 69.97041834188608789, 71.02470767604341972, 1.098024261663877565 ) ) ;
#81847=CARTESIAN_POINT ( 'NONE',  ( 2.161320418471442739, 24.18080186712590418, 3.090169943749475401 ) ) ;
#81849=ORIENTED_EDGE ( 'NONE', *, *, #75290, .F. ) ;
#81853=CARTESIAN_POINT ( 'NONE',  ( 79.15253416805734332, 60.03979343371569399, 16.13189369385897720 ) ) ;
#81862=CARTESIAN_POINT ( 'NONE',  ( 81.50142252913457241, 41.92047369999142603, -7.540709297637336661 ) ) ;
#81865=CARTESIAN_POINT ( 'NONE',  ( 88.44311045277898131, 43.83777140359737956, 0.09123111681703664766 ) ) ;
#81868=ORIENTED_EDGE ( 'NONE', *, *, #6057, .T. ) ;
#81870=CARTESIAN_POINT ( 'NONE',  ( 75.99000472157059960, 63.81542519772441580, 14.67834632195794775 ) ) ;
#81872=ORIENTED_EDGE ( 'NONE', *, *, #30226, .F. ) ;
#81874=CARTESIAN_POINT ( 'NONE',  ( 82.15600053271296588, 41.14106544737295224, 3.251814095246992498 ) ) ;
#81877=EDGE_CURVE ( 'NONE', #96813, #99018, #44452, .T. ) ;
#81882=CARTESIAN_POINT ( 'NONE',  ( 77.17961428966242465, 62.94638840390226164, 15.26134952368941633 ) ) ;
#81883=CARTESIAN_POINT ( 'NONE',  ( 16.02188117849498639, 11.11110640527290983, -2.839279412974138328 ) ) ;
#81890=CARTESIAN_POINT ( 'NONE',  ( 78.55537653917157570, 48.00561504237174404, -13.97647359956260082 ) ) ;
#81891=CARTESIAN_POINT ( 'NONE',  ( 76.28161175289729101, 64.99341775040052482, -14.27466362150210522 ) ) ;
#81893=CARTESIAN_POINT ( 'NONE',  ( 81.64977529549180701, 50.14798347333574213, -14.69385758784257767 ) ) ;
#81897=CARTESIAN_POINT ( 'NONE',  ( 84.39300954678499522, 42.06444689919337776, 1.116208777756559023 ) ) ;
#81898=CARTESIAN_POINT ( 'NONE',  ( 88.36930832042526163, 44.08004549128393990, -2.853748190838125254 ) ) ;
#81901=CARTESIAN_POINT ( 'NONE',  ( 66.21124237162977977, 69.35328529186524804, 0.1844046320002812600 ) ) ;
#81906=CARTESIAN_POINT ( 'NONE',  ( 81.38310835580871583, 44.82813863409449340, -10.54473920995311786 ) ) ;
#81909=CARTESIAN_POINT ( 'NONE',  ( 88.48648755238653507, 43.99326657310298572, 1.937087981213218457 ) ) ;
#81918=CARTESIAN_POINT ( 'NONE',  ( 86.81641918289878390, 45.77657501471897206, -8.750901752256124766 ) ) ;
#81921=CARTESIAN_POINT ( 'NONE',  ( 80.70489193592369759, 43.22441507702991004, -9.179128504869353833 ) ) ;
#81922=CARTESIAN_POINT ( 'NONE',  ( 66.30954113569532637, 68.28728378170326607, 3.992301261007330737 ) ) ;
#81927=CARTESIAN_POINT ( 'NONE',  ( 78.24153046963442648, 52.40082309350520973, 15.62826166183230114 ) ) ;
#81929=DIRECTION ( 'NONE',  ( -0.8660254037844379305, -0.5000000000000014433, -0.000000000000000000 ) ) ;
#81932=CARTESIAN_POINT ( 'NONE',  ( 84.41999685182091184, 50.11946239824889915, 13.85565564441014708 ) ) ;
#81937=CARTESIAN_POINT ( 'NONE',  ( 5.721601707324312613, 18.70171378149916563, -9.188101187500004485 ) ) ;
#81941=CARTESIAN_POINT ( 'NONE',  ( 86.26068559980312500, 43.08597108666732112, -0.9339882263466466883 ) ) ;
#81946=CARTESIAN_POINT ( 'NONE',  ( 38.14222467998226307, 24.94754757982092386, 5.678558825948272215 ) ) ;
#81948=CARTESIAN_POINT ( 'NONE',  ( 86.02630325614639162, 46.55013779904520987, -9.649467063894148211 ) ) ;
#81950=CARTESIAN_POINT ( 'NONE',  ( 17.68238808236222326, 31.18502408145591787, 5.678558825948277544 ) ) ;
#81957=CARTESIAN_POINT ( 'NONE',  ( 70.95735205513742017, 61.13278218173532963, 15.00632081318293132 ) ) ;
#81958=CARTESIAN_POINT ( 'NONE',  ( 67.24138620688670187, 66.48174940271749733, -8.670771479132932669 ) ) ;
#81963=CARTESIAN_POINT ( 'NONE',  ( 75.47623563632357957, 53.31721590068422501, 16.49647974421704433 ) ) ;
#81969=CARTESIAN_POINT ( 'NONE',  ( 85.69585619780065144, 43.36699593673009190, 4.244564163715101479 ) ) ;
#81971=CARTESIAN_POINT ( 'NONE',  ( 86.32087919958600253, 43.16070745389085772, 1.433418542445278776 ) ) ;
#81973=CARTESIAN_POINT ( 'NONE',  ( 72.16868224958085420, 71.71251872039211150, 5.498261171115576218 ) ) ;
#81976=CARTESIAN_POINT ( 'NONE',  ( 88.11938802471243548, 44.55983648551643483, -5.053413235213815469 ) ) ;
#81981=CARTESIAN_POINT ( 'NONE',  ( 28.60632300232808589, 31.91421378149921040, 9.188101187500008038 ) ) ;
#81983=CARTESIAN_POINT ( 'NONE',  ( 73.23331724570277856, 60.52924755718257188, -15.20160680498939598 ) ) ;
#81986=CARTESIAN_POINT ( 'NONE',  ( 87.60638430035473334, 45.49210694301174840, 6.833128380864941676 ) ) ;
#81990=FACE_OUTER_BOUND ( 'NONE', #21298, .T. ) ;
#81993=CARTESIAN_POINT ( 'NONE',  ( 85.74084692921037743, 48.48815037812249784, -11.76915627900790540 ) ) ;
#81996=CARTESIAN_POINT ( 'NONE',  ( 82.35755591800861453, 40.39341603438295891, 1.412376108039225864 ) ) ;
#82003=CARTESIAN_POINT ( 'NONE',  ( 73.99515186948657686, 54.97541550358009488, -16.60506967685200408 ) ) ;
#82006=VERTEX_POINT ( 'NONE', #38430 ) ;
#82009=CARTESIAN_POINT ( 'NONE',  ( 87.02439212704567240, 45.81336919377327632, -8.633490303204487404 ) ) ;
#82014=B_SPLINE_CURVE_WITH_KNOTS ( 'NONE', 3,
 ( #77051, #32464, #25356, #9685, #70456, #62849, #86718, #55238, #62339, #40545, #70980, #55729, #1067, #79101, #63361, #16257, #17775, #54233, #48159, #69457, #1581, #39532, #78580, #8166, #54740, #94301, #31447, #39037, #85726, #71480, #85201, #7660, #38548, #93293, #2075, #9165, #46652, #40039, #69947, #24854, #17254, #93805, #32953, #86219, #23848, #63858 ),
 .UNSPECIFIED., .F., .F.,
 ( 4, 1, 2, 2, 1, 2, 2, 1, 1, 2, 2, 1, 1, 2, 2, 1, 1, 2, 2, 1, 1, 1, 2, 2, 1, 1, 1, 2, 2, 4 ),
 ( 0.000000000000000000, 0.06249999999999159006, 0.09374999999998935574, 0.1249999999999871214, 0.1874999999999826528, 0.2187499999999827915, 0.2499999999999829581, 0.3124999999999871214, 0.3437499999999888978, 0.3593749999999896749, 0.3749999999999904521, 0.4374999999999901190, 0.4687499999999881206, 0.4843749999999875100, 0.4999999999999868994, 0.5624999999999862332, 0.5937499999999877875, 0.6093749999999867883, 0.6249999999999857891, 0.6874999999999792388, 0.7187499999999759082, 0.7343749999999742428, 0.7421874999999752420, 0.7499999999999763522, 0.8124999999999775735, 0.8437499999999800160, 0.8593749999999811262, 0.8671874999999835687, 0.8749999999999859002, 1.000000000000000000 ),
 .UNSPECIFIED. ) ;
#82022=DIRECTION ( 'NONE',  ( -0.9364604334398948238, 0.2023802897980871707, -0.2865031848039503726 ) ) ;
#82032=CARTESIAN_POINT ( 'NONE',  ( 87.97782240006738164, 43.76496563450900368, 2.369043524150745927 ) ) ;
#82037=VECTOR ( 'NONE', #7702, 1000.000000000000114 ) ;
#82038=CARTESIAN_POINT ( 'NONE',  ( 76.37155543872398766, 51.66608632798631362, -16.16864924473253495 ) ) ;
#82042=CARTESIAN_POINT ( 'NONE',  ( 79.30680381492646802, 47.66299911123399369, 13.58578065917975408 ) ) ;
#82045=CARTESIAN_POINT ( 'NONE',  ( 77.76918168362882966, 62.01216915286021703, 15.64204638271909609 ) ) ;
#82050=CARTESIAN_POINT ( 'NONE',  ( 68.81680935467448990, 70.26118697200512031, -1.737775333008780843 ) ) ;
#82053=B_SPLINE_CURVE_WITH_KNOTS ( 'NONE', 3,
 ( #88925, #64555, #9873, #19485, #50341, #11866, #42722, #10363, #33664, #5248, #82791, #43728, #13357, #89407, #98955, #19958, #97471, #50835, #67531, #44221, #81785, #91367, #99451, #45226 ),
 .UNSPECIFIED., .F., .F.,
 ( 4, 2, 2, 2, 2, 2, 2, 2, 2, 2, 2, 4 ),
 ( 0.000000000000000000, 0.1249999999999922839, 0.2499999999999845679, 0.3749999999999768518, 0.4374999999999790723, 0.4999999999999813483, 0.5624999999999835687, 0.6249999999999857891, 0.6874999999999881206, 0.7499999999999903411, 0.8749999999999951150, 1.000000000000000000 ),
 .UNSPECIFIED. ) ;
#82054=EDGE_CURVE ( 'NONE', #48590, #66065, #84410, .T. ) ;
#82056=EDGE_CURVE ( 'NONE', #57272, #53392, #6386, .T. ) ;
#82057=CARTESIAN_POINT ( 'NONE',  ( 33.91574581199579086, 27.78052372038643369, -10.00000000000000355 ) ) ;
#82058=CARTESIAN_POINT ( 'NONE',  ( 76.26965850597605368, 57.48574154835009864, -16.55951103678767566 ) ) ;
#82061=AXIS2_PLACEMENT_3D ( 'NONE', #1546, #24820, #9651 ) ;
#82065=CARTESIAN_POINT ( 'NONE',  ( 68.75998362855375490, 69.65436878770546514, 5.732468190288290799 ) ) ;
#82066=ORIENTED_EDGE ( 'NONE', *, *, #12122, .T. ) ;
#82067=CARTESIAN_POINT ( 'NONE',  ( 86.88781708706541451, 46.48626182808993690, 9.021352103034745440 ) ) ;
#82070=CARTESIAN_POINT ( 'NONE',  ( 40.25072390630947439, 24.20801979619931998, -3.090169943749474069 ) ) ;
#82075=CARTESIAN_POINT ( 'NONE',  ( 8.859747497914600700, 17.06628583063839599, -9.188101187500006262 ) ) ;
#82080=CARTESIAN_POINT ( 'NONE',  ( 24.22498904768565353, 14.39040679176983062, 1.333680081654574804E-15 ) ) ;
#82081=CARTESIAN_POINT ( 'NONE',  ( 87.07068318106846050, 45.96719988987016592, -8.154473134044517124 ) ) ;
#82086=CARTESIAN_POINT ( 'NONE',  ( 38.89349527680885643, 24.58380873178789727, 6.180339887498953466 ) ) ;
#82089=VERTEX_POINT ( 'NONE', #30170 ) ;
#82092=CARTESIAN_POINT ( 'NONE',  ( 67.31420450098354991, 66.64469210376232411, -8.500257707143351382 ) ) ;
#82093=ORIENTED_EDGE ( 'NONE', *, *, #25154, .T. ) ;
#82097=CARTESIAN_POINT ( 'NONE',  ( 32.45774345291223995, 27.24335787977765833, -9.188101187500008038 ) ) ;
#82099=CARTESIAN_POINT ( 'NONE',  ( 86.35226789200304154, 47.00689162210669991, -10.01921365420989751 ) ) ;
#82100=VECTOR ( 'NONE', #631, 1000.000000000000000 ) ;
#82104=CARTESIAN_POINT ( 'NONE',  ( 14.05709621874952475, 23.51421378149918340, -9.188101187500004485 ) ) ;
#82105=CARTESIAN_POINT ( 'NONE',  ( 69.00650497353377943, 64.42272793400444186, 12.49602259808233562 ) ) ;
#82106=CARTESIAN_POINT ( 'NONE',  ( 70.69086365586154841, 70.23154535277738830, -5.847355862645180480 ) ) ;
#82107=CARTESIAN_POINT ( 'NONE',  ( 18.95962131514559346, 16.11029122506294087, -8.090169943749478065 ) ) ;
#82119=CARTESIAN_POINT ( 'NONE',  ( 66.44514283687411194, 68.77124511786847449, -2.157765416611612697 ) ) ;
#82121=CARTESIAN_POINT ( 'NONE',  ( 81.88283113365912413, 55.39261312399677450, 16.27191101227217729 ) ) ;
#82122=CARTESIAN_POINT ( 'NONE',  ( 78.08878743907096975, 62.01730706715306951, -16.03713534414099939 ) ) ;
#82143=CARTESIAN_POINT ( 'NONE',  ( 67.16990927169524639, 66.79708245693808522, -9.067759095298590921 ) ) ;
#82144=VECTOR ( 'NONE', #5540, 1000.000000000000227 ) ;
#82145=CARTESIAN_POINT ( 'NONE',  ( 87.59157332177183264, 43.83901051802146043, -1.268023806040525781 ) ) ;
#82148=EDGE_LOOP ( 'NONE', ( #98581, #50563, #73186, #57152 ) ) ;
#82158=CARTESIAN_POINT ( 'NONE',  ( 85.93878220393966672, 44.20073796858249437, -6.077267220493034472 ) ) ;
#82159=CARTESIAN_POINT ( 'NONE',  ( 86.25488010490016677, 44.66640252382467935, 6.626028542311385827 ) ) ;
#82162=CARTESIAN_POINT ( 'NONE',  ( 74.35132386903860890, 58.97444165883455724, 15.77412187530554810 ) ) ;
#82165=CARTESIAN_POINT ( 'NONE',  ( 77.58957552442460326, 61.75793702469097468, 15.67560070342385892 ) ) ;
#82170=CARTESIAN_POINT ( 'NONE',  ( 73.72368916567589281, 69.52486454841584873, -9.771537494043835537 ) ) ;
#82177=B_SPLINE_SURFACE_WITH_KNOTS ( 'NONE', 3, 1, ( 
 ( #49976, #97594 ),
 ( #42842, #57560 ),
 ( #27686, #3399 ),
 ( #4885, #43853 ),
 ( #81909, #81414 ),
 ( #50958, #34761 ),
 ( #65661, #89527 ),
 ( #35267, #19603 ),
 ( #82428, #74794 ),
 ( #12488, #97118 ),
 ( #96120, #96619 ),
 ( #5372, #27183 ),
 ( #80933, #4369 ),
 ( #88536, #58070 ),
 ( #66663, #20087 ),
 ( #34274, #26674 ),
 ( #43355, #74303 ),
 ( #73286, #98079 ),
 ( #28165, #3878 ),
 ( #11986, #57059 ),
 ( #11502, #73780 ),
 ( #66172, #88041 ),
 ( #59035, #42354 ),
 ( #89053, #50463 ),
 ( #90006, #20581 ),
 ( #51462, #12994 ),
 ( #36255, #18590 ),
 ( #49468, #67158 ),
 ( #80423, #10996 ),
 ( #41868, #61543 ),
 ( #53926, #22053 ) ),
 .UNSPECIFIED., .F., .F., .F.,
 ( 4, 3, 3, 3, 3, 3, 3, 3, 3, 3, 4 ),
 ( 2, 2 ),
 ( 0.000000000000000000, 0.1333490885032350692, 0.3007194338854288218, 0.4699862290245104268, 0.5844252810809298371, 0.6686540514502736787, 0.7354980260655487045, 0.8028463152565475935, 0.8633854507757110497, 0.9437142632667278042, 1.000000000000000000 ),
 ( 0.000000000000000000, 1.000000000000000000 ),
 .UNSPECIFIED. ) ;
#82178=CARTESIAN_POINT ( 'NONE',  ( 17.67616779290014506, 25.90829794293879829, 10.00000000000000355 ) ) ;
#82181=CARTESIAN_POINT ( 'NONE',  ( 71.82585323880603312, 69.27534975156628150, -9.342054464929514523 ) ) ;
#82183=CARTESIAN_POINT ( 'NONE',  ( 72.26713406221064417, 71.94669707650473356, -3.758665421101202497 ) ) ;
#82190=CARTESIAN_POINT ( 'NONE',  ( 66.85524610400480583, 67.34209505064849566, -6.990925417236245387 ) ) ;
#82194=CARTESIAN_POINT ( 'NONE',  ( 86.51006589432671490, 46.32215150632234213, 9.708631656330311444 ) ) ;
#82195=CARTESIAN_POINT ( 'NONE',  ( 27.35777070392073185, 16.76426979415090557, 3.090169943749476733 ) ) ;
#82196=CARTESIAN_POINT ( 'NONE',  ( 85.35998281785300890, 48.55136375776380930, 12.45655298324007632 ) ) ;
#82200=CARTESIAN_POINT ( 'NONE',  ( 74.24029763082349120, 55.47955095029949035, -16.12046342301015045 ) ) ;
#82202=CARTESIAN_POINT ( 'NONE',  ( 74.81309782283618404, 67.19796050844534818, 12.47715916803399772 ) ) ;
#82212=CARTESIAN_POINT ( 'NONE',  ( 79.38761854802169182, 59.75627238307979638, 16.16632707334086660 ) ) ;
#82213=CARTESIAN_POINT ( 'NONE',  ( 36.95804531498377798, 23.19860640527294748, 2.839279412974134775 ) ) ;
#82217=CYLINDRICAL_SURFACE ( 'NONE', #78504, 10.00000000000001066 ) ;
#82219=CARTESIAN_POINT ( 'NONE',  ( 19.86064915544625009, 12.26216523072493914, -2.296566073217252530E-15 ) ) ;
#82220=CARTESIAN_POINT ( 'NONE',  ( 71.47384123275857348, 72.35069954344788812, 1.100233114707620530 ) ) ;
#82221=CARTESIAN_POINT ( 'NONE',  ( 82.43748789999787618, 54.23981479609578571, 15.60310197765542384 ) ) ;
#82224=CARTESIAN_POINT ( 'NONE',  ( 85.66595420452183873, 45.56309184094170206, -8.625663387003578819 ) ) ;
#82225=CARTESIAN_POINT ( 'NONE',  ( 27.11554978534049098, 17.78380873178787525, -6.180339887498949025 ) ) ;
#82226=CARTESIAN_POINT ( 'NONE',  ( 75.20214548854198711, 53.53950986635392439, -16.05195360511178038 ) ) ;
#82232=CARTESIAN_POINT ( 'NONE',  ( 66.39267195988500703, 68.17678030604481876, 4.478186808409195585 ) ) ;
#82240=CARTESIAN_POINT ( 'NONE',  ( 88.44266034405603705, 44.03949081389492903, -2.406584733330055847 ) ) ;
#82242=FACE_OUTER_BOUND ( 'NONE', #46661, .T. ) ;
#82244=EDGE_LOOP ( 'NONE', ( #4416, #36216, #70167, #47036 ) ) ;
#82245=CARTESIAN_POINT ( 'NONE',  ( 87.62084567981032990, 45.15010746144617571, -6.151098611497959112 ) ) ;
#82246=CARTESIAN_POINT ( 'NONE',  ( 81.25234104358975173, 49.54399800360413764, -14.03529770125688181 ) ) ;
#82249=CARTESIAN_POINT ( 'NONE',  ( 81.14511053440421051, 43.10620461581409302, 9.543047636977719961 ) ) ;
#82252=CARTESIAN_POINT ( 'NONE',  ( 74.00425782610878400, 61.02723150855160839, 15.19944699234505059 ) ) ;
#82256=ORIENTED_EDGE ( 'NONE', *, *, #42360, .T. ) ;
#82273=CARTESIAN_POINT ( 'NONE',  ( 75.65057567447028930, 57.49826290993107847, -16.09206823455592783 ) ) ;
#82274=CARTESIAN_POINT ( 'NONE',  ( 39.23990543832261579, 24.78380873178790011, -6.180339887498949025 ) ) ;
#82281=CARTESIAN_POINT ( 'NONE',  ( 71.41026323507222173, 68.20115165556771331, 9.666511346903975621 ) ) ;
#82282=CARTESIAN_POINT ( 'NONE',  ( 86.50265851752267565, 45.17908078762290813, 8.152107817765472220 ) ) ;
#82286=ORIENTED_EDGE ( 'NONE', *, *, #39262, .T. ) ;
#82302=CARTESIAN_POINT ( 'NONE',  ( 82.54945800575664805, 40.79138297396659851, 3.187804637566770349 ) ) ;
#82306=CARTESIAN_POINT ( 'NONE',  ( 74.44157817134914978, 68.05905795514840406, -11.63231436587478740 ) ) ;
#82309=CARTESIAN_POINT ( 'NONE',  ( 81.87824099083694307, 41.25415891943595881, -5.798576102226406626 ) ) ;
#82311=DIRECTION ( 'NONE',  ( -0.8660254037844378194, -0.5000000000000014433, -0.000000000000000000 ) ) ;
#82312=CARTESIAN_POINT ( 'NONE',  ( 74.07465050303007104, 67.87278060087763265, -11.60964415893985624 ) ) ;
#82320=AXIS2_PLACEMENT_3D ( 'NONE', #19336, #96340, #65399 ) ;
#82324=CARTESIAN_POINT ( 'NONE',  ( 70.65694608054928949, 68.85554525066207532, -9.031325040935593407 ) ) ;
#82325=CARTESIAN_POINT ( 'NONE',  ( 79.41031494441635630, 46.40275987550353420, -12.75878103946227782 ) ) ;
#82326=CARTESIAN_POINT ( 'NONE',  ( 71.47130384908417966, 59.27950280012738205, -15.75482166576947662 ) ) ;
#82327=FACE_OUTER_BOUND ( 'NONE', #46911, .T. ) ;
#82332=CARTESIAN_POINT ( 'NONE',  ( 66.34802823334818811, 68.15327646776096060, -4.473378551362304556 ) ) ;
#82338=CARTESIAN_POINT ( 'NONE',  ( 26.45569963029868177, 20.98920272979927049, 7.433330006724137462 ) ) ;
#82344=CARTESIAN_POINT ( 'NONE',  ( 68.43344345364462811, 64.47918733080135212, 12.19408877863543061 ) ) ;
#82353=CARTESIAN_POINT ( 'NONE',  ( 71.47987467218354141, 71.01764064272968824, 5.056666948270793327 ) ) ;
#82354=CARTESIAN_POINT ( 'NONE',  ( 74.32283972735670829, 55.33658384534070507, 16.60204640374922036 ) ) ;
#82355=CARTESIAN_POINT ( 'NONE',  ( 86.07719285220247230, 46.34390285249480002, 9.364539065597575984 ) ) ;
#82358=CARTESIAN_POINT ( 'NONE',  ( 67.91653825465498073, 69.16631803100915477, 4.245417807664631837 ) ) ;
#82362=CARTESIAN_POINT ( 'NONE',  ( 16.59523773630703758, 17.78052372038640172, -10.00000000000000355 ) ) ;
#82365=DIRECTION ( 'NONE',  ( -0.8660254037844377084, -0.5000000000000014433, -0.000000000000000000 ) ) ;
#82366=CARTESIAN_POINT ( 'NONE',  ( 86.54479369881731543, 47.18726309986306688, -10.63286291588201316 ) ) ;
#82382=CARTESIAN_POINT ( 'NONE',  ( 88.35351169220642475, 43.78681510747281180, 0.1754685934989754781 ) ) ;
#82384=CARTESIAN_POINT ( 'NONE',  ( 80.95286987779635979, 48.31441995295947578, 13.44804738609444783 ) ) ;
#82387=CARTESIAN_POINT ( 'NONE',  ( 75.69790233746202546, 62.18877547806692263, 15.18360658727204182 ) ) ;
#82391=CARTESIAN_POINT ( 'NONE',  ( 82.65950105694894035, 40.87543522790844008, 3.277353565571960115 ) ) ;
#82401=CARTESIAN_POINT ( 'NONE',  ( 76.67677140431342764, 59.69997763987031192, 15.91096609934128026 ) ) ;
#82402=CARTESIAN_POINT ( 'NONE',  ( 10.26703877906431472, 17.87878583063839599, -9.188101187500006262 ) ) ;
#82406=VECTOR ( 'NONE', #92975, 1000.000000000000114 ) ;
#82415=CARTESIAN_POINT ( 'NONE',  ( 84.78442088202375260, 42.33400169264517388, 1.646337173112248697 ) ) ;
#82416=CARTESIAN_POINT ( 'NONE',  ( 88.20386072652870268, 44.20680737956164563, -1.789751738150168636 ) ) ;
#82420=CARTESIAN_POINT ( 'NONE',  ( 76.47588893644459063, 61.71057517685051153, -15.49423374570369205 ) ) ;
#82428=CARTESIAN_POINT ( 'NONE',  ( 88.45605923504750479, 44.01628325393264163, 2.215908606781749501 ) ) ;
#82429=AXIS2_PLACEMENT_3D ( 'NONE', #55959, #8394, #7902 ) ;
#82437=CARTESIAN_POINT ( 'NONE',  ( 85.53835401965352503, 48.98340217412621911, -12.70221784291844891 ) ) ;
#82440=CARTESIAN_POINT ( 'NONE',  ( 71.78811623112386542, 71.82131630954249601, 4.652117579582786711 ) ) ;
#82444=CARTESIAN_POINT ( 'NONE',  ( 87.91725590613566510, 44.21674671100767284, -4.392329086374235025 ) ) ;
#82446=CARTESIAN_POINT ( 'NONE',  ( 78.70313684180190705, 54.56738927272936479, 15.99217558139294582 ) ) ;
#82449=CARTESIAN_POINT ( 'NONE',  ( 79.66253929351360341, 53.73098452899868249, -15.77044947192900537 ) ) ;
#82454=FACE_OUTER_BOUND ( 'NONE', #94686, .T. ) ;
#82456=CARTESIAN_POINT ( 'NONE',  ( 18.55511606660780899, 34.21091486745861232, -1.111400068045478839E-16 ) ) ;
#82462=CARTESIAN_POINT ( 'NONE',  ( 4.836955906052805787, 24.83396525600387861, -2.839279412974133887 ) ) ;
#82463=CARTESIAN_POINT ( 'NONE',  ( 68.19017624660753540, 65.83665076471868360, 10.85206676099518752 ) ) ;
#82467=CARTESIAN_POINT ( 'NONE',  ( 82.35782067460354483, 41.89994089823363055, -5.292397707111204497 ) ) ;
#82468=CARTESIAN_POINT ( 'NONE',  ( 75.65669688662353565, 65.40331689797208981, 14.28920693795837593 ) ) ;
#82470=CARTESIAN_POINT ( 'NONE',  ( 36.57256041901661803, 33.06628583063844928, -9.188101187500006262 ) ) ;
#82474=CARTESIAN_POINT ( 'NONE',  ( 28.47099635789628280, 18.29860640527293114, -2.839279412974138328 ) ) ;
#82478=CARTESIAN_POINT ( 'NONE',  ( 70.96223225445140770, 61.14671028016761056, 15.00175667792790968 ) ) ;
#82481=CARTESIAN_POINT ( 'NONE',  ( 72.58717870133969541, 71.54427304635605367, 5.456046482779852269 ) ) ;
#82485=CARTESIAN_POINT ( 'NONE',  ( 88.25688461590929990, 44.25163671709261592, -1.880183453705753127 ) ) ;
#82487=CARTESIAN_POINT ( 'NONE',  ( 84.14312167556933275, 48.98415679381830756, 0.000000000000000000 ) ) ;
#82491=CARTESIAN_POINT ( 'NONE',  ( 81.75211762113612224, 42.34667925476468042, -8.001231807219630454 ) ) ;
#82494=CARTESIAN_POINT ( 'NONE',  ( 88.05624235485146301, 44.55787864911079765, -5.145732200269208079 ) ) ;
#82496=CARTESIAN_POINT ( 'NONE',  ( 88.15573124791052351, 44.39703741701313078, -4.524867680024760475 ) ) ;
#82499=CARTESIAN_POINT ( 'NONE',  ( 32.39821438149254362, 40.74646525600392977, 2.839279412974139660 ) ) ;
#82503=( BOUNDED_CURVE ( )  B_SPLINE_CURVE ( 2, ( #61939, #7253, #22950, #23445, #93398, #54851, #54334, #93906, #32043, #39632, #70553, #85306, #31547 ),
 .UNSPECIFIED., .F., .T. ) 
 B_SPLINE_CURVE_WITH_KNOTS ( ( 3, 2, 2, 2, 2, 2, 3 ),
 ( 0.1625000000000000056, 0.1650000000000000078, 0.1700000000000000122, 0.1749999999999999889, 0.1799999999999999933, 0.1849999999999999978, 0.1875000000000000000 ),
 .UNSPECIFIED. ) 
 CURVE ( )  GEOMETRIC_REPRESENTATION_ITEM ( )  RATIONAL_B_SPLINE_CURVE ( ( 0.9755282581475768211, 0.9755282581475768211, 1.000000000000000000, 0.9510565162951535312, 1.000000000000000000, 0.9510565162951535312, 1.000000000000000000, 0.9510565162951535312, 1.000000000000000000, 0.9510565162951535312, 1.000000000000000000, 0.9755282581475768211, 0.9755282581475768211 ) ) 
 REPRESENTATION_ITEM ( '' )  );
#82510=CARTESIAN_POINT ( 'NONE',  ( 85.94199290331987129, 48.36193870280315110, 12.04004775853120357 ) ) ;
#82512=CARTESIAN_POINT ( 'NONE',  ( 71.11649605149564479, 61.92534502158513021, -14.18178967544274371 ) ) ;
#82516=CARTESIAN_POINT ( 'NONE',  ( 77.16944367370705038, 62.93815415716151307, -15.28450044950025877 ) ) ;
#82524=CARTESIAN_POINT ( 'NONE',  ( 87.18493082415903928, 46.24780984919522808, -8.452580536463766947 ) ) ;
#82536=CARTESIAN_POINT ( 'NONE',  ( 83.08198603362329493, 46.51316202230789543, 11.28621070833093931 ) ) ;
#82538=CARTESIAN_POINT ( 'NONE',  ( 69.39572770259547951, 62.82886628838792120, -13.71575758985256499 ) ) ;
#82542=CARTESIAN_POINT ( 'NONE',  ( 82.08601192207028419, 50.00142036091599351, 14.02437814591130127 ) ) ;
#82543=CARTESIAN_POINT ( 'NONE',  ( 82.40574091212634755, 41.31496069167722851, -3.377884205285225594 ) ) ;
#82548=CARTESIAN_POINT ( 'NONE',  ( 72.04273812837080015, 59.28583566120335036, 15.84548535902080246 ) ) ;
#82549=CARTESIAN_POINT ( 'NONE',  ( 80.65449906233159538, 53.35338484752109167, 15.59324704275317863 ) ) ;
#82550=CARTESIAN_POINT ( 'NONE',  ( 68.38943100534879704, 69.90328650375072073, -2.303593894763091399 ) ) ;
#82553=CARTESIAN_POINT ( 'NONE',  ( 77.78993031024410243, 61.70844822385715389, 16.06828208845740136 ) ) ;
#82566=LINE ( 'NONE', #13129, #96456 ) ;
#82574=CARTESIAN_POINT ( 'NONE',  ( 71.79738241951251609, 72.08784563739403950, -1.676743678701877238 ) ) ;
#82576=CARTESIAN_POINT ( 'NONE',  ( 87.22595043061240005, 46.05622627631750987, 8.811080105847633348 ) ) ;
#82579=CARTESIAN_POINT ( 'NONE',  ( 12.16146256644911539, 9.947547579820877672, 5.678558825948272215 ) ) ;
#82584=CARTESIAN_POINT ( 'NONE',  ( 67.57193167581756654, 67.79594878957911419, -6.919506841086756843 ) ) ;
#82600=CARTESIAN_POINT ( 'NONE',  ( 79.19871682019896753, 45.77535205480253921, -13.02187134424031534 ) ) ;
#82602=CARTESIAN_POINT ( 'NONE',  ( 33.49697393745356777, 27.84335787977765264, 9.188101187500006262 ) ) ;
#82607=CARTESIAN_POINT ( 'NONE',  ( 17.99393647837114329, 33.49540643055186706, 3.479690158560446702E-15 ) ) ;
#82608=CARTESIAN_POINT ( 'NONE',  ( 76.40434453536583703, 62.66765977773136598, 15.20766477907509184 ) ) ;
#82609=CARTESIAN_POINT ( 'NONE',  ( 71.52184754477866591, 70.29122656255715640, -6.759684521044225569 ) ) ;
#82610=CARTESIAN_POINT ( 'NONE',  ( 14.65590419365400798, 24.16454794089040448, -10.00000000000000355 ) ) ;
#82619=ADVANCED_FACE ( 'NONE', ( #69426 ), #67612, .T. ) ;
#82620=CARTESIAN_POINT ( 'NONE',  ( 71.46351114784202707, 64.97172176451604741, 13.12417365010213643 ) ) ;
#82622=CARTESIAN_POINT ( 'NONE',  ( 71.21786832307518011, 71.42957135316279960, -4.816066736783382929 ) ) ;
#82624=CARTESIAN_POINT ( 'NONE',  ( 65.82417520554362511, 68.94067023863627242, -2.334285861092879166 ) ) ;
#82635=VERTEX_POINT ( 'NONE', #87206 ) ;
#82637=VERTEX_POINT ( 'NONE', #79575 ) ;
#82642=ADVANCED_FACE ( 'NONE', ( #65325 ), #13440, .T. ) ;
#82648=ORIENTED_EDGE ( 'NONE', *, *, #95017, .F. ) ;
#82649=CARTESIAN_POINT ( 'NONE',  ( 73.50385191007055141, 63.43673688022664692, -14.15219903627441944 ) ) ;
#82650=CARTESIAN_POINT ( 'NONE',  ( 87.87264940252229906, 43.95799710625667700, -0.8674386733748262746 ) ) ;
#82654=CARTESIAN_POINT ( 'NONE',  ( 72.94880756138117306, 69.80684942108813118, -8.830661643779624370 ) ) ;
#82655=FACE_OUTER_BOUND ( 'NONE', #97460, .T. ) ;
#82656=CARTESIAN_POINT ( 'NONE',  ( 73.99515186948657686, 54.97541550358009488, -16.60506967685200408 ) ) ;
#82657=CARTESIAN_POINT ( 'NONE',  ( 80.38548996768443544, 54.44962404282426149, 16.25868990910755230 ) ) ;
#82663=CARTESIAN_POINT ( 'NONE',  ( 67.27576334028319138, 67.83911610176210161, -7.634865361317446641 ) ) ;
#82666=CARTESIAN_POINT ( 'NONE',  ( 72.89074862266798505, 70.83676290058953384, 7.267550809142558244 ) ) ;
#82669=ORIENTED_EDGE ( 'NONE', *, *, #24798, .F. ) ;
#82673=CARTESIAN_POINT ( 'NONE',  ( 81.07073587917510338, 51.75993004551867926, 15.01386952398517494 ) ) ;
#82674=CARTESIAN_POINT ( 'NONE',  ( 73.72211794458776524, 69.54036169704887982, -9.751718775917950666 ) ) ;
#82680=CARTESIAN_POINT ( 'NONE',  ( 28.12636825332733537, 17.20801979619929512, -3.090169943749474069 ) ) ;
#82683=CARTESIAN_POINT ( 'NONE',  ( 66.52392041426838887, 68.84470833973988135, -4.415679280545959706 ) ) ;
#82690=CARTESIAN_POINT ( 'NONE',  ( 66.81157939586830707, 67.57634921264273942, -6.489721810135971936 ) ) ;
#82694=CARTESIAN_POINT ( 'NONE',  ( 22.35053764064823767, 35.83705186507754803, 3.090169943749475401 ) ) ;
#82695=CARTESIAN_POINT ( 'NONE',  ( 85.31220642273653709, 48.47216915277315508, 12.41700016606928259 ) ) ;
#82697=FACE_OUTER_BOUND ( 'NONE', #58782, .T. ) ;
#82701=EDGE_CURVE ( 'NONE', #92094, #77711, #22364, .T. ) ;
#82709=CARTESIAN_POINT ( 'NONE',  ( 79.13720140929677882, 60.04739137989873399, 16.13033826897202871 ) ) ;
#82710=CARTESIAN_POINT ( 'NONE',  ( 35.85928575902275384, 36.10171378149922106, 9.188101187500008038 ) ) ;
#82717=CARTESIAN_POINT ( 'NONE',  ( 13.45569633750675465, 25.95586893147754282, 7.433330006724141015 ) ) ;
#82718=CARTESIAN_POINT ( 'NONE',  ( 71.95794525336515335, 72.58301972798899726, 1.600903759350515543 ) ) ;
#82719=CARTESIAN_POINT ( 'NONE',  ( 82.69645212816358537, 54.02937911834194296, 15.50030166553341004 ) ) ;
#82725=CARTESIAN_POINT ( 'NONE',  ( 81.38228331523285419, 42.18052851735775732, 8.075145019535051816 ) ) ;
#82729=CARTESIAN_POINT ( 'NONE',  ( 66.64262941566822462, 68.29515624540186991, 4.552616485263072832 ) ) ;
#82739=CARTESIAN_POINT ( 'NONE',  ( 81.45669997382150029, 55.98862135975878118, -16.04303691645969820 ) ) ;
#82741=VERTEX_POINT ( 'NONE', #53571 ) ;
#82745=CARTESIAN_POINT ( 'NONE',  ( 81.29539683307429243, 43.25976067956239035, 9.624898955646088439 ) ) ;
#82746=ORIENTED_EDGE ( 'NONE', *, *, #1249, .F. ) ;
#82758=ORIENTED_EDGE ( 'NONE', *, *, #29825, .T. ) ;
#82767=CARTESIAN_POINT ( 'NONE',  ( 74.73127975335565054, 57.80664375811601019, -15.99177344183713778 ) ) ;
#82770=CARTESIAN_POINT ( 'NONE',  ( 67.11701428173226702, 66.86566084198229021, 8.934729829905201370 ) ) ;
#82772=CARTESIAN_POINT ( 'NONE',  ( 84.74721491826518616, 41.70368105205244547, 1.055763243526395279 ) ) ;
#82776=CARTESIAN_POINT ( 'NONE',  ( 76.79673682827939274, 53.97105271787633285, -16.03547630156775838 ) ) ;
#82778=CARTESIAN_POINT ( 'NONE',  ( 78.94111852906270599, 46.22145796229974479, 12.82134408105561363 ) ) ;
#82780=FACE_OUTER_BOUND ( 'NONE', #595, .T. ) ;
#82784=CARTESIAN_POINT ( 'NONE',  ( 84.22619167544027619, 44.03813768368893022, 8.426601908164510490 ) ) ;
#82791=CARTESIAN_POINT ( 'NONE',  ( 84.60621859610353113, 50.62332914066485756, 13.66912872509914578 ) ) ;
#82799=CARTESIAN_POINT ( 'NONE',  ( 81.75715262849954001, 41.47753617486669242, -5.100220969704232665 ) ) ;
#82800=CARTESIAN_POINT ( 'NONE',  ( 14.38368916104982986, 8.708529653044781327, 1.583844403245360466 ) ) ;
#82804=VERTEX_POINT ( 'NONE', #38869 ) ;
#82806=EDGE_CURVE ( 'NONE', #14068, #63364, #99904, .T. ) ;
#82810=CARTESIAN_POINT ( 'NONE',  ( 5.287540158160898507, 21.79103043416546726, 8.090169943749478065 ) ) ;
#82812=CARTESIAN_POINT ( 'NONE',  ( 71.50282862545680018, 59.38978230636582367, -15.72801454580908320 ) ) ;
#82813=CARTESIAN_POINT ( 'NONE',  ( 71.98214240380765716, 72.19672774639096247, -1.652923604091230958 ) ) ;
#82816=CARTESIAN_POINT ( 'NONE',  ( 72.49386282319787256, 57.57572440859878071, 15.80166580940836596 ) ) ;
#82826=CARTESIAN_POINT ( 'NONE',  ( 26.50621139815081762, 30.70171378149920471, -9.188101187500004485 ) ) ;
#82828=CARTESIAN_POINT ( 'NONE',  ( 83.44578961920555571, 51.64149152686551503, -14.89211022975658949 ) ) ;
#82830=CARTESIAN_POINT ( 'NONE',  ( 81.65971250072203702, 41.57115319798205633, -5.463628752668030053 ) ) ;
#82840=CARTESIAN_POINT ( 'NONE',  ( 68.91246633537454613, 66.80396089893802980, 9.505547287390900379 ) ) ;
#82842=CARTESIAN_POINT ( 'NONE',  ( 71.71444459471545940, 72.49928141732988252, 0.9658765412761323166 ) ) ;
#82848=PLANE ( 'NONE',  #30553 ) ;
#82851=CARTESIAN_POINT ( 'NONE',  ( 13.51924585473484974, 23.50829794293879615, -10.00000000000000355 ) ) ;
#82852=CARTESIAN_POINT ( 'NONE',  ( 82.56691085815100450, 44.30186147993075707, 9.990707220731064098 ) ) ;
#82855=CARTESIAN_POINT ( 'NONE',  ( 86.25376498619890242, 46.94328282020536136, -10.55339115541320538 ) ) ;
#82866=CARTESIAN_POINT ( 'NONE',  ( 81.53115339417709606, 41.92267797689947884, -7.515177224797632505 ) ) ;
#82869=EDGE_LOOP ( 'NONE', ( #37478, #33974, #67076, #70624, #73768 ) ) ;
#82872=CARTESIAN_POINT ( 'NONE',  ( 81.78568384109607337, 51.89477062050791289, 14.95452106162773198 ) ) ;
#82874=CARTESIAN_POINT ( 'NONE',  ( 75.29381676803062362, 60.13143282175177973, 15.65255259757436512 ) ) ;
#82879=CARTESIAN_POINT ( 'NONE',  ( 72.97361289423018604, 68.13649966853542139, -10.75395737491361814 ) ) ;
#82882=CARTESIAN_POINT ( 'NONE',  ( 76.56819355343940003, 59.09054857262015759, 15.98656334013552893 ) ) ;
#82883=CARTESIAN_POINT ( 'NONE',  ( 14.66449673273962340, 9.262165230724928477, -2.296566073217252530E-15 ) ) ;
#82889=CARTESIAN_POINT ( 'NONE',  ( 70.98683038387876820, 61.11472152276905234, -14.49225651734632692 ) ) ;
#82895=CARTESIAN_POINT ( 'NONE',  ( 88.42385336119198769, 44.01808410483894107, -2.342466917228906098 ) ) ;
#82899=CARTESIAN_POINT ( 'NONE',  ( 70.24152351796814742, 63.55507216885125388, -13.00701345941583575 ) ) ;
#82905=CARTESIAN_POINT ( 'NONE',  ( 84.35687393656843369, 44.63875131664023854, -8.325067569704064141 ) ) ;
#82908=CARTESIAN_POINT ( 'NONE',  ( 76.03019726450892790, 65.44783958900880805, 14.37600347258596045 ) ) ;
#82916=CARTESIAN_POINT ( 'NONE',  ( 85.84416675550359344, 42.93383034132180143, 1.917673184544592013 ) ) ;
#82917=CARTESIAN_POINT ( 'NONE',  ( 83.86430188519919682, 45.36457422996819133, 9.662219384362932928 ) ) ;
#82923=CARTESIAN_POINT ( 'NONE',  ( 78.71261887716285344, 54.61647413563439812, 15.99851350793635518 ) ) ;
#82926=CARTESIAN_POINT ( 'NONE',  ( 80.53132723571809493, 53.42204839544174888, -15.60352693426686699 ) ) ;
#82930=CARTESIAN_POINT ( 'NONE',  ( 84.71425524834847920, 50.25098136614051469, 13.83365903171529077 ) ) ;
#82939=EDGE_CURVE ( 'NONE', #57243, #13423, #57568, .T. ) ;
#82943=VECTOR ( 'NONE', #30642, 1000.000000000000114 ) ;
#82949=CARTESIAN_POINT ( 'NONE',  ( 42.56377214068922399, 30.28920272979930672, -7.433330006724141015 ) ) ;
#82953=CARTESIAN_POINT ( 'NONE',  ( 25.31423016981892715, 26.56628583063841731, 9.188101187500006262 ) ) ;
#82957=CARTESIAN_POINT ( 'NONE',  ( 70.76797951062305003, 60.86569645529516492, 14.54278018258353988 ) ) ;
#82958=CARTESIAN_POINT ( 'NONE',  ( 75.84431516675671503, 65.82088634210550993, -14.12726274127321169 ) ) ;
#82963=CARTESIAN_POINT ( 'NONE',  ( 88.19053702688614749, 44.32527345396092500, -2.493626234014364673 ) ) ;
#82964=ORIENTED_EDGE ( 'NONE', *, *, #77623, .T. ) ;
#82965=CARTESIAN_POINT ( 'NONE',  ( 84.37861180241492320, 46.14357002009968056, -10.86416137306961360 ) ) ;
#82971=ORIENTED_EDGE ( 'NONE', *, *, #49674, .T. ) ;
#82978=CARTESIAN_POINT ( 'NONE',  ( 39.89592612264573290, 25.96004757982093025, -5.678558825948275768 ) ) ;
#82979=CARTESIAN_POINT ( 'NONE',  ( 71.19423160720042176, 61.06544498174218916, -14.56549237402769670 ) ) ;
#82989=CARTESIAN_POINT ( 'NONE',  ( 73.46416042179349404, 61.28524521429519467, -15.02223754724939653 ) ) ;
#82992=CARTESIAN_POINT ( 'NONE',  ( 77.07143086693146472, 63.53409821367920784, -15.43182057973166188 ) ) ;
#83002=CARTESIAN_POINT ( 'NONE',  ( 87.17963343274935539, 46.25680430639528140, -9.118192349661992324 ) ) ;
#83003=VECTOR ( 'NONE', #54875, 1000.000000000000114 ) ;
#83007=CARTESIAN_POINT ( 'NONE',  ( 26.05686017436622137, 36.81751292744056769, -6.180339887498951690 ) ) ;
#83008=CARTESIAN_POINT ( 'NONE',  ( 73.83400387536809717, 55.06300064600840471, -16.12704957102858572 ) ) ;
#83017=CARTESIAN_POINT ( 'NONE',  ( 67.31170132302078457, 68.89449653470401813, -3.954031917524302386 ) ) ;
#83024=CARTESIAN_POINT ( 'NONE',  ( 82.33638059893669947, 51.07561602432041781, 14.47696974499355704 ) ) ;
#83025=CARTESIAN_POINT ( 'NONE',  ( 82.16331024188988863, 41.19762905728452296, -3.464377343443369561 ) ) ;
#83028=CYLINDRICAL_SURFACE ( 'NONE', #12791, 16.60714546451156792 ) ;
#83029=CARTESIAN_POINT ( 'NONE',  ( 83.71913944427328147, 44.06062028468042513, 7.985639216668514173 ) ) ;
#83030=FACE_OUTER_BOUND ( 'NONE', #58124, .T. ) ;
#83033=CARTESIAN_POINT ( 'NONE',  ( 69.64148527851303072, 70.32813841140065847, -3.761399768473041139 ) ) ;
#83043=CARTESIAN_POINT ( 'NONE',  ( 43.28410984748890655, 30.15404122711137447, 8.090169943749479842 ) ) ;
#83046=CARTESIAN_POINT ( 'NONE',  ( 72.26765824385677206, 72.08528386863294202, 3.191945267484126880 ) ) ;
#83050=CARTESIAN_POINT ( 'NONE',  ( 24.34666095796415419, 37.55466486950700755, 7.012934429366973338E-14 ) ) ;
#83051=CARTESIAN_POINT ( 'NONE',  ( 46.16810866859812990, 28.78380873178791077, -6.180339887498949025 ) ) ;
#83053=CARTESIAN_POINT ( 'NONE',  ( 71.91369179320692240, 72.15417514627694118, -1.685444156100106561 ) ) ;
#83055=CARTESIAN_POINT ( 'NONE',  ( 20.80007953598619608, 32.98502408145592568, -5.678558825948271327 ) ) ;
#83058=CARTESIAN_POINT ( 'NONE',  ( 46.99896066727236388, 26.94473085651396360, 1.475505719884397138E-15 ) ) ;
#83062=CARTESIAN_POINT ( 'NONE',  ( 72.50355919934736448, 61.03236684371051268, 14.88608095558173439 ) ) ;
#83067=CARTESIAN_POINT ( 'NONE',  ( 82.14913611300819696, 41.13495720016906887, 3.242338130973200894 ) ) ;
#83068=CARTESIAN_POINT ( 'NONE',  ( 87.70552531824185394, 45.34611373530315603, -6.437115693456841647 ) ) ;
#83073=AXIS2_PLACEMENT_3D ( 'NONE', #85965, #46371, #9913 ) ;
#83082=CARTESIAN_POINT ( 'NONE',  ( 79.08035272007656147, 46.14455083862815599, -12.71395590097782602 ) ) ;
#83087=VERTEX_POINT ( 'NONE', #36760 ) ;
#83088=CARTESIAN_POINT ( 'NONE',  ( 18.13223351794271565, 28.65586893147756342, -7.433330006724137462 ) ) ;
#83089=CARTESIAN_POINT ( 'NONE',  ( 23.82048379914786906, 32.49103043416550207, -8.090169943749479842 ) ) ;
#83090=CARTESIAN_POINT ( 'NONE',  ( 71.93104225996606260, 70.29527910854686468, -7.202640768569800400 ) ) ;
#83091=CARTESIAN_POINT ( 'NONE',  ( 75.32522729562204233, 66.75955131866579961, -12.97495178021951290 ) ) ;
#83096=VERTEX_POINT ( 'NONE', #98090 ) ;
#83100=CARTESIAN_POINT ( 'NONE',  ( 65.83617023856123751, 68.96008090994861561, -2.256815018066093970 ) ) ;
#83102=LINE ( 'NONE', #4570, #43429 ) ;
#83114=CARTESIAN_POINT ( 'NONE',  ( 76.26946404230704957, 64.97317754398874001, 14.67006731301515998 ) ) ;
#83117=CARTESIAN_POINT ( 'NONE',  ( 87.83451486366641348, 43.48610523111371862, -0.3240457279886222453 ) ) ;
#83118=CARTESIAN_POINT ( 'NONE',  ( 81.32935958276657118, 56.15914934284622717, 16.09084449101850467 ) ) ;
#83124=CARTESIAN_POINT ( 'NONE',  ( 85.69563749947228359, 42.25122789774620458, -8.045052972278457832E-08 ) ) ;
#83128=CARTESIAN_POINT ( 'NONE',  ( 76.06231244383691603, 51.24788304498655833, -15.62831804942144842 ) ) ;
#83137=CARTESIAN_POINT ( 'NONE',  ( 85.15564232274995504, 43.25524388620375760, 4.736941226824257001 ) ) ;
#83139=CARTESIAN_POINT ( 'NONE',  ( 79.45319113830514368, 59.16108313430871135, -16.22659794754331131 ) ) ;
#83143=CARTESIAN_POINT ( 'NONE',  ( 77.15418484582102110, 58.25238759143534395, 16.13560698115002978 ) ) ;
#83146=CARTESIAN_POINT ( 'NONE',  ( 72.61844844480206973, 71.38675611224468298, -5.879003452896631288 ) ) ;
#83147=CARTESIAN_POINT ( 'NONE',  ( 80.40171677142443230, 49.09739724853191944, 14.02116035787424231 ) ) ;
#83155=EDGE_CURVE ( 'NONE', #22415, #67005, #8038, .T. ) ;
#83157=CARTESIAN_POINT ( 'NONE',  ( 21.47138989493050332, 31.13478043621388736, 8.090169943749478065 ) ) ;
#83160=CARTESIAN_POINT ( 'NONE',  ( 71.51226778736909750, 69.30015625669656743, -9.074508208858107494 ) ) ;
#83162=CARTESIAN_POINT ( 'NONE',  ( 72.25843749594145038, 71.93659321963055220, -3.779133617516833521 ) ) ;
#83165=ORIENTED_EDGE ( 'NONE', *, *, #18180, .T. ) ;
#83167=CARTESIAN_POINT ( 'NONE',  ( 66.47301154247004717, 67.89115917382773091, -6.669687514284739827 ) ) ;
#83172=CARTESIAN_POINT ( 'NONE',  ( 18.29780494541646974, 34.65659080271451842, -1.878358725466461243E-16 ) ) ;
#83175=CARTESIAN_POINT ( 'NONE',  ( 71.68807920414248258, 72.06984970416017688, -3.563505611461031286 ) ) ;
#83176=CARTESIAN_POINT ( 'NONE',  ( 81.74119788692269140, 59.14441083166271795, 0.000000000000000000 ) ) ;
#83190=CARTESIAN_POINT ( 'NONE',  ( 35.63920408047906818, 43.68290643055190969, 3.479690158560446702E-15 ) ) ;
#83193=CARTESIAN_POINT ( 'NONE',  ( 67.16990927169524639, 66.79708245693808522, -9.067759095298590921 ) ) ;
#83195=CARTESIAN_POINT ( 'NONE',  ( 18.76490627030545610, 13.76004757982088655, 5.678558825948272215 ) ) ;
#83196=CARTESIAN_POINT ( 'NONE',  ( 6.430760413625676186, 27.21091486745858390, -1.111400068045478839E-16 ) ) ;
#83197=CARTESIAN_POINT ( 'NONE',  ( 82.78422215508307147, 53.78621188977052725, 15.78456841880229433 ) ) ;
#83198=CARTESIAN_POINT ( 'NONE',  ( 71.39729339694994792, 59.37714758514961488, 15.21381503262609414 ) ) ;
#83203=CARTESIAN_POINT ( 'NONE',  ( 81.58052743141770691, 41.99578084072658157, 7.590836836702154145 ) ) ;
#83207=CARTESIAN_POINT ( 'NONE',  ( 26.39215011307057424, 23.43677371833802425, -10.00000000000000355 ) ) ;
#83216=FACE_OUTER_BOUND ( 'NONE', #12686, .T. ) ;
#83217=CARTESIAN_POINT ( 'NONE',  ( 80.65095556854913639, 57.57228308630149627, 16.58706730796347628 ) ) ;
#83218=CARTESIAN_POINT ( 'NONE',  ( 73.05863210132505969, 69.60576123971951290, -9.808587366596233537 ) ) ;
#83221=EDGE_CURVE ( 'NONE', #18761, #54490, #53215, .T. ) ;
#83224=CARTESIAN_POINT ( 'NONE',  ( 74.76978274660817192, 64.43581441273093446, 14.05910472376388398 ) ) ;
#83225=VERTEX_POINT ( 'NONE', #15193 ) ;
#83232=EDGE_LOOP ( 'NONE', ( #60363, #24852, #68871, #52783, #81504, #97656 ) ) ;
#83236=CARTESIAN_POINT ( 'NONE',  ( 82.47797010013799479, 53.85630837337446764, 15.85289899457425022 ) ) ;
#83237=CARTESIAN_POINT ( 'NONE',  ( 83.90596095485256001, 41.21795184261720379, -1.108148245180562033E-06 ) ) ;
#83243=CARTESIAN_POINT ( 'NONE',  ( 87.35668359673078953, 44.84080960044052233, -6.701380392922977158 ) ) ;
#83252=CARTESIAN_POINT ( 'NONE',  ( 79.75798450490407276, 52.95241734746561946, -15.59895281915799004 ) ) ;
#83253=CARTESIAN_POINT ( 'NONE',  ( 84.83954103072970554, 42.64226960066435623, 4.998593534305094899 ) ) ;
#83255=CARTESIAN_POINT ( 'NONE',  ( 79.70677143370977547, 46.01134058545614636, 12.98241517805147538 ) ) ;
#83259=FACE_OUTER_BOUND ( 'NONE', #8835, .T. ) ;
#83275=CARTESIAN_POINT ( 'NONE',  ( 74.23941942568015406, 67.87611062571697573, -11.69065606785908251 ) ) ;
#83280=CARTESIAN_POINT ( 'NONE',  ( 81.89040035157415787, 41.13959363232161337, -5.507854768277897328 ) ) ;
#83289=CARTESIAN_POINT ( 'NONE',  ( 79.16072033191956336, 59.43364827697804742, -16.53552069436850402 ) ) ;
#83290=AXIS2_PLACEMENT_3D ( 'NONE', #43930, #29252, #73858 ) ;
#83295=CARTESIAN_POINT ( 'NONE',  ( 9.265696904164599346, 17.30066082961419838, -10.00000000000000533 ) ) ;
#83297=CARTESIAN_POINT ( 'NONE',  ( 71.60869501579809082, 58.97949029833907986, -15.86055346694359436 ) ) ;
#83298=B_SPLINE_CURVE_WITH_KNOTS ( 'NONE', 3,
 ( #16782, #95354, #88251, #9713, #2101, #32981, #17802, #56274, #63886, #40066, #18799, #94822, #25386, #32496, #49681, #64390 ),
 .UNSPECIFIED., .F., .F.,
 ( 4, 1, 2, 2, 2, 1, 2, 2, 4 ),
 ( 0.000000000000000000, 0.1250000000000022760, 0.1875000000000034972, 0.2500000000000047184, 0.5000000000000039968, 0.6250000000000035527, 0.6875000000000034417, 0.7500000000000032196, 1.000000000000000000 ),
 .UNSPECIFIED. ) ;
#83301=EDGE_CURVE ( 'NONE', #57995, #26530, #68482, .T. ) ;
#83305=CARTESIAN_POINT ( 'NONE',  ( 72.83288601605435986, 57.14714021852967818, 15.89844244041831089 ) ) ;
#83307=CARTESIAN_POINT ( 'NONE',  ( 66.08643694688238668, 68.49314833729727070, -4.715610728220657855 ) ) ;
#83312=CARTESIAN_POINT ( 'NONE',  ( 30.20304716546516133, 19.29860640527293469, -2.839279412974138328 ) ) ;
#83314=CARTESIAN_POINT ( 'NONE',  ( 83.76909922093737748, 51.72725043056325234, -14.84865573977556075 ) ) ;
#83316=CARTESIAN_POINT ( 'NONE',  ( 88.44572534255364360, 43.94768732639446540, 1.766277459783989867 ) ) ;
#83318=CARTESIAN_POINT ( 'NONE',  ( 68.46226156283634623, 64.36458740167765313, 12.29825945318413005 ) ) ;
#83320=FACE_OUTER_BOUND ( 'NONE', #49060, .T. ) ;
#83324=CARTESIAN_POINT ( 'NONE',  ( 7.127696690345725727, 16.06628583063839244, -9.188101187500006262 ) ) ;
#83325=VERTEX_POINT ( 'NONE', #23911 ) ;
#83326=CARTESIAN_POINT ( 'NONE',  ( 72.23865006290039048, 71.95475215217994958, 3.607730569270007237 ) ) ;
#83328=CARTESIAN_POINT ( 'NONE',  ( 83.47336872178040323, 41.48982131955913388, -3.853860643902951022 ) ) ;
#83329=CARTESIAN_POINT ( 'NONE',  ( 71.67183227515569399, 72.09799021063221858, 0.6624418287695852392 ) ) ;
#83334=CARTESIAN_POINT ( 'NONE',  ( 72.91946395511783408, 57.64528416996791549, -16.31297782416237752 ) ) ;
#83336=CARTESIAN_POINT ( 'NONE',  ( 15.82880751958831667, 10.10801979619927415, 3.090169943749476733 ) ) ;
#83352=CARTESIAN_POINT ( 'NONE',  ( 73.17137018064387632, 69.60265530810194434, -9.888782888319330056 ) ) ;
#83353=CARTESIAN_POINT ( 'NONE',  ( 67.09339416431679126, 69.57934519908948801, 2.872329545031587994 ) ) ;
#83354=CARTESIAN_POINT ( 'NONE',  ( 81.42800912266413604, 42.13481243118283714, -7.961906169233770925 ) ) ;
#83361=CARTESIAN_POINT ( 'NONE',  ( 87.86298961015023679, 44.89260222163544256, 6.207647304897665919 ) ) ;
#83369=CARTESIAN_POINT ( 'NONE',  ( 82.85943510349244434, 53.46362409593341170, -15.31598598672309031 ) ) ;
#83371=EDGE_LOOP ( 'NONE', ( #35476, #64748, #92826, #66338 ) ) ;
#83372=DIRECTION ( 'NONE',  ( 0.8660254037844379305, 0.5000000000000014433, 0.000000000000000000 ) ) ;
#83373=CARTESIAN_POINT ( 'NONE',  ( 18.12859834787737157, 11.26216523072493736, -2.296566073217252530E-15 ) ) ;
#83381=ADVANCED_FACE ( 'NONE', ( #55298 ), #79167, .T. ) ;
#83382=CARTESIAN_POINT ( 'NONE',  ( 77.17818405207798094, 49.57096083066192449, -15.48190036198286101 ) ) ;
#83385=LINE ( 'NONE', #76739, #58046 ) ;
#83391=CARTESIAN_POINT ( 'NONE',  ( 82.47021907082941539, 53.30441442868470858, -15.33472904691311456 ) ) ;
#83394=CARTESIAN_POINT ( 'NONE',  ( 72.06470348997973474, 72.25603645428110156, 1.367373202405273602 ) ) ;
#83397=CARTESIAN_POINT ( 'NONE',  ( 76.20055470335280745, 65.09253202017347917, 14.18943646504599343 ) ) ;
#83407=CARTESIAN_POINT ( 'NONE',  ( 69.01996124760182738, 67.49486141842439224, 9.543146168910283222 ) ) ;
#83409=EDGE_CURVE ( 'NONE', #4740, #50075, #70947, .T. ) ;
#83413=CARTESIAN_POINT ( 'NONE',  ( 65.82138188502713660, 68.94138306836742913, 2.321386409612693047 ) ) ;
#83418=CARTESIAN_POINT ( 'NONE',  ( 81.37890540328889699, 53.11183844281263333, -15.40672322402467387 ) ) ;
#83424=CARTESIAN_POINT ( 'NONE',  ( 84.76921427251618013, 50.44646837537948159, 13.50760817970367533 ) ) ;
#83430=CARTESIAN_POINT ( 'NONE',  ( 81.87577037490221699, 41.13764054769151102, -5.524405591390634029 ) ) ;
#83432=CARTESIAN_POINT ( 'NONE',  ( 6.414422030351863313, 19.10171378149916421, 9.188101187500008038 ) ) ;
#83440=CARTESIAN_POINT ( 'NONE',  ( 37.97865540203802937, 30.43085787977766188, -9.188101187500008038 ) ) ;
#83442=DIRECTION ( 'NONE',  ( -0.8660254037844379305, -0.5000000000000014433, -0.000000000000000000 ) ) ;
#83444=CARTESIAN_POINT ( 'NONE',  ( 24.72364882272980324, 19.98920272979926693, 7.433330006724137462 ) ) ;
#83445=CARTESIAN_POINT ( 'NONE',  ( 14.97590445773717782, 13.81029122506293305, 8.090169943749479842 ) ) ;
#83450=CARTESIAN_POINT ( 'NONE',  ( 70.33238309585017589, 61.19012738999462897, 14.82922649093364598 ) ) ;
#83451=CARTESIAN_POINT ( 'NONE',  ( 75.92541454099094267, 65.74968322642241958, -14.18997729123868901 ) ) ;
#83457=LINE ( 'NONE', #82487, #37484 ) ;
#83460=CARTESIAN_POINT ( 'NONE',  ( 83.82679190265474745, 41.76113697558885463, 1.428417452354569850 ) ) ;
#83464=ORIENTED_EDGE ( 'NONE', *, *, #81668, .F. ) ;
#83472=CARTESIAN_POINT ( 'NONE',  ( 35.38177548881301249, 32.37878583063844218, 9.188101187500006262 ) ) ;
#83475=CARTESIAN_POINT ( 'NONE',  ( 87.63119364650854948, 45.29408460765224476, 6.394950601605615681 ) ) ;
#83480=PLANE ( 'NONE',  #91320 ) ;
#83481=CARTESIAN_POINT ( 'NONE',  ( 79.79337866746672603, 57.38101010784296108, 16.24820852827756923 ) ) ;
#83486=CARTESIAN_POINT ( 'NONE',  ( 75.86996176085413879, 60.47672722295040870, -15.68272062288790814 ) ) ;
#83489=CARTESIAN_POINT ( 'NONE',  ( 76.98305832116996328, 63.37377475765585899, -15.46912589935254623 ) ) ;
#83494=CARTESIAN_POINT ( 'NONE',  ( 27.74993340135631215, 36.99752408145592852, 5.678558825948277544 ) ) ;
#83499=CARTESIAN_POINT ( 'NONE',  ( 74.21864607481936105, 68.58553829006309854, -11.54532566021463502 ) ) ;
#83502=CARTESIAN_POINT ( 'NONE',  ( 67.33987171904671243, 68.55273472465368911, 6.369544805306559532 ) ) ;
#83504=CARTESIAN_POINT ( 'NONE',  ( 22.33482336197099016, 13.86426979415089455, -3.090169943749474069 ) ) ;
#83510=DIRECTION ( 'NONE',  ( -0.8660254037844377084, -0.5000000000000014433, -0.000000000000000000 ) ) ;
#83516=CARTESIAN_POINT ( 'NONE',  ( 67.08658855976769075, 68.82903281458501965, -3.711205762594173230 ) ) ;
#83518=CARTESIAN_POINT ( 'NONE',  ( 69.95954962829708279, 62.80909189523259073, -13.34258826528541952 ) ) ;
#83523=CARTESIAN_POINT ( 'NONE',  ( 82.02651322757263586, 41.09817291294280750, -3.386295274050155069 ) ) ;
#83527=CARTESIAN_POINT ( 'NONE',  ( 82.54609081338128362, 42.37776545139765716, 6.143319459098965041 ) ) ;
#83532=CARTESIAN_POINT ( 'NONE',  ( 71.45285423991207097, 70.68761458493762007, -5.807058293593552634 ) ) ;
#83541=CARTESIAN_POINT ( 'NONE',  ( 66.91132889924701033, 69.20890817986715149, 0.7224412942219599065 ) ) ;
#83542=CARTESIAN_POINT ( 'NONE',  ( 73.54295707248225256, 69.21941320345065662, -10.00962305751349035 ) ) ;
#83544=( NAMED_UNIT ( * ) SI_UNIT ( $, .STERADIAN. ) SOLID_ANGLE_UNIT ( ) );
#83548=VECTOR ( 'NONE', #57529, 1000.000000000000114 ) ;
#83549=CARTESIAN_POINT ( 'NONE',  ( 71.96027346690365789, 72.28811235517684963, 3.313491923126963279 ) ) ;
#83553=CARTESIAN_POINT ( 'NONE',  ( 80.32319512552398066, 50.51006391666574302, -14.68283735665326084 ) ) ;
#83554=CARTESIAN_POINT ( 'NONE',  ( 71.84099513407564075, 72.54812194311107021, -1.276242074083207001 ) ) ;
#83557=CARTESIAN_POINT ( 'NONE',  ( 18.31869600479030424, 33.68290643055186706, 3.479690158560446702E-15 ) ) ;
#83560=CARTESIAN_POINT ( 'NONE',  ( 36.03373902044236132, 43.73705186507757503, -3.090169943749475845 ) ) ;
#83566=CARTESIAN_POINT ( 'NONE',  ( 72.36041625537609434, 60.48984345533310858, 15.04059213219202640 ) ) ;
#83574=EDGE_LOOP ( 'NONE', ( #51385, #6949, #27371, #38001 ) ) ;
#83582=CARTESIAN_POINT ( 'NONE',  ( 79.38657480761875718, 46.22199533766026747, -13.24841598642484364 ) ) ;
#83583=CARTESIAN_POINT ( 'NONE',  ( 69.61542750552385428, 62.56132062511080250, -13.94275833699888345 ) ) ;
#83586=ORIENTED_EDGE ( 'NONE', *, *, #4642, .F. ) ;
#83587=CARTESIAN_POINT ( 'NONE',  ( 18.74326920199815305, 31.79752408145591858, -5.678558825948271327 ) ) ;
#83588=CARTESIAN_POINT ( 'NONE',  ( 75.26690622274593068, 56.07482427453010843, 16.14689877337623969 ) ) ;
#83589=CARTESIAN_POINT ( 'NONE',  ( 72.67905965592419193, 70.26320000030698054, -8.002569769838684621 ) ) ;
#83601=CARTESIAN_POINT ( 'NONE',  ( 81.40581815559377787, 55.82057330830384956, 16.38440887150438385 ) ) ;
#83603=B_SPLINE_CURVE_WITH_KNOTS ( 'NONE', 3,
 ( #98197, #51579, #59146, #66777, #22175, #27788, #74411, #59659, #60152, #21194, #75393, #68266, #43960, #21681, #51065, #4481, #5976, #52560, #29774, #36872, #82536, #35375, #75903, #67778, #98703, #29287, #42952, #60647, #6483, #4996, #91603, #66286, #97219, #58661, #89633, #20195, #12600, #97702, #43467, #28270, #69264, #92128, #22681, #61659, #7462, #24663 ),
 .UNSPECIFIED., .F., .F.,
 ( 4, 1, 2, 2, 1, 2, 2, 1, 1, 2, 2, 1, 1, 2, 2, 1, 1, 2, 2, 1, 1, 1, 2, 2, 1, 1, 1, 2, 2, 4 ),
 ( 0.000000000000000000, 0.06250000000000537070, 0.09375000000000875688, 0.1250000000000121292, 0.1875000000000191791, 0.2187500000000226763, 0.2500000000000262013, 0.3125000000000315303, 0.3437500000000344724, 0.3593750000000353051, 0.3750000000000361933, 0.4375000000000394684, 0.4687500000000424105, 0.4843750000000436318, 0.5000000000000448530, 0.5625000000000469624, 0.5937500000000474065, 0.6093750000000467404, 0.6250000000000460743, 0.6875000000000431877, 0.7187500000000411893, 0.7343750000000400791, 0.7421875000000380806, 0.7500000000000360822, 0.8125000000000286438, 0.8437500000000239808, 0.8593750000000223155, 0.8671875000000223155, 0.8750000000000223155, 1.000000000000000000 ),
 .UNSPECIFIED. ) ;
#83609=CARTESIAN_POINT ( 'NONE',  ( 79.67912095024387042, 45.93721481267125029, 12.94223426716299663 ) ) ;
#83616=CARTESIAN_POINT ( 'NONE',  ( 76.26477717271305323, 65.12336802401900115, 14.59904178568168120 ) ) ;
#83617=CARTESIAN_POINT ( 'NONE',  ( 66.97405472610564914, 68.05443638886698920, 6.913098729884842975 ) ) ;
#83620=B_SPLINE_SURFACE_WITH_KNOTS ( 'NONE', 3, 1, ( 
 ( #31015, #91871 ),
 ( #45219, #45706 ),
 ( #61413, #38613 ),
 ( #22426, #76158 ),
 ( #15301, #91361 ),
 ( #30021, #62402 ),
 ( #93358, #14819 ),
 ( #37121, #7216 ),
 ( #84273, #626 ),
 ( #68028, #61905 ),
 ( #68523, #30525 ),
 ( #54814, #92855 ),
 ( #29533, #99444 ),
 ( #31507, #85791 ),
 ( #46200, #69011 ),
 ( #22913, #7722 ),
 ( #76631, #16323 ),
 ( #69518, #53800 ),
 ( #60906, #38100 ),
 ( #77117, #6226 ),
 ( #46717, #132 ),
 ( #99942, #54299 ),
 ( #77645, #23409 ),
 ( #85267, #98950 ),
 ( #15813, #8230 ),
 ( #39098, #70011 ),
 ( #60405, #21925 ),
 ( #17319, #87800 ),
 ( #79673, #56311 ),
 ( #47216, #88285 ),
 ( #78138, #1132 ) ),
 .UNSPECIFIED., .F., .F., .F.,
 ( 4, 3, 3, 3, 3, 3, 3, 3, 3, 3, 4 ),
 ( 2, 2 ),
 ( 0.000000000000000000, 0.1333490885032316831, 0.3007194338854232707, 0.4699862290244899432, 0.5844252810809152932, 0.6686540514502595789, 0.7354980260655316071, 0.8028463152565562533, 0.8633854507756971719, 0.9437142632666813968, 1.000000000000000000 ),
 ( 0.000000000000000000, 1.000000000000000000 ),
 .UNSPECIFIED. ) ;
#83621=CARTESIAN_POINT ( 'NONE',  ( 81.22638650634890212, 56.17890105291410663, 16.10240317970520962 ) ) ;
#83625=CARTESIAN_POINT ( 'NONE',  ( 70.86180917824351866, 65.18287531716292449, 12.13021261807535822 ) ) ;
#83626=CARTESIAN_POINT ( 'NONE',  ( 87.36072329576109041, 44.92403384853251680, 6.858028155142561033 ) ) ;
#83629=CARTESIAN_POINT ( 'NONE',  ( 24.24684063885245422, 16.12755873383626337, -6.180339887498949025 ) ) ;
#83633=CARTESIAN_POINT ( 'NONE',  ( 76.04471674989768815, 51.35811929192740166, -16.14395075012120273 ) ) ;
#83644=CARTESIAN_POINT ( 'NONE',  ( 87.74187345177139719, 44.20045605528624577, 4.652363546664123994 ) ) ;
#83645=CARTESIAN_POINT ( 'NONE',  ( 73.36397865156375531, 67.21426321682912430, -12.28381576122694341 ) ) ;
#83646=CARTESIAN_POINT ( 'NONE',  ( 87.83899792242847582, 44.00541668311377208, -1.848955303085624058 ) ) ;
#83648=CARTESIAN_POINT ( 'NONE',  ( 72.85283338774588913, 70.95119525769652569, 7.785565881738510718 ) ) ;
#83649=CARTESIAN_POINT ( 'NONE',  ( 71.52047308030192596, 67.22020565769358313, -10.76659510055284841 ) ) ;
#83652=( BOUNDED_CURVE ( )  B_SPLINE_CURVE ( 2, ( #99675, #84014, #83504, #52551, #84991, #14067, #37350, #30259, #60143, #6957, #52065, #98693, #15044 ),
 .UNSPECIFIED., .F., .T. ) 
 B_SPLINE_CURVE_WITH_KNOTS ( ( 3, 2, 2, 2, 2, 2, 3 ),
 ( 0.2874999999999999778, 0.2899999999999999800, 0.2949999999999999845, 0.2999999999999999889, 0.3049999999999999933, 0.3099999999999999978, 0.3125000000000000000 ),
 .UNSPECIFIED. ) 
 CURVE ( )  GEOMETRIC_REPRESENTATION_ITEM ( )  RATIONAL_B_SPLINE_CURVE ( ( 0.9755282581475768211, 0.9755282581475768211, 1.000000000000000000, 0.9510565162951535312, 1.000000000000000000, 0.9510565162951535312, 1.000000000000000000, 0.9510565162951535312, 1.000000000000000000, 0.9510565162951535312, 1.000000000000000000, 0.9755282581475768211, 0.9755282581475768211 ) ) 
 REPRESENTATION_ITEM ( '' )  );
#83654=CARTESIAN_POINT ( 'NONE',  ( 86.54822389131679472, 42.74345947012793090, -2.172736160200603931E-06 ) ) ;
#83655=CARTESIAN_POINT ( 'NONE',  ( 80.64045924028067702, 49.96054635152264467, 14.37335726122271318 ) ) ;
#83663=CARTESIAN_POINT ( 'NONE',  ( 24.23155096423127475, 19.15404122711133894, 8.090169943749479842 ) ) ;
#83664=LINE ( 'NONE', #52704, #96949 ) ;
#83666=CARTESIAN_POINT ( 'NONE',  ( 18.00728827979274627, 29.13478043621388380, 8.090169943749478065 ) ) ;
#83668=CARTESIAN_POINT ( 'NONE',  ( 72.19186707540899306, 71.87388231314805864, -3.875259471157315172 ) ) ;
#83672=CARTESIAN_POINT ( 'NONE',  ( 66.98956810429928055, 67.69424080958161483, -6.459028911160978659 ) ) ;
#83673=CARTESIAN_POINT ( 'NONE',  ( 72.76037481019557163, 70.79492043649186428, -7.951079947203121279 ) ) ;
#83679=CARTESIAN_POINT ( 'NONE',  ( 25.04820903906726315, 30.16454794089042224, -10.00000000000000355 ) ) ;
#83680=CARTESIAN_POINT ( 'NONE',  ( 85.54106661513783649, 48.65811287445264810, 12.45824154186499833 ) ) ;
#83682=CARTESIAN_POINT ( 'NONE',  ( 72.10970998683657740, 71.81466167570245318, -3.920937378582701083 ) ) ;
#83694=CARTESIAN_POINT ( 'NONE',  ( 78.88646228610093658, 60.09280412644832836, 16.11190982779557146 ) ) ;
#83701=CARTESIAN_POINT ( 'NONE',  ( 12.93608109523609073, 25.65586893147755276, -7.433330006724137462 ) ) ;
#83703=CARTESIAN_POINT ( 'NONE',  ( 71.94031269653281413, 59.11929964053626918, 15.87436981764813559 ) ) ;
#83707=CARTESIAN_POINT ( 'NONE',  ( 86.56379725475841269, 45.50107930069437856, -7.807079406273517819 ) ) ;
#83709=CARTESIAN_POINT ( 'NONE',  ( 75.35001427908503047, 53.53583770442167378, -16.04486494172472888 ) ) ;
#83710=CARTESIAN_POINT ( 'NONE',  ( 81.61450380106850844, 42.00667554686729233, 7.576096789987255775 ) ) ;
#83714=CARTESIAN_POINT ( 'NONE',  ( 77.22942826013965600, 63.41635481091116588, 15.12246632917587519 ) ) ;
#83717=ORIENTED_EDGE ( 'NONE', *, *, #17831, .T. ) ;
#83723=CARTESIAN_POINT ( 'NONE',  ( 70.20579083185378977, 65.41824112225215515, 12.26219425119750639 ) ) ;
#83724=CARTESIAN_POINT ( 'NONE',  ( 80.12177396824181130, 57.42895151072963955, -16.59339316893575145 ) ) ;
#83726=ORIENTED_EDGE ( 'NONE', *, *, #74556, .F. ) ;
#83730=CARTESIAN_POINT ( 'NONE',  ( 74.55249937888110878, 63.44298656893680999, 14.44720752827713284 ) ) ;
#83732=EDGE_CURVE ( 'NONE', #44175, #2508, #69663, .T. ) ;
#83739=CARTESIAN_POINT ( 'NONE',  ( 79.48876273271771709, 46.38894273206648222, -12.71961528548989406 ) ) ;
#83753=CARTESIAN_POINT ( 'NONE',  ( 71.23563381243731385, 70.03978810160823798, 6.894242474657360731 ) ) ;
#83755=CARTESIAN_POINT ( 'NONE',  ( 66.97555164495814495, 67.03582895754806259, 8.583456203666562701 ) ) ;
#83757=CARTESIAN_POINT ( 'NONE',  ( 78.33682591320163624, 47.43237704492500484, 14.30218028890826076 ) ) ;
#83761=CARTESIAN_POINT ( 'NONE',  ( 72.24611734329810986, 70.10459536098181843, 7.832089211065604850 ) ) ;
#83763=CARTESIAN_POINT ( 'NONE',  ( 79.49710624387913072, 46.36387489428066999, 12.69932268971443357 ) ) ;
#83765=CARTESIAN_POINT ( 'NONE',  ( 83.53204454370724363, 52.39401912150449903, -15.17729711222451883 ) ) ;
#83767=ORIENTED_EDGE ( 'NONE', *, *, #35077, .T. ) ;
#83771=FACE_OUTER_BOUND ( 'NONE', #35830, .T. ) ;
#83784=CARTESIAN_POINT ( 'NONE',  ( 73.32799597867342811, 60.88228677579900960, 15.59493297680661250 ) ) ;
#83786=CARTESIAN_POINT ( 'NONE',  ( 81.65911681526914379, 41.55393351364236310, -5.423798156015772420 ) ) ;
#83796=ADVANCED_FACE ( 'NONE', ( #85141 ), #46581, .T. ) ;
#83798=CARTESIAN_POINT ( 'NONE',  ( 15.82204613103260904, 8.944730856513908535, 1.475505719884397138E-15 ) ) ;
#83800=CARTESIAN_POINT ( 'NONE',  ( 71.93836645383190387, 59.32121692304542648, -15.31782635615035026 ) ) ;
#83801=CYLINDRICAL_SURFACE ( 'NONE', #2220, 16.60714546451156792 ) ;
#83806=CARTESIAN_POINT ( 'NONE',  ( 72.75281560095611155, 57.10416661572288177, 16.38170419688453805 ) ) ;
#83808=CARTESIAN_POINT ( 'NONE',  ( 66.38349642218635438, 68.19267280352575256, -4.414189003008335277 ) ) ;
#83813=CARTESIAN_POINT ( 'NONE',  ( 20.70865909420142259, 30.14336893147755703, 7.433330006724141015 ) ) ;
#83817=CARTESIAN_POINT ( 'NONE',  ( 75.27993480048328934, 53.55678813946182260, -16.04991370599387679 ) ) ;
#83818=CARTESIAN_POINT ( 'NONE',  ( 88.26049611827410502, 43.94792280741878443, 2.484900765466354855 ) ) ;
#83820=CARTESIAN_POINT ( 'NONE',  ( 68.50372518212984119, 64.31961559923436766, 12.35208758802623130 ) ) ;
#83822=PLANE ( 'NONE',  #50373 ) ;
#83841=CARTESIAN_POINT ( 'NONE',  ( 14.86318692873816083, 16.78052372038639106, -10.00000000000000355 ) ) ;
#83842=CARTESIAN_POINT ( 'NONE',  ( 82.71715233927223210, 44.61979091911242534, 10.25119714958372796 ) ) ;
#83849=CARTESIAN_POINT ( 'NONE',  ( 79.19548930461118630, 59.90515312544784621, -16.13566294680261848 ) ) ;
#83850=AXIS2_PLACEMENT_3D ( 'NONE', #47047, #954, #22755 ) ;
#83852=CARTESIAN_POINT ( 'NONE',  ( 69.82384421004434216, 62.57021116271138794, 13.43531312277882250 ) ) ;
#83858=CARTESIAN_POINT ( 'NONE',  ( 81.39901424530387430, 42.08420399104508647, -7.907947396089951120 ) ) ;
#83859=B_SPLINE_SURFACE_WITH_KNOTS ( 'NONE', 3, 1, ( 
 ( #15763, #78595 ),
 ( #40054, #46669 ),
 ( #23865, #39051 ),
 ( #578, #31462 ),
 ( #62353, #54757 ),
 ( #85743, #33481 ),
 ( #96314, #81127 ),
 ( #17790, #88737 ),
 ( #34001, #25373 ),
 ( #10188, #64886 ),
 ( #86736, #24870 ),
 ( #17272, #79119 ),
 ( #73003, #40560 ),
 ( #50174, #55744 ),
 ( #9700, #87752 ),
 ( #72507, #2595 ),
 ( #48690, #94316 ),
 ( #71990, #48175 ),
 ( #87257, #63377 ),
 ( #49669, #80123 ),
 ( #88238, #71496 ),
 ( #56264, #95832 ),
 ( #57761, #95341 ),
 ( #63874, #1598 ),
 ( #42071, #3115 ),
 ( #42553, #11694 ),
 ( #18789, #49187 ),
 ( #26385, #64379 ),
 ( #94811, #79625 ),
 ( #56770, #10685 ),
 ( #41054, #2089 ) ),
 .UNSPECIFIED., .F., .F., .F.,
 ( 4, 3, 3, 3, 3, 3, 3, 3, 3, 3, 4 ),
 ( 2, 2 ),
 ( 0.000000000000000000, 0.1122669598086822457, 0.2243161639709664035, 0.3396355846219253349, 0.4553962076585191809, 0.5677860799922548329, 0.6749047109689760848, 0.7773884377078600361, 0.8775581155834486502, 0.9782364162378277550, 1.000000000000000000 ),
 ( 0.000000000000000000, 1.000000000000000000 ),
 .UNSPECIFIED. ) ;
#83862=ORIENTED_EDGE ( 'NONE', *, *, #77991, .T. ) ;
#83864=CARTESIAN_POINT ( 'NONE',  ( 80.96741822347986783, 48.36393785198333717, 13.47256384055967615 ) ) ;
#83866=CARTESIAN_POINT ( 'NONE',  ( 70.61809369003644576, 71.23760416348828528, 2.495634273706798023 ) ) ;
#83874=CARTESIAN_POINT ( 'NONE',  ( 82.84778848911861360, 53.43038316853105840, -15.30831281788561604 ) ) ;
#83876=ORIENTED_EDGE ( 'NONE', *, *, #84448, .F. ) ;
#83877=CARTESIAN_POINT ( 'NONE',  ( 66.33533107015807673, 68.87447202099198762, 0.1160252125227696635 ) ) ;
#83878=CARTESIAN_POINT ( 'NONE',  ( 11.06573324809563807, 29.49540643055186351, 3.479690158560446702E-15 ) ) ;
#83880=CARTESIAN_POINT ( 'NONE',  ( 80.50883317518791671, 57.72730120993126235, 16.59589928958306615 ) ) ;
#83882=VERTEX_POINT ( 'NONE', #57183 ) ;
#83896=CARTESIAN_POINT ( 'NONE',  ( 82.86724755478759619, 53.49721348986128788, -15.32433688253754589 ) ) ;
#83899=CARTESIAN_POINT ( 'NONE',  ( 87.10342204727412252, 44.68451332791826758, -5.678729796000945740 ) ) ;
#83901=CARTESIAN_POINT ( 'NONE',  ( 72.49654942766741783, 70.83148394934322312, 7.643478247317291974 ) ) ;
#83910=CARTESIAN_POINT ( 'NONE',  ( 86.19494322620172966, 45.94452022226197130, -8.806296680070143879 ) ) ;
#83911=CARTESIAN_POINT ( 'NONE',  ( 86.50609478078892778, 43.48068990056189165, 2.985191827711138224 ) ) ;
#83920=CARTESIAN_POINT ( 'NONE',  ( 78.45979614097025490, 53.37690925373113515, 15.81233777137573071 ) ) ;
#83923=CARTESIAN_POINT ( 'NONE',  ( 82.47813483566071113, 52.69574577809284932, -15.09840053849920949 ) ) ;
#83929=CARTESIAN_POINT ( 'NONE',  ( 70.78897776588866009, 71.07630443005777465, 3.566669968915905820 ) ) ;
#83935=CARTESIAN_POINT ( 'NONE',  ( 10.86724236217879458, 11.98920272979924206, 7.433330006724137462 ) ) ;
#83936=CARTESIAN_POINT ( 'NONE',  ( 67.63114784964875525, 65.81005049607071555, 10.54782815381023831 ) ) ;
#83937=EDGE_CURVE ( 'NONE', #34846, #54109, #93744, .T. ) ;
#83939=CARTESIAN_POINT ( 'NONE',  ( 11.07908504951724282, 25.13478043621386959, 8.090169943749478065 ) ) ;
#83940=CARTESIAN_POINT ( 'NONE',  ( 85.53182313537475068, 42.77618286031957950, -1.864121902114932672 ) ) ;
#83945=CARTESIAN_POINT ( 'NONE',  ( 37.59133656659162881, 37.10171378149920685, 9.188101187500008038 ) ) ;
#83947=PLANE ( 'NONE',  #73369 ) ;
#83949=CARTESIAN_POINT ( 'NONE',  ( 29.91980124543643171, 22.98920272979927759, 7.433330006724137462 ) ) ;
#83950=CARTESIAN_POINT ( 'NONE',  ( 76.44525015969811932, 62.79367595106220534, -15.57143870397577778 ) ) ;
#83955=CARTESIAN_POINT ( 'NONE',  ( 70.39483845591227862, 61.02404926470979518, 14.91624238583182915 ) ) ;
#83963=CARTESIAN_POINT ( 'NONE',  ( 73.63650596374165502, 69.59800771093053129, 10.20034856658873323 ) ) ;
#83964=VECTOR ( 'NONE', #25034, 1000.000000000000114 ) ;
#83966=CARTESIAN_POINT ( 'NONE',  ( 78.26458253827964029, 61.66843869688886315, 16.13698506349214057 ) ) ;
#83968=EDGE_LOOP ( 'NONE', ( #66720, #85861, #86602, #43671, #94050, #65214 ) ) ;
#83972=CARTESIAN_POINT ( 'NONE',  ( 84.90983652888880329, 50.15852115595398431, 13.71398460619150406 ) ) ;
#83978=CARTESIAN_POINT ( 'NONE',  ( 42.00264329202813229, 26.11110640527295601, -2.839279412974138328 ) ) ;
#83980=CARTESIAN_POINT ( 'NONE',  ( 74.10991545788023416, 62.87482685241162272, -15.05254551912109306 ) ) ;
#83981=CARTESIAN_POINT ( 'NONE',  ( 87.34834566700719449, 45.48627435691049214, 7.110058762634436924 ) ) ;
#83982=ORIENTED_EDGE ( 'NONE', *, *, #78743, .F. ) ;
#83993=CARTESIAN_POINT ( 'NONE',  ( 82.34540653027241319, 40.38296044905965232, 1.376546748157425171 ) ) ;
#83999=EDGE_CURVE ( 'NONE', #34456, #70878, #64808, .T. ) ;
#84003=CARTESIAN_POINT ( 'NONE',  ( 45.46674490716588224, 28.11110640527296312, -2.839279412974138328 ) ) ;
#84008=CARTESIAN_POINT ( 'NONE',  ( 74.18809600170575891, 68.48282398988669684, -11.62097119590897520 ) ) ;
#84011=CARTESIAN_POINT ( 'NONE',  ( 73.43762515466688967, 73.52662068827324049, 2.033788753608857291E-15 ) ) ;
#84013=CARTESIAN_POINT ( 'NONE',  ( 25.43893178701101832, 38.18528772668521754, -1.583844403245329602 ) ) ;
#84014=CARTESIAN_POINT ( 'NONE',  ( 22.53732574998906557, 13.41603393254324850, -1.583844403245362020 ) ) ;
#84015=ORIENTED_EDGE ( 'NONE', *, *, #86491, .F. ) ;
#84020=FACE_OUTER_BOUND ( 'NONE', #13080, .T. ) ;
#84025=CARTESIAN_POINT ( 'NONE',  ( 82.30224259357629535, 41.51585266698759824, -5.837696018585297963 ) ) ;
#84029=CARTESIAN_POINT ( 'NONE',  ( 71.84536423521903714, 63.91743456037271898, 13.36489245195331144 ) ) ;
#84033=CARTESIAN_POINT ( 'NONE',  ( 71.70420417316881867, 72.14386137618673445, 3.298165275896878246 ) ) ;
#84034=CARTESIAN_POINT ( 'NONE',  ( 84.77469373108432649, 46.07232203156790717, 9.879153252899332216 ) ) ;
#84038=CARTESIAN_POINT ( 'NONE',  ( 82.49266829201729934, 54.25868459827957935, -15.95543171357395273 ) ) ;
#84044=EDGE_CURVE ( 'NONE', #35356, #826, #47956, .T. ) ;
#84046=AXIS2_PLACEMENT_3D ( 'NONE', #10356, #98948, #36616 ) ;
#84049=CARTESIAN_POINT ( 'NONE',  ( 73.71089132031853808, 69.41623407880213392, -9.892556164724735979 ) ) ;
#84052=CARTESIAN_POINT ( 'NONE',  ( 42.95298936059631245, 26.92755873383629250, 6.180339887498953466 ) ) ;
#84054=CARTESIAN_POINT ( 'NONE',  ( 82.74911235343154203, 53.93399432278085470, 15.46284286724625368 ) ) ;
#84056=CARTESIAN_POINT ( 'NONE',  ( 71.70420417316881867, 72.14386137618673445, 3.298165275896887128 ) ) ;
#84064=CARTESIAN_POINT ( 'NONE',  ( 78.75692787745495593, 50.96207330215147380, -15.15038416266403587 ) ) ;
#84067=AXIS2_PLACEMENT_3D ( 'NONE', #56856, #71591, #26481 ) ;
#84068=CARTESIAN_POINT ( 'NONE',  ( 19.41443888993109823, 32.18502408145592142, 5.678558825948276656 ) ) ;
#84071=CARTESIAN_POINT ( 'NONE',  ( 9.185703322462060783, 20.70171378149917629, -9.188101187500004485 ) ) ;
#84072=CARTESIAN_POINT ( 'NONE',  ( 26.07871176553302917, 38.55466486950701466, 7.012934429366973338E-14 ) ) ;
#84073=CARTESIAN_POINT ( 'NONE',  ( 77.22649460905380181, 63.31555197798695644, 15.15381191669831651 ) ) ;
#84090=CARTESIAN_POINT ( 'NONE',  ( 77.38344707992528981, 49.10671604805792612, -15.27628165681131200 ) ) ;
#84093=DIRECTION ( 'NONE',  ( -0.4493970231495795775, 0.7783784768652820540, -0.4383711467890876734 ) ) ;
#84095=CARTESIAN_POINT ( 'NONE',  ( 72.71583986753169881, 70.26028652805152319, -8.041570622059433404 ) ) ;
#84099=CARTESIAN_POINT ( 'NONE',  ( 21.45440292344354916, 18.10170272979926764, -7.433330006724141015 ) ) ;
#84100=CARTESIAN_POINT ( 'NONE',  ( 70.34088726048339879, 70.18557938879432356, -5.457944947125428214 ) ) ;
#84105=B_SPLINE_CURVE_WITH_KNOTS ( 'NONE', 3,
 ( #49341, #42220, #74151, #3262, #88400, #73157, #34627, #34145, #96476, #35122 ),
 .UNSPECIFIED., .F., .F.,
 ( 4, 2, 2, 2, 4 ),
 ( 0.000000000000000000, 0.0002622400424273028919, 0.0005244800848546057838, 0.0007867201272819086214, 0.001048960169709211568 ),
 .UNSPECIFIED. ) ;
#84110=CARTESIAN_POINT ( 'NONE',  ( 70.58432976086416488, 62.10851096095700541, 14.48710700881215985 ) ) ;
#84111=CARTESIAN_POINT ( 'NONE',  ( 68.32631950292746126, 65.68986423853067436, -10.34564397505435096 ) ) ;
#84125=AXIS2_PLACEMENT_3D ( 'NONE', #33569, #42637, #48261 ) ;
#84127=VERTEX_POINT ( 'NONE', #35138 ) ;
#84128=EDGE_LOOP ( 'NONE', ( #50694, #56521, #57393, #36983 ) ) ;
#84130=CARTESIAN_POINT ( 'NONE',  ( 66.90211989194618525, 67.97973764059037194, 6.975494484356386415 ) ) ;
#84131=EDGE_CURVE ( 'NONE', #22055, #73884, #8761, .T. ) ;
#84133=CARTESIAN_POINT ( 'NONE',  ( 84.06866697891398132, 42.24462045465304527, -5.118976631247559972 ) ) ;
#84134=CARTESIAN_POINT ( 'NONE',  ( 67.76349224122205328, 65.58094410182457068, 10.12335088330697630 ) ) ;
#84136=CARTESIAN_POINT ( 'NONE',  ( 72.65612776400872974, 69.70796105700785006, 8.715673431363931911 ) ) ;
#84142=CARTESIAN_POINT ( 'NONE',  ( 76.21282038944568171, 51.57770476861935549, -15.67853476563008819 ) ) ;
#84145=VECTOR ( 'NONE', #55570, 1000.000000000000000 ) ;
#84150=CARTESIAN_POINT ( 'NONE',  ( 88.22000632671873177, 44.27423112938744509, 4.003506518527982116 ) ) ;
#84154=CARTESIAN_POINT ( 'NONE',  ( 79.21773931386873357, 59.07529007650229147, -16.22247798074718617 ) ) ;
#84155=CARTESIAN_POINT ( 'NONE',  ( 70.07046733978542363, 67.38152690267425271, -9.666843875404030229 ) ) ;
#84159=CARTESIAN_POINT ( 'NONE',  ( 87.08779078562172060, 43.05500592647786107, 0.7967578903178703653 ) ) ;
#84160=CARTESIAN_POINT ( 'NONE',  ( 80.71714504946366731, 50.25349500424252369, 14.48686000064734358 ) ) ;
#84163=ORIENTED_EDGE ( 'NONE', *, *, #17547, .F. ) ;
#84169=CARTESIAN_POINT ( 'NONE',  ( 21.11941962201201051, 24.14441083166261137, 10.00000000000000533 ) ) ;
#84172=CARTESIAN_POINT ( 'NONE',  ( 19.40821860046903069, 26.90829794293880539, 10.00000000000000355 ) ) ;
#84178=CARTESIAN_POINT ( 'NONE',  ( 66.78940807508750765, 67.55366617704474663, -6.509619371764820528 ) ) ;
#84179=CARTESIAN_POINT ( 'NONE',  ( 72.69528318058601712, 70.26191488565096677, -8.019772805389131065 ) ) ;
#84183=CARTESIAN_POINT ( 'NONE',  ( 21.76190656055422323, 36.65659080271452552, -1.878358725466461243E-16 ) ) ;
#84184=CARTESIAN_POINT ( 'NONE',  ( 82.86315813168180000, 41.72223458103137261, -3.985406787420944674 ) ) ;
#84186=CARTESIAN_POINT ( 'NONE',  ( 71.65684213956077997, 72.06054752937143348, -3.528960205221522095 ) ) ;
#84187=DIRECTION ( 'NONE',  ( -0.5000000000000013323, 0.8660254037844378194, 0.000000000000000000 ) ) ;
#84198=CARTESIAN_POINT ( 'NONE',  ( 70.94848769240661568, 70.27665202542853251, -7.050353750945653530 ) ) ;
#84200=CARTESIAN_POINT ( 'NONE',  ( 27.96887745124769253, 39.08080186712594895, -3.090169943749475845 ) ) ;
#84201=CARTESIAN_POINT ( 'NONE',  ( 37.50955192761952617, 39.84336893147759184, -7.433330006724137462 ) ) ;
#84204=CARTESIAN_POINT ( 'NONE',  ( 81.79317580962712952, 59.05438242866674159, 0.4890738003669033995 ) ) ;
#84207=CARTESIAN_POINT ( 'NONE',  ( 22.66683848874176022, 18.80170272979926693, 7.433330006724137462 ) ) ;
#84208=CARTESIAN_POINT ( 'NONE',  ( 12.53574365251956912, 15.43677371833799938, -10.00000000000000355 ) ) ;
#84209=CARTESIAN_POINT ( 'NONE',  ( 71.52294418693975331, 59.11029950019791812, 15.81128158456864341 ) ) ;
#84212=CARTESIAN_POINT ( 'NONE',  ( 87.53583079710631409, 45.45925790797146249, -6.823327534849023657 ) ) ;
#84213=CARTESIAN_POINT ( 'NONE',  ( 82.57543265243437247, 45.76368055541952629, -11.49294040874591438 ) ) ;
#84214=CARTESIAN_POINT ( 'NONE',  ( 81.21214610088644292, 42.40786911149225347, 7.597942034095414243 ) ) ;
#84215=CARTESIAN_POINT ( 'NONE',  ( 80.74781574657598071, 57.21644485803223290, 16.56566952311892749 ) ) ;
#84218=CARTESIAN_POINT ( 'NONE',  ( 70.55924477032505138, 71.08919147220014167, -2.935579350952730593 ) ) ;
#84219=CARTESIAN_POINT ( 'NONE',  ( 77.07146940206541785, 63.73911480020577613, 14.98531907972277644 ) ) ;
#84222=ORIENTED_EDGE ( 'NONE', *, *, #67059, .T. ) ;
#84228=FACE_OUTER_BOUND ( 'NONE', #55509, .T. ) ;
#84229=CARTESIAN_POINT ( 'NONE',  ( 80.25249281668115486, 57.81819139295711807, 16.60223264289303557 ) ) ;
#84239=ORIENTED_EDGE ( 'NONE', *, *, #86010, .T. ) ;
#84242=CARTESIAN_POINT ( 'NONE',  ( 78.43441866794225348, 47.91884018220574148, -14.51553613075758342 ) ) ;
#84244=ORIENTED_EDGE ( 'NONE', *, *, #91412, .F. ) ;
#84247=CARTESIAN_POINT ( 'NONE',  ( 73.29569962742016287, 69.82617127822150849, 9.116539184905871451 ) ) ;
#84249=CARTESIAN_POINT ( 'NONE',  ( 82.29966782571446515, 53.62663270485408873, 15.81823675489985348 ) ) ;
#84255=EDGE_CURVE ( 'NONE', #8972, #66666, #41231, .T. ) ;
#84256=CARTESIAN_POINT ( 'NONE',  ( 71.55865654871253412, 70.58727594908697256, 6.225150381871440430 ) ) ;
#84257=CARTESIAN_POINT ( 'NONE',  ( 79.83401254395657531, 57.87045807247318407, 16.26439772172797404 ) ) ;
#84258=CARTESIAN_POINT ( 'NONE',  ( 67.16256804578090112, 66.80979783321159005, 8.146902435796073760 ) ) ;
#84260=CARTESIAN_POINT ( 'NONE',  ( 78.00127999931594047, 47.84930604673201060, 14.05929021715905414 ) ) ;
#84261=VERTEX_POINT ( 'NONE', #18465 ) ;
#84263=CARTESIAN_POINT ( 'NONE',  ( 71.60104883639283457, 68.65505837569367031, 9.270974577602569155 ) ) ;
#84265=CARTESIAN_POINT ( 'NONE',  ( 79.50366146091808162, 45.80427587621628760, 12.91999808083510004 ) ) ;
#84273=CARTESIAN_POINT ( 'NONE',  ( 72.44040225518423881, 71.75621485965102408, 5.770394931239954950 ) ) ;
#84282=CARTESIAN_POINT ( 'NONE',  ( 82.21410988452117863, 40.73976263626466476, 3.762362152834606732 ) ) ;
#84290=LINE ( 'NONE', #14836, #68911 ) ;
#84291=CARTESIAN_POINT ( 'NONE',  ( 68.47880282939688357, 64.40332810061045166, -12.27537564787820479 ) ) ;
#84299=CARTESIAN_POINT ( 'NONE',  ( 11.51180284259942610, 11.81029122506292595, 8.090169943749479842 ) ) ;
#84306=CARTESIAN_POINT ( 'NONE',  ( 72.64662832737921860, 57.19814123590507648, 15.87563656662714351 ) ) ;
#84308=CARTESIAN_POINT ( 'NONE',  ( 66.33628465374795269, 68.06039941485154543, -4.733060476579643350 ) ) ;
#84314=CARTESIAN_POINT ( 'NONE',  ( 32.24243340009443415, 30.56628583063843152, 9.188101187500006262 ) ) ;
#84317=LINE ( 'NONE', #67071, #16049 ) ;
#84319=CARTESIAN_POINT ( 'NONE',  ( 88.48118267945454818, 44.00993189541001982, 2.076335272536713905 ) ) ;
#84321=CARTESIAN_POINT ( 'NONE',  ( 68.93235832526967499, 64.11431000937152191, 12.06237109868430579 ) ) ;
#84327=CARTESIAN_POINT ( 'NONE',  ( 12.88253908977640094, 9.298606405272902720, -2.839279412974138328 ) ) ;
#84334=CARTESIAN_POINT ( 'NONE',  ( 66.66342508697567837, 67.67433879810248243, 6.129251300726011209 ) ) ;
#84339=DIRECTION ( 'NONE',  ( -0.7467472232290864875, 0.000000000000000000, -0.6651079495838618794 ) ) ;
#84346=CARTESIAN_POINT ( 'NONE',  ( 79.22574914704956939, 60.04803162267381111, -16.48148452078547521 ) ) ;
#84348=CARTESIAN_POINT ( 'NONE',  ( 70.00411547750407237, 62.73190158012358353, 13.40270835498630575 ) ) ;
#84353=ORIENTED_EDGE ( 'NONE', *, *, #61885, .T. ) ;
#84362=CARTESIAN_POINT ( 'NONE',  ( 82.41087058299665102, 41.30607584110375541, 3.329617797228953346 ) ) ;
#84368=CARTESIAN_POINT ( 'NONE',  ( 17.75393198606386136, 12.11110640527291160, -2.839279412974138328 ) ) ;
#84369=EDGE_CURVE ( 'NONE', #91598, #38047, #82053, .T. ) ;
#84373=ORIENTED_EDGE ( 'NONE', *, *, #15747, .T. ) ;
#84377=CARTESIAN_POINT ( 'NONE',  ( 82.66171877364854481, 45.89212660847477565, -10.89646859988845407 ) ) ;
#84382=CARTESIAN_POINT ( 'NONE',  ( 75.06185269395858484, 67.24559711482956459, -12.98328508234620848 ) ) ;
#84389=CARTESIAN_POINT ( 'NONE',  ( 72.07832455930082460, 72.32227812425290381, 0.7968372639566179139 ) ) ;
#84390=CARTESIAN_POINT ( 'NONE',  ( 72.65255621578388912, 70.92891038547531934, 7.631180297043450800 ) ) ;
#84393=LINE ( 'NONE', #84890, #20415 ) ;
#84394=ORIENTED_EDGE ( 'NONE', *, *, #49010, .T. ) ;
#84396=DIRECTION ( 'NONE',  ( -0.5000000000000082157, 0.8660254037844338226, 0.000000000000000000 ) ) ;
#84398=EDGE_CURVE ( 'NONE', #75472, #1759, #60411, .T. ) ;
#84400=CARTESIAN_POINT ( 'NONE',  ( 86.83833563368834518, 43.79545931766734412, 3.564591285478730054 ) ) ;
#84403=CARTESIAN_POINT ( 'NONE',  ( 69.10006990169640062, 67.64574319074527864, 9.412775915974314955 ) ) ;
#84408=CARTESIAN_POINT ( 'NONE',  ( 83.51092623577891061, 51.50185674319120466, -14.43088262691036583 ) ) ;
#84410=LINE ( 'NONE', #59562, #24284 ) ;
#84412=CARTESIAN_POINT ( 'NONE',  ( 80.64963530044916240, 57.33823058590956379, -16.23392529860869260 ) ) ;
#84416=CARTESIAN_POINT ( 'NONE',  ( 70.81256171061001226, 61.11968107447890475, -14.44615878937885967 ) ) ;
#84430=CARTESIAN_POINT ( 'NONE',  ( 19.81074232005190794, 13.29860640527291693, -2.839279412974138328 ) ) ;
#84431=CARTESIAN_POINT ( 'NONE',  ( 76.02121808213912857, 59.89693054018422913, -16.23481010780869838 ) ) ;
#84439=CARTESIAN_POINT ( 'NONE',  ( 36.89851624356406745, 36.70171378149922248, -9.188101187500004485 ) ) ;
#84440=CARTESIAN_POINT ( 'NONE',  ( 33.92686603480522223, 41.36126292948897998, 6.180339887498949913 ) ) ;
#84441=FACE_BOUND ( 'NONE', #6308, .T. ) ;
#84443=CARTESIAN_POINT ( 'NONE',  ( 29.64435718874111458, 29.06628583063843152, -9.188101187500006262 ) ) ;
#84448=EDGE_CURVE ( 'NONE', #56753, #11364, #46966, .T. ) ;
#84451=CARTESIAN_POINT ( 'NONE',  ( 84.51862751403463392, 49.89385305662934655, -13.69084041065644897 ) ) ;
#84455=FACE_OUTER_BOUND ( 'NONE', #84574, .T. ) ;
#84458=B_SPLINE_CURVE_WITH_KNOTS ( 'NONE', 3,
 ( #2416, #85424, #53955, #24072, #69669, #70670, #38254, #93002, #15971, #84912, #25069, #40258, #55453, #14965, #23555, #94517 ),
 .UNSPECIFIED., .F., .F.,
 ( 4, 1, 2, 2, 2, 1, 2, 2, 4 ),
 ( 0.000000000000000000, 0.1250000000000077161, 0.1875000000000082712, 0.2500000000000088263, 0.5000000000000096589, 0.6250000000000094369, 0.6875000000000069944, 0.7500000000000045519, 1.000000000000000000 ),
 .UNSPECIFIED. ) ;
#84459=CARTESIAN_POINT ( 'NONE',  ( 73.11654091825437263, 69.80299609433679109, 9.611781565164262631 ) ) ;
#84460=CARTESIAN_POINT ( 'NONE',  ( 34.51575008502857855, 31.87878583063843863, -9.188101187500006262 ) ) ;
#84461=ORIENTED_EDGE ( 'NONE', *, *, #35498, .F. ) ;
#84467=CARTESIAN_POINT ( 'NONE',  ( 84.78687102586546587, 50.23207448519301721, 13.79854428445948678 ) ) ;
#84470=CARTESIAN_POINT ( 'NONE',  ( 37.97985170016632850, 33.87878583063844928, -9.188101187500006262 ) ) ;
#84471=CARTESIAN_POINT ( 'NONE',  ( 81.46946648389129564, 55.43478263998397182, -16.31964423845217738 ) ) ;
#84472=CARTESIAN_POINT ( 'NONE',  ( 76.34528211662409092, 62.05049414262115448, -15.76804433278676143 ) ) ;
#84474=CARTESIAN_POINT ( 'NONE',  ( 87.11840409666331198, 45.31431352401795465, 7.035673371054458336 ) ) ;
#84484=CARTESIAN_POINT ( 'NONE',  ( 82.56099630686816226, 41.03468078478306325, 1.095390248834374303 ) ) ;
#84486=CARTESIAN_POINT ( 'NONE',  ( 76.77731254116882553, 64.09355814141258634, -15.16545583891342908 ) ) ;
#84490=B_SPLINE_CURVE_WITH_KNOTS ( 'NONE', 3,
 ( #82003, #34365, #65262, #42931, #35357, #25785, #65751, #73870, #64777, #96206 ),
 .UNSPECIFIED., .F., .F.,
 ( 4, 2, 2, 2, 4 ),
 ( 0.000000000000000000, 0.0002622400424272904778, 0.0005244800848545809555, 0.0007867201272818714333, 0.001048960169709161911 ),
 .UNSPECIFIED. ) ;
#84491=CARTESIAN_POINT ( 'NONE',  ( 41.11799749075662191, 32.24335787977766898, -9.188101187500008038 ) ) ;
#84496=CARTESIAN_POINT ( 'NONE',  ( 71.89123681271787802, 63.83798092845757566, -13.42677533865197681 ) ) ;
#84501=CARTESIAN_POINT ( 'NONE',  ( 74.08065690531797998, 54.82731643721707826, -16.13522336645905142 ) ) ;
#84503=CARTESIAN_POINT ( 'NONE',  ( 36.90034965944521872, 21.70852965304481685, 1.583844403245330712 ) ) ;
#84506=LINE ( 'NONE', #29280, #70620 ) ;
#84512=CARTESIAN_POINT ( 'NONE',  ( 72.23865006290039048, 71.95475215217994958, 3.607730569270007237 ) ) ;
#84514=CARTESIAN_POINT ( 'NONE',  ( 69.80892481568059793, 63.14429736086585621, -13.67003195746243271 ) ) ;
#84529=CARTESIAN_POINT ( 'NONE',  ( 75.29676475605360508, 65.28063746041759430, -14.24902546994322883 ) ) ;
#84536=CARTESIAN_POINT ( 'NONE',  ( 66.95904190137821388, 69.24049710015358983, 0.6601133702874718567 ) ) ;
#84538=CARTESIAN_POINT ( 'NONE',  ( 75.85475627067550874, 51.57392296393066289, 15.72404477719369353 ) ) ;
#84546=CARTESIAN_POINT ( 'NONE',  ( 67.86860378221429357, 65.58690806574966814, -10.91583492536020294 ) ) ;
#84552=CARTESIAN_POINT ( 'NONE',  ( 27.21537010445219096, 39.21091486745862653, 7.012934429366973338E-14 ) ) ;
#84556=CARTESIAN_POINT ( 'NONE',  ( 77.15888728817564868, 49.30424767902741934, 15.39427361423193652 ) ) ;
#84557=CARTESIAN_POINT ( 'NONE',  ( 27.74991983456899902, 18.94754757982090254, 5.678558825948272215 ) ) ;
#84560=CARTESIAN_POINT ( 'NONE',  ( 8.301057521190555732, 26.83396525600388571, -2.839279412974133887 ) ) ;
#84566=CARTESIAN_POINT ( 'NONE',  ( 72.67973169220425689, 61.70005665674018758, 14.67617656207863952 ) ) ;
#84568=CARTESIAN_POINT ( 'NONE',  ( 77.70055685185792527, 55.96283670942377597, -16.15846975066150293 ) ) ;
#84574=EDGE_LOOP ( 'NONE', ( #34952, #50667, #4717, #34518 ) ) ;
#84580=CARTESIAN_POINT ( 'NONE',  ( 79.13141068964681324, 45.89859103142725871, -12.52778249399242405 ) ) ;
#84582=CARTESIAN_POINT ( 'NONE',  ( 85.92861092779033072, 42.96335125230519481, 4.056038327995186599 ) ) ;
#84586=CARTESIAN_POINT ( 'NONE',  ( 14.90450122504689823, 30.64646525600389637, -2.839279412974133887 ) ) ;
#84595=CARTESIAN_POINT ( 'NONE',  ( 67.72007239575214044, 65.87765530913392809, -10.53033397204468535 ) ) ;
#84611=VERTEX_POINT ( 'NONE', #43848 ) ;
#84614=CARTESIAN_POINT ( 'NONE',  ( 66.48824783888160539, 67.83064937571610642, 6.804944701791020734 ) ) ;
#84615=CARTESIAN_POINT ( 'NONE',  ( 87.63077671684244763, 43.37939755374765838, -0.6475992473115442793 ) ) ;
#84616=CARTESIAN_POINT ( 'NONE',  ( 81.22503698233943226, 55.71330003141861198, 16.38398667929945773 ) ) ;
#84620=ORIENTED_EDGE ( 'NONE', *, *, #86371, .F. ) ;
#84633=CARTESIAN_POINT ( 'NONE',  ( 87.85193346898986988, 44.00982651358195596, -1.829615609843908253 ) ) ;
#84636=CARTESIAN_POINT ( 'NONE',  ( 72.99830029227618411, 70.81959382475521636, 8.127746218293808056 ) ) ;
#84638=CARTESIAN_POINT ( 'NONE',  ( 74.51773952002177737, 66.51868515611822374, -12.81989038982261597 ) ) ;
#84644=CARTESIAN_POINT ( 'NONE',  ( 84.04820955589276821, 51.68058956114519020, 14.75728579592695766 ) ) ;
#84650=DIRECTION ( 'NONE',  ( -0.1710100716628374096, 0.2961981327260301833, 0.9396926207859057634 ) ) ;
#84652=CARTESIAN_POINT ( 'NONE',  ( 73.67824366220462196, 55.52431661992799405, 16.58293632014991559 ) ) ;
#84653=CARTESIAN_POINT ( 'NONE',  ( 19.21972384509095733, 29.83478043621388309, -8.090169943749479842 ) ) ;
#84663=CARTESIAN_POINT ( 'NONE',  ( 66.71375026165955546, 67.41994310576295391, -6.688024140652689020 ) ) ;
#84665=CARTESIAN_POINT ( 'NONE',  ( 72.81630190666359681, 70.85884106002271210, -7.900673142507891100 ) ) ;
#84671=CARTESIAN_POINT ( 'NONE',  ( 30.24436146177389162, 33.16454794089043645, -10.00000000000000355 ) ) ;
#84681=CARTESIAN_POINT ( 'NONE',  ( 44.08964769951546714, 27.58380873178790793, 6.180339887498953466 ) ) ;
#84684=CARTESIAN_POINT ( 'NONE',  ( 66.87061822793073418, 67.94793007289314346, 7.000923078224633223 ) ) ;
#84685=CARTESIAN_POINT ( 'NONE',  ( 36.78662229117171734, 22.20801979619930933, -3.090169943749474069 ) ) ;
#84686=CARTESIAN_POINT ( 'NONE',  ( 42.15419773769040290, 26.19860640527295814, 2.839279412974134775 ) ) ;
#84693=CARTESIAN_POINT ( 'NONE',  ( 18.74326920199815305, 31.79752408145591858, -5.678558825948271327 ) ) ;
#84695=CARTESIAN_POINT ( 'NONE',  ( 72.04081558064058299, 59.27854915901136934, 15.34716367762108824 ) ) ;
#84698=CARTESIAN_POINT ( 'NONE',  ( 40.84394904227130496, 31.78052372038643725, -10.00000000000000355 ) ) ;
#84699=CARTESIAN_POINT ( 'NONE',  ( 87.62133583293774564, 45.31115884160845297, -7.293173845241971875 ) ) ;
#84701=CARTESIAN_POINT ( 'NONE',  ( 81.74304277033319011, 42.07055560370181269, 7.558611063322482337 ) ) ;
#84704=CARTESIAN_POINT ( 'NONE',  ( 72.31870688955723381, 71.66728745601001549, -5.813503713761849490 ) ) ;
#84706=CARTESIAN_POINT ( 'NONE',  ( 28.84760059290936951, 18.78380873178787880, -6.180339887498949025 ) ) ;
#84710=CARTESIAN_POINT ( 'NONE',  ( 73.05863210132505969, 69.60576123971952711, -9.808587366596247747 ) ) ;
#84714=CYLINDRICAL_SURFACE ( 'NONE', #35119, 16.60714546451156792 ) ;
#84715=CARTESIAN_POINT ( 'NONE',  ( 80.14478464935454838, 57.78471241749840459, 16.60281329265516348 ) ) ;
#84718=ORIENTED_EDGE ( 'NONE', *, *, #36810, .T. ) ;
#84726=CYLINDRICAL_SURFACE ( 'NONE', #55198, 16.60714546451156792 ) ;
#84729=B_SPLINE_CURVE_WITH_KNOTS ( 'NONE', 3,
 ( #10495, #41378, #72317, #33814, #64701, #95652, #49486, #41887, #72826, #98100, #61559, #92506, #69163, #52973, #29193, #38248, #44862, #99587, #53461, #61057, #29681, #5393, #60061, #92028, #36277, #68169, #74814, #22574, #82449, #91024, #51481, #13986, #22077, #82926, #67176, #45365, #60554, #83418, #91511, #75803, #5884, #21588, #83923, #28678, #99097, #75303 ),
 .UNSPECIFIED., .F., .F.,
 ( 4, 1, 1, 1, 2, 2, 1, 1, 1, 2, 2, 1, 1, 2, 2, 1, 1, 2, 2, 1, 1, 2, 2, 1, 2, 2, 1, 2, 2, 4 ),
 ( 0.000000000000000000, 0.06250000000000432987, 0.09375000000000677236, 0.1093750000000077022, 0.1171875000000101169, 0.1250000000000125178, 0.1875000000000266454, 0.2187500000000355826, 0.2343750000000378308, 0.2421875000000389966, 0.2500000000000401346, 0.3125000000000325295, 0.3437500000000286993, 0.3593750000000287548, 0.3750000000000287548, 0.4375000000000236478, 0.4687500000000210942, 0.4843750000000198730, 0.5000000000000186517, 0.5625000000000140998, 0.5937500000000134337, 0.6093750000000115463, 0.6250000000000096589, 0.6875000000000064393, 0.7187500000000063283, 0.7500000000000063283, 0.8125000000000061062, 0.8437500000000059952, 0.8750000000000059952, 1.000000000000000000 ),
 .UNSPECIFIED. ) ;
#84731=CARTESIAN_POINT ( 'NONE',  ( 24.39104846783644831, 37.58029201028042365, 1.583844403245397769 ) ) ;
#84733=CARTESIAN_POINT ( 'NONE',  ( 83.25425189550011851, 52.37281273071425858, 14.86008439172370110 ) ) ;
#84736=CARTESIAN_POINT ( 'NONE',  ( 86.68854498236711947, 46.42444261617848866, 9.093522239322870959 ) ) ;
#84742=CARTESIAN_POINT ( 'NONE',  ( 7.533646096595723485, 16.30066082961419482, -10.00000000000000533 ) ) ;
#84748=CARTESIAN_POINT ( 'NONE',  ( 73.78444379368663419, 64.77329786477272933, -13.56033333088950066 ) ) ;
#84749=CARTESIAN_POINT ( 'NONE',  ( 78.15171962155767460, 47.58880439823153097, 14.43428839942771447 ) ) ;
#84753=CARTESIAN_POINT ( 'NONE',  ( 84.43516343181975969, 42.02615065117144866, -0.07733096528512554968 ) ) ;
#84754=CARTESIAN_POINT ( 'NONE',  ( 87.72955037964742075, 45.02833699891566255, -6.646681420800613971 ) ) ;
#84755=CARTESIAN_POINT ( 'NONE',  ( 79.09664598837733251, 45.97851813324576398, 13.19840075976098426 ) ) ;
#84758=EDGE_CURVE ( 'NONE', #22248, #82006, #87834, .T. ) ;
#84759=DIRECTION ( 'NONE',  ( -0.8660254037844377084, -0.5000000000000014433, -0.000000000000000000 ) ) ;
#84764=DIRECTION ( 'NONE',  ( -0.8660254037844377084, -0.5000000000000014433, -0.000000000000000000 ) ) ;
#84774=CARTESIAN_POINT ( 'NONE',  ( 68.79270342570836760, 66.32932566076951275, -9.981102178220000454 ) ) ;
#84775=ORIENTED_EDGE ( 'NONE', *, *, #13452, .T. ) ;
#84776=CARTESIAN_POINT ( 'NONE',  ( 71.49814397558004941, 64.90871843161637855, 12.62364874555859551 ) ) ;
#84780=CARTESIAN_POINT ( 'NONE',  ( 81.97090630940145672, 41.81567222034367859, -5.612609715771486485 ) ) ;
#84790=CARTESIAN_POINT ( 'NONE',  ( 11.88462290154380874, 22.56454794089040305, 10.00000000000000355 ) ) ;
#84793=PLANE ( 'NONE',  #86362 ) ;
#84797=CARTESIAN_POINT ( 'NONE',  ( 72.75680339015909226, 57.15378132276418199, 15.89129174203703521 ) ) ;
#84799=CARTESIAN_POINT ( 'NONE',  ( 16.09091216865756024, 14.45404122711132366, -8.090169943749478065 ) ) ;
#84805=CARTESIAN_POINT ( 'NONE',  ( 35.63556891041371699, 26.28920272979929607, -7.433330006724141015 ) ) ;
#84812=CARTESIAN_POINT ( 'NONE',  ( 68.52700701264937777, 64.29941490235316337, 12.37827088797565978 ) ) ;
#84814=CARTESIAN_POINT ( 'NONE',  ( 80.22679522040971278, 47.49802419697316225, 13.74028476495392681 ) ) ;
#84819=CARTESIAN_POINT ( 'NONE',  ( 5.211622267866312441, 23.98502408145590081, -5.678558825948271327 ) ) ;
#84823=CARTESIAN_POINT ( 'NONE',  ( 69.93840568465007834, 62.63376372532634662, 13.43677035550434873 ) ) ;
#84835=CARTESIAN_POINT ( 'NONE',  ( 26.39431744575845684, 16.20801979619929156, -3.090169943749474069 ) ) ;
#84839=CARTESIAN_POINT ( 'NONE',  ( 79.29174861055801671, 59.84975646172946995, -16.14905532231970042 ) ) ;
#84842=CARTESIAN_POINT ( 'NONE',  ( 69.75455253191417171, 62.54871372033364452, 13.42486103269802911 ) ) ;
#84847=CARTESIAN_POINT ( 'NONE',  ( 81.61705240089096947, 42.28877732484014729, -8.032517907699986637 ) ) ;
#84851=CARTESIAN_POINT ( 'NONE',  ( 74.29311029226887797, 65.49125867801090806, 13.36500919525239972 ) ) ;
#84853=CARTESIAN_POINT ( 'NONE',  ( 71.26884625214724167, 71.79727854084720207, 1.363308781743589604 ) ) ;
#84856=DIRECTION ( 'NONE',  ( -0.4924038765061016787, 0.8528685319524424990, -0.1736481776669404342 ) ) ;
#84860=B_SPLINE_CURVE_WITH_KNOTS ( 'NONE', 3,
 ( #44545, #89722, #75479, #82121, #12694, #36455, #67358, #98286, #6063, #36957, #67868, #29372, #60238, #91199, #73486, #52646, #83601, #4070, #330, #85481, #54503, #32725, #71753, #46930, #6571, #38818, #2346, #77847, #8931, #47913, #75994 ),
 .UNSPECIFIED., .F., .F.,
 ( 4, 3, 3, 3, 3, 3, 3, 3, 3, 3, 4 ),
 ( 0.000000000000000000, 0.1333490885032341255, 0.3007194338854348725, 0.4699862290245032659, 0.5844252810809253962, 0.6686540514502775645, 0.7354980260655532565, 0.8028463152565672445, 0.8633854507757174890, 0.9437142632667334663, 1.000000000000000000 ),
 .UNSPECIFIED. ) ;
#84861=FACE_OUTER_BOUND ( 'NONE', #33626, .T. ) ;
#84864=CARTESIAN_POINT ( 'NONE',  ( 11.44039960990914651, 28.64646525600389282, -2.839279412974133887 ) ) ;
#84871=CARTESIAN_POINT ( 'NONE',  ( 79.73452763708452551, 44.91547317212032198, 11.49829713998203040 ) ) ;
#84873=CARTESIAN_POINT ( 'NONE',  ( 67.73992565572970648, 65.91850390810078864, -10.49939607295521959 ) ) ;
#84874=TOROIDAL_SURFACE ( 'NONE', #24953, 15.10714546451156970, 0.5000000000000000000 ) ;
#84880=CARTESIAN_POINT ( 'NONE',  ( 75.03626624455306171, 62.25040173119386111, -15.04310718129558211 ) ) ;
#84887=CARTESIAN_POINT ( 'NONE',  ( 72.96752522106987726, 70.88037482455226268, 8.005050465142893756 ) ) ;
#84890=CARTESIAN_POINT ( 'NONE',  ( 65.88310562893971678, 69.02589174555536999, 1.996831191813055240 ) ) ;
#84896=CARTESIAN_POINT ( 'NONE',  ( 84.82746753971869680, 42.25127123179836985, 0.4482709252177607961 ) ) ;
#84898=CARTESIAN_POINT ( 'NONE',  ( 83.07807837777205862, 43.85925945439043971, 8.248572388415514212 ) ) ;
#84910=CARTESIAN_POINT ( 'NONE',  ( 83.14218550195334956, 50.27791214501019113, 14.33927766777896906 ) ) ;
#84912=CARTESIAN_POINT ( 'NONE',  ( 72.62777135225290692, 66.58284297640395266, 12.45031013499460038 ) ) ;
#84915=CARTESIAN_POINT ( 'NONE',  ( 69.26629474405157794, 69.23362429141876362, 6.083831639397693891 ) ) ;
#84919=CARTESIAN_POINT ( 'NONE',  ( 74.69795600089807408, 60.20801014145679630, 16.00524392222005332 ) ) ;
#84920=CARTESIAN_POINT ( 'NONE',  ( 81.98204644731730184, 41.14170830008083612, -5.380964918418897902 ) ) ;
#84922=CARTESIAN_POINT ( 'NONE',  ( 15.62556418158687244, 11.94754757982088123, 5.678558825948272215 ) ) ;
#84925=CARTESIAN_POINT ( 'NONE',  ( 14.19121639173650706, 20.14441083166259716, 10.00000000000000533 ) ) ;
#84933=CARTESIAN_POINT ( 'NONE',  ( 86.47816187992320636, 47.39707827577768029, 10.33711315380114115 ) ) ;
#84935=CARTESIAN_POINT ( 'NONE',  ( 23.65314546706850862, 31.84336893147757408, -7.433330006724137462 ) ) ;
#84936=CARTESIAN_POINT ( 'NONE',  ( 72.71768624772042244, 63.97145380353339306, -14.16538725607713012 ) ) ;
#84940=CARTESIAN_POINT ( 'NONE',  ( 84.82070890866113189, 50.11195492342548619, -13.71672402108478295 ) ) ;
#84941=CARTESIAN_POINT ( 'NONE',  ( 83.87686851671099930, 42.61110357726119702, 6.252421602106308818 ) ) ;
#84949=CARTESIAN_POINT ( 'NONE',  ( 36.63328578856461348, 23.01110640527294748, 2.839279412974134775 ) ) ;
#84956=CARTESIAN_POINT ( 'NONE',  ( 86.51235478091771824, 47.18193832426288736, -10.10603714529630537 ) ) ;
#84958=CARTESIAN_POINT ( 'NONE',  ( 84.54065070028998718, 50.22889876405420040, 13.87834917160721737 ) ) ;
#84962=CARTESIAN_POINT ( 'NONE',  ( 81.60881798005151211, 55.57634303931474307, -16.32954282162994275 ) ) ;
#84963=CARTESIAN_POINT ( 'NONE',  ( 71.79755147005840854, 63.53309442284064801, -14.10203765313787017 ) ) ;
#84976=CARTESIAN_POINT ( 'NONE',  ( 78.44203751522360335, 61.21016990572091032, 16.24725970467587999 ) ) ;
#84979=CARTESIAN_POINT ( 'NONE',  ( 70.39799145693270077, 61.05877478468345743, -14.90226077307323393 ) ) ;
#84980=CARTESIAN_POINT ( 'NONE',  ( 37.26657704017246431, 36.91421378149922816, 9.188101187500008038 ) ) ;
#84984=CARTESIAN_POINT ( 'NONE',  ( 73.86461842229320496, 68.29997319365683950, -11.61748300246921417 ) ) ;
#84986=CARTESIAN_POINT ( 'NONE',  ( 74.72625485415514390, 63.07837140537560572, -14.64344360945962720 ) ) ;
#84989=CARTESIAN_POINT ( 'NONE',  ( 73.55883212634472557, 67.59623184424712861, 11.56650193424350093 ) ) ;
#84991=CARTESIAN_POINT ( 'NONE',  ( 20.69167212271446488, 17.11029122506294087, -8.090169943749478065 ) ) ;
#85004=CARTESIAN_POINT ( 'NONE',  ( 29.42114147039228200, 17.39040679176983772, 1.333680081654574804E-15 ) ) ;
#85006=CARTESIAN_POINT ( 'NONE',  ( 69.76254693980804689, 63.15031056092325201, -13.65041900308473366 ) ) ;
#85008=ORIENTED_EDGE ( 'NONE', *, *, #79193, .F. ) ;
#85017=CARTESIAN_POINT ( 'NONE',  ( 82.95985630027486479, 42.92152901241345830, 6.769544279123342001 ) ) ;
#85019=CARTESIAN_POINT ( 'NONE',  ( 70.38723355792234315, 61.09782911607875633, -14.88300479815616484 ) ) ;
#85020=CARTESIAN_POINT ( 'NONE',  ( 70.84106301243626547, 70.60106795950503056, -5.124797883556153621 ) ) ;
#85022=CARTESIAN_POINT ( 'NONE',  ( 66.47763888060634940, 67.99612994687967671, 6.463816603905435443 ) ) ;
#85027=CARTESIAN_POINT ( 'NONE',  ( 84.84691229513632038, 49.95470102045879912, -13.19661209231484378 ) ) ;
#85029=CARTESIAN_POINT ( 'NONE',  ( 73.22483582419529569, 69.61542381504622767, -9.909891866396675297 ) ) ;
#85030=CARTESIAN_POINT ( 'NONE',  ( 75.84045651381646280, 51.64986437825746179, 15.74133474855197257 ) ) ;
#85040=CARTESIAN_POINT ( 'NONE',  ( 87.91358676412336592, 43.93313586519735736, 0.4560764699024720814 ) ) ;
#85041=CARTESIAN_POINT ( 'NONE',  ( 83.14106290878449101, 49.68186538430950350, -13.54780265075754286 ) ) ;
#85047=CARTESIAN_POINT ( 'NONE',  ( 18.53877768333399345, 26.10171378149918198, 9.188101187500008038 ) ) ;
#85050=CARTESIAN_POINT ( 'NONE',  ( 12.32384911305235420, 19.06628583063839955, -9.188101187500006262 ) ) ;
#85055=CARTESIAN_POINT ( 'NONE',  ( 74.39841895140679640, 68.21392270468032848, 11.45628786500076579 ) ) ;
#85059=CARTESIAN_POINT ( 'NONE',  ( 80.00137380443280222, 55.11996643375317717, -15.99434914381717832 ) ) ;
#85064=CARTESIAN_POINT ( 'NONE',  ( 77.48665757143110966, 49.22860469427720886, 15.29917572744006904 ) ) ;
#85070=CARTESIAN_POINT ( 'NONE',  ( 67.65269435575517321, 68.60991329069676681, -5.309777227589590254 ) ) ;
#85074=CARTESIAN_POINT ( 'NONE',  ( 79.45382063701610775, 46.23955422872901977, -13.23447544246345409 ) ) ;
#85078=CARTESIAN_POINT ( 'NONE',  ( 26.87427219475921092, 30.91421378149919974, 9.188101187500008038 ) ) ;
#85081=CARTESIAN_POINT ( 'NONE',  ( 75.01383350950911222, 67.34328350408776487, -12.89590634041038086 ) ) ;
#85086=B_SPLINE_CURVE_WITH_KNOTS ( 'NONE', 3,
 ( #39368, #78410, #38883, #17085, #46475, #39861, #16091, #56067, #8011, #69786, #62171, #70282, #62675, #396, #77406, #85027, #86553, #32785, #93122, #70798, #30801, #23673, #47485, #63190 ),
 .UNSPECIFIED., .F., .F.,
 ( 4, 2, 2, 2, 2, 2, 2, 2, 2, 2, 2, 4 ),
 ( 0.000000000000000000, 0.1250000000000021927, 0.2500000000000043854, 0.3750000000000065503, 0.4375000000000026090, 0.4999999999999986677, 0.5624999999999946709, 0.6249999999999906741, 0.6874999999999866773, 0.7499999999999825695, 0.8749999999999913403, 1.000000000000000000 ),
 .UNSPECIFIED. ) ;
#85088=AXIS2_PLACEMENT_3D ( 'NONE', #96000, #42232, #89881 ) ;
#85091=CARTESIAN_POINT ( 'NONE',  ( 67.90944760599185770, 65.67478569269405853, 10.85168271666284312 ) ) ;
#85092=CARTESIAN_POINT ( 'NONE',  ( 67.91597355651013856, 65.35775589351075610, -10.44541676389640372 ) ) ;
#85093=CARTESIAN_POINT ( 'NONE',  ( 69.31540213678381690, 70.94726294322936155, -2.438276973829965222 ) ) ;
#85101=ORIENTED_EDGE ( 'NONE', *, *, #21060, .T. ) ;
#85109=CARTESIAN_POINT ( 'NONE',  ( 66.61936531471503997, 67.57008932741632634, 6.288575924362496572 ) ) ;
#85112=CARTESIAN_POINT ( 'NONE',  ( 80.99918023960148616, 56.04449057398856127, 16.10194400669177384 ) ) ;
#85113=CARTESIAN_POINT ( 'NONE',  ( 78.61788708802706083, 48.81601089383328684, -14.35964102986092605 ) ) ;
#85114=CARTESIAN_POINT ( 'NONE',  ( 72.56631922146607394, 69.50290373287580792, 8.912124407776673252 ) ) ;
#85116=VERTEX_POINT ( 'NONE', #9817 ) ;
#85121=CARTESIAN_POINT ( 'NONE',  ( 83.86025440731803826, 41.72852670257621810, 0.4223142476417495184 ) ) ;
#85138=( BOUNDED_CURVE ( )  B_SPLINE_CURVE ( 2, ( #76790, #54461, #45385, #44880, #83939, #15988, #84925, #46888, #75820, #6407, #93015, #99613, #22594 ),
 .UNSPECIFIED., .F., .T. ) 
 B_SPLINE_CURVE_WITH_KNOTS ( ( 3, 2, 2, 2, 2, 2, 3 ),
 ( 0.2124999999999999944, 0.2149999999999999967, 0.2200000000000000011, 0.2250000000000000056, 0.2300000000000000100, 0.2349999999999999867, 0.2374999999999999889 ),
 .UNSPECIFIED. ) 
 CURVE ( )  GEOMETRIC_REPRESENTATION_ITEM ( )  RATIONAL_B_SPLINE_CURVE ( ( 0.9755282581475768211, 0.9755282581475768211, 1.000000000000000000, 0.9510565162951535312, 1.000000000000000000, 0.9510565162951535312, 1.000000000000000000, 0.9510565162951535312, 1.000000000000000000, 0.9510565162951535312, 1.000000000000000000, 0.9755282581475768211, 0.9755282581475768211 ) ) 
 REPRESENTATION_ITEM ( '' )  );
#85139=AXIS2_PLACEMENT_3D ( 'NONE', #99325, #60777, #39473 ) ;
#85140=CARTESIAN_POINT ( 'NONE',  ( 72.53309028193872621, 70.86290320417140265, 7.626211012637808651 ) ) ;
#85141=FACE_OUTER_BOUND ( 'NONE', #71534, .T. ) ;
#85145=CARTESIAN_POINT ( 'NONE',  ( 82.29787399700251171, 40.87733562811993693, 1.011763546004324166 ) ) ;
#85147=CARTESIAN_POINT ( 'NONE',  ( 84.07404364193551771, 51.51966214638419927, 14.67759748506154516 ) ) ;
#85149=ORIENTED_EDGE ( 'NONE', *, *, #67447, .F. ) ;
#85152=CARTESIAN_POINT ( 'NONE',  ( 79.57426776854913442, 46.24084366570345850, -13.18946159588284317 ) ) ;
#85154=FACE_BOUND ( 'NONE', #31324, .T. ) ;
#85156=CARTESIAN_POINT ( 'NONE',  ( 24.92020183544706668, 36.16126292948897003, -6.180339887498951690 ) ) ;
#85160=VECTOR ( 'NONE', #85406, 1000.000000000000114 ) ;
#85161=B_SPLINE_CURVE_WITH_KNOTS ( 'NONE', 3,
 ( #94726, #72423, #17701, #72924, #81048, #79025, #40478, #25286, #18704, #56172, #64803, #73405, #95244, #10602, #95748, #49585, #25813, #26794, #42470, #3990, #34877, #65777, #27299, #75399, #51071, #66783, #35879, #43473, #97708, #82542, #59153, #60158, #91122, #52079, #28786, #83024, #19712, #21687, #74904, #81528, #90123, #98203, #51586, #20697, #50578, #36371 ),
 .UNSPECIFIED., .F., .F.,
 ( 4, 1, 1, 1, 2, 2, 1, 1, 1, 2, 2, 1, 1, 2, 2, 1, 1, 2, 2, 1, 1, 2, 2, 1, 2, 2, 1, 2, 2, 4 ),
 ( 0.000000000000000000, 0.06250000000000525968, 0.09375000000000867362, 0.1093750000000097006, 0.1171875000000108941, 0.1250000000000120737, 0.1875000000000127676, 0.2187500000000126288, 0.2343750000000140166, 0.2421875000000151823, 0.2500000000000163758, 0.3125000000000134892, 0.3437500000000127676, 0.3593750000000120459, 0.3750000000000112133, 0.4375000000000153766, 0.4687500000000188183, 0.4843750000000199285, 0.5000000000000210942, 0.5625000000000184297, 0.5937500000000172085, 0.6093750000000160982, 0.6250000000000149880, 0.6875000000000138778, 0.7187500000000124345, 0.7500000000000108802, 0.8125000000000085487, 0.8437500000000075495, 0.8750000000000064393, 1.000000000000000000 ),
 .UNSPECIFIED. ) ;
#85165=VERTEX_POINT ( 'NONE', #96435 ) ;
#85167=B_SPLINE_CURVE_WITH_KNOTS ( 'NONE', 3,
 ( #56175, #17704, #79547, #64298, #25816, #95247, #11121, #39971, #26305, #31880 ),
 .UNSPECIFIED., .F., .F.,
 ( 4, 2, 2, 2, 4 ),
 ( 0.000000000000000000, 0.0002622400424273102102, 0.0005244800848546204205, 0.0007867201272819306307, 0.001048960169709240841 ),
 .UNSPECIFIED. ) ;
#85168=CARTESIAN_POINT ( 'NONE',  ( 72.75722467535679527, 70.26520034150425431, -8.071865018468246333 ) ) ;
#85174=CARTESIAN_POINT ( 'NONE',  ( 32.64838280634442214, 30.80066082961423746, 10.00000000000000533 ) ) ;
#85175=CARTESIAN_POINT ( 'NONE',  ( 83.27929122224395542, 41.83289114379940798, -3.541494727109722351 ) ) ;
#85177=CARTESIAN_POINT ( 'NONE',  ( 81.57324034346744668, 55.97255112923638620, 16.04000112846837212 ) ) ;
#85178=CARTESIAN_POINT ( 'NONE',  ( 83.27435412308909690, 44.55311305779904529, 9.827056061616449512 ) ) ;
#85185=DIRECTION ( 'NONE',  ( 0.5000000000000013323, -0.8660254037844378194, 0.000000000000000000 ) ) ;
#85191=CARTESIAN_POINT ( 'NONE',  ( 69.95523204135938045, 62.90150226501648234, 13.86126985460704297 ) ) ;
#85193=CARTESIAN_POINT ( 'NONE',  ( 18.65184876021338312, 28.95586893147755703, 7.433330006724141015 ) ) ;
#85195=CARTESIAN_POINT ( 'NONE',  ( 71.42966913292450215, 59.23173737558743568, 15.26165678737305065 ) ) ;
#85200=CARTESIAN_POINT ( 'NONE',  ( 15.64721481668148328, 11.96004757982089295, -5.678558825948275768 ) ) ;
#85201=CARTESIAN_POINT ( 'NONE',  ( 73.98867670750783532, 59.60256495767924179, -15.59328569222777183 ) ) ;
#85202=CARTESIAN_POINT ( 'NONE',  ( 81.51617444448474714, 41.98210561432389909, 7.630276461086227258 ) ) ;
#85206=CARTESIAN_POINT ( 'NONE',  ( 72.61141802365665399, 71.36933893402679985, -5.910933643996240328 ) ) ;
#85210=CARTESIAN_POINT ( 'NONE',  ( 66.29454943693276903, 69.24199052626691753, -2.144636311159408226 ) ) ;
#85212=ORIENTED_EDGE ( 'NONE', *, *, #22512, .F. ) ;
#85214=CARTESIAN_POINT ( 'NONE',  ( 86.62800554614717896, 43.31088370039552160, -1.499291040926804763 ) ) ;
#85219=CARTESIAN_POINT ( 'NONE',  ( 84.14312167556933275, 48.98415679381830756, 0.000000000000000000 ) ) ;
#85227=ORIENTED_EDGE ( 'NONE', *, *, #77006, .T. ) ;
#85228=CARTESIAN_POINT ( 'NONE',  ( 33.16918417342686354, 21.01110640527294038, 2.839279412974134775 ) ) ;
#85230=CARTESIAN_POINT ( 'NONE',  ( 78.19043972245502516, 47.52173921620315156, -13.84048554213443261 ) ) ;
#85234=CARTESIAN_POINT ( 'NONE',  ( 78.19098230064227550, 47.51660667919665570, -14.38750087007935186 ) ) ;
#85235=CARTESIAN_POINT ( 'NONE',  ( 83.81658881107364323, 52.06750489740826993, 14.58996321880578151 ) ) ;
#85250=CARTESIAN_POINT ( 'NONE',  ( 70.80090459924991819, 69.25659177360545016, 7.761957622020450920 ) ) ;
#85252=CARTESIAN_POINT ( 'NONE',  ( 67.56978446451059028, 66.68927659431298594, 8.641485439713591177 ) ) ;
#85253=CARTESIAN_POINT ( 'NONE',  ( 68.80791472686313170, 65.65516334055519110, -10.66944597666374861 ) ) ;
#85254=CARTESIAN_POINT ( 'NONE',  ( 78.21265317814797413, 47.50325902310300563, 14.37429833372570620 ) ) ;
#85258=CARTESIAN_POINT ( 'NONE',  ( 70.21724893432667614, 65.14247767143801582, 11.87715301600730911 ) ) ;
#85260=CARTESIAN_POINT ( 'NONE',  ( 87.60591442325252842, 44.91970625728536959, -6.572271063428638982 ) ) ;
#85261=DIRECTION ( 'NONE',  ( 0.1039558454088763267, -0.1800568059919503139, 0.9781476007338069101 ) ) ;
#85263=CARTESIAN_POINT ( 'NONE',  ( 83.91468266313496827, 51.82819685387456587, -14.47034327719529045 ) ) ;
#85266=DIRECTION ( 'NONE',  ( 0.7162481363636786780, 0.000000000000000000, -0.6978456900745014790 ) ) ;
#85267=CARTESIAN_POINT ( 'NONE',  ( 72.05417303993513656, 71.64307123591491688, 5.506498905688426149 ) ) ;
#85279=CARTESIAN_POINT ( 'NONE',  ( 72.55067284226147706, 68.13922894791654983, 10.49063991969712184 ) ) ;
#85280=CARTESIAN_POINT ( 'NONE',  ( 88.03972809732340465, 44.75281308623453924, -4.524080385986239961 ) ) ;
#85285=LINE ( 'NONE', #91380, #12321 ) ;
#85293=CARTESIAN_POINT ( 'NONE',  ( 88.01007674647709678, 44.79289111569436699, 4.713013503925086667 ) ) ;
#85296=CARTESIAN_POINT ( 'NONE',  ( 11.69612814616573893, 25.49103043416548076, -8.090169943749479842 ) ) ;
#85304=CARTESIAN_POINT ( 'NONE',  ( 73.16329361895407146, 57.31197931467701068, 16.38585881187776749 ) ) ;
#85306=CARTESIAN_POINT ( 'NONE',  ( 18.98444911510674160, 11.36477965099639675, 1.583844403245364907 ) ) ;
#85312=CARTESIAN_POINT ( 'NONE',  ( 25.62156559687931434, 36.83396525600391413, -2.839279412974133887 ) ) ;
#85317=CARTESIAN_POINT ( 'NONE',  ( 71.63103492117565452, 72.07843208848032646, 3.395715836721224790 ) ) ;
#85318=CARTESIAN_POINT ( 'NONE',  ( 66.50888126359876651, 68.78582482296066303, 2.298140800692767716 ) ) ;
#85324=CARTESIAN_POINT ( 'NONE',  ( 9.878523645489616811, 21.10171378149916777, 9.188101187500008038 ) ) ;
#85327=CARTESIAN_POINT ( 'NONE',  ( 88.21965799167087141, 44.33377460087322675, -2.453011004722113420 ) ) ;
#85329=LINE ( 'NONE', #17903, #83003 ) ;
#85333=FACE_OUTER_BOUND ( 'NONE', #20417, .T. ) ;
#85341=CARTESIAN_POINT ( 'NONE',  ( 85.21473396346020479, 45.07546406142533613, -8.320173855083872638 ) ) ;
#85342=ORIENTED_EDGE ( 'NONE', *, *, #33431, .F. ) ;
#85344=CARTESIAN_POINT ( 'NONE',  ( 79.13444159074370532, 60.15296345131730504, -16.46386276767553269 ) ) ;
#85345=CARTESIAN_POINT ( 'NONE',  ( 11.19180257851625448, 22.16454794089040092, -10.00000000000000355 ) ) ;
#85347=CARTESIAN_POINT ( 'NONE',  ( 69.94244964693436373, 62.64957029637712083, 13.42917468561056715 ) ) ;
#85352=CARTESIAN_POINT ( 'NONE',  ( 81.49773370583855581, 42.20892728461021193, -8.015322006907149799 ) ) ;
#85355=VERTEX_POINT ( 'NONE', #7162 ) ;
#85356=CARTESIAN_POINT ( 'NONE',  ( 73.27092031662876082, 60.84575549105485948, 15.12685931616829649 ) ) ;
#85357=B_SPLINE_CURVE_WITH_KNOTS ( 'NONE', 3,
 ( #2237, #95481, #56904, #80264, #13325, #13802, #29019, #60876, #21896, #74639, #52784, #37097, #67496, #98429, #66996, #44188 ),
 .UNSPECIFIED., .F., .F.,
 ( 4, 1, 2, 2, 2, 1, 2, 2, 4 ),
 ( 0.000000000000000000, 0.1249999999999920619, 0.1874999999999899247, 0.2499999999999877875, 0.4999999999999824585, 0.6249999999999813483, 0.6874999999999823475, 0.7499999999999832356, 1.000000000000000000 ),
 .UNSPECIFIED. ) ;
#85358=ORIENTED_EDGE ( 'NONE', *, *, #39011, .T. ) ;
#85359=CARTESIAN_POINT ( 'NONE',  ( 68.84931682549257914, 69.27838879186909082, 5.464616672756219096 ) ) ;
#85364=CARTESIAN_POINT ( 'NONE',  ( 81.05763270389509501, 43.67158023151814916, 9.470390458390101074 ) ) ;
#85369=CARTESIAN_POINT ( 'NONE',  ( 82.73042059842214258, 53.63367031839453603, -15.74978661431508264 ) ) ;
#85374=CARTESIAN_POINT ( 'NONE',  ( 17.19524200933981817, 21.87878583063841020, -9.188101187500006262 ) ) ;
#85376=CARTESIAN_POINT ( 'NONE',  ( 80.02542612678608691, 57.59583086733049839, 16.60012225046075329 ) ) ;
#85377=PLANE ( 'NONE',  #60589 ) ;
#85383=CARTESIAN_POINT ( 'NONE',  ( 83.83491441254412280, 45.74439801777876369, -10.08379609569576196 ) ) ;
#85386=ORIENTED_EDGE ( 'NONE', *, *, #56220, .T. ) ;
#85394=CARTESIAN_POINT ( 'NONE',  ( 11.59314018038319283, 18.64441083166259361, -10.00000000000000533 ) ) ;
#85399=CARTESIAN_POINT ( 'NONE',  ( 75.79515598915105556, 65.48576791014883725, 14.28791538466101585 ) ) ;
#85406=DIRECTION ( 'NONE',  ( -0.3715724127386920705, 0.6435822975543701308, -0.6691306063588670083 ) ) ;
#85408=CARTESIAN_POINT ( 'NONE',  ( 74.02866129013209218, 68.91877476116354728, -11.13505360475025263 ) ) ;
#85413=VERTEX_POINT ( 'NONE', #68962 ) ;
#85418=CARTESIAN_POINT ( 'NONE',  ( 80.35245384971769056, 57.10990684815718765, -16.23186976984165852 ) ) ;
#85424=CARTESIAN_POINT ( 'NONE',  ( 71.08204727005846735, 61.55506161651749153, 14.86215617804459832 ) ) ;
#85427=CARTESIAN_POINT ( 'NONE',  ( 67.69237348538018750, 66.82088825431439716, 8.559571887000263501 ) ) ;
#85436=CARTESIAN_POINT ( 'NONE',  ( 10.03310832875943603, 27.83396525600388571, -2.839279412974133887 ) ) ;
#85447=CARTESIAN_POINT ( 'NONE',  ( 81.35996782917339942, 56.22057934968196946, -16.44131086233301531 ) ) ;
#85456=CARTESIAN_POINT ( 'NONE',  ( 79.22961533192220429, 50.25035061149957727, 14.80838524028136050 ) ) ;
#85457=CARTESIAN_POINT ( 'NONE',  ( 75.28650001057752661, 66.67572118895705557, 13.44401380721711270 ) ) ;
#85462=ORIENTED_EDGE ( 'NONE', *, *, #6421, .T. ) ;
#85464=EDGE_CURVE ( 'NONE', #65130, #18732, #28993, .T. ) ;
#85465=CARTESIAN_POINT ( 'NONE',  ( 43.56148901884012048, 27.01110640527296169, 2.839279412974134775 ) ) ;
#85471=FACE_OUTER_BOUND ( 'NONE', #52764, .T. ) ;
#85476=CARTESIAN_POINT ( 'NONE',  ( 80.33241032415608629, 44.91708578747144287, 11.19148706010553163 ) ) ;
#85477=CARTESIAN_POINT ( 'NONE',  ( 86.32721218574307898, 47.55264674982593931, -11.12316258729872054 ) ) ;
#85481=CARTESIAN_POINT ( 'NONE',  ( 81.32396741884589630, 55.80035763937271298, 16.38826086546822580 ) ) ;
#85489=CARTESIAN_POINT ( 'NONE',  ( 82.57480368249606784, 41.04376301281223505, 1.111617510708537093 ) ) ;
#85492=CARTESIAN_POINT ( 'NONE',  ( 76.71798530001490235, 63.32448642232582614, -15.43374014074777989 ) ) ;
#85495=CARTESIAN_POINT ( 'NONE',  ( 70.40053591592641169, 61.13412726347223725, -14.87056803518813908 ) ) ;
#85507=CARTESIAN_POINT ( 'NONE',  ( 72.07340273975241018, 61.96641754224930310, 14.42752318807301748 ) ) ;
#85516=CARTESIAN_POINT ( 'NONE',  ( 65.74174769441147248, 69.08343887585857601, -0.02323972613207190424 ) ) ;
#85523=EDGE_CURVE ( 'NONE', #23117, #65477, #27469, .T. ) ;
#85538=CARTESIAN_POINT ( 'NONE',  ( 74.41143754142076716, 68.29725791098579180, 11.39274163773210446 ) ) ;
#85539=CARTESIAN_POINT ( 'NONE',  ( 68.07599697842495345, 69.84362665757917910, 1.500371073846174408 ) ) ;
#85541=CARTESIAN_POINT ( 'NONE',  ( 68.59054070044055607, 66.75779901073921963, -10.13948842260730743 ) ) ;
#85552=CARTESIAN_POINT ( 'NONE',  ( 73.44884507967250897, 69.80860085198864340, -9.835095417347671898 ) ) ;
#85553=CARTESIAN_POINT ( 'NONE',  ( 76.14697209829881785, 51.34588985376412751, 15.63759721918819778 ) ) ;
#85563=CARTESIAN_POINT ( 'NONE',  ( 88.22650267082845232, 44.11417692641830968, 0.5019829077109546622 ) ) ;
#85565=CARTESIAN_POINT ( 'NONE',  ( 83.67203105669065621, 49.52337951222926193, -13.28627613491497605 ) ) ;
#85567=CARTESIAN_POINT ( 'NONE',  ( 77.06710730379538177, 49.53326525838865280, 15.49076735042929442 ) ) ;
#85571=CARTESIAN_POINT ( 'NONE',  ( 23.88951478931043937, 35.83396525600391413, -2.839279412974133887 ) ) ;
#85572=LINE ( 'NONE', #32311, #41772 ) ;
#85574=CARTESIAN_POINT ( 'NONE',  ( 9.878523645489616811, 21.10171378149917487, 9.188101187500008038 ) ) ;
#85576=CARTESIAN_POINT ( 'NONE',  ( 77.23319965423435463, 63.36835149973478565, 15.13843137913277914 ) ) ;
#85580=CARTESIAN_POINT ( 'NONE',  ( 69.39596420143790567, 62.75002488050670024, -13.76244142531616887 ) ) ;
#85584=CARTESIAN_POINT ( 'NONE',  ( 87.42519804963990282, 45.01967495469427405, -6.116160441020238814 ) ) ;
#85588=EDGE_LOOP ( 'NONE', ( #39965, #53622, #71749, #8573 ) ) ;
#85590=CARTESIAN_POINT ( 'NONE',  ( 82.31933756389703660, 53.70313499084333131, 15.83617117143144881 ) ) ;
#85594=CARTESIAN_POINT ( 'NONE',  ( 67.55901250501347022, 68.59136760746119421, -5.217548882598939564 ) ) ;
#85595=ADVANCED_FACE ( 'NONE', ( #64372 ), #86229, .T. ) ;
#85601=CARTESIAN_POINT ( 'NONE',  ( 81.46486379701710234, 43.57149586615976489, 9.885361616454591882 ) ) ;
#85604=CARTESIAN_POINT ( 'NONE',  ( 32.62131273085646654, 21.76004757982090965, 5.678558825948272215 ) ) ;
#85606=CARTESIAN_POINT ( 'NONE',  ( 75.06349586682162567, 67.01194365216524318, -13.14257922886206664 ) ) ;
#85612=CARTESIAN_POINT ( 'NONE',  ( 67.84042995000689302, 66.00558543355286645, -10.46828802347326359 ) ) ;
#85613=CARTESIAN_POINT ( 'NONE',  ( 81.57878911124544175, 55.16394943497986958, -15.91603754490293632 ) ) ;
#85615=CARTESIAN_POINT ( 'NONE',  ( 35.44051388448051654, 36.16454794089043645, -10.00000000000000355 ) ) ;
#85627=CARTESIAN_POINT ( 'NONE',  ( 66.81926193948103787, 67.91930224376029912, 6.999017448319921009 ) ) ;
#85628=CARTESIAN_POINT ( 'NONE',  ( 72.84093999290330146, 56.97456911652175648, -16.40692799624909171 ) ) ;
#85631=CARTESIAN_POINT ( 'NONE',  ( 81.14348526936038297, 56.16770390221125098, 16.10765411318869411 ) ) ;
#85635=ORIENTED_EDGE ( 'NONE', *, *, #99046, .F. ) ;
#85641=CARTESIAN_POINT ( 'NONE',  ( 76.45097149964601613, 51.61755418639809534, -15.65867827852782845 ) ) ;
#85643=CARTESIAN_POINT ( 'NONE',  ( 76.23134959265127009, 65.22726518599165502, -14.14128234971493647 ) ) ;
#85659=CARTESIAN_POINT ( 'NONE',  ( 72.02537281085561460, 67.13575061744317907, -11.13262944115481545 ) ) ;
#85660=ORIENTED_EDGE ( 'NONE', *, *, #76595, .F. ) ;
#85664=CARTESIAN_POINT ( 'NONE',  ( 72.22505610272034460, 71.11034894417089447, -5.995499026437220103 ) ) ;
#85667=EDGE_CURVE ( 'NONE', #33229, #5854, #6993, .T. ) ;
#85675=FACE_BOUND ( 'NONE', #23882, .T. ) ;
#85677=CARTESIAN_POINT ( 'NONE',  ( 33.32252067603396029, 20.20801979619930577, -3.090169943749474069 ) ) ;
#85688=B_SPLINE_CURVE_WITH_KNOTS ( 'NONE', 3,
 ( #77954, #24731, #78973, #71356, #8053, #47530, #23721, #24244, #54115, #62218 ),
 .UNSPECIFIED., .F., .F.,
 ( 4, 2, 2, 2, 4 ),
 ( 0.000000000000000000, 0.0002622400424272615296, 0.0005244800848545230591, 0.0007867201272817845887, 0.001048960169709046118 ),
 .UNSPECIFIED. ) ;
#85693=CARTESIAN_POINT ( 'NONE',  ( 31.78235740255998820, 30.30066082961423746, -10.00000000000000533 ) ) ;
#85696=CARTESIAN_POINT ( 'NONE',  ( 81.52168578289229117, 56.03111392393292078, 16.05417868975104057 ) ) ;
#85711=CARTESIAN_POINT ( 'NONE',  ( 67.16990927158769864, 66.79708245712438952, -9.067759095352206700 ) ) ;
#85712=ADVANCED_FACE ( 'NONE', ( #63253 ), #91121, .T. ) ;
#85716=CARTESIAN_POINT ( 'NONE',  ( 18.54180792094154029, 32.74646525600390135, 2.839279412974139660 ) ) ;
#85723=CARTESIAN_POINT ( 'NONE',  ( 11.28581492663932906, 21.91421378149917487, 9.188101187500008038 ) ) ;
#85726=CARTESIAN_POINT ( 'NONE',  ( 74.53866558554922506, 59.42414767716603308, -15.71004193905537250 ) ) ;
#85727=CARTESIAN_POINT ( 'NONE',  ( 71.65515660876562265, 72.43366598492664821, -1.354044368658560815 ) ) ;
#85728=CARTESIAN_POINT ( 'NONE',  ( 39.59743582264582784, 38.56454794089045635, 10.00000000000000355 ) ) ;
#85732=CARTESIAN_POINT ( 'NONE',  ( 72.32516777325903945, 71.91622842696713747, -5.210293257461823480 ) ) ;
#85734=CARTESIAN_POINT ( 'NONE',  ( 84.69349035698814987, 42.09509699793907345, 3.525966048916779449 ) ) ;
#85737=CARTESIAN_POINT ( 'NONE',  ( 67.66242840994728169, 69.85685045095124224, 3.195176300350167420 ) ) ;
#85738=CARTESIAN_POINT ( 'NONE',  ( 83.30637669978878534, 42.44484529871528622, -5.357148773537285358 ) ) ;
#85739=B_SPLINE_CURVE_WITH_KNOTS ( 'NONE', 3,
 ( #13034, #43896, #84933, #39272, #31676, #31183, #71724, #86962, #1808, #61585, #70182, #40773, #93536, #1307, #62074, #46373, #24588, #8894, #62574, #70692, #790, #94038, #94534, #86460 ),
 .UNSPECIFIED., .F., .F.,
 ( 4, 2, 2, 2, 2, 2, 2, 2, 2, 2, 2, 4 ),
 ( 0.000000000000000000, 0.1250000000000079103, 0.2500000000000158207, 0.3750000000000237588, 0.4375000000000213718, 0.5000000000000189848, 0.5625000000000166533, 0.6250000000000142109, 0.6875000000000118794, 0.7500000000000094369, 0.8750000000000047740, 1.000000000000000000 ),
 .UNSPECIFIED. ) ;
#85742=CARTESIAN_POINT ( 'NONE',  ( 72.09323793696012217, 72.40190342410335234, -3.152634433464706287 ) ) ;
#85743=CARTESIAN_POINT ( 'NONE',  ( 72.67720189414116305, 57.07760858790099689, -16.37924670756266110 ) ) ;
#85744=CARTESIAN_POINT ( 'NONE',  ( 76.62413771374467331, 63.45693921867285070, 15.36854489724363759 ) ) ;
#85746=AXIS2_PLACEMENT_3D ( 'NONE', #87742, #19296, #95329 ) ;
#85752=CARTESIAN_POINT ( 'NONE',  ( 32.96772289237024012, 21.96004757982091959, -5.678558825948276656 ) ) ;
#85758=( BOUNDED_CURVE ( )  B_SPLINE_CURVE ( 2, ( #46135, #77049, #70, #30953, #36557, #98391, #28983, #21374, #94299, #48158, #32951, #62847, #40544, #2579, #78072, #64359, #77577, #40038, #32463, #39036, #63856, #1065, #79099, #63359, #87239, #55727, #24853, #70454, #8658, #95322, #31445, #39530, #1580, #86715, #47147, #2072, #9683, #17253, #71479, #16256, #31944, #94794, #93803, #25879, #23844, #25355, #79607, #56247, #17773, #70979, #48674, #10170, #55234, #41037, #71974, #78578, #33464, #85200, #15743, #24363, #46650, #86218, #9163, #8165, #69946, #563, #62338, #93292, #54738, #85723, #57741, #5062, #10670, #95815, #64868, #42537, #20266, #27363, #41547, #97773, #35944, #26369, #72492, #18274, #43026, #73967, #19774, #57244, #51140, #34943, #27854, #4551, #33984, #88219, #66845, #89706, #12164, #50642, #35451, #65840, #3093, #82104, #12675, #88719, #58246, #43543, #56754, #87736, #66354, #97287, #81595, #73470, #19289, #49650, #49168, #74484, #80104, #18771, #80607, #11184, #42051, #72985, #3577, #34457, #65355, #96294, #26863, #50156, #81108, #11676, #4053, #96804, #89225, #14651, #5551, #28858, #7537, #99757, #84099, #91680, #76460, #30346, #52631, #61232, #84586, #29357, #29847, #92197, #69343, #76934, #45528, #68833, #53142, #14151, #91185, #21259, #28342, #15123, #38428, #21747, #60222, #75981, #83088, #90704, #67343, #22751, #46018, #75462, #7040, #44029, #45037, #6555, #53630, #59736, #52139, #98270, #98775, #60716, #22241, #59220, #90196, #20770, #51658, #83587, #37428, #82607, #37920, #13173, #74970, #68338, #67854, #6047, #13659, #36436, #44530, #36942, #99262, #48035, #9046, #32341, #25238, #17137, #24737, #63244, #94184, #31338, #47042, #87120, #46524, #77958, #61730, #71360, #39916, #8549, #62727, #100263, #48552, #86604, #62222, #70852, #63747, #93684, #56124, #55620, #32838, #54621, #47534, #40427, #94681, #78979, #69835, #1461, #9565, #17654, #79492, #38930, #93174, #10054, #1952, #40919, #39419, #86112, #78462, #30844, #92679, #77463, #447, #23231, #54119, #85078, #15625, #8057, #23726, #85604, #16143, #70337, #948, #31826, #24248, #55125, #16639, #58137, #12055, #96684, #57630, #34346, #64758, #12556, #58619, #81981, #65241, #3469, #10556, #66247, #51027, #41430, #88110, #89594, #41942, #3945, #95706, #88608, #50047, #97183, #2980, #33872, #72373, #72877, #34828, #65728, #42909, #27749, #96187, #26254, #71866, #81000, #33344, #57128, #20159, #18661, #27254, #11067, #49540, #80494, #2464, #26747, #19666, #56640, #50529, #11564, #89117, #64243, #19175, #81485, #42424, #95194, #73849, #4438, #73357, #35337, #25766, #87624, #18152, #49051, #79987, #5935, #43430, #92085, #29732, #5445, #83472, #6923, #60605, #97665, #91561, #59109, #43923, #82978, #99144, #13552, #52038, #13064, #52523, #22131, #99644, #22632, #82499, #74863, #37811, #45417, #44916, #44426, #90594, #53022, #68720, #53518, #83978, #66732, #21639, #36328, #84470, #4957, #14540, #76351, #6441, #51538, #30229, #67230, #61110, #14036, #74375, #35838, #20649, #98158, #28233, #28740, #59616, #37320, #21158, #75862, #75355, #36830, #67739, #98663, #29244, #60111, #91076, #68220, #78339, #38812, #17013, #46407, #39789, #16023, #55995, #7940, #69717, #62100, #70210, #62604, #324 ),
 .UNSPECIFIED., .F., .T. ) 
 B_SPLINE_CURVE_WITH_KNOTS ( ( 3, 2, 2, 2, 2, 2, 2, 2, 2, 2, 2, 2, 2, 2, 2, 2, 2, 2, 2, 2, 2, 2, 2, 2, 2, 2, 2, 2, 2, 2, 2, 2, 2, 2, 2, 2, 2, 2, 2, 2, 2, 2, 2, 2, 2, 2, 2, 2, 2, 2, 2, 2, 2, 2, 2, 2, 2, 2, 2, 2, 2, 2, 2, 2, 2, 2, 2, 2, 2, 2, 2, 2, 2, 2, 2, 2, 2, 2, 2, 2, 2, 2, 2, 2, 2, 2, 2, 2, 2, 2, 2, 2, 2, 2, 2, 2, 2, 2, 2, 2, 2, 2, 2, 2, 2, 2, 2, 2, 2, 2, 2, 2, 2, 2, 2, 2, 2, 2, 2, 2, 2, 2, 2, 2, 2, 2, 2, 2, 2, 2, 2, 2, 2, 2, 2, 2, 2, 2, 2, 2, 2, 2, 2, 2, 2, 2, 2, 2, 2, 2, 2, 2, 2, 2, 2, 2, 2, 2, 2, 2, 2, 2, 2, 2, 2, 2, 2, 2, 2, 2, 2, 2, 2, 2, 2, 2, 2, 2, 2, 2, 2, 2, 2, 2, 2, 2, 2, 2, 2, 2, 2, 2, 2, 2, 2, 2, 2, 2, 2, 2, 3 ),
 ( 0.000000000000000000, 0.005000000000000000104, 0.01000000000000000021, 0.01499999999999999944, 0.02000000000000000042, 0.02500000000000000139, 0.02999999999999999889, 0.03500000000000000333, 0.04000000000000000083, 0.04499999999999999833, 0.05000000000000000278, 0.05500000000000000028, 0.05999999999999999778, 0.06500000000000000222, 0.07000000000000000666, 0.07499999999999999722, 0.08000000000000000167, 0.08500000000000000611, 0.08999999999999999667, 0.09500000000000000111, 0.1000000000000000056, 0.1049999999999999961, 0.1100000000000000006, 0.1150000000000000050, 0.1199999999999999956, 0.1250000000000000000, 0.1300000000000000044, 0.1350000000000000089, 0.1400000000000000133, 0.1449999999999999900, 0.1499999999999999944, 0.1549999999999999989, 0.1600000000000000033, 0.1650000000000000078, 0.1700000000000000122, 0.1749999999999999889, 0.1799999999999999933, 0.1849999999999999978, 0.1900000000000000022, 0.1950000000000000067, 0.2000000000000000111, 0.2049999999999999878, 0.2099999999999999922, 0.2149999999999999967, 0.2200000000000000011, 0.2250000000000000056, 0.2300000000000000100, 0.2349999999999999867, 0.2399999999999999911, 0.2449999999999999956, 0.2500000000000000000, 0.2550000000000000044, 0.2600000000000000089, 0.2650000000000000133, 0.2700000000000000178, 0.2750000000000000222, 0.2800000000000000266, 0.2849999999999999756, 0.2899999999999999800, 0.2949999999999999845, 0.2999999999999999889, 0.3049999999999999933, 0.3099999999999999978, 0.3150000000000000022, 0.3200000000000000067, 0.3250000000000000111, 0.3300000000000000155, 0.3350000000000000200, 0.3400000000000000244, 0.3449999999999999734, 0.3499999999999999778, 0.3549999999999999822, 0.3599999999999999867, 0.3649999999999999911, 0.3699999999999999956, 0.3750000000000000000, 0.3800000000000000044, 0.3850000000000000089, 0.3900000000000000133, 0.3950000000000000178, 0.4000000000000000222, 0.4050000000000000266, 0.4099999999999999756, 0.4149999999999999800, 0.4199999999999999845, 0.4249999999999999889, 0.4299999999999999933, 0.4349999999999999978, 0.4400000000000000022, 0.4450000000000000067, 0.4500000000000000111, 0.4550000000000000155, 0.4600000000000000200, 0.4650000000000000244, 0.4699999999999999734, 0.4749999999999999778, 0.4799999999999999822, 0.4849999999999999867, 0.4899999999999999911, 0.4949999999999999956, 0.5000000000000000000, 0.5050000000000000044, 0.5100000000000000089, 0.5150000000000000133, 0.5200000000000000178, 0.5250000000000000222, 0.5300000000000000266, 0.5350000000000000311, 0.5400000000000000355, 0.5450000000000000400, 0.5500000000000000444, 0.5550000000000000488, 0.5600000000000000533, 0.5649999999999999467, 0.5699999999999999512, 0.5749999999999999556, 0.5799999999999999600, 0.5849999999999999645, 0.5899999999999999689, 0.5949999999999999734, 0.5999999999999999778, 0.6049999999999999822, 0.6099999999999999867, 0.6149999999999999911, 0.6199999999999999956, 0.6250000000000000000, 0.6300000000000000044, 0.6350000000000000089, 0.6400000000000000133, 0.6450000000000000178, 0.6500000000000000222, 0.6550000000000000266, 0.6600000000000000311, 0.6650000000000000355, 0.6700000000000000400, 0.6750000000000000444, 0.6800000000000000488, 0.6850000000000000533, 0.6899999999999999467, 0.6949999999999999512, 0.6999999999999999556, 0.7049999999999999600, 0.7099999999999999645, 0.7149999999999999689, 0.7199999999999999734, 0.7249999999999999778, 0.7299999999999999822, 0.7349999999999999867, 0.7399999999999999911, 0.7449999999999999956, 0.7500000000000000000, 0.7550000000000000044, 0.7600000000000000089, 0.7650000000000000133, 0.7700000000000000178, 0.7750000000000000222, 0.7800000000000000266, 0.7850000000000000311, 0.7900000000000000355, 0.7950000000000000400, 0.8000000000000000444, 0.8050000000000000488, 0.8100000000000000533, 0.8149999999999999467, 0.8199999999999999512, 0.8249999999999999556, 0.8299999999999999600, 0.8349999999999999645, 0.8399999999999999689, 0.8449999999999999734, 0.8499999999999999778, 0.8549999999999999822, 0.8599999999999999867, 0.8649999999999999911, 0.8699999999999999956, 0.8750000000000000000, 0.8800000000000000044, 0.8850000000000000089, 0.8900000000000000133, 0.8950000000000000178, 0.9000000000000000222, 0.9050000000000000266, 0.9100000000000000311, 0.9150000000000000355, 0.9200000000000000400, 0.9250000000000000444, 0.9300000000000000488, 0.9350000000000000533, 0.9399999999999999467, 0.9449999999999999512, 0.9499999999999999556, 0.9549999999999999600, 0.9599999999999999645, 0.9649999999999999689, 0.9699999999999999734, 0.9749999999999999778, 0.9799999999999999822, 0.9849999999999999867, 0.9899999999999999911, 0.9949999999999999956, 1.000000000000000000 ),
 .UNSPECIFIED. ) 
 CURVE ( )  GEOMETRIC_REPRESENTATION_ITEM ( )  RATIONAL_B_SPLINE_CURVE ( ( 1.000000000000000000, 0.9510565162951535312, 1.000000000000000000, 0.9510565162951535312, 1.000000000000000000, 0.9510565162951535312, 1.000000000000000000, 0.9510565162951535312, 1.000000000000000000, 0.9510565162951535312, 1.000000000000000000, 0.9510565162951535312, 1.000000000000000000, 0.9510565162951535312, 1.000000000000000000, 0.9510565162951535312, 1.000000000000000000, 0.9510565162951535312, 1.000000000000000000, 0.9510565162951535312, 1.000000000000000000, 0.9510565162951535312, 1.000000000000000000, 0.9510565162951535312, 1.000000000000000000, 0.9510565162951535312, 1.000000000000000000, 0.9510565162951535312, 1.000000000000000000, 0.9510565162951535312, 1.000000000000000000, 0.9510565162951535312, 1.000000000000000000, 0.9510565162951535312, 1.000000000000000000, 0.9510565162951535312, 1.000000000000000000, 0.9510565162951535312, 1.000000000000000000, 0.9510565162951535312, 1.000000000000000000, 0.9510565162951535312, 1.000000000000000000, 0.9510565162951535312, 1.000000000000000000, 0.9510565162951535312, 1.000000000000000000, 0.9510565162951535312, 1.000000000000000000, 0.9510565162951535312, 1.000000000000000000, 0.9510565162951535312, 1.000000000000000000, 0.9510565162951535312, 1.000000000000000000, 0.9510565162951535312, 1.000000000000000000, 0.9510565162951535312, 1.000000000000000000, 0.9510565162951535312, 1.000000000000000000, 0.9510565162951535312, 1.000000000000000000, 0.9510565162951535312, 1.000000000000000000, 0.9510565162951535312, 1.000000000000000000, 0.9510565162951535312, 1.000000000000000000, 0.9510565162951535312, 1.000000000000000000, 0.9510565162951535312, 1.000000000000000000, 0.9510565162951535312, 1.000000000000000000, 0.9510565162951535312, 1.000000000000000000, 0.9510565162951535312, 1.000000000000000000, 0.9510565162951535312, 1.000000000000000000, 0.9510565162951535312, 1.000000000000000000, 0.9510565162951535312, 1.000000000000000000, 0.9510565162951535312, 1.000000000000000000, 0.9510565162951535312, 1.000000000000000000, 0.9510565162951535312, 1.000000000000000000, 0.9510565162951535312, 1.000000000000000000, 0.9510565162951535312, 1.000000000000000000, 0.9510565162951535312, 1.000000000000000000, 0.9510565162951535312, 1.000000000000000000, 0.9510565162951535312, 1.000000000000000000, 0.9510565162951535312, 1.000000000000000000, 0.9510565162951535312, 1.000000000000000000, 0.9510565162951535312, 1.000000000000000000, 0.9510565162951535312, 1.000000000000000000, 0.9510565162951535312, 1.000000000000000000, 0.9510565162951535312, 1.000000000000000000, 0.9510565162951535312, 1.000000000000000000, 0.9510565162951535312, 1.000000000000000000, 0.9510565162951535312, 1.000000000000000000, 0.9510565162951535312, 1.000000000000000000, 0.9510565162951535312, 1.000000000000000000, 0.9510565162951535312, 1.000000000000000000, 0.9510565162951535312, 1.000000000000000000, 0.9510565162951535312, 1.000000000000000000, 0.9510565162951535312, 1.000000000000000000, 0.9510565162951535312, 1.000000000000000000, 0.9510565162951535312, 1.000000000000000000, 0.9510565162951535312, 1.000000000000000000, 0.9510565162951535312, 1.000000000000000000, 0.9510565162951535312, 1.000000000000000000, 0.9510565162951535312, 1.000000000000000000, 0.9510565162951535312, 1.000000000000000000, 0.9510565162951535312, 1.000000000000000000, 0.9510565162951535312, 1.000000000000000000, 0.9510565162951535312, 1.000000000000000000, 0.9510565162951535312, 1.000000000000000000, 0.9510565162951535312, 1.000000000000000000, 0.9510565162951535312, 1.000000000000000000, 0.9510565162951535312, 1.000000000000000000, 0.9510565162951535312, 1.000000000000000000, 0.9510565162951535312, 1.000000000000000000, 0.9510565162951535312, 1.000000000000000000, 0.9510565162951535312, 1.000000000000000000, 0.9510565162951535312, 1.000000000000000000, 0.9510565162951535312, 1.000000000000000000, 0.9510565162951535312, 1.000000000000000000, 0.9510565162951535312, 1.000000000000000000, 0.9510565162951535312, 1.000000000000000000, 0.9510565162951535312, 1.000000000000000000, 0.9510565162951535312, 1.000000000000000000, 0.9510565162951535312, 1.000000000000000000, 0.9510565162951535312, 1.000000000000000000, 0.9510565162951535312, 1.000000000000000000, 0.9510565162951535312, 1.000000000000000000, 0.9510565162951535312, 1.000000000000000000, 0.9510565162951535312, 1.000000000000000000, 0.9510565162951535312, 1.000000000000000000, 0.9510565162951535312, 1.000000000000000000, 0.9510565162951535312, 1.000000000000000000, 0.9510565162951535312, 1.000000000000000000, 0.9510565162951535312, 1.000000000000000000, 0.9510565162951535312, 1.000000000000000000, 0.9510565162951535312, 1.000000000000000000, 0.9510565162951535312, 1.000000000000000000, 0.9510565162951535312, 1.000000000000000000, 0.9510565162951535312, 1.000000000000000000, 0.9510565162951535312, 1.000000000000000000, 0.9510565162951535312, 1.000000000000000000, 0.9510565162951535312, 1.000000000000000000, 0.9510565162951535312, 1.000000000000000000, 0.9510565162951535312, 1.000000000000000000, 0.9510565162951535312, 1.000000000000000000, 0.9510565162951535312, 1.000000000000000000, 0.9510565162951535312, 1.000000000000000000, 0.9510565162951535312, 1.000000000000000000, 0.9510565162951535312, 1.000000000000000000, 0.9510565162951535312, 1.000000000000000000, 0.9510565162951535312, 1.000000000000000000, 0.9510565162951535312, 1.000000000000000000, 0.9510565162951535312, 1.000000000000000000, 0.9510565162951535312, 1.000000000000000000, 0.9510565162951535312, 1.000000000000000000, 0.9510565162951535312, 1.000000000000000000, 0.9510565162951535312, 1.000000000000000000, 0.9510565162951535312, 1.000000000000000000, 0.9510565162951535312, 1.000000000000000000, 0.9510565162951535312, 1.000000000000000000, 0.9510565162951535312, 1.000000000000000000, 0.9510565162951535312, 1.000000000000000000, 0.9510565162951535312, 1.000000000000000000, 0.9510565162951535312, 1.000000000000000000, 0.9510565162951535312, 1.000000000000000000, 0.9510565162951535312, 1.000000000000000000, 0.9510565162951535312, 1.000000000000000000, 0.9510565162951535312, 1.000000000000000000, 0.9510565162951535312, 1.000000000000000000, 0.9510565162951535312, 1.000000000000000000, 0.9510565162951535312, 1.000000000000000000, 0.9510565162951535312, 1.000000000000000000, 0.9510565162951535312, 1.000000000000000000, 0.9510565162951535312, 1.000000000000000000, 0.9510565162951535312, 1.000000000000000000, 0.9510565162951535312, 1.000000000000000000, 0.9510565162951535312, 1.000000000000000000, 0.9510565162951535312, 1.000000000000000000, 0.9510565162951535312, 1.000000000000000000, 0.9510565162951535312, 1.000000000000000000, 0.9510565162951535312, 1.000000000000000000, 0.9510565162951535312, 1.000000000000000000, 0.9510565162951535312, 1.000000000000000000, 0.9510565162951535312, 1.000000000000000000, 0.9510565162951535312, 1.000000000000000000, 0.9510565162951535312, 1.000000000000000000, 0.9510565162951535312, 1.000000000000000000, 0.9510565162951535312, 1.000000000000000000, 0.9510565162951535312, 1.000000000000000000, 0.9510565162951535312, 1.000000000000000000, 0.9510565162951535312, 1.000000000000000000, 0.9510565162951535312, 1.000000000000000000, 0.9510565162951535312, 1.000000000000000000, 0.9510565162951535312, 1.000000000000000000, 0.9510565162951535312, 1.000000000000000000, 0.9510565162951535312, 1.000000000000000000, 0.9510565162951535312, 1.000000000000000000, 0.9510565162951535312, 1.000000000000000000, 0.9510565162951535312, 1.000000000000000000, 0.9510565162951535312, 1.000000000000000000, 0.9510565162951535312, 1.000000000000000000, 0.9510565162951535312, 1.000000000000000000, 0.9510565162951535312, 1.000000000000000000, 0.9510565162951535312, 1.000000000000000000, 0.9510565162951535312, 1.000000000000000000, 0.9510565162951535312, 1.000000000000000000, 0.9510565162951535312, 1.000000000000000000, 0.9510565162951535312, 1.000000000000000000, 0.9510565162951535312, 1.000000000000000000, 0.9510565162951535312, 1.000000000000000000, 0.9510565162951535312, 1.000000000000000000, 0.9510565162951535312, 1.000000000000000000, 0.9510565162951535312, 1.000000000000000000, 0.9510565162951535312, 1.000000000000000000, 0.9510565162951535312, 1.000000000000000000, 0.9510565162951535312, 1.000000000000000000, 0.9510565162951535312, 1.000000000000000000, 0.9510565162951535312, 1.000000000000000000, 0.9510565162951535312, 1.000000000000000000, 0.9510565162951535312, 1.000000000000000000, 0.9510565162951535312, 1.000000000000000000, 0.9510565162951535312, 1.000000000000000000, 0.9510565162951535312, 1.000000000000000000, 0.9510565162951535312, 1.000000000000000000, 0.9510565162951535312, 1.000000000000000000, 0.9510565162951535312, 1.000000000000000000, 0.9510565162951535312, 1.000000000000000000, 0.9510565162951535312, 1.000000000000000000, 0.9510565162951535312, 1.000000000000000000, 0.9510565162951535312, 1.000000000000000000, 0.9510565162951535312, 1.000000000000000000, 0.9510565162951535312, 1.000000000000000000, 0.9510565162951535312, 1.000000000000000000 ) ) 
 REPRESENTATION_ITEM ( '' )  );
#85763=EDGE_LOOP ( 'NONE', ( #28139, #38815, #87745, #25931 ) ) ;
#85774=CARTESIAN_POINT ( 'NONE',  ( 69.95426054967219898, 67.58280296741347115, 9.346954025415000089 ) ) ;
#85779=CARTESIAN_POINT ( 'NONE',  ( 78.51983995760878088, 47.43908030793226516, 14.25121724663956790 ) ) ;
#85783=CARTESIAN_POINT ( 'NONE',  ( 82.30608073536585323, 41.08216667689982415, -2.629353525907028644 ) ) ;
#85784=CARTESIAN_POINT ( 'NONE',  ( 87.53367671268780725, 44.88112536278567433, -6.578546970659244764 ) ) ;
#85791=CARTESIAN_POINT ( 'NONE',  ( 72.39889165046784569, 71.58181683135407525, 5.112090114424422183 ) ) ;
#85794=ADVANCED_FACE ( 'NONE', ( #14552 ), #61121, .T. ) ;
#85799=LINE ( 'NONE', #10241, #17468 ) ;
#85802=CARTESIAN_POINT ( 'NONE',  ( 85.55409210693744626, 48.30986647782642507, -11.71318688851061651 ) ) ;
#85804=CARTESIAN_POINT ( 'NONE',  ( 70.76613391576567835, 62.53219004156024141, 13.77722632876776920 ) ) ;
#85805=CARTESIAN_POINT ( 'NONE',  ( 79.58936028502597537, 59.22294857574252802, 16.56770033466462166 ) ) ;
#85815=B_SPLINE_SURFACE_WITH_KNOTS ( 'NONE', 3, 1, ( 
 ( #28978, #59854 ),
 ( #90817, #21370 ),
 ( #52256, #83198 ),
 ( #46132, #8160 ),
 ( #13761, #14755 ),
 ( #6161, #60832 ),
 ( #15739, #85195 ),
 ( #45637, #37057 ),
 ( #44640, #38544 ),
 ( #14262, #21859 ),
 ( #84209, #53736 ),
 ( #46647, #61839 ),
 ( #68943, #30454 ),
 ( #38033, #76565 ),
 ( #62335, #31441 ),
 ( #29462, #67964 ),
 ( #75574, #77572 ),
 ( #69451, #98882 ),
 ( #77045, #52741 ),
 ( #7146, #60337 ),
 ( #91294, #67 ),
 ( #39033, #6666 ),
 ( #83703, #45153 ),
 ( #76092, #37543 ),
 ( #22357, #68449 ),
 ( #99377, #29956 ),
 ( #30950, #91792 ),
 ( #53254, #61344 ),
 ( #92303, #93286 ),
 ( #22852, #84695 ),
 ( #7653, #92786 ) ),
 .UNSPECIFIED., .F., .F., .F.,
 ( 4, 3, 3, 3, 3, 3, 3, 3, 3, 3, 4 ),
 ( 2, 2 ),
 ( 0.000000000000000000, 0.1122669598086816489, 0.2243161639709700117, 0.3396355846219164532, 0.4553962076585098551, 0.5677860799922355151, 0.6749047109689640944, 0.7773884377078206231, 0.8775581155834345504, 0.9782364162378064387, 1.000000000000000000 ),
 ( 0.000000000000000000, 1.000000000000000000 ),
 .UNSPECIFIED. ) ;
#85819=CARTESIAN_POINT ( 'NONE',  ( 88.04376564059177213, 44.77267915597603576, 4.588252583283844999 ) ) ;
#85821=CARTESIAN_POINT ( 'NONE',  ( 11.19180257851625448, 22.16454794089040092, -10.00000000000000355 ) ) ;
#85824=CARTESIAN_POINT ( 'NONE',  ( 73.97544314932677878, 54.88016228234857152, -16.13337635542186277 ) ) ;
#85830=CARTESIAN_POINT ( 'NONE',  ( 71.12491932460929434, 69.18585904456776348, 8.936385494539548446 ) ) ;
#85831=CARTESIAN_POINT ( 'NONE',  ( 8.916318567990060728, 28.08080186712591342, -3.090169943749475845 ) ) ;
#85838=CARTESIAN_POINT ( 'NONE',  ( 35.02453322635827959, 23.14754757982091959, -5.678558825948276656 ) ) ;
#85844=CARTESIAN_POINT ( 'NONE',  ( 87.98804127167099409, 43.77408088403166175, 2.388364124389108945 ) ) ;
#85846=CARTESIAN_POINT ( 'NONE',  ( 65.86157430945659996, 69.00948543913943922, 2.025254867008428050 ) ) ;
#85851=CARTESIAN_POINT ( 'NONE',  ( 6.742211794378569323, 25.93396525600388003, 2.839279412974139660 ) ) ;
#85861=ORIENTED_EDGE ( 'NONE', *, *, #77637, .F. ) ;
#85865=ORIENTED_EDGE ( 'NONE', *, *, #12703, .T. ) ;
#85866=CARTESIAN_POINT ( 'NONE',  ( 68.45344762042827824, 64.57392882346940155, 12.12708197196866600 ) ) ;
#85870=CARTESIAN_POINT ( 'NONE',  ( 68.69482932751195392, 64.02698956824444565, -12.02621948774222993 ) ) ;
#85873=CARTESIAN_POINT ( 'NONE',  ( 69.96429914230955660, 62.67588759707778934, 13.42142011397352874 ) ) ;
#85877=CARTESIAN_POINT ( 'NONE',  ( 66.34774863042578374, 68.89465645501611846, 3.924861168553110513 ) ) ;
#85878=CARTESIAN_POINT ( 'NONE',  ( 29.54281338067077911, 40.55466486950702176, -1.111400068045478839E-16 ) ) ;
#85882=CARTESIAN_POINT ( 'NONE',  ( 80.25311165466112584, 46.21449285432851184, 12.30778873727355638 ) ) ;
#85884=FACE_OUTER_BOUND ( 'NONE', #30725, .T. ) ;
#85885=AXIS2_PLACEMENT_3D ( 'NONE', #38984, #9102, #94237 ) ;
#85888=DIRECTION ( 'NONE',  ( 0.5000000000000014433, -0.8660254037844378194, 0.000000000000000000 ) ) ;
#85893=CARTESIAN_POINT ( 'NONE',  ( 82.61614429202859355, 53.50419195261176242, -15.73127852458025622 ) ) ;
#85896=CARTESIAN_POINT ( 'NONE',  ( 26.78885238572174998, 16.26216523072495690, -2.296566073217252530E-15 ) ) ;
#85905=CARTESIAN_POINT ( 'NONE',  ( 83.71006973597178558, 45.75904905664672384, -10.17439447765971039 ) ) ;
#85919=CARTESIAN_POINT ( 'NONE',  ( 75.64192366613818308, 65.38353595949358521, 14.29496885373930581 ) ) ;
#85927=FACE_OUTER_BOUND ( 'NONE', #44749, .T. ) ;
#85929=CARTESIAN_POINT ( 'NONE',  ( 84.92266591929319475, 45.12665518879106941, 8.618535221689526793 ) ) ;
#85932=CARTESIAN_POINT ( 'NONE',  ( 74.34814666111280701, 67.93757562633051350, -11.69177540040551655 ) ) ;
#85942=CARTESIAN_POINT ( 'NONE',  ( 77.22649460905378760, 63.31555197798695644, 15.15381191669832184 ) ) ;
#85947=CARTESIAN_POINT ( 'NONE',  ( 71.43092631454221930, 71.71198063924084920, 2.470412517165702759 ) ) ;
#85951=CARTESIAN_POINT ( 'NONE',  ( 74.93919869194499483, 61.43846615714554815, 15.72264986953730492 ) ) ;
#85956=CARTESIAN_POINT ( 'NONE',  ( 13.18987451683679524, 19.56628583063839244, 9.188101187500006262 ) ) ;
#85965=CARTESIAN_POINT ( 'NONE',  ( 74.83655476910676896, 53.51806293180212037, 16.54630480343736920 ) ) ;
#85971=CARTESIAN_POINT ( 'NONE',  ( 81.67261577379798609, 49.77584566285921852, 14.52435489019822690 ) ) ;
#85976=CARTESIAN_POINT ( 'NONE',  ( 81.37674444193763179, 55.19836804271280783, -15.94010240901345199 ) ) ;
#85979=CARTESIAN_POINT ( 'NONE',  ( 73.62250635243425734, 69.55784274833358438, 10.23584637956793308 ) ) ;
#85980=CARTESIAN_POINT ( 'NONE',  ( 39.54951596113196644, 25.76004757982093096, 5.678558825948272215 ) ) ;
#85982=CARTESIAN_POINT ( 'NONE',  ( 78.44203751522358914, 61.21016990572090322, 16.24725970467587643 ) ) ;
#85986=CARTESIAN_POINT ( 'NONE',  ( 86.40472769894839189, 47.00022269315729773, -10.52150423465797502 ) ) ;
#85990=ADVANCED_FACE ( 'NONE', ( #92332 ), #84726, .T. ) ;
#85992=CARTESIAN_POINT ( 'NONE',  ( 80.90512323705502240, 45.42831638329423072, -12.03671141704919556 ) ) ;
#85998=CARTESIAN_POINT ( 'NONE',  ( 77.20442761108157015, 49.22956228998022965, -15.35833876822225186 ) ) ;
#86000=VERTEX_POINT ( 'NONE', #40569 ) ;
#86001=CARTESIAN_POINT ( 'NONE',  ( 87.02439212704567240, 45.81336919377327632, -8.633490303204487404 ) ) ;
#86002=CARTESIAN_POINT ( 'NONE',  ( 79.30460723929135725, 53.73768979410964164, 15.82503211290379674 ) ) ;
#86008=CARTESIAN_POINT ( 'NONE',  ( 82.67120877686448921, 40.53284241866003867, 0.8934199165528524667 ) ) ;
#86010=EDGE_CURVE ( 'NONE', #54888, #95476, #17801, .T. ) ;
#86015=CARTESIAN_POINT ( 'NONE',  ( 34.13026518906141860, 41.74646525600392977, 2.839279412974139660 ) ) ;
#86017=CARTESIAN_POINT ( 'NONE',  ( 85.57852021786813168, 48.96074862228688573, -12.66870494374460066 ) ) ;
#86018=ORIENTED_EDGE ( 'NONE', *, *, #46900, .T. ) ;
#86023=CARTESIAN_POINT ( 'NONE',  ( 73.29586284545086983, 66.59957193289693578, 12.21858630789641076 ) ) ;
#86025=CARTESIAN_POINT ( 'NONE',  ( 79.26867134682716198, 56.64247672455211102, 16.58182463307725385 ) ) ;
#86032=ORIENTED_EDGE ( 'NONE', *, *, #20114, .F. ) ;
#86038=CARTESIAN_POINT ( 'NONE',  ( 71.64316818921395225, 72.05741665177615118, -3.509880912999884917 ) ) ;
#86042=ORIENTED_EDGE ( 'NONE', *, *, #49194, .F. ) ;
#86044=CARTESIAN_POINT ( 'NONE',  ( 73.10296688250903685, 63.30412816941502285, 14.61027101223241864 ) ) ;
#86051=CARTESIAN_POINT ( 'NONE',  ( 74.28707621773548908, 68.55768173149772338, 11.60544092197707755 ) ) ;
#86052=( BOUNDED_CURVE ( )  B_SPLINE_CURVE ( 2, ( #83324, #75701, #4812, #35694, #30081, #51897, #45276, #6288, #37181, #68081, #14392, #43777, #99003, #60968, #74722, #66594, #84327, #16874, #76685, #54351, #55847, #45762, #70063, #84819, #39150, #32583, #38155, #63480, #40160, #78698, #8780, #9285, #681, #15357, #32065, #31562, #47270, #100000, #62453, #7782, #16379, #54870, #46253, #69073, #30583, #23461, #85851, #61471, #71101, #85324, #1700, #77177, #93420, #94417, #22969, #47759, #24970, #23971, #92419, #78192, #86842, #39650, #70571, #1189, #7273, #38672, #62976, #53856, #69575, #93924, #24478, #55359, #183, #31066, #61957, #92909, #86337, #15869, #46778, #77701, #8284, #88846, #50268, #49286, #40664, #95930, #17377, #73102, #3694, #95444, #48795, #72609, #87851, #57367, #72097, #34573, #88341, #49777, #25996, #87368, #18391, #18898, #80222, #17898, #80734, #73586, #56867, #25479, #10790, #81221, #4166, #79726, #34096, #96922, #3211, #56371, #11308, #79231, #41664, #64986, #9804, #26490, #10288, #65474, #42166, #96416, #71601, #26983, #41160, #57867, #19409, #11797, #27490, #42652, #2697, #35063, #2197, #65970, #58359, #48286, #33080, #63973, #94916, #64484, #33588, #13628, #76904, #38399, #30316, #85047, #60689, #14621, #68802, #15096, #36909, #99729, #92650, #75431, #61203, #92170, #45500, #90673, #44502, #43996, #45002, #6015, #36406, #91151, #21229, #45987, #7501, #69312, #75948, #67310, #22214, #74938, #22720, #53599, #21716, #67822, #99229, #91647, #29815, #52600, #61698, #83557, #53111, #84068, #76433, #7008, #37893, #6524, #98744, #84557, #100234, #14121, #52108, #37400, #30818, #23200, #29324, #68306, #54091, #83055, #98238, #5522, #28824, #60190, #59707, #38901, #56610, #55589, #69805, #39885, #9013, #17105, #15594, #77430, #71836, #77928, #87084, #17620, #25207, #94153, #70820, #24218, #95162, #86085, #86572, #39388, #415, #23693, #1429, #31304, #33312, #46494, #32310, #54589, #63211, #2434, #8029, #62192, #93143, #16609, #85571, #16115, #93653, #47013, #48000, #8519, #55098, #62696, #71331, #70305, #918, #31794, #47505, #78432, #24706, #78945, #9533, #40394, #1923, #32809, #63714, #94652, #56090, #48524, #79461, #10025, #40887, #64211, #25730, #34797, #73327, #34313, #4927, #65211, #65699, #96653, #27223, #80461, #89088, #57598, #88578, #49022, #58106, #41909, #66215, #58588, #42879, #96153, #66700, #19140, #20123, #64724, #10523, #73815, #26716, #11032, #72844, #50014, #3436, #80968, #28200, #50995, #26220, #18629, #49507, #11533, #74338, #42393, #35303, #81946, #97154, #19637, #50497, #81451, #97635, #12023, #4407, #43395, #12524, #18120, #27720, #87594, #35806, #79955, #41398, #2947, #72341, #33836, #95673, #20619, #98633, #91045, #51503, #29215, #6412, #83440, #82470, #60578, #13032, #14007, #21129, #29701, #99119, #99618, #69189, #53487, #13522, #30196, #43894, #44885, #60082, #75826, #21612, #61082, #7388, #76795, #5904, #84439, #68190, #74834, #91534, #38278, #5414, #22098, #92053, #83945, #36297, #52492, #14507, #67200, #45390, #76320, #6895, #98122, #82949, #28706, #59076, #52006, #37784, #68686, #22599, #100118, #14984, #44390, #45871, #59584, #90047, #90560, #75325, #36794, #67706, #79347, #48400, #77817, #47387, #294, #63591 ),
 .UNSPECIFIED., .F., .T. ) 
 B_SPLINE_CURVE_WITH_KNOTS ( ( 3, 2, 2, 2, 2, 2, 2, 2, 2, 2, 2, 2, 2, 2, 2, 2, 2, 2, 2, 2, 2, 2, 2, 2, 2, 2, 2, 2, 2, 2, 2, 2, 2, 2, 2, 2, 2, 2, 2, 2, 2, 2, 2, 2, 2, 2, 2, 2, 2, 2, 2, 2, 2, 2, 2, 2, 2, 2, 2, 2, 2, 2, 2, 2, 2, 2, 2, 2, 2, 2, 2, 2, 2, 2, 2, 2, 2, 2, 2, 2, 2, 2, 2, 2, 2, 2, 2, 2, 2, 2, 2, 2, 2, 2, 2, 2, 2, 2, 2, 2, 2, 2, 2, 2, 2, 2, 2, 2, 2, 2, 2, 2, 2, 2, 2, 2, 2, 2, 2, 2, 2, 2, 2, 2, 2, 2, 2, 2, 2, 2, 2, 2, 2, 2, 2, 2, 2, 2, 2, 2, 2, 2, 2, 2, 2, 2, 2, 2, 2, 2, 2, 2, 2, 2, 2, 2, 2, 2, 2, 2, 2, 2, 2, 2, 2, 2, 2, 2, 2, 2, 2, 2, 2, 2, 2, 2, 2, 2, 2, 2, 2, 2, 2, 2, 2, 2, 2, 2, 2, 2, 2, 2, 2, 2, 2, 2, 2, 2, 2, 2, 3 ),
 ( 0.000000000000000000, 0.005000000000000000104, 0.01000000000000000021, 0.01499999999999999944, 0.02000000000000000042, 0.02500000000000000139, 0.02999999999999999889, 0.03500000000000000333, 0.04000000000000000083, 0.04499999999999999833, 0.05000000000000000278, 0.05500000000000000028, 0.05999999999999999778, 0.06500000000000000222, 0.07000000000000000666, 0.07499999999999999722, 0.08000000000000000167, 0.08500000000000000611, 0.08999999999999999667, 0.09500000000000000111, 0.1000000000000000056, 0.1049999999999999961, 0.1100000000000000006, 0.1150000000000000050, 0.1199999999999999956, 0.1250000000000000000, 0.1300000000000000044, 0.1350000000000000089, 0.1400000000000000133, 0.1449999999999999900, 0.1499999999999999944, 0.1549999999999999989, 0.1600000000000000033, 0.1650000000000000078, 0.1700000000000000122, 0.1749999999999999889, 0.1799999999999999933, 0.1849999999999999978, 0.1900000000000000022, 0.1950000000000000067, 0.2000000000000000111, 0.2049999999999999878, 0.2099999999999999922, 0.2149999999999999967, 0.2200000000000000011, 0.2250000000000000056, 0.2300000000000000100, 0.2349999999999999867, 0.2399999999999999911, 0.2449999999999999956, 0.2500000000000000000, 0.2550000000000000044, 0.2600000000000000089, 0.2650000000000000133, 0.2700000000000000178, 0.2750000000000000222, 0.2800000000000000266, 0.2849999999999999756, 0.2899999999999999800, 0.2949999999999999845, 0.2999999999999999889, 0.3049999999999999933, 0.3099999999999999978, 0.3150000000000000022, 0.3200000000000000067, 0.3250000000000000111, 0.3300000000000000155, 0.3350000000000000200, 0.3400000000000000244, 0.3449999999999999734, 0.3499999999999999778, 0.3549999999999999822, 0.3599999999999999867, 0.3649999999999999911, 0.3699999999999999956, 0.3750000000000000000, 0.3800000000000000044, 0.3850000000000000089, 0.3900000000000000133, 0.3950000000000000178, 0.4000000000000000222, 0.4050000000000000266, 0.4099999999999999756, 0.4149999999999999800, 0.4199999999999999845, 0.4249999999999999889, 0.4299999999999999933, 0.4349999999999999978, 0.4400000000000000022, 0.4450000000000000067, 0.4500000000000000111, 0.4550000000000000155, 0.4600000000000000200, 0.4650000000000000244, 0.4699999999999999734, 0.4749999999999999778, 0.4799999999999999822, 0.4849999999999999867, 0.4899999999999999911, 0.4949999999999999956, 0.5000000000000000000, 0.5050000000000000044, 0.5100000000000000089, 0.5150000000000000133, 0.5200000000000000178, 0.5250000000000000222, 0.5300000000000000266, 0.5350000000000000311, 0.5400000000000000355, 0.5450000000000000400, 0.5500000000000000444, 0.5550000000000000488, 0.5600000000000000533, 0.5649999999999999467, 0.5699999999999999512, 0.5749999999999999556, 0.5799999999999999600, 0.5849999999999999645, 0.5899999999999999689, 0.5949999999999999734, 0.5999999999999999778, 0.6049999999999999822, 0.6099999999999999867, 0.6149999999999999911, 0.6199999999999999956, 0.6250000000000000000, 0.6300000000000000044, 0.6350000000000000089, 0.6400000000000000133, 0.6450000000000000178, 0.6500000000000000222, 0.6550000000000000266, 0.6600000000000000311, 0.6650000000000000355, 0.6700000000000000400, 0.6750000000000000444, 0.6800000000000000488, 0.6850000000000000533, 0.6899999999999999467, 0.6949999999999999512, 0.6999999999999999556, 0.7049999999999999600, 0.7099999999999999645, 0.7149999999999999689, 0.7199999999999999734, 0.7249999999999999778, 0.7299999999999999822, 0.7349999999999999867, 0.7399999999999999911, 0.7449999999999999956, 0.7500000000000000000, 0.7550000000000000044, 0.7600000000000000089, 0.7650000000000000133, 0.7700000000000000178, 0.7750000000000000222, 0.7800000000000000266, 0.7850000000000000311, 0.7900000000000000355, 0.7950000000000000400, 0.8000000000000000444, 0.8050000000000000488, 0.8100000000000000533, 0.8149999999999999467, 0.8199999999999999512, 0.8249999999999999556, 0.8299999999999999600, 0.8349999999999999645, 0.8399999999999999689, 0.8449999999999999734, 0.8499999999999999778, 0.8549999999999999822, 0.8599999999999999867, 0.8649999999999999911, 0.8699999999999999956, 0.8750000000000000000, 0.8800000000000000044, 0.8850000000000000089, 0.8900000000000000133, 0.8950000000000000178, 0.9000000000000000222, 0.9050000000000000266, 0.9100000000000000311, 0.9150000000000000355, 0.9200000000000000400, 0.9250000000000000444, 0.9300000000000000488, 0.9350000000000000533, 0.9399999999999999467, 0.9449999999999999512, 0.9499999999999999556, 0.9549999999999999600, 0.9599999999999999645, 0.9649999999999999689, 0.9699999999999999734, 0.9749999999999999778, 0.9799999999999999822, 0.9849999999999999867, 0.9899999999999999911, 0.9949999999999999956, 1.000000000000000000 ),
 .UNSPECIFIED. ) 
 CURVE ( )  GEOMETRIC_REPRESENTATION_ITEM ( )  RATIONAL_B_SPLINE_CURVE ( ( 1.000000000000000000, 0.9510565162951535312, 1.000000000000000000, 0.9510565162951535312, 1.000000000000000000, 0.9510565162951535312, 1.000000000000000000, 0.9510565162951535312, 1.000000000000000000, 0.9510565162951535312, 1.000000000000000000, 0.9510565162951535312, 1.000000000000000000, 0.9510565162951535312, 1.000000000000000000, 0.9510565162951535312, 1.000000000000000000, 0.9510565162951535312, 1.000000000000000000, 0.9510565162951535312, 1.000000000000000000, 0.9510565162951535312, 1.000000000000000000, 0.9510565162951535312, 1.000000000000000000, 0.9510565162951535312, 1.000000000000000000, 0.9510565162951535312, 1.000000000000000000, 0.9510565162951535312, 1.000000000000000000, 0.9510565162951535312, 1.000000000000000000, 0.9510565162951535312, 1.000000000000000000, 0.9510565162951535312, 1.000000000000000000, 0.9510565162951535312, 1.000000000000000000, 0.9510565162951535312, 1.000000000000000000, 0.9510565162951535312, 1.000000000000000000, 0.9510565162951535312, 1.000000000000000000, 0.9510565162951535312, 1.000000000000000000, 0.9510565162951535312, 1.000000000000000000, 0.9510565162951535312, 1.000000000000000000, 0.9510565162951535312, 1.000000000000000000, 0.9510565162951535312, 1.000000000000000000, 0.9510565162951535312, 1.000000000000000000, 0.9510565162951535312, 1.000000000000000000, 0.9510565162951535312, 1.000000000000000000, 0.9510565162951535312, 1.000000000000000000, 0.9510565162951535312, 1.000000000000000000, 0.9510565162951535312, 1.000000000000000000, 0.9510565162951535312, 1.000000000000000000, 0.9510565162951535312, 1.000000000000000000, 0.9510565162951535312, 1.000000000000000000, 0.9510565162951535312, 1.000000000000000000, 0.9510565162951535312, 1.000000000000000000, 0.9510565162951535312, 1.000000000000000000, 0.9510565162951535312, 1.000000000000000000, 0.9510565162951535312, 1.000000000000000000, 0.9510565162951535312, 1.000000000000000000, 0.9510565162951535312, 1.000000000000000000, 0.9510565162951535312, 1.000000000000000000, 0.9510565162951535312, 1.000000000000000000, 0.9510565162951535312, 1.000000000000000000, 0.9510565162951535312, 1.000000000000000000, 0.9510565162951535312, 1.000000000000000000, 0.9510565162951535312, 1.000000000000000000, 0.9510565162951535312, 1.000000000000000000, 0.9510565162951535312, 1.000000000000000000, 0.9510565162951535312, 1.000000000000000000, 0.9510565162951535312, 1.000000000000000000, 0.9510565162951535312, 1.000000000000000000, 0.9510565162951535312, 1.000000000000000000, 0.9510565162951535312, 1.000000000000000000, 0.9510565162951535312, 1.000000000000000000, 0.9510565162951535312, 1.000000000000000000, 0.9510565162951535312, 1.000000000000000000, 0.9510565162951535312, 1.000000000000000000, 0.9510565162951535312, 1.000000000000000000, 0.9510565162951535312, 1.000000000000000000, 0.9510565162951535312, 1.000000000000000000, 0.9510565162951535312, 1.000000000000000000, 0.9510565162951535312, 1.000000000000000000, 0.9510565162951535312, 1.000000000000000000, 0.9510565162951535312, 1.000000000000000000, 0.9510565162951535312, 1.000000000000000000, 0.9510565162951535312, 1.000000000000000000, 0.9510565162951535312, 1.000000000000000000, 0.9510565162951535312, 1.000000000000000000, 0.9510565162951535312, 1.000000000000000000, 0.9510565162951535312, 1.000000000000000000, 0.9510565162951535312, 1.000000000000000000, 0.9510565162951535312, 1.000000000000000000, 0.9510565162951535312, 1.000000000000000000, 0.9510565162951535312, 1.000000000000000000, 0.9510565162951535312, 1.000000000000000000, 0.9510565162951535312, 1.000000000000000000, 0.9510565162951535312, 1.000000000000000000, 0.9510565162951535312, 1.000000000000000000, 0.9510565162951535312, 1.000000000000000000, 0.9510565162951535312, 1.000000000000000000, 0.9510565162951535312, 1.000000000000000000, 0.9510565162951535312, 1.000000000000000000, 0.9510565162951535312, 1.000000000000000000, 0.9510565162951535312, 1.000000000000000000, 0.9510565162951535312, 1.000000000000000000, 0.9510565162951535312, 1.000000000000000000, 0.9510565162951535312, 1.000000000000000000, 0.9510565162951535312, 1.000000000000000000, 0.9510565162951535312, 1.000000000000000000, 0.9510565162951535312, 1.000000000000000000, 0.9510565162951535312, 1.000000000000000000, 0.9510565162951535312, 1.000000000000000000, 0.9510565162951535312, 1.000000000000000000, 0.9510565162951535312, 1.000000000000000000, 0.9510565162951535312, 1.000000000000000000, 0.9510565162951535312, 1.000000000000000000, 0.9510565162951535312, 1.000000000000000000, 0.9510565162951535312, 1.000000000000000000, 0.9510565162951535312, 1.000000000000000000, 0.9510565162951535312, 1.000000000000000000, 0.9510565162951535312, 1.000000000000000000, 0.9510565162951535312, 1.000000000000000000, 0.9510565162951535312, 1.000000000000000000, 0.9510565162951535312, 1.000000000000000000, 0.9510565162951535312, 1.000000000000000000, 0.9510565162951535312, 1.000000000000000000, 0.9510565162951535312, 1.000000000000000000, 0.9510565162951535312, 1.000000000000000000, 0.9510565162951535312, 1.000000000000000000, 0.9510565162951535312, 1.000000000000000000, 0.9510565162951535312, 1.000000000000000000, 0.9510565162951535312, 1.000000000000000000, 0.9510565162951535312, 1.000000000000000000, 0.9510565162951535312, 1.000000000000000000, 0.9510565162951535312, 1.000000000000000000, 0.9510565162951535312, 1.000000000000000000, 0.9510565162951535312, 1.000000000000000000, 0.9510565162951535312, 1.000000000000000000, 0.9510565162951535312, 1.000000000000000000, 0.9510565162951535312, 1.000000000000000000, 0.9510565162951535312, 1.000000000000000000, 0.9510565162951535312, 1.000000000000000000, 0.9510565162951535312, 1.000000000000000000, 0.9510565162951535312, 1.000000000000000000, 0.9510565162951535312, 1.000000000000000000, 0.9510565162951535312, 1.000000000000000000, 0.9510565162951535312, 1.000000000000000000, 0.9510565162951535312, 1.000000000000000000, 0.9510565162951535312, 1.000000000000000000, 0.9510565162951535312, 1.000000000000000000, 0.9510565162951535312, 1.000000000000000000, 0.9510565162951535312, 1.000000000000000000, 0.9510565162951535312, 1.000000000000000000, 0.9510565162951535312, 1.000000000000000000, 0.9510565162951535312, 1.000000000000000000, 0.9510565162951535312, 1.000000000000000000, 0.9510565162951535312, 1.000000000000000000, 0.9510565162951535312, 1.000000000000000000, 0.9510565162951535312, 1.000000000000000000, 0.9510565162951535312, 1.000000000000000000, 0.9510565162951535312, 1.000000000000000000, 0.9510565162951535312, 1.000000000000000000, 0.9510565162951535312, 1.000000000000000000, 0.9510565162951535312, 1.000000000000000000, 0.9510565162951535312, 1.000000000000000000, 0.9510565162951535312, 1.000000000000000000, 0.9510565162951535312, 1.000000000000000000, 0.9510565162951535312, 1.000000000000000000, 0.9510565162951535312, 1.000000000000000000, 0.9510565162951535312, 1.000000000000000000, 0.9510565162951535312, 1.000000000000000000, 0.9510565162951535312, 1.000000000000000000, 0.9510565162951535312, 1.000000000000000000, 0.9510565162951535312, 1.000000000000000000, 0.9510565162951535312, 1.000000000000000000, 0.9510565162951535312, 1.000000000000000000, 0.9510565162951535312, 1.000000000000000000, 0.9510565162951535312, 1.000000000000000000, 0.9510565162951535312, 1.000000000000000000, 0.9510565162951535312, 1.000000000000000000, 0.9510565162951535312, 1.000000000000000000, 0.9510565162951535312, 1.000000000000000000, 0.9510565162951535312, 1.000000000000000000, 0.9510565162951535312, 1.000000000000000000, 0.9510565162951535312, 1.000000000000000000, 0.9510565162951535312, 1.000000000000000000, 0.9510565162951535312, 1.000000000000000000, 0.9510565162951535312, 1.000000000000000000, 0.9510565162951535312, 1.000000000000000000, 0.9510565162951535312, 1.000000000000000000, 0.9510565162951535312, 1.000000000000000000, 0.9510565162951535312, 1.000000000000000000, 0.9510565162951535312, 1.000000000000000000, 0.9510565162951535312, 1.000000000000000000, 0.9510565162951535312, 1.000000000000000000, 0.9510565162951535312, 1.000000000000000000, 0.9510565162951535312, 1.000000000000000000, 0.9510565162951535312, 1.000000000000000000, 0.9510565162951535312, 1.000000000000000000, 0.9510565162951535312, 1.000000000000000000, 0.9510565162951535312, 1.000000000000000000, 0.9510565162951535312, 1.000000000000000000, 0.9510565162951535312, 1.000000000000000000, 0.9510565162951535312, 1.000000000000000000, 0.9510565162951535312, 1.000000000000000000, 0.9510565162951535312, 1.000000000000000000, 0.9510565162951535312, 1.000000000000000000, 0.9510565162951535312, 1.000000000000000000, 0.9510565162951535312, 1.000000000000000000, 0.9510565162951535312, 1.000000000000000000, 0.9510565162951535312, 1.000000000000000000, 0.9510565162951535312, 1.000000000000000000, 0.9510565162951535312, 1.000000000000000000, 0.9510565162951535312, 1.000000000000000000, 0.9510565162951535312, 1.000000000000000000, 0.9510565162951535312, 1.000000000000000000, 0.9510565162951535312, 1.000000000000000000 ) ) 
 REPRESENTATION_ITEM ( '' )  );
#86053=CARTESIAN_POINT ( 'NONE',  ( 74.04521871459132853, 68.62337475623881744, 10.92041412683466106 ) ) ;
#86054=CARTESIAN_POINT ( 'NONE',  ( 71.04896452076110336, 71.47008843830593605, -2.670135699880026969 ) ) ;
#86066=FACE_OUTER_BOUND ( 'NONE', #65878, .T. ) ;
#86074=CARTESIAN_POINT ( 'NONE',  ( 72.94248495762835205, 57.43054579428017803, -15.86422397714476773 ) ) ;
#86078=CARTESIAN_POINT ( 'NONE',  ( 88.35351169220642475, 43.78681510747281180, 0.1754685934989752005 ) ) ;
#86082=CARTESIAN_POINT ( 'NONE',  ( 71.67184923690800247, 72.06465046553262255, -3.547063142499712551 ) ) ;
#86083=CARTESIAN_POINT ( 'NONE',  ( 70.84625275103223885, 71.05098293809255949, -5.242152369257887301 ) ) ;
#86085=CARTESIAN_POINT ( 'NONE',  ( 22.87854050506884818, 34.18502408145592852, 5.678558825948276656 ) ) ;
#86087=CARTESIAN_POINT ( 'NONE',  ( 83.86604369230676070, 46.91831489429971214, -11.24295167143095497 ) ) ;
#86088=CARTESIAN_POINT ( 'NONE',  ( 16.17343562415726765, 11.19860640527290840, 2.839279412974134775 ) ) ;
#86090=CARTESIAN_POINT ( 'NONE',  ( 76.75190111695991391, 63.66135907976974551, 15.32171075625996259 ) ) ;
#86093=CARTESIAN_POINT ( 'NONE',  ( 73.92247914240149953, 66.41009877986448373, 12.60535242438584191 ) ) ;
#86099=CARTESIAN_POINT ( 'NONE',  ( 77.03809386778178236, 49.55778004163211392, 14.99421684170569335 ) ) ;
#86104=CARTESIAN_POINT ( 'NONE',  ( 71.74269501503555091, 72.54435722921776630, -0.3765977487197710860 ) ) ;
#86107=CARTESIAN_POINT ( 'NONE',  ( 72.49520321802694411, 71.62171839754151392, 6.144630347475399823 ) ) ;
#86111=ORIENTED_EDGE ( 'NONE', *, *, #71507, .F. ) ;
#86112=CARTESIAN_POINT ( 'NONE',  ( 26.18145187173165311, 30.51421378149920116, -9.188101187500004485 ) ) ;
#86114=CARTESIAN_POINT ( 'NONE',  ( 84.60735463175657856, 50.53152741511170376, -13.60229262011999296 ) ) ;
#86116=DIRECTION ( 'NONE',  ( -0.8660254037844379305, -0.5000000000000014433, -0.000000000000000000 ) ) ;
#86120=CARTESIAN_POINT ( 'NONE',  ( 68.14508661930936739, 65.47790460345626684, 10.45464874189764615 ) ) ;
#86121=CARTESIAN_POINT ( 'NONE',  ( 67.90305891752841205, 66.04211081269261285, -10.46789290119909843 ) ) ;
#86124=CARTESIAN_POINT ( 'NONE',  ( 70.27722316875779995, 71.69590253475411146, -0.4825279500921932363 ) ) ;
#86129=CARTESIAN_POINT ( 'NONE',  ( 79.35100834308954632, 59.73271264539057057, 16.51943372556189971 ) ) ;
#86131=EDGE_LOOP ( 'NONE', ( #67621, #86374, #16254, #36494 ) ) ;
#86142=CARTESIAN_POINT ( 'NONE',  ( 80.98575723459396158, 56.01296387717067660, 16.09851198889879242 ) ) ;
#86146=ORIENTED_EDGE ( 'NONE', *, *, #26322, .F. ) ;
#86153=CARTESIAN_POINT ( 'NONE',  ( 75.84431516675671503, 65.82088634210550993, -14.12726274127321169 ) ) ;
#86156=CARTESIAN_POINT ( 'NONE',  ( 87.51647913336859119, 44.56403561216111342, 4.883618514853089287 ) ) ;
#86157=CARTESIAN_POINT ( 'NONE',  ( 84.48772039313885784, 43.72266692861629878, -6.677769858850941986 ) ) ;
#86163=DIRECTION ( 'NONE',  ( 0.8660254037844377084, 0.5000000000000015543, -0.000000000000000000 ) ) ;
#86167=CARTESIAN_POINT ( 'NONE',  ( 80.87517248313827167, 58.64441083166272506, 0.000000000000000000 ) ) ;
#86171=EDGE_CURVE ( 'NONE', #14510, #93933, #45558, .T. ) ;
#86176=CARTESIAN_POINT ( 'NONE',  ( 73.70324744805795092, 55.29378421878942618, 16.59304382234686770 ) ) ;
#86178=CARTESIAN_POINT ( 'NONE',  ( 27.37565231528585485, 31.50829794293882458, -10.00000000000000355 ) ) ;
#86183=CARTESIAN_POINT ( 'NONE',  ( 66.22544472841278207, 69.36168339246576409, 0.1681495645362244273 ) ) ;
#86189=CARTESIAN_POINT ( 'NONE',  ( 81.83513327003998938, 41.26677966152606558, 5.885019063842929832 ) ) ;
#86192=DIRECTION ( 'NONE',  ( 0.5000000000000014433, -0.8660254037844378194, 0.000000000000000000 ) ) ;
#86193=CARTESIAN_POINT ( 'NONE',  ( 27.54669006335486614, 38.83705186507756224, 3.090169943749475401 ) ) ;
#86194=CARTESIAN_POINT ( 'NONE',  ( 78.44203751522358914, 61.21016990572090322, 16.24725970467587643 ) ) ;
#86196=CARTESIAN_POINT ( 'NONE',  ( 73.68461719894507667, 68.07295893857846636, 11.72993004162934483 ) ) ;
#86197=CARTESIAN_POINT ( 'NONE',  ( 87.18660594880147130, 46.21918437583570238, -8.412104891579501142 ) ) ;
#86198=CARTESIAN_POINT ( 'NONE',  ( 87.98594423550160570, 43.75089820288620501, -2.253463800273097561 ) ) ;
#86203=CARTESIAN_POINT ( 'NONE',  ( 67.68514482100736984, 66.83340866827894899, -8.536435324610977204 ) ) ;
#86204=CARTESIAN_POINT ( 'NONE',  ( 77.54361356138011274, 49.75803992512373952, -14.96129575302290249 ) ) ;
#86207=FACE_OUTER_BOUND ( 'NONE', #19924, .T. ) ;
#86209=DIRECTION ( 'NONE',  ( 0.5000000000000014433, -0.8660254037844378194, 0.000000000000000000 ) ) ;
#86212=CARTESIAN_POINT ( 'NONE',  ( 20.38389956778225809, 29.95586893147755703, 7.433330006724141015 ) ) ;
#86217=ORIENTED_EDGE ( 'NONE', *, *, #48882, .F. ) ;
#86218=CARTESIAN_POINT ( 'NONE',  ( 10.59299460361177303, 21.51421378149917629, -9.188101187500004485 ) ) ;
#86219=CARTESIAN_POINT ( 'NONE',  ( 71.63674389864488035, 60.29001788040124410, -14.97147996658655345 ) ) ;
#86220=CARTESIAN_POINT ( 'NONE',  ( 71.54037008220826976, 72.37285432226113358, -1.295160433098011543 ) ) ;
#86223=CARTESIAN_POINT ( 'NONE',  ( 69.80538936212087719, 70.80406902493081134, -1.980385850607123688 ) ) ;
#86224=CARTESIAN_POINT ( 'NONE',  ( 85.57888796130104936, 49.00383361444075803, 12.24411226656481588 ) ) ;
#86229=CYLINDRICAL_SURFACE ( 'NONE', #77878, 10.00000000000001066 ) ;
#86230=CARTESIAN_POINT ( 'NONE',  ( 86.80341134427941086, 43.38235068936107552, -1.253824059860942697 ) ) ;
#86233=CARTESIAN_POINT ( 'NONE',  ( 71.73704408672971056, 72.08698097738312072, -3.607164568159269891 ) ) ;
#86234=CARTESIAN_POINT ( 'NONE',  ( 79.88594259850813728, 58.03267954034458143, 16.26759869156149563 ) ) ;
#86235=CARTESIAN_POINT ( 'NONE',  ( 76.83059214691050443, 63.69233987691562504, 15.32693845983791547 ) ) ;
#86239=ORIENTED_EDGE ( 'NONE', *, *, #30161, .F. ) ;
#86243=CARTESIAN_POINT ( 'NONE',  ( 23.73796034364816521, 35.74646525600390845, 2.839279412974139660 ) ) ;
#86245=CARTESIAN_POINT ( 'NONE',  ( 78.55537653917157570, 48.00561504237174404, -13.97647359956258484 ) ) ;
#86247=CARTESIAN_POINT ( 'NONE',  ( 74.20995892610953604, 68.60058487300136676, 11.02733404855581867 ) ) ;
#86248=CARTESIAN_POINT ( 'NONE',  ( 28.06847263831340555, 31.90829794293881960, 10.00000000000000355 ) ) ;
#86252=CARTESIAN_POINT ( 'NONE',  ( 86.58038954912636598, 46.32280579057140812, 9.040469064792965526 ) ) ;
#86253=CARTESIAN_POINT ( 'NONE',  ( 84.47030363695364485, 42.96640489140571617, -4.988567256042748532 ) ) ;
#86255=CARTESIAN_POINT ( 'NONE',  ( 77.75744084045382465, 52.33839962637683385, 16.14298180521786108 ) ) ;
#86266=CARTESIAN_POINT ( 'NONE',  ( 67.62155312284794206, 66.73364273201507046, 8.622086810066367235 ) ) ;
#86268=LINE ( 'NONE', #2628, #86919 ) ;
#86273=CARTESIAN_POINT ( 'NONE',  ( 83.48755897335753673, 41.55649808380166377, -1.266732648212113288 ) ) ;
#86277=CARTESIAN_POINT ( 'NONE',  ( 83.81305692926204642, 51.81190264249386956, -14.87427321595085417 ) ) ;
#86283=CARTESIAN_POINT ( 'NONE',  ( 74.59316757514828566, 66.97468268737705444, 12.54339389648529490 ) ) ;
#86287=VECTOR ( 'NONE', #90588, 1000.000000000000114 ) ;
#86292=CARTESIAN_POINT ( 'NONE',  ( 85.39315930365103213, 48.29864428352725980, -11.77802199426026952 ) ) ;
#86294=CARTESIAN_POINT ( 'NONE',  ( 70.78878230292833962, 62.60719215080742828, 13.74527488084627969 ) ) ;
#86296=EDGE_CURVE ( 'NONE', #69987, #54157, #60576, .T. ) ;
#86297=CARTESIAN_POINT ( 'NONE',  ( 80.07527276020931595, 44.25619389524629810, -11.41694498886655751 ) ) ;
#86303=CARTESIAN_POINT ( 'NONE',  ( 69.81243019392553606, 62.22010195957141576, -13.63492759933605392 ) ) ;
#86308=CARTESIAN_POINT ( 'NONE',  ( 17.55409693860148579, 9.944730856513913864, 1.475505719884397138E-15 ) ) ;
#86311=CARTESIAN_POINT ( 'NONE',  ( 72.27312669154171942, 72.08082049040204708, 3.221098087670088539 ) ) ;
#86312=CARTESIAN_POINT ( 'NONE',  ( 8.974214183003985212, 13.38052372038638538, 10.00000000000000533 ) ) ;
#86314=CARTESIAN_POINT ( 'NONE',  ( 8.129038565245441106, 16.64441083166258650, -10.00000000000000533 ) ) ;
#86321=FACE_OUTER_BOUND ( 'NONE', #9484, .T. ) ;
#86324=CARTESIAN_POINT ( 'NONE',  ( 30.66313333631613247, 33.10171378149921395, 9.188101187500008038 ) ) ;
#86330=CARTESIAN_POINT ( 'NONE',  ( 66.27754257038655794, 68.64336138396897979, 2.347787006359736139 ) ) ;
#86337=CARTESIAN_POINT ( 'NONE',  ( 18.07869151248302941, 12.29860640527291338, -2.839279412974138328 ) ) ;
#86347=CARTESIAN_POINT ( 'NONE',  ( 71.94643353573425770, 71.53214566342799685, 5.625104812542567778 ) ) ;
#86354=CARTESIAN_POINT ( 'NONE',  ( 86.13128675074533191, 47.68336462356251815, 10.84980215260790182 ) ) ;
#86356=CARTESIAN_POINT ( 'NONE',  ( 70.51627874990606415, 69.09918821448661674, 8.581095468001166182 ) ) ;
#86362=AXIS2_PLACEMENT_3D ( 'NONE', #22457, #53833, #53352 ) ;
#86363=CARTESIAN_POINT ( 'NONE',  ( 14.21206617776240044, 23.90829794293879473, 10.00000000000000355 ) ) ;
#86371=EDGE_CURVE ( 'NONE', #21644, #12155, #98736, .T. ) ;
#86374=ORIENTED_EDGE ( 'NONE', *, *, #11368, .F. ) ;
#86375=CARTESIAN_POINT ( 'NONE',  ( 73.10630316137316242, 60.13848896484078210, 15.30670999211671024 ) ) ;
#86376=VERTEX_POINT ( 'NONE', #9911 ) ;
#86377=CARTESIAN_POINT ( 'NONE',  ( 67.34792581060418115, 67.11477767218006818, 7.860511789199255084 ) ) ;
#86379=CARTESIAN_POINT ( 'NONE',  ( 83.44125680345078422, 49.92309224034626425, 13.59759453135232299 ) ) ;
#86380=CARTESIAN_POINT ( 'NONE',  ( 70.61396107802190159, 67.75272294984722521, 9.594151586959256406 ) ) ;
#86385=CARTESIAN_POINT ( 'NONE',  ( 21.67811977205257890, 27.91421378149918553, 9.188101187500008038 ) ) ;
#86405=CARTESIAN_POINT ( 'NONE',  ( 82.39390361753967795, 40.40531233075657980, -1.316817214398767089 ) ) ;
#86410=CARTESIAN_POINT ( 'NONE',  ( 75.67360416972866233, 65.58707386806378281, 13.80094545836168685 ) ) ;
#86412=ADVANCED_FACE ( 'NONE', ( #83320 ), #83822, .T. ) ;
#86415=ORIENTED_EDGE ( 'NONE', *, *, #40532, .F. ) ;
#86419=CARTESIAN_POINT ( 'NONE',  ( 68.38173023771584269, 69.91662463375536163, 2.194006220653268890 ) ) ;
#86424=CARTESIAN_POINT ( 'NONE',  ( 74.22019797964286170, 68.67351823779483766, -11.46693203622143820 ) ) ;
#86428=VERTEX_POINT ( 'NONE', #37661 ) ;
#86445=CARTESIAN_POINT ( 'NONE',  ( 75.58214075417596689, 65.23491603964200181, 14.35294216029142333 ) ) ;
#86449=CARTESIAN_POINT ( 'NONE',  ( 12.48623565965559479, 28.18502408145590721, 5.678558825948277544 ) ) ;
#86460=CARTESIAN_POINT ( 'NONE',  ( 85.85265132163429769, 47.44586991713102009, 10.77177032529229450 ) ) ;
#86466=CARTESIAN_POINT ( 'NONE',  ( 71.97141114645215509, 72.59821799906346484, 1.534520970786815042 ) ) ;
#86469=CYLINDRICAL_SURFACE ( 'NONE', #61439, 10.00000000000001066 ) ;
#86473=CARTESIAN_POINT ( 'NONE',  ( 41.71939737199939202, 29.80170272979930246, 7.433330006724137462 ) ) ;
#86474=CARTESIAN_POINT ( 'NONE',  ( 72.84734729035820067, 70.28725029195504703, -8.119559778710620179 ) ) ;
#86478=CARTESIAN_POINT ( 'NONE',  ( 85.03178579546401750, 43.95759251389035427, -7.567310116846363677 ) ) ;
#86481=CARTESIAN_POINT ( 'NONE',  ( 86.17795171810620047, 46.97265431477908493, -10.08908967461300143 ) ) ;
#86482=FACE_OUTER_BOUND ( 'NONE', #99035, .T. ) ;
#86485=CARTESIAN_POINT ( 'NONE',  ( 87.09656651665102345, 44.84278129179941885, -7.000152984404905965 ) ) ;
#86491=EDGE_CURVE ( 'NONE', #56024, #47030, #40823, .T. ) ;
#86492=ORIENTED_EDGE ( 'NONE', *, *, #55939, .F. ) ;
#86493=CARTESIAN_POINT ( 'NONE',  ( 77.14681100394483337, 49.55006509007303350, -14.96847495592216681 ) ) ;
#86502=DIRECTION ( 'NONE',  ( 0.4972609476841349796, -0.8612812260087746585, 0.1045284632676570652 ) ) ;
#86504=CARTESIAN_POINT ( 'NONE',  ( 76.74023481339004604, 63.31925950119924096, -15.43993991125870124 ) ) ;
#86510=CARTESIAN_POINT ( 'NONE',  ( 85.70574795423719650, 48.48025216897318046, -12.24584271313005601 ) ) ;
#86516=CARTESIAN_POINT ( 'NONE',  ( 72.99445915097255977, 65.45724384055469613, 12.87776796020878933 ) ) ;
#86518=CARTESIAN_POINT ( 'NONE',  ( 79.17346404451581066, 56.03057509265897096, 16.54773837286879967 ) ) ;
#86521=VERTEX_POINT ( 'NONE', #14869 ) ;
#86530=LINE ( 'NONE', #94110, #44583 ) ;
#86531=CARTESIAN_POINT ( 'NONE',  ( 87.74907107289486419, 44.16117455547063742, -4.521424286948807492 ) ) ;
#86544=CARTESIAN_POINT ( 'NONE',  ( 74.25054168435488577, 68.57848501580748746, 11.06803135282628325 ) ) ;
#86545=CARTESIAN_POINT ( 'NONE',  ( 69.82525098749390224, 70.94647340042538985, -0.9569406247209537586 ) ) ;
#86549=FACE_OUTER_BOUND ( 'NONE', #47171, .T. ) ;
#86553=CARTESIAN_POINT ( 'NONE',  ( 84.83525364562130733, 49.93448604028102267, -13.18857086666493217 ) ) ;
#86554=CARTESIAN_POINT ( 'NONE',  ( 77.87908970151455890, 62.02332377074587555, 15.65384233240896350 ) ) ;
#86556=CARTESIAN_POINT ( 'NONE',  ( 76.42510427590111988, 51.13649333467196811, 16.04694757192931931 ) ) ;
#86560=CARTESIAN_POINT ( 'NONE',  ( 71.77313022743312843, 71.85913065286145240, 2.952583973247177251 ) ) ;
#86568=CARTESIAN_POINT ( 'NONE',  ( 88.33060278926279807, 43.77373715677852317, 0.1867717842524379002 ) ) ;
#86572=CARTESIAN_POINT ( 'NONE',  ( 24.17276070933917609, 32.14336893147756768, 7.433330006724141015 ) ) ;
#86574=CARTESIAN_POINT ( 'NONE',  ( 80.57150847499261204, 47.56777207323567325, -13.10156609182119958 ) ) ;
#86575=CARTESIAN_POINT ( 'NONE',  ( 11.93836421708519779, 28.93396525600389069, 2.839279412974139660 ) ) ;
#86584=CARTESIAN_POINT ( 'NONE',  ( 87.58100233665301459, 44.90480556695516867, -6.571228966301012164 ) ) ;
#86588=VERTEX_POINT ( 'NONE', #77698 ) ;
#86589=CARTESIAN_POINT ( 'NONE',  ( 86.10640163849959094, 46.41140333115836114, 9.428975133176919599 ) ) ;
#86593=DIRECTION ( 'NONE',  ( 0.4493970231495826861, -0.7783784768652872721, -0.4383711467890751834 ) ) ;
#86594=CARTESIAN_POINT ( 'NONE',  ( 73.16639139570222028, 68.70606694088236566, -10.26624930846365125 ) ) ;
#86597=B_SPLINE_CURVE_WITH_KNOTS ( 'NONE', 3,
 ( #23612, #92575, #83481, #6932, #61120, #75872, #6450, #68230, #99153, #29741, #79881, #9949, #71756, #32229, #79385, #24135, #70732, #87516, #86002, #87002, #57021, #8934, #40810, #63131, #46933, #32728, #2351, #18049, #70224, #39306, #40314, #94075, #33231, #55021, #1343, #48944, #16528, #17530, #16032, #24627, #93567, #55508, #77850, #63632, #64135, #10443 ),
 .UNSPECIFIED., .F., .F.,
 ( 4, 1, 2, 2, 1, 2, 2, 1, 1, 2, 2, 1, 1, 2, 2, 1, 1, 2, 2, 1, 1, 1, 2, 2, 1, 1, 1, 2, 2, 4 ),
 ( 0.000000000000000000, 0.06250000000000156819, 0.09375000000000216493, 0.1250000000000027756, 0.1875000000000044131, 0.2187500000000063283, 0.2500000000000082157, 0.3125000000000114908, 0.3437500000000141553, 0.3593750000000145439, 0.3750000000000149880, 0.4375000000000159317, 0.4687500000000164868, 0.4843750000000155431, 0.5000000000000145439, 0.5625000000000082157, 0.5937500000000061062, 0.6093750000000054401, 0.6250000000000046629, 0.6875000000000074385, 0.7187500000000093259, 0.7343750000000107692, 0.7421875000000118794, 0.7500000000000128786, 0.8125000000000160982, 0.8437500000000163203, 0.8593750000000163203, 0.8671875000000154321, 0.8750000000000145439, 1.000000000000000000 ),
 .UNSPECIFIED. ) ;
#86598=ORIENTED_EDGE ( 'NONE', *, *, #1768, .F. ) ;
#86599=CYLINDRICAL_SURFACE ( 'NONE', #89545, 10.00000000000001066 ) ;
#86602=ORIENTED_EDGE ( 'NONE', *, *, #61268, .T. ) ;
#86604=CARTESIAN_POINT ( 'NONE',  ( 29.50362127723248662, 19.96004757982091604, -5.678558825948275768 ) ) ;
#86605=CARTESIAN_POINT ( 'NONE',  ( 75.27101761674283864, 66.49390254752692897, -13.13272271682535930 ) ) ;
#86606=CARTESIAN_POINT ( 'NONE',  ( 74.14312167556930433, 66.30466486950707861, 1.224646799147354045E-15 ) ) ;
#86621=CARTESIAN_POINT ( 'NONE',  ( 70.79942557690317528, 62.94285302112024993, -14.11492782255271017 ) ) ;
#86626=CARTESIAN_POINT ( 'NONE',  ( 78.01756760496483878, 61.41364688087467272, -16.16017056289257425 ) ) ;
#86633=CARTESIAN_POINT ( 'NONE',  ( 85.36737598551003714, 42.56170592440086153, 0.09984784679323620293 ) ) ;
#86634=CARTESIAN_POINT ( 'NONE',  ( 86.12135434523638366, 46.98046262810483142, -10.13131473785488090 ) ) ;
#86640=ADVANCED_FACE ( 'NONE', ( #64480 ), #79227, .T. ) ;
#86642=B_SPLINE_SURFACE_WITH_KNOTS ( 'NONE', 3, 1, ( 
 ( #42746, #96513 ),
 ( #57966, #73680 ),
 ( #41254, #22327 ),
 ( #68917, #38004 ),
 ( #8135, #92759 ),
 ( #38513, #90787 ),
 ( #99348, #53227 ),
 ( #69425, #46613 ),
 ( #45123, #14728 ),
 ( #30924, #23313 ),
 ( #39008, #45609 ),
 ( #28944, #59821 ),
 ( #77545, #29432 ),
 ( #84665, #99842 ),
 ( #97019, #38 ),
 ( #91761, #21338 ),
 ( #83673, #6130 ),
 ( #76541, #6639 ),
 ( #30426, #67935 ),
 ( #37026, #13731 ),
 ( #61809, #76060 ),
 ( #52715, #53708 ),
 ( #61315, #37514 ),
 ( #68421, #91265 ),
 ( #29927, #60802 ),
 ( #7119, #14237 ),
 ( #54200, #85168 ),
 ( #92278, #52223 ),
 ( #98856, #22825 ),
 ( #60308, #84179 ),
 ( #15208, #46103 ) ),
 .UNSPECIFIED., .F., .F., .F.,
 ( 4, 3, 3, 3, 3, 3, 3, 3, 3, 3, 4 ),
 ( 2, 2 ),
 ( 0.000000000000000000, 0.1333490885032285189, 0.3007194338854188853, 0.4699862290244924967, 0.5844252810809184018, 0.6686540514502693489, 0.7354980260655538116, 0.8028463152565737948, 0.8633854507757268149, 0.9437142632667515629, 1.000000000000000000 ),
 ( 0.000000000000000000, 1.000000000000000000 ),
 .UNSPECIFIED. ) ;
#86646=CARTESIAN_POINT ( 'NONE',  ( 75.75917444283010127, 65.12044684595205979, -14.46054081031674876 ) ) ;
#86649=CARTESIAN_POINT ( 'NONE',  ( 87.84403297180379866, 44.29423158952226203, 4.754374079557551980 ) ) ;
#86651=CARTESIAN_POINT ( 'NONE',  ( 83.03297025961435907, 43.66274663663242706, -7.959272922208247003 ) ) ;
#86657=CARTESIAN_POINT ( 'NONE',  ( 76.61888230025124358, 51.35972145274619294, 16.07233720520855158 ) ) ;
#86661=CARTESIAN_POINT ( 'NONE',  ( 85.85494225371405719, 44.84660830416275701, 7.405870140133522739 ) ) ;
#86663=CARTESIAN_POINT ( 'NONE',  ( 83.98894966577088894, 51.79070771454841093, 14.82098776213804570 ) ) ;
#86668=CARTESIAN_POINT ( 'NONE',  ( 72.77272354753068839, 64.36932843330238541, -13.45330500611205338 ) ) ;
#86670=FACE_OUTER_BOUND ( 'NONE', #57174, .T. ) ;
#86673=CARTESIAN_POINT ( 'NONE',  ( 35.46999748293995225, 20.28848085856233396, 1.475505719884397138E-15 ) ) ;
#86680=CARTESIAN_POINT ( 'NONE',  ( 81.84495297315717721, 46.76928670720106851, 12.06671785398880203 ) ) ;
#86687=CARTESIAN_POINT ( 'NONE',  ( 37.50785463075374793, 23.78380873178790011, -6.180339887498949025 ) ) ;
#86690=AXIS2_PLACEMENT_3D ( 'NONE', #84215, #76572, #14762 ) ;
#86691=CARTESIAN_POINT ( 'NONE',  ( 81.64869726432758057, 55.83996916651700815, 16.01049500238219636 ) ) ;
#86697=CARTESIAN_POINT ( 'NONE',  ( 67.68514482100736984, 66.83340866827894899, -8.536435324610977204 ) ) ;
#86702=CYLINDRICAL_SURFACE ( 'NONE', #75589, 10.00000000000001066 ) ;
#86710=CARTESIAN_POINT ( 'NONE',  ( 19.72598728594001116, 34.49540643055188127, 3.479690158560446702E-15 ) ) ;
#86715=CARTESIAN_POINT ( 'NONE',  ( 13.56875384759882941, 10.76004757982087945, 5.678558825948272215 ) ) ;
#86718=CARTESIAN_POINT ( 'NONE',  ( 78.98302057781839380, 57.72790023617148591, -16.24074392209231377 ) ) ;
#86719=CARTESIAN_POINT ( 'NONE',  ( 71.88488839165290756, 72.57896392602057745, -1.213109508826733407 ) ) ;
#86724=CARTESIAN_POINT ( 'NONE',  ( 85.05360768983020137, 48.89064580773020907, 12.39253331958761883 ) ) ;
#86725=CARTESIAN_POINT ( 'NONE',  ( 82.81737761406506593, 40.62361263874299055, 0.9906565629087065172 ) ) ;
#86729=VERTEX_POINT ( 'NONE', #32061 ) ;
#86732=VERTEX_POINT ( 'NONE', #24967 ) ;
#86736=CARTESIAN_POINT ( 'NONE',  ( 72.59376736060184498, 57.25557935749301208, -16.34525399114337674 ) ) ;
#86737=CARTESIAN_POINT ( 'NONE',  ( 76.72979488479921883, 63.64413466080264214, 15.32332512078611053 ) ) ;
#86743=AXIS2_PLACEMENT_3D ( 'NONE', #40467, #10591, #10092 ) ;
#86747=CARTESIAN_POINT ( 'NONE',  ( 29.31959766232195008, 28.87878583063843152, -9.188101187500006262 ) ) ;
#86749=CARTESIAN_POINT ( 'NONE',  ( 78.48406258408499525, 47.91922444745478771, -14.50189708698971636 ) ) ;
#86751=CARTESIAN_POINT ( 'NONE',  ( 74.01669459151050035, 68.61891074470059948, 11.40943161386742943 ) ) ;
#86756=ORIENTED_EDGE ( 'NONE', *, *, #60011, .T. ) ;
#86757=CARTESIAN_POINT ( 'NONE',  ( 79.15788838581835307, 56.95875276203359050, -16.19999125909624382 ) ) ;
#86758=CARTESIAN_POINT ( 'NONE',  ( 85.33874453257102743, 43.13968784339352425, -4.066132831716157803 ) ) ;
#86761=ORIENTED_EDGE ( 'NONE', *, *, #21554, .F. ) ;
#86763=CARTESIAN_POINT ( 'NONE',  ( 70.38949794949537875, 69.79236328211965201, -6.331911208559731108 ) ) ;
#86773=ORIENTED_EDGE ( 'NONE', *, *, #72937, .F. ) ;
#86776=CARTESIAN_POINT ( 'NONE',  ( 82.78931075109494486, 41.26378757911983541, -2.085430941142616845 ) ) ;
#86780=CARTESIAN_POINT ( 'NONE',  ( 83.74759088628145776, 52.16275448854534602, -14.64583489767789359 ) ) ;
#86783=CARTESIAN_POINT ( 'NONE',  ( 80.54323102745749452, 57.15263273657545540, -16.22921413641979527 ) ) ;
#86794=CARTESIAN_POINT ( 'NONE',  ( 74.01261531380109204, 61.39505503205761272, -15.55988254646882041 ) ) ;
#86796=CARTESIAN_POINT ( 'NONE',  ( 69.97056695745257571, 70.69477875497891262, -3.199289782720719177 ) ) ;
#86798=CARTESIAN_POINT ( 'NONE',  ( 82.06139759189935035, 41.84807635679941029, -5.567411470978655075 ) ) ;
#86805=CARTESIAN_POINT ( 'NONE',  ( 22.23522817490527359, 21.03677371833801857, 10.00000000000000533 ) ) ;
#86809=CARTESIAN_POINT ( 'NONE',  ( 87.63430470890591550, 44.67548875376495943, 5.011216075979657347 ) ) ;
#86810=VECTOR ( 'NONE', #35963, 1000.000000000000114 ) ;
#86812=CARTESIAN_POINT ( 'NONE',  ( 10.81481306776012019, 28.01751292744054922, 6.180339887498949913 ) ) ;
#86813=CARTESIAN_POINT ( 'NONE',  ( 78.97208057699353390, 50.23458188978398908, -15.35366105675574389 ) ) ;
#86816=CARTESIAN_POINT ( 'NONE',  ( 73.92154985004793843, 55.00500715705026522, -16.60400407066505224 ) ) ;
#86822=CARTESIAN_POINT ( 'NONE',  ( 66.50747487571916849, 68.84019554392912710, -4.400006582833474233 ) ) ;
#86826=CARTESIAN_POINT ( 'NONE',  ( 70.34454795188869980, 61.29844696716961749, 14.78467410895967760 ) ) ;
#86829=CARTESIAN_POINT ( 'NONE',  ( 33.43441462842632461, 34.70171378149921537, -9.188101187500004485 ) ) ;
#86831=CARTESIAN_POINT ( 'NONE',  ( 80.41925082966935179, 57.89142005328343288, -16.24736989457703373 ) ) ;
#86834=CARTESIAN_POINT ( 'NONE',  ( 32.17146729527596705, 24.28920272979928541, -7.433330006724141015 ) ) ;
#86837=CARTESIAN_POINT ( 'NONE',  ( 66.30487963216988589, 69.19110079912826450, 2.493735217155242267 ) ) ;
#86842=CARTESIAN_POINT ( 'NONE',  ( 12.32384911305235420, 19.06628583063839955, -9.188101187500006262 ) ) ;
#86845=CARTESIAN_POINT ( 'NONE',  ( 84.65536491870415148, 49.91664468313385328, -13.65730316586987669 ) ) ;
#86852=CARTESIAN_POINT ( 'NONE',  ( 87.65066030812953102, 45.32478036133853294, 6.436761220525266225 ) ) ;
#86857=CARTESIAN_POINT ( 'NONE',  ( 86.22850481619846619, 47.19188645326008924, 10.82438011396962096 ) ) ;
#86865=CARTESIAN_POINT ( 'NONE',  ( 79.21589564954884111, 59.07845406483318129, -16.22212184578609495 ) ) ;
#86866=CARTESIAN_POINT ( 'NONE',  ( 12.81113585708611957, 26.13478043621386959, 8.090169943749478065 ) ) ;
#86867=VERTEX_POINT ( 'NONE', #88842 ) ;
#86877=ORIENTED_EDGE ( 'NONE', *, *, #10419, .T. ) ;
#86878=CARTESIAN_POINT ( 'NONE',  ( 74.23636598098558181, 65.21952277656190233, 13.49801994419013873 ) ) ;
#86883=CARTESIAN_POINT ( 'NONE',  ( 72.29246316029069419, 70.94367127312519017, 6.361853069214371104 ) ) ;
#86885=CARTESIAN_POINT ( 'NONE',  ( 82.75811122462442881, 53.31634770240417254, -15.29016885083995980 ) ) ;
#86886=CYLINDRICAL_SURFACE ( 'NONE', #77376, 10.00000000000001066 ) ;
#86889=CARTESIAN_POINT ( 'NONE',  ( 27.42516030814984163, 18.76004757982090609, 5.678558825948272215 ) ) ;
#86900=AXIS2_PLACEMENT_3D ( 'NONE', #68753, #19334, #99180 ) ;
#86905=CARTESIAN_POINT ( 'NONE',  ( 14.26996179277632848, 9.208019796199270246, -3.090169943749474069 ) ) ;
#86906=CARTESIAN_POINT ( 'NONE',  ( 75.04096107751730926, 66.95220489134598552, -13.17375343603499971 ) ) ;
#86910=CARTESIAN_POINT ( 'NONE',  ( 82.32772868565227498, 40.91284795898661031, -1.238209237945167018 ) ) ;
#86914=LINE ( 'NONE', #79307, #60837 ) ;
#86919=VECTOR ( 'NONE', #9214, 1000.000000000000114 ) ;
#86925=CARTESIAN_POINT ( 'NONE',  ( 80.82015971479509631, 46.89095932202825878, -12.57338494565948217 ) ) ;
#86926=CARTESIAN_POINT ( 'NONE',  ( 84.47342800902475801, 44.30953683796652598, 7.759599405057208799 ) ) ;
#86929=CARTESIAN_POINT ( 'NONE',  ( 82.92763370183318727, 43.61014228372319934, 7.996515586641524287 ) ) ;
#86930=CARTESIAN_POINT ( 'NONE',  ( 74.23555041547366784, 68.49601928387086502, -11.11897725275786719 ) ) ;
#86936=CARTESIAN_POINT ( 'NONE',  ( 84.26780123106441067, 48.10812409167185422, 12.07091365660302884 ) ) ;
#86939=CARTESIAN_POINT ( 'NONE',  ( 69.12672858200176051, 64.33651235087042153, -11.97836756590942642 ) ) ;
#86951=CARTESIAN_POINT ( 'NONE',  ( 21.25954720759204974, 17.98920272979926338, 7.433330006724137462 ) ) ;
#86952=CARTESIAN_POINT ( 'NONE',  ( 75.28739987566954994, 66.81623516066271407, 13.35525127813182245 ) ) ;
#86960=CARTESIAN_POINT ( 'NONE',  ( 81.96605124766598749, 41.04055892413879292, -3.298067608424472219 ) ) ;
#86962=CARTESIAN_POINT ( 'NONE',  ( 86.37884356567975885, 47.61826986380418703, 10.63568397185587067 ) ) ;
#86973=CARTESIAN_POINT ( 'NONE',  ( 10.03096235389214286, 7.350182197602630474, 1.163414459189986274E-15 ) ) ;
#86979=CARTESIAN_POINT ( 'NONE',  ( 41.11799749075662191, 32.24335787977766898, -9.188101187500008038 ) ) ;
#86981=EDGE_LOOP ( 'NONE', ( #38338, #1069, #6475, #70860 ) ) ;
#86986=CARTESIAN_POINT ( 'NONE',  ( 86.15816146546031007, 46.97362167137357147, -10.10205920913481847 ) ) ;
#86990=CARTESIAN_POINT ( 'NONE',  ( 78.08492915682273861, 51.99795259853134155, -15.56358649237862579 ) ) ;
#86996=ORIENTED_EDGE ( 'NONE', *, *, #15466, .F. ) ;
#86999=CARTESIAN_POINT ( 'NONE',  ( 77.20793521647205182, 49.23014827807851646, -14.84469579315973675 ) ) ;
#87001=CARTESIAN_POINT ( 'NONE',  ( 74.30633198134589179, 55.67512901695737781, 16.11735991574911253 ) ) ;
#87002=CARTESIAN_POINT ( 'NONE',  ( 79.23877006284985214, 53.37623035401563243, 15.75486908137112607 ) ) ;
#87003=ORIENTED_EDGE ( 'NONE', *, *, #50508, .T. ) ;
#87014=CARTESIAN_POINT ( 'NONE',  ( 75.50851089389813353, 54.04939035683948134, 16.08387913541453784 ) ) ;
#87016=CARTESIAN_POINT ( 'NONE',  ( 41.44275701717577221, 32.43085787977767609, -9.188101187500008038 ) ) ;
#87018=CARTESIAN_POINT ( 'NONE',  ( 76.28872632190457637, 51.00282802105010660, -16.03419075268625349 ) ) ;
#87024=CARTESIAN_POINT ( 'NONE',  ( 72.70287041210059442, 64.35211551445759426, 13.43818951508896120 ) ) ;
#87029=ORIENTED_EDGE ( 'NONE', *, *, #96274, .T. ) ;
#87049=CARTESIAN_POINT ( 'NONE',  ( 14.52789699003380974, 30.16126292948894871, -6.180339887498951690 ) ) ;
#87050=CARTESIAN_POINT ( 'NONE',  ( 73.77685717047434366, 68.42255065178834172, 10.96230068806748825 ) ) ;
#87051=CARTESIAN_POINT ( 'NONE',  ( 67.69698224970645128, 69.54660018620847950, 2.034176490069760312 ) ) ;
#87058=CARTESIAN_POINT ( 'NONE',  ( 78.99848661620951873, 60.24637179098722584, -16.44349368446545867 ) ) ;
#87061=VECTOR ( 'NONE', #63016, 1000.000000000000114 ) ;
#87063=DIRECTION ( 'NONE',  ( 0.5000000000000014433, -0.8660254037844378194, 0.000000000000000000 ) ) ;
#87072=CARTESIAN_POINT ( 'NONE',  ( 72.79244417080386143, 57.34122303501653306, -15.86467494005183099 ) ) ;
#87076=CARTESIAN_POINT ( 'NONE',  ( 76.93764771006534886, 63.33963654317832948, -15.47180374620822008 ) ) ;
#87079=CARTESIAN_POINT ( 'NONE',  ( 88.37182738025107653, 44.19934082970731026, 0.1226661121921119174 ) ) ;
#87080=CARTESIAN_POINT ( 'NONE',  ( 12.03141808487008824, 12.11029122506292488, -8.090169943749478065 ) ) ;
#87084=CARTESIAN_POINT ( 'NONE',  ( 26.18025557360336464, 27.06628583063842797, -9.188101187500006262 ) ) ;
#87088=CARTESIAN_POINT ( 'NONE',  ( 23.10163885443276754, 15.19860640527292261, 2.839279412974134775 ) ) ;
#87090=CARTESIAN_POINT ( 'NONE',  ( 76.54295893941512929, 63.70811625220086682, 14.88924590245834345 ) ) ;
#87092=CARTESIAN_POINT ( 'NONE',  ( 73.64338300972052309, 65.35231775803438836, 13.17446611551941693 ) ) ;
#87094=CARTESIAN_POINT ( 'NONE',  ( 86.72740319991413571, 46.97082492543196963, 10.28929863393111610 ) ) ;
#87096=CARTESIAN_POINT ( 'NONE',  ( 87.54287973956584779, 45.08362754214010693, -6.108144277352557161 ) ) ;
#87104=ORIENTED_EDGE ( 'NONE', *, *, #58748, .F. ) ;
#87106=CARTESIAN_POINT ( 'NONE',  ( 65.82437655349816907, 69.12761348810168727, -0.3171013769033966812 ) ) ;
#87112=FACE_OUTER_BOUND ( 'NONE', #35435, .T. ) ;
#87120=CARTESIAN_POINT ( 'NONE',  ( 20.82173017108080515, 32.99752408145592142, 5.678558825948276656 ) ) ;
#87121=CARTESIAN_POINT ( 'NONE',  ( 84.72527825293784076, 50.50787217764868586, -13.97547420692928277 ) ) ;
#87122=CARTESIAN_POINT ( 'NONE',  ( 78.58789454043932210, 49.48878357515709325, -14.64335108961764753 ) ) ;
#87131=CARTESIAN_POINT ( 'NONE',  ( 68.01260680319232677, 65.70736637594835372, 10.87867279016386846 ) ) ;
#87135=CARTESIAN_POINT ( 'NONE',  ( 34.21278864456112956, 38.49103043416551628, -8.090169943749479842 ) ) ;
#87138=CARTESIAN_POINT ( 'NONE',  ( 76.62458508144393932, 61.22216847580316568, -16.02601530327725854 ) ) ;
#87140=CARTESIAN_POINT ( 'NONE',  ( 83.00815485991435594, 53.30142267139500234, 15.60062745561815589 ) ) ;
#87148=CARTESIAN_POINT ( 'NONE',  ( 80.07914371544711685, 44.88103632949623290, -11.28840885768255831 ) ) ;
#87149=CARTESIAN_POINT ( 'NONE',  ( 66.61164111217610184, 67.57600878003083267, 6.268342412446013867 ) ) ;
#87151=CARTESIAN_POINT ( 'NONE',  ( 83.51043124159053832, 41.69464146566779306, -2.173292712442712826 ) ) ;
#87152=CARTESIAN_POINT ( 'NONE',  ( 83.49336806191682570, 47.60227169604173270, -12.02527693348223359 ) ) ;
#87156=VECTOR ( 'NONE', #51524, 1000.000000000000000 ) ;
#87161=EDGE_CURVE ( 'NONE', #92377, #5574, #20216, .T. ) ;
#87162=CARTESIAN_POINT ( 'NONE',  ( 31.74858474661088081, 18.73415679381823651, -6.890680421881970419E-14 ) ) ;
#87163=CARTESIAN_POINT ( 'NONE',  ( 69.81648863541811068, 69.35147540035858071, -6.558477812184903222 ) ) ;
#87165=CARTESIAN_POINT ( 'NONE',  ( 88.04657803224654344, 44.71669033064829080, 4.399168146237476762 ) ) ;
#87167=CARTESIAN_POINT ( 'NONE',  ( 86.58890667216479642, 43.96449127922488032, -4.508632658051355158 ) ) ;
#87172=CARTESIAN_POINT ( 'NONE',  ( 72.41389820116259557, 70.72247311216294463, 7.745007521649676541 ) ) ;
#87177=CARTESIAN_POINT ( 'NONE',  ( 84.30145135017787084, 42.73273955677608882, 4.648230990532672635 ) ) ;
#87180=CARTESIAN_POINT ( 'NONE',  ( 83.19273697349305507, 52.30514367268771991, 14.84689007325454213 ) ) ;
#87187=CARTESIAN_POINT ( 'NONE',  ( 76.90746743093833970, 62.93938289886319382, -15.23233999435670150 ) ) ;
#87189=CARTESIAN_POINT ( 'NONE',  ( 74.30611599946955437, 55.28061810189145575, 16.60300916044171160 ) ) ;
#87190=CARTESIAN_POINT ( 'NONE',  ( 69.63353853914595959, 62.64057578429665796, -13.33088475737029732 ) ) ;
#87192=CARTESIAN_POINT ( 'NONE',  ( 24.08934983677281494, 38.00034080476292075, -1.878358725466461243E-16 ) ) ;
#87195=CARTESIAN_POINT ( 'NONE',  ( 72.46511837996447980, 71.56249752072032777, 6.234640293157904800 ) ) ;
#87196=CARTESIAN_POINT ( 'NONE',  ( 72.02976470237955198, 59.30830629416842470, -15.33705471575644808 ) ) ;
#87198=EDGE_CURVE ( 'NONE', #92094, #65643, #83457, .T. ) ;
#87202=CARTESIAN_POINT ( 'NONE',  ( 82.50577570618477807, 48.91507585382240109, 13.31341743689232082 ) ) ;
#87206=CARTESIAN_POINT ( 'NONE',  ( 84.89744547285587828, 41.79037650531964943, -3.168800655305855967E-06 ) ) ;
#87209=CARTESIAN_POINT ( 'NONE',  ( 36.11248442148217919, 32.80066082961424456, 10.00000000000000533 ) ) ;
#87213=CARTESIAN_POINT ( 'NONE',  ( 81.30729757080379727, 56.16728312479073537, 16.09392928925141319 ) ) ;
#87214=CARTESIAN_POINT ( 'NONE',  ( 5.030029564959478172, 25.83705186507751606, 3.090169943749475401 ) ) ;
#87215=PRODUCT_DEFINITION_SHAPE ( 'NONE', 'NONE',  #77462 ) ;
#87219=CARTESIAN_POINT ( 'NONE',  ( 68.57390157943029863, 66.83352816882218406, -9.225073082748975750 ) ) ;
#87226=B_SPLINE_CURVE_WITH_KNOTS ( 'NONE', 3,
 ( #81529, #51072, #35880, #33916, #26303, #20202, #97226, #96735, #65293, #41989 ),
 .UNSPECIFIED., .F., .F.,
 ( 4, 2, 2, 2, 4 ),
 ( 0.000000000000000000, 0.0002622400424272822378, 0.0005244800848545644757, 0.0007867201272818467135, 0.001048960169709128951 ),
 .UNSPECIFIED. ) ;
#87234=CARTESIAN_POINT ( 'NONE',  ( 30.11465696128792757, 23.10170272979928541, -7.433330006724141015 ) ) ;
#87239=CARTESIAN_POINT ( 'NONE',  ( 4.512196379633642174, 24.64646525600387861, -2.839279412974133887 ) ) ;
#87240=DIRECTION ( 'NONE',  ( 0.2938926261462335709, -0.5090369604551240323, 0.8090169943749504489 ) ) ;
#87242=EDGE_CURVE ( 'NONE', #84611, #16883, #67389, .T. ) ;
#87257=CARTESIAN_POINT ( 'NONE',  ( 72.68761047489735461, 57.54079809338966101, -16.30797607761032353 ) ) ;
#87258=CARTESIAN_POINT ( 'NONE',  ( 76.75190111695991391, 63.66135907976974551, 15.32171075625996259 ) ) ;
#87269=CARTESIAN_POINT ( 'NONE',  ( 33.34238925418374322, 21.11110640527294180, -2.839279412974138328 ) ) ;
#87271=CARTESIAN_POINT ( 'NONE',  ( 78.43208466135750712, 48.00925285049068947, -14.01282328640595232 ) ) ;
#87273=ORIENTED_EDGE ( 'NONE', *, *, #65292, .F. ) ;
#87274=CARTESIAN_POINT ( 'NONE',  ( 73.77733668265750566, 68.41783923479601981, 11.46675506585085813 ) ) ;
#87280=CARTESIAN_POINT ( 'NONE',  ( 78.58888364635852497, 57.18144897753006006, -16.20312259563071677 ) ) ;
#87282=CARTESIAN_POINT ( 'NONE',  ( 77.52183548858428708, 51.28834266016709620, 15.94339560165845171 ) ) ;
#87292=CARTESIAN_POINT ( 'NONE',  ( 67.28413888684362121, 66.89988542115362691, 9.018600864293709662 ) ) ;
#87301=CARTESIAN_POINT ( 'NONE',  ( 83.48909022670937929, 51.62989903239390088, -14.87641496889664694 ) ) ;
#87302=CARTESIAN_POINT ( 'NONE',  ( 76.47316661484272515, 51.61210842333346704, -15.65491330287230376 ) ) ;
#87304=CARTESIAN_POINT ( 'NONE',  ( 80.46436188522254440, 57.84947393126303439, -16.24692113171143504 ) ) ;
#87306=CARTESIAN_POINT ( 'NONE',  ( 72.73213343415878285, 70.95121167556251862, 7.670646158728279929 ) ) ;
#87314=CARTESIAN_POINT ( 'NONE',  ( 85.58533047404948491, 48.36141062822003533, -12.20656690058575400 ) ) ;
#87316=CARTESIAN_POINT ( 'NONE',  ( 87.92187120394066824, 44.49289898744115135, -3.958561838072920391 ) ) ;
#87317=EDGE_CURVE ( 'NONE', #98946, #33229, #91646, .T. ) ;
#87318=CARTESIAN_POINT ( 'NONE',  ( 80.01318412846774208, 44.36046053175815729, -11.54377855748506043 ) ) ;
#87320=CARTESIAN_POINT ( 'NONE',  ( 81.76576923011752740, 41.62693581818646749, 5.446883335929131320 ) ) ;
#87326=ADVANCED_FACE ( 'NONE', ( #70707 ), #63605, .T. ) ;
#87327=CARTESIAN_POINT ( 'NONE',  ( 79.01371845142224970, 52.41748766984506602, -15.53612108484040100 ) ) ;
#87332=CARTESIAN_POINT ( 'NONE',  ( 10.81481306776012019, 28.01751292744054922, 6.180339887498949913 ) ) ;
#87335=CARTESIAN_POINT ( 'NONE',  ( 23.63615849558155446, 18.81029122506294726, 8.090169943749479842 ) ) ;
#87337=DIRECTION ( 'NONE',  ( -0.06958655048002569676, 0.1205274409548614395, -0.9902680687415721383 ) ) ;
#87347=B_SPLINE_CURVE_WITH_KNOTS ( 'NONE', 3,
 ( #28024, #23399, #18699, #53792, #124, #69510, #92358, #25807, #77636, #54807, #49093, #2505, #7713, #84754, #77109, #80028, #70509, #33387, #22906, #85260, #11113, #64289, #85784, #10596, #41469, #56682, #23906, #15805, #72417, #15293, #62392 ),
 .UNSPECIFIED., .F., .F.,
 ( 4, 3, 3, 3, 3, 3, 3, 3, 3, 3, 4 ),
 ( 0.000000000000000000, 0.1333490885032282969, 0.3007194338854215498, 0.4699862290245004903, 0.5844252810809279497, 0.6686540514502673505, 0.7354980260655414881, 0.8028463152565613603, 0.8633854507757170449, 0.9437142632667081532, 1.000000000000000000 ),
 .UNSPECIFIED. ) ;
#87354=CARTESIAN_POINT ( 'NONE',  ( 34.04545031248176912, 37.84336893147759184, -7.433330006724137462 ) ) ;
#87358=CARTESIAN_POINT ( 'NONE',  ( 32.78250297933140445, 27.43085787977765477, -9.188101187500008038 ) ) ;
#87361=CARTESIAN_POINT ( 'NONE',  ( 66.08627282113103263, 68.62029620053424139, 1.806069293516707974 ) ) ;
#87363=CARTESIAN_POINT ( 'NONE',  ( 42.70400705346037284, 26.78380873178790367, -6.180339887498949025 ) ) ;
#87366=CARTESIAN_POINT ( 'NONE',  ( 4.795442299662375341, 20.95586893147752861, 7.433330006724141015 ) ) ;
#87368=CARTESIAN_POINT ( 'NONE',  ( 17.19404571121151903, 18.43085787977762280, -9.188101187500008038 ) ) ;
#87371=CARTESIAN_POINT ( 'NONE',  ( 84.72693717884534692, 49.96098312850357104, -13.65910992477957819 ) ) ;
#87374=CARTESIAN_POINT ( 'NONE',  ( 32.92963059540232251, 19.41603393254328225, -1.583844403245396437 ) ) ;
#87376=CARTESIAN_POINT ( 'NONE',  ( 66.25406239667182717, 68.20281254162030393, 4.159574302714934113 ) ) ;
#87377=CARTESIAN_POINT ( 'NONE',  ( 87.29309660270801885, 45.46152261598134459, 7.123530500323841608 ) ) ;
#87380=VERTEX_POINT ( 'NONE', #72233 ) ;
#87382=CARTESIAN_POINT ( 'NONE',  ( 85.88667062683153119, 47.52433287832054276, 10.83178577085193339 ) ) ;
#87384=CARTESIAN_POINT ( 'NONE',  ( 77.20308883393413169, 54.63758335188173731, 16.07556225031585484 ) ) ;
#87387=CARTESIAN_POINT ( 'NONE',  ( 78.39257131096576359, 61.24758009167359063, -15.88576424600291226 ) ) ;
#87398=CARTESIAN_POINT ( 'NONE',  ( 34.80818111321084274, 38.83478043621391151, -8.090169943749479842 ) ) ;
#87399=EDGE_LOOP ( 'NONE', ( #39181, #67894, #9033, #6199 ) ) ;
#87402=ORIENTED_EDGE ( 'NONE', *, *, #38188, .F. ) ;
#87403=PLANE ( 'NONE',  #80051 ) ;
#87404=ORIENTED_EDGE ( 'NONE', *, *, #12283, .F. ) ;
#87409=CARTESIAN_POINT ( 'NONE',  ( 69.44161659878608361, 65.07538059710674361, 11.53483947389128339 ) ) ;
#87417=CARTESIAN_POINT ( 'NONE',  ( 25.05680157815287146, 15.26216523072494624, -2.296566073217252530E-15 ) ) ;
#87425=CARTESIAN_POINT ( 'NONE',  ( 86.78549426258130950, 45.83013854792883990, 8.849882187839872572 ) ) ;
#87429=CARTESIAN_POINT ( 'NONE',  ( 79.14312167556931854, 57.64441083166269664, 0.000000000000000000 ) ) ;
#87436=CARTESIAN_POINT ( 'NONE',  ( 82.55952464939674940, 40.51136557279177453, -1.425512534736172565 ) ) ;
#87445=CARTESIAN_POINT ( 'NONE',  ( 68.00113622733728391, 69.59165091443878737, 2.730665754880787333 ) ) ;
#87446=DIRECTION ( 'NONE',  ( 0.000000000000000000, -0.4385670422228005183, 0.8986984752829750844 ) ) ;
#87450=CARTESIAN_POINT ( 'NONE',  ( 74.47004568639763988, 68.24076931554098735, -11.48438178457268855 ) ) ;
#87453=EDGE_LOOP ( 'NONE', ( #48435, #24368, #55738, #18638, #19466 ) ) ;
#87454=CARTESIAN_POINT ( 'NONE',  ( 84.02477065797984324, 47.37122689846454904, 11.56964593643152739 ) ) ;
#87469=CARTESIAN_POINT ( 'NONE',  ( 17.24455747906367264, 28.14336893147755347, 7.433330006724141015 ) ) ;
#87470=CARTESIAN_POINT ( 'NONE',  ( 75.22042510487506206, 66.98545636449729557, 12.77795336576078356 ) ) ;
#87481=CARTESIAN_POINT ( 'NONE',  ( 81.54078422002766047, 55.47956193386177404, -16.32023236213573369 ) ) ;
#87485=CARTESIAN_POINT ( 'NONE',  ( 79.98829826350832661, 44.59498145193617802, 11.76229303994366049 ) ) ;
#87486=CARTESIAN_POINT ( 'NONE',  ( 80.29398387428507533, 55.37432886148820188, 16.01591544229163944 ) ) ;
#87488=CARTESIAN_POINT ( 'NONE',  ( 72.34691042023506213, 71.90931229659582868, -5.260778230539377098 ) ) ;
#87491=ORIENTED_EDGE ( 'NONE', *, *, #57998, .T. ) ;
#87492=CARTESIAN_POINT ( 'NONE',  ( 85.04793144752864009, 49.76842598555754194, 13.42690168825989439 ) ) ;
#87493=B_SPLINE_SURFACE_WITH_KNOTS ( 'NONE', 3, 1, ( 
 ( #28458, #23219 ),
 ( #36551, #5663 ),
 ( #8045, #90317 ),
 ( #98386, #67458 ),
 ( #90816, #51778 ),
 ( #28977, #46511 ),
 ( #97393, #82719 ),
 ( #77449, #51255 ),
 ( #69823, #52255 ),
 ( #83197, #54108 ),
 ( #13287, #38918 ),
 ( #75573, #66469 ),
 ( #7522, #82221 ),
 ( #31323, #12794 ),
 ( #38415, #20383 ),
 ( #69330, #43146 ),
 ( #44148, #89810 ),
 ( #434, #89337 ),
 ( #100251, #19889 ),
 ( #50760, #5174 ),
 ( #12286, #74087 ),
 ( #4679, #35569 ),
 ( #27961, #17641 ),
 ( #48539, #87611 ),
 ( #62210, #2450 ),
 ( #79478, #71348 ),
 ( #85590, #16131 ),
 ( #1939, #54607 ),
 ( #70837, #18139 ),
 ( #48021, #49039 ),
 ( #64229, #56628 ) ),
 .UNSPECIFIED., .F., .F., .F.,
 ( 4, 3, 3, 3, 3, 3, 3, 3, 3, 3, 4 ),
 ( 2, 2 ),
 ( 0.000000000000000000, 0.1333490885032384554, 0.3007194338854541904, 0.4699862290245523377, 0.5844252810809684728, 0.6686540514502963273, 0.7354980260655706870, 0.8028463152565942229, 0.8633854507757449115, 0.9437142632667596676, 1.000000000000000000 ),
 ( 0.000000000000000000, 1.000000000000000000 ),
 .UNSPECIFIED. ) ;
#87494=CARTESIAN_POINT ( 'NONE',  ( 37.70440764347101492, 39.95586893147758900, 7.433330006724141015 ) ) ;
#87497=CARTESIAN_POINT ( 'NONE',  ( 77.72205534048291042, 61.52847525230063042, 16.09962475150207339 ) ) ;
#87501=CARTESIAN_POINT ( 'NONE',  ( 79.35100834308954632, 59.73271264539057057, 16.51943372556190326 ) ) ;
#87506=CARTESIAN_POINT ( 'NONE',  ( 80.32950597564698114, 44.91110509010904650, 11.18754419191202842 ) ) ;
#87513=CARTESIAN_POINT ( 'NONE',  ( 77.28211008475351207, 49.15284714648134923, -15.31460611935377614 ) ) ;
#87515=CARTESIAN_POINT ( 'NONE',  ( 74.52921011339299184, 56.62722107306336738, 16.07648648383083057 ) ) ;
#87516=CARTESIAN_POINT ( 'NONE',  ( 79.35712722355306425, 54.04372616740326407, 15.87919829441960395 ) ) ;
#87519=B_SPLINE_CURVE_WITH_KNOTS ( 'NONE', 3,
 ( #20491, #58940, #28067, #12900, #97985, #58459, #81816, #52358, #28563, #43756, #35168, #98493, #59950, #66079, #75680, #51362, #90921, #90425, #36654, #89433, #20998, #67062, #73686, #74202, #12392, #66573, #81323, #13385, #89911, #97499, #97025, #57973, #43257, #11895, #42752, #21471, #44255, #74700, #88957, #5279, #96520, #4792, #4270, #19512, #29085, #13867 ),
 .UNSPECIFIED., .F., .F.,
 ( 4, 1, 2, 2, 1, 2, 2, 1, 1, 2, 2, 1, 1, 2, 2, 1, 1, 2, 2, 1, 1, 1, 2, 2, 1, 1, 1, 2, 2, 4 ),
 ( 0.000000000000000000, 0.06249999999999743261, 0.09374999999999712730, 0.1249999999999968359, 0.1874999999999944766, 0.2187499999999914790, 0.2499999999999884814, 0.3124999999999819589, 0.3437499999999775735, 0.3593749999999752420, 0.3749999999999729661, 0.4374999999999674150, 0.4687499999999651390, 0.4843749999999640288, 0.4999999999999628630, 0.5624999999999517053, 0.5937499999999452660, 0.6093749999999420464, 0.6249999999999387157, 0.6874999999999311662, 0.7187499999999272804, 0.7343749999999259481, 0.7421874999999252820, 0.7499999999999247269, 0.8124999999999363842, 0.8437499999999431566, 0.8593749999999458211, 0.8671874999999463762, 0.8749999999999469313, 1.000000000000000000 ),
 .UNSPECIFIED. ) ;
#87520=CARTESIAN_POINT ( 'NONE',  ( 81.93012584742906768, 41.13374663330952785, 3.753794840019959889 ) ) ;
#87529=ORIENTED_EDGE ( 'NONE', *, *, #78743, .T. ) ;
#87531=ORIENTED_EDGE ( 'NONE', *, *, #72190, .T. ) ;
#87532=ORIENTED_EDGE ( 'NONE', *, *, #66448, .T. ) ;
#87545=CARTESIAN_POINT ( 'NONE',  ( 65.97972133490638669, 68.67132386035298452, -0.2592375539653856698 ) ) ;
#87546=VERTEX_POINT ( 'NONE', #79856 ) ;
#87550=DIRECTION ( 'NONE',  ( 0.5000000000000013323, -0.8660254037844378194, 0.000000000000000000 ) ) ;
#87555=ORIENTED_EDGE ( 'NONE', *, *, #31701, .T. ) ;
#87557=CARTESIAN_POINT ( 'NONE',  ( 74.91474539609477290, 61.54304851710285362, -15.22267036536665330 ) ) ;
#87560=CARTESIAN_POINT ( 'NONE',  ( 74.43453170551926235, 65.24630961380456995, -13.55578908557625972 ) ) ;
#87564=CARTESIAN_POINT ( 'NONE',  ( 80.62015840900424735, 43.33333764377209008, -9.369712834007803082 ) ) ;
#87569=CARTESIAN_POINT ( 'NONE',  ( 88.07467786089314643, 44.31731248180877714, -4.422775558719206579 ) ) ;
#87572=EDGE_CURVE ( 'NONE', #30496, #48220, #72064, .T. ) ;
#87580=EDGE_CURVE ( 'NONE', #69750, #32340, #62331, .T. ) ;
#87583=CARTESIAN_POINT ( 'NONE',  ( 81.01231947336798100, 53.36392349131256196, -15.94611761156046192 ) ) ;
#87584=CARTESIAN_POINT ( 'NONE',  ( 66.48085443433819819, 68.27321713501613942, -4.336635036640815954 ) ) ;
#87590=DIRECTION ( 'NONE',  ( 0.5000000000000014433, -0.8660254037844378194, 0.000000000000000000 ) ) ;
#87594=CARTESIAN_POINT ( 'NONE',  ( 30.44305165777243971, 40.68290643055189548, 3.479690158560446702E-15 ) ) ;
#87598=CARTESIAN_POINT ( 'NONE',  ( 18.31506083472495661, 16.28920272979926054, -7.433330006724141015 ) ) ;
#87600=CARTESIAN_POINT ( 'NONE',  ( 76.51987890029035100, 63.61070592637643983, 14.91914813192732403 ) ) ;
#87605=CARTESIAN_POINT ( 'NONE',  ( 86.10659305072458380, 47.03284479452093336, 10.73441527774546245 ) ) ;
#87609=CARTESIAN_POINT ( 'NONE',  ( 74.90174054662361414, 53.21786585885936915, 16.51862851041579461 ) ) ;
#87611=CARTESIAN_POINT ( 'NONE',  ( 82.14148480337546232, 54.17133474984891706, 15.63111399271332047 ) ) ;
#87623=EDGE_CURVE ( 'NONE', #51674, #69479, #75648, .T. ) ;
#87624=CARTESIAN_POINT ( 'NONE',  ( 33.10965510200716722, 34.51421378149920827, -9.188101187500004485 ) ) ;
#87625=CARTESIAN_POINT ( 'NONE',  ( 84.86548878997092515, 50.26520129761993871, -13.37165312599878320 ) ) ;
#87626=CARTESIAN_POINT ( 'NONE',  ( 86.00921005490911853, 47.65307992534832948, -10.85841856809923378 ) ) ;
#87636=CARTESIAN_POINT ( 'NONE',  ( 81.65607015944604541, 55.82719893760320673, -16.00789492171315942 ) ) ;
#87639=CARTESIAN_POINT ( 'NONE',  ( 70.63617790867836277, 60.90204785445763491, 15.02499658488835443 ) ) ;
#87647=CARTESIAN_POINT ( 'NONE',  ( 77.77867966053455007, 61.43039905302717330, -16.12786080876372807 ) ) ;
#87651=CARTESIAN_POINT ( 'NONE',  ( 80.01822028430966327, 44.43016943383536699, -11.60302980327384859 ) ) ;
#87657=EDGE_CURVE ( 'NONE', #93313, #63730, #23775, .T. ) ;
#87663=CARTESIAN_POINT ( 'NONE',  ( 75.87525401958798454, 64.72722897157592570, -14.29033900848947525 ) ) ;
#87667=CARTESIAN_POINT ( 'NONE',  ( 87.86423278622298483, 44.30858544867225390, 4.762156274856222282 ) ) ;
#87668=ORIENTED_EDGE ( 'NONE', *, *, #30604, .F. ) ;
#87669=CARTESIAN_POINT ( 'NONE',  ( 86.65373920060009993, 43.97555830415484479, -4.434315822418210651 ) ) ;
#87672=CARTESIAN_POINT ( 'NONE',  ( 82.01519968974108110, 40.98639441602998801, -2.953312919879617304 ) ) ;
#87680=CARTESIAN_POINT ( 'NONE',  ( 85.35261164803672784, 44.05229582933603183, 6.432725872221583430 ) ) ;
#87682=CARTESIAN_POINT ( 'NONE',  ( 77.79577372677249514, 62.02059634206501926, 15.64361606394993842 ) ) ;
#87685=EDGE_CURVE ( 'NONE', #10543, #36817, #25339, .T. ) ;
#87686=ORIENTED_EDGE ( 'NONE', *, *, #30362, .F. ) ;
#87687=CARTESIAN_POINT ( 'NONE',  ( 27.17098259457989684, 39.18528772668521043, -1.583844403245329602 ) ) ;
#87692=CARTESIAN_POINT ( 'NONE',  ( 86.98925081226386169, 46.40596221211884398, -8.809588356812493970 ) ) ;
#87693=CARTESIAN_POINT ( 'NONE',  ( 38.34546801798370552, 23.10801979619931501, 3.090169943749476733 ) ) ;
#87697=CARTESIAN_POINT ( 'NONE',  ( 84.81921465843747399, 43.36599167773228203, -5.564511731166422948 ) ) ;
#87702=CARTESIAN_POINT ( 'NONE',  ( 87.10409928669704982, 46.39511029792537045, 8.719520416454489720 ) ) ;
#87705=CARTESIAN_POINT ( 'NONE',  ( 82.10990542498430500, 41.84899041517287088, 5.504228460268151046 ) ) ;
#87709=CARTESIAN_POINT ( 'NONE',  ( 42.70400705346036574, 26.78380873178790367, -6.180339887498949025 ) ) ;
#87714=CARTESIAN_POINT ( 'NONE',  ( 15.56473500984127512, 9.390406791769814632, -7.779800476318352071E-15 ) ) ;
#87715=CARTESIAN_POINT ( 'NONE',  ( 87.13594473370017113, 46.33577775587144032, -8.608104698120229159 ) ) ;
#87718=CARTESIAN_POINT ( 'NONE',  ( 69.46904662810460707, 66.79780009071521363, -9.892305524425870189 ) ) ;
#87719=CARTESIAN_POINT ( 'NONE',  ( 39.48212635690286021, 23.76426979415093044, 3.090169943749476733 ) ) ;
#87730=CARTESIAN_POINT ( 'NONE',  ( 72.73830096649396637, 70.17554807097293690, 8.869713815284775649 ) ) ;
#87731=CARTESIAN_POINT ( 'NONE',  ( 27.26159103020561147, 24.24335787977764767, -9.188101187500008038 ) ) ;
#87736=CARTESIAN_POINT ( 'NONE',  ( 12.16147613323643029, 27.99752408145590721, 5.678558825948276656 ) ) ;
#87738=CARTESIAN_POINT ( 'NONE',  ( 87.78081971166569986, 44.10618430004836910, 2.676874261813567468 ) ) ;
#87742=CARTESIAN_POINT ( 'NONE',  ( 79.14312167556931854, 57.64441083166269664, 0.000000000000000000 ) ) ;
#87743=CARTESIAN_POINT ( 'NONE',  ( 76.32984284614508397, 63.49129372016874839, -15.29838449762297614 ) ) ;
#87745=ORIENTED_EDGE ( 'NONE', *, *, #24516, .F. ) ;
#87748=CARTESIAN_POINT ( 'NONE',  ( 16.72324493992723049, 11.78380873178785748, -6.180339887498949025 ) ) ;
#87751=CARTESIAN_POINT ( 'NONE',  ( 72.09461912472968947, 72.35512880999853280, -3.358616764072534178 ) ) ;
#87752=CARTESIAN_POINT ( 'NONE',  ( 72.72402067594053676, 57.21056264940069269, -15.87973078800185966 ) ) ;
#87753=CARTESIAN_POINT ( 'NONE',  ( 78.26014935871903333, 61.04899649461657418, -15.91113552180851620 ) ) ;
#87759=ORIENTED_EDGE ( 'NONE', *, *, #56731, .F. ) ;
#87761=ORIENTED_EDGE ( 'NONE', *, *, #13845, .F. ) ;
#87762=CARTESIAN_POINT ( 'NONE',  ( 40.27059248445925732, 25.11110640527295601, -2.839279412974138328 ) ) ;
#87767=CARTESIAN_POINT ( 'NONE',  ( 74.41176536287696308, 68.30213538679808494, 11.38880159922067747 ) ) ;
#87773=CARTESIAN_POINT ( 'NONE',  ( 76.57256817690921480, 57.91657040172975712, -16.10350934941853041 ) ) ;
#87774=CARTESIAN_POINT ( 'NONE',  ( 83.57479903228094997, 42.82924647053130229, -5.872390686928415704 ) ) ;
#87779=CARTESIAN_POINT ( 'NONE',  ( 68.22269823808483125, 69.38605919497339869, -4.074953496159504418 ) ) ;
#87785=CARTESIAN_POINT ( 'NONE',  ( 75.51323141522172477, 65.35427051582675517, 13.87231131232226744 ) ) ;
#87790=CARTESIAN_POINT ( 'NONE',  ( 84.35801967554498049, 44.16480482089680493, -7.626279337594716878 ) ) ;
#87791=DIRECTION ( 'NONE',  ( 0.5000000000000014433, -0.8660254037844378194, 0.000000000000000000 ) ) ;
#87794=CARTESIAN_POINT ( 'NONE',  ( 74.90473642350332284, 61.75549325437163617, 15.17546568179592725 ) ) ;
#87797=CARTESIAN_POINT ( 'NONE',  ( 80.31886729598942054, 57.42767889257750369, -16.58902572440456780 ) ) ;
#87800=CARTESIAN_POINT ( 'NONE',  ( 72.07793231134587586, 71.39460431499534820, 5.116661974763394127 ) ) ;
#87802=CARTESIAN_POINT ( 'NONE',  ( 71.50240432004942193, 72.40933122983058468, 5.654570818603106787E-06 ) ) ;
#87804=EDGE_CURVE ( 'NONE', #14885, #40695, #87925, .T. ) ;
#87805=CARTESIAN_POINT ( 'NONE',  ( 67.74046153704668427, 68.49183975612825748, 5.712584250058917235 ) ) ;
#87808=B_SPLINE_CURVE_WITH_KNOTS ( 'NONE', 3,
 ( #25720, #79452, #79947, #88071, #15715, #32800, #72835, #78935, #3428, #64715, #46617, #95664, #10511, #10016, #40879, #9522, #41390, #40384, #1915, #46107, #87076, #33302, #72333, #71323, #56081, #41894, #77021, #71826, #64203, #33825, #2937 ),
 .UNSPECIFIED., .F., .F.,
 ( 4, 3, 3, 3, 3, 3, 3, 3, 3, 3, 4 ),
 ( 0.000000000000000000, 0.1333490885032290463, 0.3007194338854137228, 0.4699862290245038765, 0.5844252810809251741, 0.6686540514502686827, 0.7354980260655517021, 0.8028463152565618044, 0.8633854507757415808, 0.9437142632667480102, 1.000000000000000000 ),
 .UNSPECIFIED. ) ;
#87818=CYLINDRICAL_SURFACE ( 'NONE', #14357, 16.60714546451156792 ) ;
#87823=CARTESIAN_POINT ( 'NONE',  ( 23.65144817020273393, 15.78380873178787347, -6.180339887498949025 ) ) ;
#87824=CARTESIAN_POINT ( 'NONE',  ( 85.68485941944548756, 48.66523437743575187, 11.91861461389293808 ) ) ;
#87825=CARTESIAN_POINT ( 'NONE',  ( 66.04572084532792076, 69.25630126843506673, 0.2739672973347200835 ) ) ;
#87828=CARTESIAN_POINT ( 'NONE',  ( 66.54213899643076502, 67.99313125863469054, -6.545993785947124444 ) ) ;
#87833=CARTESIAN_POINT ( 'NONE',  ( 73.27328646083023500, 70.16270934360544231, -9.274526489422589393 ) ) ;
#87834=( BOUNDED_CURVE ( )  B_SPLINE_CURVE ( 2, ( #70128, #69641, #31129, #92973, #39713, #70641, #85394, #55420, #46845, #77767, #8352, #16938, #47824 ),
 .UNSPECIFIED., .F., .T. ) 
 B_SPLINE_CURVE_WITH_KNOTS ( ( 3, 2, 2, 2, 2, 2, 3 ),
 ( 0.1375000000000000111, 0.1400000000000000133, 0.1449999999999999900, 0.1499999999999999944, 0.1549999999999999989, 0.1600000000000000033, 0.1625000000000000056 ),
 .UNSPECIFIED. ) 
 CURVE ( )  GEOMETRIC_REPRESENTATION_ITEM ( )  RATIONAL_B_SPLINE_CURVE ( ( 0.9755282581475768211, 0.9755282581475768211, 1.000000000000000000, 0.9510565162951535312, 1.000000000000000000, 0.9510565162951535312, 1.000000000000000000, 0.9510565162951535312, 1.000000000000000000, 0.9510565162951535312, 1.000000000000000000, 0.9755282581475768211, 0.9755282581475768211 ) ) 
 REPRESENTATION_ITEM ( '' )  );
#87840=CARTESIAN_POINT ( 'NONE',  ( 32.39518414388500389, 34.10171378149920685, 9.188101187500008038 ) ) ;
#87843=CARTESIAN_POINT ( 'NONE',  ( 37.97865540203802937, 30.43085787977766188, -9.188101187500008038 ) ) ;
#87846=CARTESIAN_POINT ( 'NONE',  ( 66.30954113569532637, 68.28728378170326607, 3.992301261007330737 ) ) ;
#87849=CARTESIAN_POINT ( 'NONE',  ( 7.976297994771393896, 26.64646525600388571, -2.839279412974133887 ) ) ;
#87851=CARTESIAN_POINT ( 'NONE',  ( 17.79544559245429625, 15.98920272979925628, 7.433330006724137462 ) ) ;
#87855=CARTESIAN_POINT ( 'NONE',  ( 88.20990559483804816, 44.21161532246393477, -1.798209583089680041 ) ) ;
#87859=LINE ( 'NONE', #64996, #63903 ) ;
#87860=CARTESIAN_POINT ( 'NONE',  ( 87.34977546134365411, 44.90968568749347867, 6.842696035241847774 ) ) ;
#87865=CARTESIAN_POINT ( 'NONE',  ( 86.07940076415255248, 47.67293344237150166, 10.86953268328462308 ) ) ;
#87866=ORIENTED_EDGE ( 'NONE', *, *, #94384, .T. ) ;
#87867=CARTESIAN_POINT ( 'NONE',  ( 76.78470638831343820, 52.79280447672221044, 15.85451643790141141 ) ) ;
#87869=EDGE_LOOP ( 'NONE', ( #35067, #80885, #68608, #19659 ) ) ;
#87870=CARTESIAN_POINT ( 'NONE',  ( 78.27822849507501246, 61.67779232024188474, -15.77509627637905432 ) ) ;
#87872=CARTESIAN_POINT ( 'NONE',  ( 16.78929260308981952, 21.64441083166260427, -10.00000000000000533 ) ) ;
#87882=EDGE_CURVE ( 'NONE', #85116, #43189, #69715, .T. ) ;
#87886=EDGE_CURVE ( 'NONE', #76398, #7306, #41906, .T. ) ;
#87900=CARTESIAN_POINT ( 'NONE',  ( 16.63655203261577498, 31.64646525600389637, -2.839279412974133887 ) ) ;
#87903=CARTESIAN_POINT ( 'NONE',  ( 77.54655217216907204, 49.73132247284985397, -15.46410396994591530 ) ) ;
#87910=CARTESIAN_POINT ( 'NONE',  ( 35.87562414229657293, 44.21091486745863364, 7.012934429366973338E-14 ) ) ;
#87921=CARTESIAN_POINT ( 'NONE',  ( 82.56903123641447451, 41.04314473016881237, -1.144421423674383265 ) ) ;
#87925=B_SPLINE_CURVE_WITH_KNOTS ( 'NONE', 3,
 ( #74844, #52502, #82958, #59087, #83451, #14018, #68202, #92063, #90061, #20630, #99129, #14520, #45402, #61092, #5424, #76332, #6905, #44400, #46902, #16500, #62583, #55480, #23585, #39280, #24099, #54478, #9407, #25093, #8901, #69700, #308 ),
 .UNSPECIFIED., .F., .F.,
 ( 4, 3, 3, 3, 3, 3, 3, 3, 3, 3, 4 ),
 ( 0.000000000000000000, 0.1333490885032302675, 0.3007194338854343174, 0.4699862290245060414, 0.5844252810809307253, 0.6686540514502736787, 0.7354980260655518132, 0.8028463152565562533, 0.8633854507757269259, 0.9437142632667357978, 1.000000000000000000 ),
 .UNSPECIFIED. ) ;
#87930=CARTESIAN_POINT ( 'NONE',  ( 74.39670515357231295, 68.40078795844485171, -11.29786485497992921 ) ) ;
#87932=CARTESIAN_POINT ( 'NONE',  ( 82.99579283926775020, 42.25164479318972610, 5.310766221622300165 ) ) ;
#87936=CARTESIAN_POINT ( 'NONE',  ( 6.599962460801562791, 15.76159833115048770, -9.594050593750004907 ) ) ;
#87940=CARTESIAN_POINT ( 'NONE',  ( 81.65310433048475147, 42.64019311979919280, 7.560891536010023728 ) ) ;
#87956=CARTESIAN_POINT ( 'NONE',  ( 15.22926075146606273, 30.83396525600389637, -2.839279412974133887 ) ) ;
#87957=CARTESIAN_POINT ( 'NONE',  ( 75.15861105040980306, 67.07800672539922004, 12.69370984594314322 ) ) ;
#87968=CARTESIAN_POINT ( 'NONE',  ( 81.76698870106028494, 55.35579676949175365, -15.92943682233255132 ) ) ;
#87974=CARTESIAN_POINT ( 'NONE',  ( 83.70712025649116583, 51.47757175601724811, -14.37168843583688194 ) ) ;
#87975=CARTESIAN_POINT ( 'NONE',  ( 72.27803260052462520, 71.63036165027699553, -5.844549976855538453 ) ) ;
#87977=ORIENTED_EDGE ( 'NONE', *, *, #40844, .F. ) ;
#87979=CARTESIAN_POINT ( 'NONE',  ( 11.39908531360041088, 14.78052372038638929, -10.00000000000000355 ) ) ;
#87981=EDGE_LOOP ( 'NONE', ( #39336, #86598, #95590, #66858 ) ) ;
#87984=CARTESIAN_POINT ( 'NONE',  ( 86.33534873861279380, 44.01410524257547507, -6.217298191315958178 ) ) ;
#87985=ORIENTED_EDGE ( 'NONE', *, *, #39011, .F. ) ;
#87986=CARTESIAN_POINT ( 'NONE',  ( 78.71329144889060103, 59.90182516230142795, 16.12092670603864875 ) ) ;
#87987=PLANE ( 'NONE',  #54021 ) ;
#87989=CARTESIAN_POINT ( 'NONE',  ( 80.18538372971539729, 51.32048852683736584, -15.03707885865879135 ) ) ;
#87990=CARTESIAN_POINT ( 'NONE',  ( 73.43921776615482599, 70.07059797397528200, -9.512040028895288657 ) ) ;
#87993=ORIENTED_EDGE ( 'NONE', *, *, #20478, .T. ) ;
#88005=CARTESIAN_POINT ( 'NONE',  ( 81.98366634404946751, 41.07155685126597433, 3.381361522722056367 ) ) ;
#88014=CARTESIAN_POINT ( 'NONE',  ( 70.86275222855024936, 61.11972120349191329, -14.45886437636409916 ) ) ;
#88015=CARTESIAN_POINT ( 'NONE',  ( 6.802937163926562114, 15.87878583063839066, -9.188101187500006262 ) ) ;
#88017=CARTESIAN_POINT ( 'NONE',  ( 85.61207876059154387, 48.93336676014416753, -12.63415981529851173 ) ) ;
#88027=CARTESIAN_POINT ( 'NONE',  ( 16.89228056887236917, 28.49103043416548786, -8.090169943749479842 ) ) ;
#88031=CARTESIAN_POINT ( 'NONE',  ( 66.03170575037515277, 68.70116307984658022, -0.02812428434925291418 ) ) ;
#88040=DIRECTION ( 'NONE',  ( 0.3715724127386967335, -0.6435822975543782354, -0.6691306063588567943 ) ) ;
#88041=CARTESIAN_POINT ( 'NONE',  ( 87.94262069806690363, 44.22295065580315310, 2.813175635398602825 ) ) ;
#88045=CARTESIAN_POINT ( 'NONE',  ( 71.02243149778057330, 62.59254995015435696, -13.81378205064200415 ) ) ;
#88046=CARTESIAN_POINT ( 'NONE',  ( 80.52088211617494551, 57.79340230469777850, 16.24652106404656138 ) ) ;
#88049=CARTESIAN_POINT ( 'NONE',  ( 80.75062256945429340, 43.57525148357456857, -9.564875268673995734 ) ) ;
#88054=CARTESIAN_POINT ( 'NONE',  ( 88.18084728802688232, 44.43898297010869669, -4.607830584147581732 ) ) ;
#88055=CARTESIAN_POINT ( 'NONE',  ( 2.966658798487924908, 25.21091486745858035, 1.000260061240931054E-15 ) ) ;
#88058=CARTESIAN_POINT ( 'NONE',  ( 77.29821696115968166, 51.33252059662452638, 15.49558435715045945 ) ) ;
#88063=DIRECTION ( 'NONE',  ( -0.8660254037844378194, -0.5000000000000013323, -0.000000000000000000 ) ) ;
#88065=CARTESIAN_POINT ( 'NONE',  ( 81.58661138081841102, 53.69171030639404307, -15.56960227015292197 ) ) ;
#88066=CARTESIAN_POINT ( 'NONE',  ( 79.25417529428960961, 46.14802681996067690, -13.25003384320201683 ) ) ;
#88068=CARTESIAN_POINT ( 'NONE',  ( 73.34110816220993456, 69.83660377678546638, 9.135763230745686414 ) ) ;
#88071=CARTESIAN_POINT ( 'NONE',  ( 76.90757676121016573, 64.01000647765765450, -15.22607040013521029 ) ) ;
#88075=CARTESIAN_POINT ( 'NONE',  ( 82.28500086614531028, 51.41804074472770480, -15.07771380314018295 ) ) ;
#88076=FACE_OUTER_BOUND ( 'NONE', #22673, .T. ) ;
#88080=CARTESIAN_POINT ( 'NONE',  ( 85.71737152317884068, 47.69513843210439319, -11.59802438570544858 ) ) ;
#88082=CARTESIAN_POINT ( 'NONE',  ( 22.55376741186237055, 15.94754757982089544, 5.678558825948272215 ) ) ;
#88084=CARTESIAN_POINT ( 'NONE',  ( 76.52245355297571905, 63.63306135144966902, 14.91177216842233477 ) ) ;
#88092=CARTESIAN_POINT ( 'NONE',  ( 72.54789201874723403, 71.57418066018787783, 5.334923225846505801 ) ) ;
#88097=CARTESIAN_POINT ( 'NONE',  ( 85.33078790130267066, 46.00342033433972233, 9.479200480945582541 ) ) ;
#88110=CARTESIAN_POINT ( 'NONE',  ( 35.07444006175263240, 22.11110640527294535, -2.839279412974138328 ) ) ;
#88111=CARTESIAN_POINT ( 'NONE',  ( 77.75401164654779507, 49.70357266593546797, -14.90152202399484160 ) ) ;
#88127=EDGE_CURVE ( 'NONE', #50908, #26854, #15364, .T. ) ;
#88134=ORIENTED_EDGE ( 'NONE', *, *, #10502, .T. ) ;
#88136=CARTESIAN_POINT ( 'NONE',  ( 79.95079703291114015, 44.75747180391820024, -11.24531851929095083 ) ) ;
#88138=CARTESIAN_POINT ( 'NONE',  ( 82.70475790854101206, 41.40672355988375841, -3.064047408685779406 ) ) ;
#88149=CARTESIAN_POINT ( 'NONE',  ( 73.30483403957811106, 69.17932697374328654, -9.895411455429695025 ) ) ;
#88153=CARTESIAN_POINT ( 'NONE',  ( 88.05492707984328149, 44.74075123808635368, 4.463746458969096054 ) ) ;
#88157=CARTESIAN_POINT ( 'NONE',  ( 82.03757150437812129, 40.99183643444361991, -2.920132542340025950 ) ) ;
#88160=CARTESIAN_POINT ( 'NONE',  ( 72.46511837996449401, 71.56249752072032777, 6.234640293157917235 ) ) ;
#88165=CARTESIAN_POINT ( 'NONE',  ( 82.89553795050942142, 41.40690226224887738, 2.584278410276873217 ) ) ;
#88167=CARTESIAN_POINT ( 'NONE',  ( 83.37296956034946049, 51.74080471427828343, 14.95189368521468154 ) ) ;
#88169=B_SPLINE_CURVE_WITH_KNOTS ( 'NONE', 3,
 ( #92929, #93441, #15893, #16399, #6312, #63998, #47782, #72119, #57391, #78216, #25502, #17918, #95953, #80246, #70596, #48816 ),
 .UNSPECIFIED., .F., .F.,
 ( 4, 1, 2, 2, 2, 1, 2, 2, 4 ),
 ( 0.000000000000000000, 0.1249999999999958367, 0.1874999999999937550, 0.2499999999999916733, 0.4999999999999926725, 0.6249999999999928946, 0.6874999999999948930, 0.7499999999999967804, 1.000000000000000000 ),
 .UNSPECIFIED. ) ;
#88173=CARTESIAN_POINT ( 'NONE',  ( 73.78779888375932217, 64.08313911669114304, -13.94799677262989768 ) ) ;
#88174=CARTESIAN_POINT ( 'NONE',  ( 74.22098529628976848, 55.36760511359434389, 16.12280093334807063 ) ) ;
#88175=DIRECTION ( 'NONE',  ( 0.2649596321166021728, -0.4589235447807153423, -0.8480480961564252906 ) ) ;
#88177=CARTESIAN_POINT ( 'NONE',  ( 33.26462506102002692, 34.90829794293883026, 10.00000000000000355 ) ) ;
#88178=CARTESIAN_POINT ( 'NONE',  ( 78.07878065217096264, 47.77350909806117585, 13.99880554328534110 ) ) ;
#88180=CARTESIAN_POINT ( 'NONE',  ( 84.89744547285587828, 41.79037650531964943, -3.168800655305855967E-06 ) ) ;
#88181=CARTESIAN_POINT ( 'NONE',  ( 87.56744345830549037, 43.91593491218741718, -2.248609772235193649 ) ) ;
#88183=CARTESIAN_POINT ( 'NONE',  ( 82.98570375819691947, 51.14804373459350728, 14.38639528083483832 ) ) ;
#88186=CARTESIAN_POINT ( 'NONE',  ( 86.67787608365236451, 46.41355258656824390, 9.087135552152110662 ) ) ;
#88187=CARTESIAN_POINT ( 'NONE',  ( 24.18060153781336297, 14.36477965099640564, 1.583844403245364907 ) ) ;
#88189=CARTESIAN_POINT ( 'NONE',  ( 87.29394575703194903, 46.02912284201620707, 8.718719511823859847 ) ) ;
#88191=CARTESIAN_POINT ( 'NONE',  ( 32.15421140596747307, 42.65659080271453263, -1.878358725466461243E-16 ) ) ;
#88197=CARTESIAN_POINT ( 'NONE',  ( 86.80242440116035141, 45.86160641078058831, -8.224216122728513767 ) ) ;
#88202=CARTESIAN_POINT ( 'NONE',  ( 75.24955243259913118, 53.08423708156048093, 16.48597916460597901 ) ) ;
#88214=CARTESIAN_POINT ( 'NONE',  ( 33.34238925418374322, 21.11110640527294180, -2.839279412974138328 ) ) ;
#88219=CARTESIAN_POINT ( 'NONE',  ( 18.76490627030545610, 13.76004757982088655, 5.678558825948272215 ) ) ;
#88234=CARTESIAN_POINT ( 'NONE',  ( 69.88883377749583303, 71.12950566994834389, -3.160072888935177460 ) ) ;
#88236=CARTESIAN_POINT ( 'NONE',  ( 35.65891684237409720, 42.36126292948898708, 6.180339887498949913 ) ) ;
#88238=CARTESIAN_POINT ( 'NONE',  ( 72.74315697103594403, 57.58733809446825092, -16.30555998160541264 ) ) ;
#88239=CARTESIAN_POINT ( 'NONE',  ( 77.91028351001615704, 61.39461664896379034, -16.15133184208620420 ) ) ;
#88249=CARTESIAN_POINT ( 'NONE',  ( 35.92184506804998279, 29.24335787977765477, -9.188101187500008038 ) ) ;
#88251=CARTESIAN_POINT ( 'NONE',  ( 71.76089672477446868, 70.71256120569563564, -7.122520486804837958 ) ) ;
#88254=CARTESIAN_POINT ( 'NONE',  ( 73.77070425341645432, 68.39923094797843817, 10.98015304846415141 ) ) ;
#88259=CARTESIAN_POINT ( 'NONE',  ( 73.16301214023302180, 58.99354537464945025, -15.59469135662974537 ) ) ;
#88260=CARTESIAN_POINT ( 'NONE',  ( 78.83027756516089823, 59.16041374580647272, 16.54524128708894537 ) ) ;
#88265=LINE ( 'NONE', #34498, #35130 ) ;
#88267=VECTOR ( 'NONE', #2206, 1000.000000000000114 ) ;
#88268=PLANE ( 'NONE',  #69302 ) ;
#88269=CARTESIAN_POINT ( 'NONE',  ( 75.52043138733441197, 65.40259152114373364, 13.85004969525200380 ) ) ;
#88275=CARTESIAN_POINT ( 'NONE',  ( 83.46551755975433196, 44.18061934712438443, -8.403307044377809731 ) ) ;
#88281=VERTEX_POINT ( 'NONE', #23467 ) ;
#88282=CARTESIAN_POINT ( 'NONE',  ( 80.21108484470566680, 57.40951183915923650, -16.59077246605596301 ) ) ;
#88285=CARTESIAN_POINT ( 'NONE',  ( 72.05642296158499960, 71.36845324389531697, 5.149965714867518862 ) ) ;
#88291=CARTESIAN_POINT ( 'NONE',  ( 67.70493856312646130, 68.44720612190054965, 5.765748310548177713 ) ) ;
#88295=CARTESIAN_POINT ( 'NONE',  ( 15.25129666230372827, 24.50829794293880326, -10.00000000000000355 ) ) ;
#88299=VECTOR ( 'NONE', #16777, 1000.000000000000227 ) ;
#88303=CARTESIAN_POINT ( 'NONE',  ( 83.93867512875034720, 50.77184042243444395, -13.93002038390009467 ) ) ;
#88307=CARTESIAN_POINT ( 'NONE',  ( 66.48112308386458835, 67.80287055615345082, -6.850275035659466383 ) ) ;
#88312=CARTESIAN_POINT ( 'NONE',  ( 25.03708881625783889, 16.58380873178787240, 6.180339887498953466 ) ) ;
#88317=CARTESIAN_POINT ( 'NONE',  ( 74.02679248361786790, 55.63944272452155815, -16.58679916994908865 ) ) ;
#88323=DIRECTION ( 'NONE',  ( 0.000000000000000000, -0.5247752241695049502, -0.8512408378936280329 ) ) ;
#88330=CARTESIAN_POINT ( 'NONE',  ( 42.15419773769040290, 26.19860640527295814, 2.839279412974134775 ) ) ;
#88333=CARTESIAN_POINT ( 'NONE',  ( 37.28583507901048932, 30.03085787977765975, 9.188101187500006262 ) ) ;
#88334=CARTESIAN_POINT ( 'NONE',  ( 17.15438521794160920, 32.83705186507754092, 3.090169943749475401 ) ) ;
#88339=CARTESIAN_POINT ( 'NONE',  ( 12.93244592517074487, 8.262165230724926701, -2.296566073217252530E-15 ) ) ;
#88341=CARTESIAN_POINT ( 'NONE',  ( 19.81074232005190794, 13.29860640527291693, -2.839279412974138328 ) ) ;
#88352=CARTESIAN_POINT ( 'NONE',  ( 87.11797949770195260, 45.31116807351030218, 7.029999331949805530 ) ) ;
#88353=ORIENTED_EDGE ( 'NONE', *, *, #95552, .F. ) ;
#88358=CARTESIAN_POINT ( 'NONE',  ( 86.40526999274889874, 47.59822202186899176, 10.59880268136866555 ) ) ;
#88360=CARTESIAN_POINT ( 'NONE',  ( 77.55915319031737454, 56.41274902163431904, 16.17439937459049659 ) ) ;
#88363=CARTESIAN_POINT ( 'NONE',  ( 68.81024624021658553, 64.23859217638603525, -11.91047422207082462 ) ) ;
#88364=CARTESIAN_POINT ( 'NONE',  ( 88.49889760693197616, 43.86969135779091999, -0.01036396331279294640 ) ) ;
#88367=CARTESIAN_POINT ( 'NONE',  ( 80.48551130740291626, 43.60439347182430225, 9.783031566464561735 ) ) ;
#88374=ORIENTED_EDGE ( 'NONE', *, *, #47648, .F. ) ;
#88378=EDGE_CURVE ( 'NONE', #47529, #2005, #52655, .T. ) ;
#88394=CARTESIAN_POINT ( 'NONE',  ( 29.15721111571870594, 19.76004757982090965, 5.678558825948272215 ) ) ;
#88397=ORIENTED_EDGE ( 'NONE', *, *, #79289, .T. ) ;
#88400=CARTESIAN_POINT ( 'NONE',  ( 69.46922245526401696, 62.68787098779524314, 13.82297688367849808 ) ) ;
#88410=EDGE_CURVE ( 'NONE', #99877, #35455, #23572, .T. ) ;
#88423=CARTESIAN_POINT ( 'NONE',  ( 87.88902802526534686, 43.91876200309240375, 0.4180276961671919311 ) ) ;
#88425=CARTESIAN_POINT ( 'NONE',  ( 75.96002837510272343, 51.45078221087327108, 16.17316520771503008 ) ) ;
#88433=CARTESIAN_POINT ( 'NONE',  ( 83.52367447683917590, 46.08189511659875848, 10.61866891795677681 ) ) ;
#88436=CARTESIAN_POINT ( 'NONE',  ( 68.66220828135105592, 64.65574856808412108, -12.15835882835606618 ) ) ;
#88439=CARTESIAN_POINT ( 'NONE',  ( 79.62821684406628719, 47.63998313237675575, 14.03196863946704909 ) ) ;
#88448=ADVANCED_FACE ( 'NONE', ( #77583 ), #33802, .T. ) ;
#88451=CARTESIAN_POINT ( 'NONE',  ( 81.87359138893998534, 41.32955797152818889, 5.976920566253458134 ) ) ;
#88453=CARTESIAN_POINT ( 'NONE',  ( 21.16812676580727270, 15.14754757982089650, -5.678558825948276656 ) ) ;
#88454=CARTESIAN_POINT ( 'NONE',  ( 74.86089102438639031, 67.20426264302339803, 12.49187069351280499 ) ) ;
#88456=CARTESIAN_POINT ( 'NONE',  ( 81.74030608389443842, 41.67103928136101842, -5.586802174944530464 ) ) ;
#88464=CARTESIAN_POINT ( 'NONE',  ( 81.76809963683952276, 55.60016907699685618, -15.96690463567013474 ) ) ;
#88466=CARTESIAN_POINT ( 'NONE',  ( 74.50030574182822818, 64.90152822149880762, -14.20405048683398874 ) ) ;
#88469=CARTESIAN_POINT ( 'NONE',  ( 83.69031307077386828, 42.59536443435012387, 5.155235521226168238 ) ) ;
#88470=CARTESIAN_POINT ( 'NONE',  ( 79.53253147591188110, 51.45198067062761993, 15.17816704916131521 ) ) ;
#88472=DIRECTION ( 'NONE',  ( 0.4386133837897754351, 0.6599160945941884293, 0.6100238090894790632 ) ) ;
#88477=CARTESIAN_POINT ( 'NONE',  ( 5.452216952852307230, 26.08080186712590631, -3.090169943749475845 ) ) ;
#88484=CARTESIAN_POINT ( 'NONE',  ( 78.92848498041493599, 59.73641368792644357, 16.49589861780994227 ) ) ;
#88487=ORIENTED_EDGE ( 'NONE', *, *, #42310, .F. ) ;
#88488=CARTESIAN_POINT ( 'NONE',  ( 76.84355992005671965, 52.38483315033376186, -15.78702513624113557 ) ) ;
#88496=ORIENTED_EDGE ( 'NONE', *, *, #57578, .F. ) ;
#88501=CARTESIAN_POINT ( 'NONE',  ( 82.03343428350656552, 41.08618529242319539, 3.321173257777776389 ) ) ;
#88507=CARTESIAN_POINT ( 'NONE',  ( 18.59950357648009955, 34.23654200823202842, 1.583844403245363353 ) ) ;
#88509=ORIENTED_EDGE ( 'NONE', *, *, #10509, .T. ) ;
#88510=CARTESIAN_POINT ( 'NONE',  ( 70.47390418687882629, 61.30276010542613108, -14.81569727497708833 ) ) ;
#88513=VECTOR ( 'NONE', #66798, 1000.000000000000114 ) ;
#88516=AXIS2_PLACEMENT_3D ( 'NONE', #82143, #36477, #53545 ) ;
#88521=CARTESIAN_POINT ( 'NONE',  ( 81.38451658133408273, 39.76220097505215989, 0.000000000000000000 ) ) ;
#88524=CARTESIAN_POINT ( 'NONE',  ( 76.44099679799769831, 51.64620055149545408, -16.15625289873146286 ) ) ;
#88525=CARTESIAN_POINT ( 'NONE',  ( 88.28491662655248717, 43.90562524633402575, -2.137378875048265403 ) ) ;
#88526=ORIENTED_EDGE ( 'NONE', *, *, #21938, .F. ) ;
#88528=CARTESIAN_POINT ( 'NONE',  ( 66.28466101247255438, 68.84525821111240873, 0.1138578521233850477 ) ) ;
#88535=CARTESIAN_POINT ( 'NONE',  ( 82.35285118013293015, 53.50770157854819331, -15.77620284334257938 ) ) ;
#88536=CARTESIAN_POINT ( 'NONE',  ( 88.33437046889027044, 43.98075787490867583, 2.428164790499226733 ) ) ;
#88539=CARTESIAN_POINT ( 'NONE',  ( 74.52678402073020436, 61.66496649313184975, -15.10502237438445228 ) ) ;
#88540=CARTESIAN_POINT ( 'NONE',  ( 80.39194534802405201, 57.98788175658641109, 16.25790314543759152 ) ) ;
#88541=CARTESIAN_POINT ( 'NONE',  ( 73.65091262424760998, 65.48395239458849915, -13.12340454139720514 ) ) ;
#88542=CARTESIAN_POINT ( 'NONE',  ( 82.29734961797254300, 53.60383310410945512, 15.81226994477781211 ) ) ;
#88543=CARTESIAN_POINT ( 'NONE',  ( 80.80860232633280305, 43.61757695342358687, -9.575079427039360880 ) ) ;
#88549=CARTESIAN_POINT ( 'NONE',  ( 88.16744270275496831, 44.54586846255803323, -4.939063992914634937 ) ) ;
#88553=CYLINDRICAL_SURFACE ( 'NONE', #66824, 16.60714546451156792 ) ;
#88559=CARTESIAN_POINT ( 'NONE',  ( 89.87110602656373715, 45.06299687293669365, 0.3596699001693225983 ) ) ;
#88563=CARTESIAN_POINT ( 'NONE',  ( 75.51089968197061353, 55.97360561932201506, -16.15470048074736198 ) ) ;
#88564=DIRECTION ( 'NONE',  ( 0.5000000000000014433, -0.8660254037844378194, 0.000000000000000000 ) ) ;
#88572=CARTESIAN_POINT ( 'NONE',  ( 73.11370943405387379, 57.30880053450761125, 15.89862119264240370 ) ) ;
#88574=CARTESIAN_POINT ( 'NONE',  ( 84.59307794881090103, 43.06915618060124729, -6.352897038551593489 ) ) ;
#88576=CARTESIAN_POINT ( 'NONE',  ( 75.58531661750802755, 65.25623013732912625, 14.34312269817976215 ) ) ;
#88578=CARTESIAN_POINT ( 'NONE',  ( 27.35361640444819287, 37.83396525600391413, -2.839279412974133887 ) ) ;
#88580=CARTESIAN_POINT ( 'NONE',  ( 74.86122976112790184, 57.66712160362105521, 16.46677789332469999 ) ) ;
#88582=CARTESIAN_POINT ( 'NONE',  ( 14.99289142922413021, 26.84336893147755276, -7.433330006724137462 ) ) ;
#88588=CARTESIAN_POINT ( 'NONE',  ( 86.70421956006907749, 47.09494090442339598, 10.43848816880117525 ) ) ;
#88593=CARTESIAN_POINT ( 'NONE',  ( 75.03955294907601115, 53.26399608549274234, 16.03606609946628581 ) ) ;
#88595=CARTESIAN_POINT ( 'NONE',  ( 85.73923958617189101, 47.08247690321802281, 10.46103602312257586 ) ) ;
#88601=CARTESIAN_POINT ( 'NONE',  ( 77.27195188805879411, 63.42260127183214991, -15.13583386105102058 ) ) ;
#88608=CARTESIAN_POINT ( 'NONE',  ( 29.64555348686940661, 32.51421378149921537, -9.188101187500004485 ) ) ;
#88609=CARTESIAN_POINT ( 'NONE',  ( 73.61114153562050433, 60.42089198535372674, -15.30486817249622256 ) ) ;
#88617=CARTESIAN_POINT ( 'NONE',  ( 85.76129479494518648, 48.67511999704337455, -11.90588009047172235 ) ) ;
#88634=CARTESIAN_POINT ( 'NONE',  ( 87.14099742722598307, 46.04774061545423081, -8.211005622168064733 ) ) ;
#88636=B_SPLINE_SURFACE_WITH_KNOTS ( 'NONE', 3, 1, ( 
 ( #32645, #2266 ),
 ( #740, #31624 ),
 ( #8842, #63541 ),
 ( #10362, #16441 ),
 ( #9349, #9872 ),
 ( #47336, #63043 ),
 ( #39712, #33663 ),
 ( #70640, #25554 ),
 ( #46844, #48353 ),
 ( #93988, #48864 ),
 ( #78762, #8350 ),
 ( #62522, #1254 ),
 ( #32135, #24539 ),
 ( #86405, #94992 ),
 ( #24039, #16937 ),
 ( #64553, #47823 ),
 ( #1765, #56442 ),
 ( #94482, #25038 ),
 ( #26060, #55917 ),
 ( #87436, #86910 ),
 ( #17447, #40729 ),
 ( #41230, #33148 ),
 ( #72169, #77766 ),
 ( #2774, #95514 ),
 ( #56936, #15939 ),
 ( #58429, #72681 ),
 ( #3761, #11382 ),
 ( #50339, #27058 ),
 ( #58911, #19956 ),
 ( #50833, #87921 ),
 ( #42720, #49352 ) ),
 .UNSPECIFIED., .F., .F., .F.,
 ( 4, 3, 3, 3, 3, 3, 3, 3, 3, 3, 4 ),
 ( 2, 2 ),
 ( 0.000000000000000000, 0.1122669598086781934, 0.2243161639709670419, 0.3396355846219092367, 0.4553962076585101326, 0.5677860799922354040, 0.6749047109689589874, 0.7773884377078243979, 0.8775581155834022429, 0.9782364162377785721, 1.000000000000000000 ),
 ( 0.000000000000000000, 1.000000000000000000 ),
 .UNSPECIFIED. ) ;
#88637=CARTESIAN_POINT ( 'NONE',  ( 68.35453417343931903, 65.67399229982113695, 10.37910612949749911 ) ) ;
#88638=CARTESIAN_POINT ( 'NONE',  ( 7.070540392147681708, 27.58029201028040234, 1.583844403245363353 ) ) ;
#88643=EDGE_LOOP ( 'NONE', ( #72420, #26768, #27237, #3576 ) ) ;
#88646=EDGE_CURVE ( 'NONE', #73177, #47570, #35619, .T. ) ;
#88648=CARTESIAN_POINT ( 'NONE',  ( 72.28450659106211162, 69.33006679800452332, -8.955401149264922367 ) ) ;
#88650=CARTESIAN_POINT ( 'NONE',  ( 69.72987185967514279, 62.73297604805756578, -13.30854282143535094 ) ) ;
#88654=VECTOR ( 'NONE', #10445, 1000.000000000000114 ) ;
#88657=FACE_OUTER_BOUND ( 'NONE', #86131, .T. ) ;
#88667=CARTESIAN_POINT ( 'NONE',  ( 77.95413687424900218, 62.00520656085893734, 15.66750427035592708 ) ) ;
#88669=DIRECTION ( 'NONE',  ( -0.8660254037844378194, -0.5000000000000013323, -0.000000000000000000 ) ) ;
#88670=CARTESIAN_POINT ( 'NONE',  ( 70.43471136582493841, 64.87908352274641288, -12.18040581727293414 ) ) ;
#88672=CARTESIAN_POINT ( 'NONE',  ( 5.338489584578805847, 26.58029201028039878, 1.583844403245363353 ) ) ;
#88674=CARTESIAN_POINT ( 'NONE',  ( 39.48888774545857672, 24.92755873383629250, 6.180339887498953466 ) ) ;
#88676=CARTESIAN_POINT ( 'NONE',  ( 75.48012123268173923, 53.33211347945791658, 16.49774674168797617 ) ) ;
#88678=CARTESIAN_POINT ( 'NONE',  ( 87.83899792242847582, 44.00541668311378629, -1.848955303085625390 ) ) ;
#88680=CARTESIAN_POINT ( 'NONE',  ( 80.51198428680065433, 43.68793065238016737, 9.861687463089015893 ) ) ;
#88684=CARTESIAN_POINT ( 'NONE',  ( 86.77687789830739007, 46.46486760889777656, 9.079242751187690530 ) ) ;
#88685=CARTESIAN_POINT ( 'NONE',  ( 23.30503800868897102, 15.58380873178786707, 6.180339887498953466 ) ) ;
#88687=CARTESIAN_POINT ( 'NONE',  ( 72.04834849415196629, 72.28436413801229321, -0.8995985284803085236 ) ) ;
#88689=AXIS2_PLACEMENT_3D ( 'NONE', #97700, #5481, #36363 ) ;
#88690=CARTESIAN_POINT ( 'NONE',  ( 86.89976093607516816, 45.97909969559822940, 8.962991326411129833 ) ) ;
#88692=CARTESIAN_POINT ( 'NONE',  ( 39.74423100597210379, 28.11029122506297639, -8.090169943749478065 ) ) ;
#88701=( BOUNDED_SURFACE ( )  B_SPLINE_SURFACE ( 1, 2, ( 
 ( #61469, #22967, #93922, #24476, #55357, #80732, #81219, #10788, #87366, #3692, #72607, #18896, #71599, #41662, #79724, #88339, #57365, #57865, #27488, #11795, #72095, #88844, #9802, #3209, #18389, #34094, #49284, #19407, #65968, #35061, #64482, #64984, #17896, #50266, #42650, #34571, #58357, #95928, #49775, #42164, #73584, #10286, #73100, #96920, #48793, #65472, #96414, #11306, #4164, #17375, #48284, #41158, #26488, #40662, #56369, #2695, #25477, #79229, #26981, #25994, #33586, #2195, #95442, #56865, #87849, #33078, #80220, #63971, #94914, #36549, #75080, #36051, #6664, #66954, #67456, #98384, #28975, #59850, #90814, #90315, #58839, #21367, #45151, #97883, #97391, #20887, #21857, #76090, #51253, #5661, #68447, #52253, #27959, #83195, #29460, #82219, #13285, #52739, #28456, #12792, #5172, #29954, #83701, #89808, #20381, #43655, #74597, #37541, #82717, #59335, #12284, #43144, #51776, #13758, #81711, #14260, #44146, #99375, #44637, #75571, #89335, #66467, #91292, #19887, #6159, #4677, #37055, #50758, #74086, #35567, #67962, #98880, #60335, #38542, #68941, #62333, #99868, #69449, #7651, #16251, #7144, #30452, #60830, #61837, #61342, #53252, #65, #38031, #62842, #31937, #93797, #92784, #84207, #39031, #91790, #47141, #78066, #30948, #92301, #15737, #23339, #557, #15234, #8653, #31439, #93284, #54227, #22850, #85193, #53734, #23840, #46645, #77570, #22355, #69940, #46130, #39524, #24358, #70449, #8158, #40032, #54733, #55229, #84693, #14753, #1058, #85716, #77043, #86212, #45635, #1574, #16750, #76563, #47638, #78572, #9156, #70972, #94293, #88714, #94789, #3571, #18269, #63850, #17768, #18766, #86710, #41032, #33457, #32946, #73465, #19283, #34452, #63354, #71969, #42532, #95317, #3088, #25348, #48151, #87731, #65350, #72486, #24847, #2573, #64353, #55722, #25874, #80099, #56749, #17246, #56241, #71473, #32457, #72980, #49163, #49643, #41541, #50151, #87234, #96289, #10665, #48669, #79602, #80601, #79094, #33979, #64863, #10165, #9678, #81103, #26858, #40539, #95810, #2066, #26364, #57239, #88214, #11179, #42046, #57734, #11670, #65833, #43538, #35937, #96799, #74479, #51653, #28337, #27358, #27848, #43021, #4048, #45888, #66840, #22621, #13168, #73960, #58240, #89220, #82097, #44022, #19768, #38298, #12670, #61601, #4545, #90189, #30720, #81590, #7406, #100134, #82602, #50637, #20765, #84949, #46395, #12159, #5057, #34938, #35446, #97767, #66348, #6912, #97281, #59215, #51135, #61099, #58726, #89701, #20261, #76339, #37800, #68708, #99634, #30216, #69208, #76812, #92553, #92071, #53506, #84460, #15000, #23099, #53990, #15494, #8414, #32204, #47402, #17001, #31686, #32707, #47890, #9415, #85980, #46910, #78329, #70196, #78832, #8909, #39777, #38800, #55487, #62593, #55982, #48415, #63606, #16507, #56505, #70708, #79364, #54486, #314, #94546, #1322, #806, #93548, #31202, #18028, #40289, #62091, #63109, #94053, #71232, #77320, #69706, #24109, #55002, #93037, #7927, #1824, #23593, #24606, #86473, #25101, #85465, #16010, #33211, #39286, #9928, #86979, #17510, #40790, #71736, #77831, #2329, #64109, #95061, #25621, #87494, #20023, #79858, #57497, #58973, #11441, #19541, #80357, #64620, #3819, #50898, #88987, #10421 ),
 ( #50402, #81357, #89465, #89943, #43290, #3340, #81847, #41294, #34701, #49911, #73227, #80868, #12421, #97531, #66604, #96059, #65602, #18527, #74237, #4823, #35204, #48921, #96555, #11927, #73717, #35706, #41800, #4300, #28100, #10928, #66107, #97055, #42783, #72234, #2840, #33730, #72747, #42294, #95575, #87979, #34216, #56997, #26120, #27125, #88477, #65111, #27626, #49410, #26618, #19039, #58007, #58491, #45288, #44289, #83336, #21508, #75218, #30097, #5801, #13900, #44781, #75717, #6301, #37192, #67595, #28595, #68094, #68590, #36686, #67095, #98525, #76222, #99513, #90458, #52393, #91944, #99016, #98019, #29602, #83841, #21028, #22495, #60979, #14406, #51399, #29114, #20520, #90952, #60475, #51911, #59477, #91433, #6798, #21994, #43791, #59982, #52889, #74734, #37678, #82362, #12931, #82851, #5313, #13421, #36189, #51211, #73541, #27921, #19847, #80685, #34052, #64942, #88799, #50715, #3167, #43615, #19366, #66915, #11260, #96876, #36014, #88295, #12752, #5132, #89293, #26448, #27444, #90275, #51738, #95887, #81180, #41621, #72563, #50225, #18850, #12242, #49732, #11747, #57820, #66427, #57323, #42123, #10745, #42610, #73054, #3649, #4124, #34529, #74555, #82178, #97845, #35018, #65429, #81669, #96370, #97355, #58804, #65920, #26936, #58318, #43101, #74044, #4632, #89768, #35526, #20339, #28414, #59294, #20846, #75533, #84169, #52703, #83663, #44104, #60789, #37014, #61306, #53697, #37994, #91253, #61800, #14226, #84653, #59809, #5619, #68906, #21818, #6118, #67922, #36513, #23302, #22315, #67414, #6627, #76047, #14716, #82680, #75043, #38501, #44598, #15198, #68411, #13722, #98845, #99832, #98342, #45113, #37504, #83157, #30416, #92268, #60296, #29422, #99338, #29917, #53218, #91752, #22816, #45599, #76533, #7110, #52210, #46094, #77007, #7612, #69416, #28, #28933, #30913, #92748, #13246, #90776, #21327, #62805, #33415, #24319, #56196, #31407, #77534, #9639, #93762, #78028, #47107, #8126, #95272, #94254, #38999, #78533, #47605, #55685, #54192, #15703, #10120, #16215, #25308, #39989, #85677, #39486, #40498, #69905, #55195, #86178, #54694, #85156, #40984, #87192, #46601, #16712, #64315, #9118, #24807, #8620, #519, #70930, #17725, #86673, #62293, #1535, #32417, #93250, #63311, #17205, #48108, #23805, #70412, #1020, #31901, #94746, #79050, #71430, #2019, #32905, #63813, #48627, #79562, #71929, #2533, #58685, #34411, #82057, #26324, #11629, #51090, #3048, #27810, #20221, #4013, #41501, #42490, #5019, #66800, #10624, #96252, #56710, #87693, #3535, #33935, #27321, #64822, #65312, #72942, #81548, #72442, #95768, #25835, #26816, #57197, #18225, #57697, #88177, #89659, #97244, #12626, #88674, #49121, #34895, #80056, #43496, #18723, #74438, #35900, #65796, #49607, #73424, #80559, #11137, #42009, #19247, #50112, #81066, #96754, #58205, #89182, #19730, #50597, #12117, #42981, #73919, #4504, #35404, #66312, #67298, #90146, #44489, #43984, #99714, #68789, #30302, #29313, #20723, #75934, #97727, #53096, #84052, #75419, #28807, #52589, #67807, #37390, #52098, #14610, #68294, #29802, #6004, #98225, #98734, #90661, #99217, #60178, #91142, #59172, #6512, #83043, #76423, #61188, #45487, #36897, #76890, #21704, #92156, #74926 ) ),
 .UNSPECIFIED., .F., .F., .T. ) 
 B_SPLINE_SURFACE_WITH_KNOTS ( ( 2, 2 ),
 ( 3, 2, 2, 2, 2, 2, 2, 2, 2, 2, 2, 2, 2, 2, 2, 2, 2, 2, 2, 2, 2, 2, 2, 2, 2, 2, 2, 2, 2, 2, 2, 2, 2, 2, 2, 2, 2, 2, 2, 2, 2, 2, 2, 2, 2, 2, 2, 2, 2, 2, 2, 2, 2, 2, 2, 2, 2, 2, 2, 2, 2, 2, 2, 2, 2, 2, 2, 2, 2, 2, 2, 2, 2, 2, 2, 2, 2, 2, 2, 2, 2, 2, 2, 2, 2, 2, 2, 2, 2, 2, 2, 2, 2, 2, 2, 2, 2, 2, 2, 2, 2, 2, 2, 2, 2, 2, 2, 2, 2, 2, 2, 2, 2, 2, 2, 2, 2, 2, 2, 2, 2, 2, 2, 2, 2, 2, 2, 2, 2, 2, 2, 2, 2, 2, 2, 2, 2, 2, 2, 2, 2, 2, 2, 2, 2, 2, 2, 2, 2, 2, 2, 2, 2, 2, 2, 2, 2, 2, 2, 2, 2, 2, 2, 2, 2, 2, 2, 2, 2, 2, 2, 2, 2, 2, 2, 2, 2, 2, 2, 2, 2, 2, 2, 2, 2, 2, 2, 2, 2, 2, 2, 2, 2, 2, 2, 2, 2, 2, 2, 2, 3 ),
 ( 0.000000000000000000, 1.000000000000000000 ),
 ( 0.000000000000000000, 0.005000000000000000104, 0.01000000000000000021, 0.01499999999999999944, 0.02000000000000000042, 0.02500000000000000139, 0.02999999999999999889, 0.03500000000000000333, 0.04000000000000000083, 0.04499999999999999833, 0.05000000000000000278, 0.05500000000000000028, 0.05999999999999999778, 0.06500000000000000222, 0.07000000000000000666, 0.07499999999999999722, 0.08000000000000000167, 0.08500000000000000611, 0.08999999999999999667, 0.09500000000000000111, 0.1000000000000000056, 0.1049999999999999961, 0.1100000000000000006, 0.1150000000000000050, 0.1199999999999999956, 0.1250000000000000000, 0.1300000000000000044, 0.1350000000000000089, 0.1400000000000000133, 0.1449999999999999900, 0.1499999999999999944, 0.1549999999999999989, 0.1600000000000000033, 0.1650000000000000078, 0.1700000000000000122, 0.1749999999999999889, 0.1799999999999999933, 0.1849999999999999978, 0.1900000000000000022, 0.1950000000000000067, 0.2000000000000000111, 0.2049999999999999878, 0.2099999999999999922, 0.2149999999999999967, 0.2200000000000000011, 0.2250000000000000056, 0.2300000000000000100, 0.2349999999999999867, 0.2399999999999999911, 0.2449999999999999956, 0.2500000000000000000, 0.2550000000000000044, 0.2600000000000000089, 0.2650000000000000133, 0.2700000000000000178, 0.2750000000000000222, 0.2800000000000000266, 0.2849999999999999756, 0.2899999999999999800, 0.2949999999999999845, 0.2999999999999999889, 0.3049999999999999933, 0.3099999999999999978, 0.3150000000000000022, 0.3200000000000000067, 0.3250000000000000111, 0.3300000000000000155, 0.3350000000000000200, 0.3400000000000000244, 0.3449999999999999734, 0.3499999999999999778, 0.3549999999999999822, 0.3599999999999999867, 0.3649999999999999911, 0.3699999999999999956, 0.3750000000000000000, 0.3800000000000000044, 0.3850000000000000089, 0.3900000000000000133, 0.3950000000000000178, 0.4000000000000000222, 0.4050000000000000266, 0.4099999999999999756, 0.4149999999999999800, 0.4199999999999999845, 0.4249999999999999889, 0.4299999999999999933, 0.4349999999999999978, 0.4400000000000000022, 0.4450000000000000067, 0.4500000000000000111, 0.4550000000000000155, 0.4600000000000000200, 0.4650000000000000244, 0.4699999999999999734, 0.4749999999999999778, 0.4799999999999999822, 0.4849999999999999867, 0.4899999999999999911, 0.4949999999999999956, 0.5000000000000000000, 0.5050000000000000044, 0.5100000000000000089, 0.5150000000000000133, 0.5200000000000000178, 0.5250000000000000222, 0.5300000000000000266, 0.5350000000000000311, 0.5400000000000000355, 0.5450000000000000400, 0.5500000000000000444, 0.5550000000000000488, 0.5600000000000000533, 0.5649999999999999467, 0.5699999999999999512, 0.5749999999999999556, 0.5799999999999999600, 0.5849999999999999645, 0.5899999999999999689, 0.5949999999999999734, 0.5999999999999999778, 0.6049999999999999822, 0.6099999999999999867, 0.6149999999999999911, 0.6199999999999999956, 0.6250000000000000000, 0.6300000000000000044, 0.6350000000000000089, 0.6400000000000000133, 0.6450000000000000178, 0.6500000000000000222, 0.6550000000000000266, 0.6600000000000000311, 0.6650000000000000355, 0.6700000000000000400, 0.6750000000000000444, 0.6800000000000000488, 0.6850000000000000533, 0.6899999999999999467, 0.6949999999999999512, 0.6999999999999999556, 0.7049999999999999600, 0.7099999999999999645, 0.7149999999999999689, 0.7199999999999999734, 0.7249999999999999778, 0.7299999999999999822, 0.7349999999999999867, 0.7399999999999999911, 0.7449999999999999956, 0.7500000000000000000, 0.7550000000000000044, 0.7600000000000000089, 0.7650000000000000133, 0.7700000000000000178, 0.7750000000000000222, 0.7800000000000000266, 0.7850000000000000311, 0.7900000000000000355, 0.7950000000000000400, 0.8000000000000000444, 0.8050000000000000488, 0.8100000000000000533, 0.8149999999999999467, 0.8199999999999999512, 0.8249999999999999556, 0.8299999999999999600, 0.8349999999999999645, 0.8399999999999999689, 0.8449999999999999734, 0.8499999999999999778, 0.8549999999999999822, 0.8599999999999999867, 0.8649999999999999911, 0.8699999999999999956, 0.8750000000000000000, 0.8800000000000000044, 0.8850000000000000089, 0.8900000000000000133, 0.8950000000000000178, 0.9000000000000000222, 0.9050000000000000266, 0.9100000000000000311, 0.9150000000000000355, 0.9200000000000000400, 0.9250000000000000444, 0.9300000000000000488, 0.9350000000000000533, 0.9399999999999999467, 0.9449999999999999512, 0.9499999999999999556, 0.9549999999999999600, 0.9599999999999999645, 0.9649999999999999689, 0.9699999999999999734, 0.9749999999999999778, 0.9799999999999999822, 0.9849999999999999867, 0.9899999999999999911, 0.9949999999999999956, 1.000000000000000000 ),
 .UNSPECIFIED. ) 
 GEOMETRIC_REPRESENTATION_ITEM ( )  RATIONAL_B_SPLINE_SURFACE ( (
 ( 1.000000000000000000, 0.9510565162951535312, 1.000000000000000000, 0.9510565162951535312, 1.000000000000000000, 0.9510565162951535312, 1.000000000000000000, 0.9510565162951535312, 1.000000000000000000, 0.9510565162951535312, 1.000000000000000000, 0.9510565162951535312, 1.000000000000000000, 0.9510565162951535312, 1.000000000000000000, 0.9510565162951535312, 1.000000000000000000, 0.9510565162951535312, 1.000000000000000000, 0.9510565162951535312, 1.000000000000000000, 0.9510565162951535312, 1.000000000000000000, 0.9510565162951535312, 1.000000000000000000, 0.9510565162951535312, 1.000000000000000000, 0.9510565162951535312, 1.000000000000000000, 0.9510565162951535312, 1.000000000000000000, 0.9510565162951535312, 1.000000000000000000, 0.9510565162951535312, 1.000000000000000000, 0.9510565162951535312, 1.000000000000000000, 0.9510565162951535312, 1.000000000000000000, 0.9510565162951535312, 1.000000000000000000, 0.9510565162951535312, 1.000000000000000000, 0.9510565162951535312, 1.000000000000000000, 0.9510565162951535312, 1.000000000000000000, 0.9510565162951535312, 1.000000000000000000, 0.9510565162951535312, 1.000000000000000000, 0.9510565162951535312, 1.000000000000000000, 0.9510565162951535312, 1.000000000000000000, 0.9510565162951535312, 1.000000000000000000, 0.9510565162951535312, 1.000000000000000000, 0.9510565162951535312, 1.000000000000000000, 0.9510565162951535312, 1.000000000000000000, 0.9510565162951535312, 1.000000000000000000, 0.9510565162951535312, 1.000000000000000000, 0.9510565162951535312, 1.000000000000000000, 0.9510565162951535312, 1.000000000000000000, 0.9510565162951535312, 1.000000000000000000, 0.9510565162951535312, 1.000000000000000000, 0.9510565162951535312, 1.000000000000000000, 0.9510565162951535312, 1.000000000000000000, 0.9510565162951535312, 1.000000000000000000, 0.9510565162951535312, 1.000000000000000000, 0.9510565162951535312, 1.000000000000000000, 0.9510565162951535312, 1.000000000000000000, 0.9510565162951535312, 1.000000000000000000, 0.9510565162951535312, 1.000000000000000000, 0.9510565162951535312, 1.000000000000000000, 0.9510565162951535312, 1.000000000000000000, 0.9510565162951535312, 1.000000000000000000, 0.9510565162951535312, 1.000000000000000000, 0.9510565162951535312, 1.000000000000000000, 0.9510565162951535312, 1.000000000000000000, 0.9510565162951535312, 1.000000000000000000, 0.9510565162951535312, 1.000000000000000000, 0.9510565162951535312, 1.000000000000000000, 0.9510565162951535312, 1.000000000000000000, 0.9510565162951535312, 1.000000000000000000, 0.9510565162951535312, 1.000000000000000000, 0.9510565162951535312, 1.000000000000000000, 0.9510565162951535312, 1.000000000000000000, 0.9510565162951535312, 1.000000000000000000, 0.9510565162951535312, 1.000000000000000000, 0.9510565162951535312, 1.000000000000000000, 0.9510565162951535312, 1.000000000000000000, 0.9510565162951535312, 1.000000000000000000, 0.9510565162951535312, 1.000000000000000000, 0.9510565162951535312, 1.000000000000000000, 0.9510565162951535312, 1.000000000000000000, 0.9510565162951535312, 1.000000000000000000, 0.9510565162951535312, 1.000000000000000000, 0.9510565162951535312, 1.000000000000000000, 0.9510565162951535312, 1.000000000000000000, 0.9510565162951535312, 1.000000000000000000, 0.9510565162951535312, 1.000000000000000000, 0.9510565162951535312, 1.000000000000000000, 0.9510565162951535312, 1.000000000000000000, 0.9510565162951535312, 1.000000000000000000, 0.9510565162951535312, 1.000000000000000000, 0.9510565162951535312, 1.000000000000000000, 0.9510565162951535312, 1.000000000000000000, 0.9510565162951535312, 1.000000000000000000, 0.9510565162951535312, 1.000000000000000000, 0.9510565162951535312, 1.000000000000000000, 0.9510565162951535312, 1.000000000000000000, 0.9510565162951535312, 1.000000000000000000, 0.9510565162951535312, 1.000000000000000000, 0.9510565162951535312, 1.000000000000000000, 0.9510565162951535312, 1.000000000000000000, 0.9510565162951535312, 1.000000000000000000, 0.9510565162951535312, 1.000000000000000000, 0.9510565162951535312, 1.000000000000000000, 0.9510565162951535312, 1.000000000000000000, 0.9510565162951535312, 1.000000000000000000, 0.9510565162951535312, 1.000000000000000000, 0.9510565162951535312, 1.000000000000000000, 0.9510565162951535312, 1.000000000000000000, 0.9510565162951535312, 1.000000000000000000, 0.9510565162951535312, 1.000000000000000000, 0.9510565162951535312, 1.000000000000000000, 0.9510565162951535312, 1.000000000000000000, 0.9510565162951535312, 1.000000000000000000, 0.9510565162951535312, 1.000000000000000000, 0.9510565162951535312, 1.000000000000000000, 0.9510565162951535312, 1.000000000000000000, 0.9510565162951535312, 1.000000000000000000, 0.9510565162951535312, 1.000000000000000000, 0.9510565162951535312, 1.000000000000000000, 0.9510565162951535312, 1.000000000000000000, 0.9510565162951535312, 1.000000000000000000, 0.9510565162951535312, 1.000000000000000000, 0.9510565162951535312, 1.000000000000000000, 0.9510565162951535312, 1.000000000000000000, 0.9510565162951535312, 1.000000000000000000, 0.9510565162951535312, 1.000000000000000000, 0.9510565162951535312, 1.000000000000000000, 0.9510565162951535312, 1.000000000000000000, 0.9510565162951535312, 1.000000000000000000, 0.9510565162951535312, 1.000000000000000000, 0.9510565162951535312, 1.000000000000000000, 0.9510565162951535312, 1.000000000000000000, 0.9510565162951535312, 1.000000000000000000, 0.9510565162951535312, 1.000000000000000000, 0.9510565162951535312, 1.000000000000000000, 0.9510565162951535312, 1.000000000000000000, 0.9510565162951535312, 1.000000000000000000, 0.9510565162951535312, 1.000000000000000000, 0.9510565162951535312, 1.000000000000000000, 0.9510565162951535312, 1.000000000000000000, 0.9510565162951535312, 1.000000000000000000, 0.9510565162951535312, 1.000000000000000000, 0.9510565162951535312, 1.000000000000000000, 0.9510565162951535312, 1.000000000000000000, 0.9510565162951535312, 1.000000000000000000, 0.9510565162951535312, 1.000000000000000000, 0.9510565162951535312, 1.000000000000000000, 0.9510565162951535312, 1.000000000000000000, 0.9510565162951535312, 1.000000000000000000, 0.9510565162951535312, 1.000000000000000000, 0.9510565162951535312, 1.000000000000000000, 0.9510565162951535312, 1.000000000000000000, 0.9510565162951535312, 1.000000000000000000, 0.9510565162951535312, 1.000000000000000000, 0.9510565162951535312, 1.000000000000000000, 0.9510565162951535312, 1.000000000000000000, 0.9510565162951535312, 1.000000000000000000, 0.9510565162951535312, 1.000000000000000000, 0.9510565162951535312, 1.000000000000000000, 0.9510565162951535312, 1.000000000000000000, 0.9510565162951535312, 1.000000000000000000, 0.9510565162951535312, 1.000000000000000000, 0.9510565162951535312, 1.000000000000000000, 0.9510565162951535312, 1.000000000000000000, 0.9510565162951535312, 1.000000000000000000, 0.9510565162951535312, 1.000000000000000000, 0.9510565162951535312, 1.000000000000000000, 0.9510565162951535312, 1.000000000000000000, 0.9510565162951535312, 1.000000000000000000, 0.9510565162951535312, 1.000000000000000000, 0.9510565162951535312, 1.000000000000000000, 0.9510565162951535312, 1.000000000000000000, 0.9510565162951535312, 1.000000000000000000, 0.9510565162951535312, 1.000000000000000000, 0.9510565162951535312, 1.000000000000000000, 0.9510565162951535312, 1.000000000000000000, 0.9510565162951535312, 1.000000000000000000, 0.9510565162951535312, 1.000000000000000000, 0.9510565162951535312, 1.000000000000000000, 0.9510565162951535312, 1.000000000000000000, 0.9510565162951535312, 1.000000000000000000, 0.9510565162951535312, 1.000000000000000000, 0.9510565162951535312, 1.000000000000000000, 0.9510565162951535312, 1.000000000000000000, 0.9510565162951535312, 1.000000000000000000, 0.9510565162951535312, 1.000000000000000000, 0.9510565162951535312, 1.000000000000000000, 0.9510565162951535312, 1.000000000000000000, 0.9510565162951535312, 1.000000000000000000, 0.9510565162951535312, 1.000000000000000000, 0.9510565162951535312, 1.000000000000000000, 0.9510565162951535312, 1.000000000000000000, 0.9510565162951535312, 1.000000000000000000, 0.9510565162951535312, 1.000000000000000000, 0.9510565162951535312, 1.000000000000000000, 0.9510565162951535312, 1.000000000000000000, 0.9510565162951535312, 1.000000000000000000, 0.9510565162951535312, 1.000000000000000000, 0.9510565162951535312, 1.000000000000000000, 0.9510565162951535312, 1.000000000000000000, 0.9510565162951535312, 1.000000000000000000, 0.9510565162951535312, 1.000000000000000000, 0.9510565162951535312, 1.000000000000000000, 0.9510565162951535312, 1.000000000000000000, 0.9510565162951535312, 1.000000000000000000, 0.9510565162951535312, 1.000000000000000000, 0.9510565162951535312, 1.000000000000000000, 0.9510565162951535312, 1.000000000000000000, 0.9510565162951535312, 1.000000000000000000, 0.9510565162951535312, 1.000000000000000000, 0.9510565162951535312, 1.000000000000000000, 0.9510565162951535312, 1.000000000000000000, 0.9510565162951535312, 1.000000000000000000),
 ( 1.000000000000000000, 0.9510565162951535312, 1.000000000000000000, 0.9510565162951535312, 1.000000000000000000, 0.9510565162951535312, 1.000000000000000000, 0.9510565162951535312, 1.000000000000000000, 0.9510565162951535312, 1.000000000000000000, 0.9510565162951535312, 1.000000000000000000, 0.9510565162951535312, 1.000000000000000000, 0.9510565162951535312, 1.000000000000000000, 0.9510565162951535312, 1.000000000000000000, 0.9510565162951535312, 1.000000000000000000, 0.9510565162951535312, 1.000000000000000000, 0.9510565162951535312, 1.000000000000000000, 0.9510565162951535312, 1.000000000000000000, 0.9510565162951535312, 1.000000000000000000, 0.9510565162951535312, 1.000000000000000000, 0.9510565162951535312, 1.000000000000000000, 0.9510565162951535312, 1.000000000000000000, 0.9510565162951535312, 1.000000000000000000, 0.9510565162951535312, 1.000000000000000000, 0.9510565162951535312, 1.000000000000000000, 0.9510565162951535312, 1.000000000000000000, 0.9510565162951535312, 1.000000000000000000, 0.9510565162951535312, 1.000000000000000000, 0.9510565162951535312, 1.000000000000000000, 0.9510565162951535312, 1.000000000000000000, 0.9510565162951535312, 1.000000000000000000, 0.9510565162951535312, 1.000000000000000000, 0.9510565162951535312, 1.000000000000000000, 0.9510565162951535312, 1.000000000000000000, 0.9510565162951535312, 1.000000000000000000, 0.9510565162951535312, 1.000000000000000000, 0.9510565162951535312, 1.000000000000000000, 0.9510565162951535312, 1.000000000000000000, 0.9510565162951535312, 1.000000000000000000, 0.9510565162951535312, 1.000000000000000000, 0.9510565162951535312, 1.000000000000000000, 0.9510565162951535312, 1.000000000000000000, 0.9510565162951535312, 1.000000000000000000, 0.9510565162951535312, 1.000000000000000000, 0.9510565162951535312, 1.000000000000000000, 0.9510565162951535312, 1.000000000000000000, 0.9510565162951535312, 1.000000000000000000, 0.9510565162951535312, 1.000000000000000000, 0.9510565162951535312, 1.000000000000000000, 0.9510565162951535312, 1.000000000000000000, 0.9510565162951535312, 1.000000000000000000, 0.9510565162951535312, 1.000000000000000000, 0.9510565162951535312, 1.000000000000000000, 0.9510565162951535312, 1.000000000000000000, 0.9510565162951535312, 1.000000000000000000, 0.9510565162951535312, 1.000000000000000000, 0.9510565162951535312, 1.000000000000000000, 0.9510565162951535312, 1.000000000000000000, 0.9510565162951535312, 1.000000000000000000, 0.9510565162951535312, 1.000000000000000000, 0.9510565162951535312, 1.000000000000000000, 0.9510565162951535312, 1.000000000000000000, 0.9510565162951535312, 1.000000000000000000, 0.9510565162951535312, 1.000000000000000000, 0.9510565162951535312, 1.000000000000000000, 0.9510565162951535312, 1.000000000000000000, 0.9510565162951535312, 1.000000000000000000, 0.9510565162951535312, 1.000000000000000000, 0.9510565162951535312, 1.000000000000000000, 0.9510565162951535312, 1.000000000000000000, 0.9510565162951535312, 1.000000000000000000, 0.9510565162951535312, 1.000000000000000000, 0.9510565162951535312, 1.000000000000000000, 0.9510565162951535312, 1.000000000000000000, 0.9510565162951535312, 1.000000000000000000, 0.9510565162951535312, 1.000000000000000000, 0.9510565162951535312, 1.000000000000000000, 0.9510565162951535312, 1.000000000000000000, 0.9510565162951535312, 1.000000000000000000, 0.9510565162951535312, 1.000000000000000000, 0.9510565162951535312, 1.000000000000000000, 0.9510565162951535312, 1.000000000000000000, 0.9510565162951535312, 1.000000000000000000, 0.9510565162951535312, 1.000000000000000000, 0.9510565162951535312, 1.000000000000000000, 0.9510565162951535312, 1.000000000000000000, 0.9510565162951535312, 1.000000000000000000, 0.9510565162951535312, 1.000000000000000000, 0.9510565162951535312, 1.000000000000000000, 0.9510565162951535312, 1.000000000000000000, 0.9510565162951535312, 1.000000000000000000, 0.9510565162951535312, 1.000000000000000000, 0.9510565162951535312, 1.000000000000000000, 0.9510565162951535312, 1.000000000000000000, 0.9510565162951535312, 1.000000000000000000, 0.9510565162951535312, 1.000000000000000000, 0.9510565162951535312, 1.000000000000000000, 0.9510565162951535312, 1.000000000000000000, 0.9510565162951535312, 1.000000000000000000, 0.9510565162951535312, 1.000000000000000000, 0.9510565162951535312, 1.000000000000000000, 0.9510565162951535312, 1.000000000000000000, 0.9510565162951535312, 1.000000000000000000, 0.9510565162951535312, 1.000000000000000000, 0.9510565162951535312, 1.000000000000000000, 0.9510565162951535312, 1.000000000000000000, 0.9510565162951535312, 1.000000000000000000, 0.9510565162951535312, 1.000000000000000000, 0.9510565162951535312, 1.000000000000000000, 0.9510565162951535312, 1.000000000000000000, 0.9510565162951535312, 1.000000000000000000, 0.9510565162951535312, 1.000000000000000000, 0.9510565162951535312, 1.000000000000000000, 0.9510565162951535312, 1.000000000000000000, 0.9510565162951535312, 1.000000000000000000, 0.9510565162951535312, 1.000000000000000000, 0.9510565162951535312, 1.000000000000000000, 0.9510565162951535312, 1.000000000000000000, 0.9510565162951535312, 1.000000000000000000, 0.9510565162951535312, 1.000000000000000000, 0.9510565162951535312, 1.000000000000000000, 0.9510565162951535312, 1.000000000000000000, 0.9510565162951535312, 1.000000000000000000, 0.9510565162951535312, 1.000000000000000000, 0.9510565162951535312, 1.000000000000000000, 0.9510565162951535312, 1.000000000000000000, 0.9510565162951535312, 1.000000000000000000, 0.9510565162951535312, 1.000000000000000000, 0.9510565162951535312, 1.000000000000000000, 0.9510565162951535312, 1.000000000000000000, 0.9510565162951535312, 1.000000000000000000, 0.9510565162951535312, 1.000000000000000000, 0.9510565162951535312, 1.000000000000000000, 0.9510565162951535312, 1.000000000000000000, 0.9510565162951535312, 1.000000000000000000, 0.9510565162951535312, 1.000000000000000000, 0.9510565162951535312, 1.000000000000000000, 0.9510565162951535312, 1.000000000000000000, 0.9510565162951535312, 1.000000000000000000, 0.9510565162951535312, 1.000000000000000000, 0.9510565162951535312, 1.000000000000000000, 0.9510565162951535312, 1.000000000000000000, 0.9510565162951535312, 1.000000000000000000, 0.9510565162951535312, 1.000000000000000000, 0.9510565162951535312, 1.000000000000000000, 0.9510565162951535312, 1.000000000000000000, 0.9510565162951535312, 1.000000000000000000, 0.9510565162951535312, 1.000000000000000000, 0.9510565162951535312, 1.000000000000000000, 0.9510565162951535312, 1.000000000000000000, 0.9510565162951535312, 1.000000000000000000, 0.9510565162951535312, 1.000000000000000000, 0.9510565162951535312, 1.000000000000000000, 0.9510565162951535312, 1.000000000000000000, 0.9510565162951535312, 1.000000000000000000, 0.9510565162951535312, 1.000000000000000000, 0.9510565162951535312, 1.000000000000000000, 0.9510565162951535312, 1.000000000000000000, 0.9510565162951535312, 1.000000000000000000, 0.9510565162951535312, 1.000000000000000000, 0.9510565162951535312, 1.000000000000000000, 0.9510565162951535312, 1.000000000000000000, 0.9510565162951535312, 1.000000000000000000, 0.9510565162951535312, 1.000000000000000000, 0.9510565162951535312, 1.000000000000000000, 0.9510565162951535312, 1.000000000000000000, 0.9510565162951535312, 1.000000000000000000, 0.9510565162951535312, 1.000000000000000000, 0.9510565162951535312, 1.000000000000000000, 0.9510565162951535312, 1.000000000000000000, 0.9510565162951535312, 1.000000000000000000, 0.9510565162951535312, 1.000000000000000000, 0.9510565162951535312, 1.000000000000000000, 0.9510565162951535312, 1.000000000000000000, 0.9510565162951535312, 1.000000000000000000, 0.9510565162951535312, 1.000000000000000000, 0.9510565162951535312, 1.000000000000000000, 0.9510565162951535312, 1.000000000000000000, 0.9510565162951535312, 1.000000000000000000, 0.9510565162951535312, 1.000000000000000000, 0.9510565162951535312, 1.000000000000000000, 0.9510565162951535312, 1.000000000000000000, 0.9510565162951535312, 1.000000000000000000, 0.9510565162951535312, 1.000000000000000000, 0.9510565162951535312, 1.000000000000000000, 0.9510565162951535312, 1.000000000000000000, 0.9510565162951535312, 1.000000000000000000, 0.9510565162951535312, 1.000000000000000000, 0.9510565162951535312, 1.000000000000000000, 0.9510565162951535312, 1.000000000000000000, 0.9510565162951535312, 1.000000000000000000, 0.9510565162951535312, 1.000000000000000000, 0.9510565162951535312, 1.000000000000000000, 0.9510565162951535312, 1.000000000000000000, 0.9510565162951535312, 1.000000000000000000, 0.9510565162951535312, 1.000000000000000000, 0.9510565162951535312, 1.000000000000000000, 0.9510565162951535312, 1.000000000000000000, 0.9510565162951535312, 1.000000000000000000, 0.9510565162951535312, 1.000000000000000000, 0.9510565162951535312, 1.000000000000000000, 0.9510565162951535312, 1.000000000000000000, 0.9510565162951535312, 1.000000000000000000, 0.9510565162951535312, 1.000000000000000000, 0.9510565162951535312, 1.000000000000000000) ) ) 
 REPRESENTATION_ITEM ( '' )  SURFACE ( )  );
#88702=CARTESIAN_POINT ( 'NONE',  ( 75.99750771566300500, 65.44421971917601866, -13.95497799904430458 ) ) ;
#88705=ORIENTED_EDGE ( 'NONE', *, *, #18310, .F. ) ;
#88708=CARTESIAN_POINT ( 'NONE',  ( 67.47994349727724739, 66.77496821803354976, -8.450748656079085208 ) ) ;
#88714=CARTESIAN_POINT ( 'NONE',  ( 26.65055534615017763, 21.10170272979927830, -7.433330006724141015 ) ) ;
#88719=CARTESIAN_POINT ( 'NONE',  ( 11.81506597172265316, 27.79752408145591502, -5.678558825948271327 ) ) ;
#88720=CARTESIAN_POINT ( 'NONE',  ( 76.03876470936320686, 60.18435193765323987, 15.76689522733356164 ) ) ;
#88727=CARTESIAN_POINT ( 'NONE',  ( 75.27341285390555470, 63.90702616464435692, -14.88884485943207459 ) ) ;
#88737=CARTESIAN_POINT ( 'NONE',  ( 72.74966122630479504, 56.93859335219654838, -15.92450643838010471 ) ) ;
#88738=CARTESIAN_POINT ( 'NONE',  ( 77.86555730066851311, 62.20866292688850763, -15.95979438352862090 ) ) ;
#88742=ADVANCED_FACE ( 'NONE', ( #30849 ), #76465, .T. ) ;
#88746=CARTESIAN_POINT ( 'NONE',  ( 38.25529575686164208, 27.80170272979929535, 7.433330006724137462 ) ) ;
#88748=CARTESIAN_POINT ( 'NONE',  ( 74.96244436416358781, 66.36905339528264847, -13.09731569639688509 ) ) ;
#88757=CARTESIAN_POINT ( 'NONE',  ( 73.23650963592969276, 58.97240520736598768, -15.60991212256156402 ) ) ;
#88762=CARTESIAN_POINT ( 'NONE',  ( 69.50635844379594630, 69.67114699658039001, -5.427956398610904287 ) ) ;
#88767=CARTESIAN_POINT ( 'NONE',  ( 80.31808946940563487, 54.04802570103038306, 16.19007400800021301 ) ) ;
#88780=ADVANCED_FACE ( 'NONE', ( #37926 ), #92686, .T. ) ;
#88782=CARTESIAN_POINT ( 'NONE',  ( 74.53493183439029224, 59.86322019391595717, 15.61592258559468505 ) ) ;
#88784=ORIENTED_EDGE ( 'NONE', *, *, #64364, .F. ) ;
#88785=CARTESIAN_POINT ( 'NONE',  ( 80.47734257382147405, 57.78184453145892263, -16.59809864164601478 ) ) ;
#88787=CARTESIAN_POINT ( 'NONE',  ( 71.94586788039056557, 72.25955706396953815, 0.6154238980746699061 ) ) ;
#88799=CARTESIAN_POINT ( 'NONE',  ( 19.03539854152464628, 16.15404122711133184, 8.090169943749479842 ) ) ;
#88805=EDGE_CURVE ( 'NONE', #82637, #23731, #93690, .T. ) ;
#88807=CARTESIAN_POINT ( 'NONE',  ( 25.91265234538223439, 15.36477965099640919, 1.583844403245364907 ) ) ;
#88816=CARTESIAN_POINT ( 'NONE',  ( 24.15577373785222193, 19.11029122506294797, -8.090169943749478065 ) ) ;
#88819=CARTESIAN_POINT ( 'NONE',  ( 72.21763474066925426, 71.89576300834814049, -3.847854183869324984 ) ) ;
#88821=CARTESIAN_POINT ( 'NONE',  ( 73.89313514058181909, 55.59551747721973669, -16.58534802875433911 ) ) ;
#88825=CARTESIAN_POINT ( 'NONE',  ( 75.87740499823547680, 55.03138904370663198, 16.59596780044815389 ) ) ;
#88826=CARTESIAN_POINT ( 'NONE',  ( 30.89548221274965556, 26.03677371833803633, 10.00000000000000533 ) ) ;
#88834=CARTESIAN_POINT ( 'NONE',  ( 30.44305165777243971, 40.68290643055189548, 3.479690158560446702E-15 ) ) ;
#88837=CARTESIAN_POINT ( 'NONE',  ( 36.41017387241338810, 23.94754757982092030, 5.678558825948272215 ) ) ;
#88842=CARTESIAN_POINT ( 'NONE',  ( 87.93887446415499198, 44.76116579897428238, -4.704258403839747693 ) ) ;
#88844=CARTESIAN_POINT ( 'NONE',  ( 7.128892988474023085, 19.51421378149916563, -9.188101187500004485 ) ) ;
#88845=CARTESIAN_POINT ( 'NONE',  ( 71.90360357134966307, 72.59530952775405410, 1.145984468326222805 ) ) ;
#88846=CARTESIAN_POINT ( 'NONE',  ( 12.64980493759981250, 22.70171378149917985, -9.188101187500004485 ) ) ;
#88852=CARTESIAN_POINT ( 'NONE',  ( 81.09965965012654010, 42.48948382993172856, 7.836446954449344915 ) ) ;
#88857=CARTESIAN_POINT ( 'NONE',  ( 66.48584631922960853, 68.21027895571930344, 4.536531987665620491 ) ) ;
#88858=CARTESIAN_POINT ( 'NONE',  ( 87.14442862271327783, 45.34583212582730738, 7.067040553115585766 ) ) ;
#88866=CARTESIAN_POINT ( 'NONE',  ( 77.58762503914641684, 56.56502062187109914, 16.17780933088086925 ) ) ;
#88876=ORIENTED_EDGE ( 'NONE', *, *, #98251, .T. ) ;
#88879=CARTESIAN_POINT ( 'NONE',  ( 73.13476967714908028, 57.39438153525127007, 15.88807208273858684 ) ) ;
#88880=B_SPLINE_SURFACE_WITH_KNOTS ( 'NONE', 3, 1, ( 
 ( #18455, #49343 ),
 ( #41726, #72671 ),
 ( #38606, #6724 ),
 ( #125, #46194 ),
 ( #84755, #30013 ),
 ( #53310, #98448 ),
 ( #21429, #98943 ),
 ( #45696, #15294 ),
 ( #76623, #82778 ),
 ( #7209, #67518 ),
 ( #30517, #14812 ),
 ( #29526, #22419 ),
 ( #5723, #44702 ),
 ( #92359, #77110 ),
 ( #36611, #60898 ),
 ( #13344, #69511 ),
 ( #60398, #59401 ),
 ( #29039, #91354 ),
 ( #53794, #76150 ),
 ( #84265, #99436 ),
 ( #90377, #68515 ),
 ( #91862, #21917 ),
 ( #38092, #7714 ),
 ( #37115, #61406 ),
 ( #20955, #51838 ),
 ( #44209, #69004 ),
 ( #75145, #99933 ),
 ( #52806, #59910 ),
 ( #90881, #22907 ),
 ( #52316, #83763 ),
 ( #83255, #13822 ) ),
 .UNSPECIFIED., .F., .F., .F.,
 ( 4, 3, 3, 3, 3, 3, 3, 3, 3, 3, 4 ),
 ( 2, 2 ),
 ( 0.000000000000000000, 0.1122669598086770831, 0.2243161639709709554, 0.3396355846219147323, 0.4553962076585074126, 0.5677860799922471724, 0.6749047109689605417, 0.7773884377078307262, 0.8775581155834273339, 0.9782364162377794603, 1.000000000000000000 ),
 ( 0.000000000000000000, 1.000000000000000000 ),
 .UNSPECIFIED. ) ;
#88892=CARTESIAN_POINT ( 'NONE',  ( 12.29152061481545566, 25.83478043621387243, -8.090169943749479842 ) ) ;
#88899=CARTESIAN_POINT ( 'NONE',  ( 29.87828763904599683, 19.11110640527293469, -2.839279412974138328 ) ) ;
#88904=ORIENTED_EDGE ( 'NONE', *, *, #88410, .T. ) ;
#88911=B_SPLINE_CURVE_WITH_KNOTS ( 'NONE', 3,
 ( #46924, #86485, #8425, #61611, #47904, #78844, #31698, #55012, #93558, #45902, #24124, #9428, #94558, #85992, #47414, #16519 ),
 .UNSPECIFIED., .F., .F.,
 ( 4, 1, 2, 2, 2, 1, 2, 2, 4 ),
 ( 0.000000000000000000, 0.1249999999999982792, 0.1874999999999990286, 0.2499999999999997780, 0.5000000000000002220, 0.6250000000000003331, 0.6875000000000003331, 0.7500000000000002220, 1.000000000000000000 ),
 .UNSPECIFIED. ) ;
#88925=CARTESIAN_POINT ( 'NONE',  ( 84.80172950927561715, 50.19486025153374698, 13.34007759942641336 ) ) ;
#88932=CARTESIAN_POINT ( 'NONE',  ( 73.83553503644242255, 68.51229284434135991, 11.41127707145445491 ) ) ;
#88937=CARTESIAN_POINT ( 'NONE',  ( 4.482002306134333480, 24.36126292948892669, 6.180339887498949913 ) ) ;
#88940=DIRECTION ( 'NONE',  ( 0.5000000000000006661, -0.8660254037844383745, 2.435752736085845824E-15 ) ) ;
#88941=ADVANCED_FACE ( 'NONE', ( #26750 ), #63249, .T. ) ;
#88944=ORIENTED_EDGE ( 'NONE', *, *, #57176, .T. ) ;
#88947=ADVANCED_FACE ( 'NONE', ( #64247 ), #94684, .T. ) ;
#88948=AXIS2_PLACEMENT_3D ( 'NONE', #67699, #37778, #6888 ) ;
#88950=ADVANCED_FACE ( 'NONE', ( #49057 ), #95197, .T. ) ;
#88951=CARTESIAN_POINT ( 'NONE',  ( 68.71802935033312565, 64.09262139948224046, -11.98471630605159177 ) ) ;
#88953=CARTESIAN_POINT ( 'NONE',  ( 80.92193103463624482, 53.39041974847280159, 15.96582457958936274 ) ) ;
#88957=CARTESIAN_POINT ( 'NONE',  ( 68.43296295610389279, 66.95241442033321277, 8.990821635125779920 ) ) ;
#88964=CARTESIAN_POINT ( 'NONE',  ( 17.13451663979182626, 31.93396525600390135, 2.839279412974139660 ) ) ;
#88965=CARTESIAN_POINT ( 'NONE',  ( 74.81608510805732237, 67.12708246140779522, 12.96692076351790490 ) ) ;
#88975=CARTESIAN_POINT ( 'NONE',  ( 81.74618951931624622, 55.66798611840641087, -15.97864541239357727 ) ) ;
#88977=CARTESIAN_POINT ( 'NONE',  ( 71.68087887753404175, 71.27905009602892505, 4.678563896432837765 ) ) ;
#88979=CARTESIAN_POINT ( 'NONE',  ( 71.80888402837304341, 72.55032655444115619, 1.016447747306864269 ) ) ;
#88980=CARTESIAN_POINT ( 'NONE',  ( 83.66549642538166154, 42.56717918585069782, 5.117918876049285970 ) ) ;
#88981=CARTESIAN_POINT ( 'NONE',  ( 80.02440815614393443, 53.77024961372720924, 15.74125996130883465 ) ) ;
#88987=CARTESIAN_POINT ( 'NONE',  ( 42.85004829832550399, 33.24335787977766188, -9.188101187500008038 ) ) ;
#88989=ORIENTED_EDGE ( 'NONE', *, *, #24292, .F. ) ;
#88997=LINE ( 'NONE', #19550, #18485 ) ;
#89001=ORIENTED_EDGE ( 'NONE', *, *, #1566, .T. ) ;
#89004=CARTESIAN_POINT ( 'NONE',  ( 79.04618249573870514, 51.69161574664858705, -15.34666239050040026 ) ) ;
#89007=ORIENTED_EDGE ( 'NONE', *, *, #19483, .T. ) ;
#89012=ORIENTED_EDGE ( 'NONE', *, *, #30530, .F. ) ;
#89018=CARTESIAN_POINT ( 'NONE',  ( 81.94547001506749950, 41.15136089338242442, 3.786739421817370665 ) ) ;
#89021=DIRECTION ( 'NONE',  ( -0.8660254037844377084, -0.5000000000000014433, -0.000000000000000000 ) ) ;
#89022=EDGE_CURVE ( 'NONE', #21377, #43244, #16645, .T. ) ;
#89026=CARTESIAN_POINT ( 'NONE',  ( 70.70031318904726447, 61.05212235982030933, -14.44737232470619404 ) ) ;
#89027=CARTESIAN_POINT ( 'NONE',  ( 6.007877864960585512, 21.65586893147753855, -7.433330006724137462 ) ) ;
#89037=CARTESIAN_POINT ( 'NONE',  ( 83.12008827683904144, 49.71316083303308631, -14.04899104105282603 ) ) ;
#89042=CARTESIAN_POINT ( 'NONE',  ( 88.21629111658447187, 43.86250281267856366, -2.113840622537501268 ) ) ;
#89045=CARTESIAN_POINT ( 'NONE',  ( 66.16044157329372410, 68.77389650870436810, 0.09421816583955693047 ) ) ;
#89046=ORIENTED_EDGE ( 'NONE', *, *, #36705, .F. ) ;
#89049=PLANE ( 'NONE',  #67657 ) ;
#89053=CARTESIAN_POINT ( 'NONE',  ( 88.09744597521934395, 43.85530739230785002, 2.493575494356675915 ) ) ;
#89055=ORIENTED_EDGE ( 'NONE', *, *, #849, .F. ) ;
#89056=CARTESIAN_POINT ( 'NONE',  ( 77.93608175853721320, 60.44472089337216403, -15.94298384165975335 ) ) ;
#89060=CARTESIAN_POINT ( 'NONE',  ( 80.63072111635572981, 43.41492672548933029, -9.458890991678615023 ) ) ;
#89066=CARTESIAN_POINT ( 'NONE',  ( 87.93946558867349950, 44.22841546557597781, -4.388681702043149890 ) ) ;
#89071=CARTESIAN_POINT ( 'NONE',  ( 76.46473898121278978, 51.50464710109596211, 15.63208781809325210 ) ) ;
#89075=CARTESIAN_POINT ( 'NONE',  ( 84.70570963598828484, 50.54194691030828324, 13.58719792634913048 ) ) ;
#89076=CARTESIAN_POINT ( 'NONE',  ( 81.76693488703203627, 53.61405564248835276, -15.52540917180992608 ) ) ;
#89077=CARTESIAN_POINT ( 'NONE',  ( 79.49584607199039965, 46.25465621355715484, -13.22861432332135045 ) ) ;
#89088=CARTESIAN_POINT ( 'NONE',  ( 28.84929788977513709, 34.84336893147758474, -7.433330006724137462 ) ) ;
#89089=CARTESIAN_POINT ( 'NONE',  ( 85.07407126341273340, 47.84811938996161018, -12.04656201052697639 ) ) ;
#89090=CARTESIAN_POINT ( 'NONE',  ( 85.32304387868026652, 46.66374142128459113, -10.20885714811630685 ) ) ;
#89092=CARTESIAN_POINT ( 'NONE',  ( 21.14648969749996610, 33.18502408145591431, 5.678558825948277544 ) ) ;
#89102=CARTESIAN_POINT ( 'NONE',  ( 74.92637023225178439, 53.29515228095790036, 16.04570802865760726 ) ) ;
#89107=CARTESIAN_POINT ( 'NONE',  ( 84.09425856091186802, 41.95143607498360439, 1.796127423495148090 ) ) ;
#89110=CARTESIAN_POINT ( 'NONE',  ( 77.29872171176955931, 63.11034017860918510, -15.25129268891816636 ) ) ;
#89112=CARTESIAN_POINT ( 'NONE',  ( 72.19330168037886608, 71.72436257440323004, 5.504111378373452546 ) ) ;
#89113=CARTESIAN_POINT ( 'NONE',  ( 11.51180284259942610, 11.81029122506292595, 8.090169943749479842 ) ) ;
#89115=CARTESIAN_POINT ( 'NONE',  ( 87.76333951327919181, 44.16327574611633366, -4.502641440754707958 ) ) ;
#89117=CARTESIAN_POINT ( 'NONE',  ( 33.64972468124413751, 31.37878583063843152, 9.188101187500006262 ) ) ;
#89118=CARTESIAN_POINT ( 'NONE',  ( 74.26468799828701606, 60.22538159402847668, -15.47038156723467317 ) ) ;
#89124=CARTESIAN_POINT ( 'NONE',  ( 68.21928072586437963, 65.89764169037908914, 10.80738802253310382 ) ) ;
#89126=CARTESIAN_POINT ( 'NONE',  ( 85.68248700152321362, 48.85324039464858714, -12.07567358188643603 ) ) ;
#89155=ORIENTED_EDGE ( 'NONE', *, *, #17833, .T. ) ;
#89159=CARTESIAN_POINT ( 'NONE',  ( 68.46675863972684795, 69.16680760964652563, -5.177149215189699838 ) ) ;
#89161=CARTESIAN_POINT ( 'NONE',  ( 69.65303681785772483, 62.65480059021348325, -13.32895749987356560 ) ) ;
#89167=CARTESIAN_POINT ( 'NONE',  ( 81.96261277299991832, 41.02826309496089152, -3.256590647522187965 ) ) ;
#89168=CARTESIAN_POINT ( 'NONE',  ( 80.52662281699345215, 43.47104460342509213, 9.598632849592865668 ) ) ;
#89173=CARTESIAN_POINT ( 'NONE',  ( 80.85680478625504009, 54.83540491762479263, 15.90941129233622675 ) ) ;
#89179=CARTESIAN_POINT ( 'NONE',  ( 71.12330115413381293, 70.98152915379483829, -4.639273218532493637 ) ) ;
#89181=LINE ( 'NONE', #3533, #15832 ) ;
#89182=CARTESIAN_POINT ( 'NONE',  ( 39.82000823235115661, 28.15404122711136736, 8.090169943749479842 ) ) ;
#89186=CARTESIAN_POINT ( 'NONE',  ( 85.00527620810069607, 43.38834873272450210, -5.370498173854784341 ) ) ;
#89190=ORIENTED_EDGE ( 'NONE', *, *, #56864, .F. ) ;
#89191=CARTESIAN_POINT ( 'NONE',  ( 86.62141849789249193, 46.36649306945518134, 9.067576869787547622 ) ) ;
#89193=CARTESIAN_POINT ( 'NONE',  ( 71.51903464973995028, 72.36264346112822921, -1.271393898589449512 ) ) ;
#89198=CARTESIAN_POINT ( 'NONE',  ( 41.38738224522862907, 24.86426979415093186, -3.090169943749474069 ) ) ;
#89202=CARTESIAN_POINT ( 'NONE',  ( 68.98552337397570966, 67.88664236019715759, -8.139828674801092845 ) ) ;
#89203=CARTESIAN_POINT ( 'NONE',  ( 87.14537157594897110, 46.05544232951319827, -8.218268012384905674 ) ) ;
#89204=CARTESIAN_POINT ( 'NONE',  ( 80.15404930735284950, 58.24487849859603017, -16.60713908503101877 ) ) ;
#89210=EDGE_LOOP ( 'NONE', ( #48471, #4078, #791, #36570 ) ) ;
#89215=CARTESIAN_POINT ( 'NONE',  ( 67.66662286171703045, 66.83249233868968986, -8.522559018194412417 ) ) ;
#89220=CARTESIAN_POINT ( 'NONE',  ( 33.57875857642567752, 25.10170272979928896, -7.433330006724141015 ) ) ;
#89224=VERTEX_POINT ( 'NONE', #34830 ) ;
#89225=CARTESIAN_POINT ( 'NONE',  ( 20.93478768117288524, 17.80170272979926338, 7.433330006724137462 ) ) ;
#89232=CARTESIAN_POINT ( 'NONE',  ( 70.48357858576694923, 65.23080690043917684, -12.53072601663070706 ) ) ;
#89242=CARTESIAN_POINT ( 'NONE',  ( 78.40057582686800686, 61.29346224198984316, -15.87704840749689161 ) ) ;
#89249=VERTEX_POINT ( 'NONE', #74377 ) ;
#89251=CARTESIAN_POINT ( 'NONE',  ( 38.91320803870388545, 23.26216523072497466, -2.296566073217252530E-15 ) ) ;
#89261=CARTESIAN_POINT ( 'NONE',  ( 74.49454245850880341, 63.15023117209727843, -14.55457805515772840 ) ) ;
#89269=CARTESIAN_POINT ( 'NONE',  ( 84.14312167556933275, 48.98415679381830756, 0.000000000000000000 ) ) ;
#89280=CARTESIAN_POINT ( 'NONE',  ( 74.23186439702232065, 58.41354208856498786, 15.85634166313547588 ) ) ;
#89284=CARTESIAN_POINT ( 'NONE',  ( 76.89472034703643999, 56.68234231651032928, 16.18388797058281980 ) ) ;
#89293=CARTESIAN_POINT ( 'NONE',  ( 12.38042018312781067, 30.08080186712591697, -3.090169943749475845 ) ) ;
#89295=CARTESIAN_POINT ( 'NONE',  ( 81.58361516609492980, 41.71275962428084227, 5.900248587975138292 ) ) ;
#89309=CARTESIAN_POINT ( 'NONE',  ( 17.39660613652184296, 31.81751292744056059, -6.180339887498951690 ) ) ;
#89310=CARTESIAN_POINT ( 'NONE',  ( 88.08725135673812190, 43.63233996731285202, 0.09640656973314638833 ) ) ;
#89312=CARTESIAN_POINT ( 'NONE',  ( 72.10046935555597258, 72.37486351763082837, -3.289382622874389206 ) ) ;
#89314=CARTESIAN_POINT ( 'NONE',  ( 74.13991727214688865, 55.63178720252560794, -16.58981027534304431 ) ) ;
#89316=CARTESIAN_POINT ( 'NONE',  ( 75.97157031761298640, 55.45432131483929794, 16.60500414049532480 ) ) ;
#89319=EDGE_CURVE ( 'NONE', #81254, #38046, #99946, .T. ) ;
#89325=CARTESIAN_POINT ( 'NONE',  ( 80.52836418950521136, 57.78044297351195269, -16.24599850453018846 ) ) ;
#89327=CARTESIAN_POINT ( 'NONE',  ( 79.18223904501012100, 60.01793730243658587, 16.13539395559152467 ) ) ;
#89328=CARTESIAN_POINT ( 'NONE',  ( 39.23796756512304995, 23.44966523072497822, -2.296566073217252530E-15 ) ) ;
#89329=CARTESIAN_POINT ( 'NONE',  ( 82.10523990517461357, 41.85707133252695655, -5.529865280922476423 ) ) ;
#89335=CARTESIAN_POINT ( 'NONE',  ( 17.19524200933981817, 21.87878583063841020, -9.188101187500006262 ) ) ;
#89337=CARTESIAN_POINT ( 'NONE',  ( 82.27982384062090659, 54.25399372119451158, 15.63186620393292436 ) ) ;
#89342=CARTESIAN_POINT ( 'NONE',  ( 75.11546922477293720, 53.61976721164031545, -16.54181461514712836 ) ) ;
#89343=CARTESIAN_POINT ( 'NONE',  ( 81.13608137687064925, 42.60696278352305910, 7.988320930663083352 ) ) ;
#89346=CARTESIAN_POINT ( 'NONE',  ( 67.38519378865026965, 69.44927455685115092, 1.146917413897621918 ) ) ;
#89347=CARTESIAN_POINT ( 'NONE',  ( 66.51856882819618022, 68.22589165948441803, 4.545885137720724778 ) ) ;
#89348=CARTESIAN_POINT ( 'NONE',  ( 87.12892733211938889, 45.32551623454932610, 7.045331451850512572 ) ) ;
#89349=ORIENTED_EDGE ( 'NONE', *, *, #65244, .T. ) ;
#89350=ORIENTED_EDGE ( 'NONE', *, *, #8847, .F. ) ;
#89355=CARTESIAN_POINT ( 'NONE',  ( 80.47503692277169307, 57.63887959601478883, -16.59359448248663682 ) ) ;
#89359=CARTESIAN_POINT ( 'NONE',  ( 82.92091453256576017, 49.04847585767068807, -13.26297005650615368 ) ) ;
#89363=CARTESIAN_POINT ( 'NONE',  ( 73.49378489868225017, 58.86888438589103600, 15.66859131630157087 ) ) ;
#89381=EDGE_CURVE ( 'NONE', #54783, #85413, #64700, .T. ) ;
#89383=ORIENTED_EDGE ( 'NONE', *, *, #19417, .T. ) ;
#89384=CARTESIAN_POINT ( 'NONE',  ( 78.20921595494600354, 56.55723432008092288, -16.20170577005126233 ) ) ;
#89387=CARTESIAN_POINT ( 'NONE',  ( 77.52175738690283424, 49.76289862564163968, -14.96722493358440964 ) ) ;
#89393=CARTESIAN_POINT ( 'NONE',  ( 82.82392674575149272, 51.78329203972547390, -14.70596644949177367 ) ) ;
#89407=CARTESIAN_POINT ( 'NONE',  ( 84.49949969528468330, 50.67006985176584521, 13.73213175918632523 ) ) ;
#89411=ORIENTED_EDGE ( 'NONE', *, *, #75362, .F. ) ;
#89414=CARTESIAN_POINT ( 'NONE',  ( 74.23555041547365363, 68.49601928387087924, -11.11897725275786719 ) ) ;
#89415=CARTESIAN_POINT ( 'NONE',  ( 74.55808943708029801, 66.56006064317872983, 13.25253988228418933 ) ) ;
#89421=ORIENTED_EDGE ( 'NONE', *, *, #59652, .T. ) ;
#89422=B_SPLINE_CURVE_WITH_KNOTS ( 'NONE', 3,
 ( #59992, #4309, #21519, #97543 ),
 .UNSPECIFIED., .F., .F.,
 ( 4, 4 ),
 ( 0.7749614532321769111, 1.000000000000000000 ),
 .UNSPECIFIED. ) ;
#89428=CARTESIAN_POINT ( 'NONE',  ( 79.31945258186283354, 46.38531387088102775, -12.78158360291588203 ) ) ;
#89433=CARTESIAN_POINT ( 'NONE',  ( 69.93400774566801203, 69.49255144249838168, 6.423098758560858990 ) ) ;
#89437=CARTESIAN_POINT ( 'NONE',  ( 84.95610959662400319, 47.13610345203377960, 11.47420349594596800 ) ) ;
#89439=CARTESIAN_POINT ( 'NONE',  ( 21.31005897544419980, 27.70171378149919050, -9.188101187500004485 ) ) ;
#89444=CARTESIAN_POINT ( 'NONE',  ( 74.62401959271109320, 66.89443057110609914, 13.05059976691390311 ) ) ;
#89445=CARTESIAN_POINT ( 'NONE',  ( 20.17205688044380452, 16.81029122506294371, 8.090169943749479842 ) ) ;
#89451=CARTESIAN_POINT ( 'NONE',  ( 81.46946648389129564, 55.43478263998397182, -16.31964423845218093 ) ) ;
#89453=CARTESIAN_POINT ( 'NONE',  ( 70.27326910769903634, 69.23385671948467746, 7.233023378589638064 ) ) ;
#89457=B_SPLINE_SURFACE_WITH_KNOTS ( 'NONE', 3, 1, ( 
 ( #98441, #84258 ),
 ( #76615, #52796 ),
 ( #83755, #37595 ),
 ( #14316, #99428 ),
 ( #30005, #60889 ),
 ( #22411, #14805 ),
 ( #45688, #38085 ),
 ( #68997, #75137 ),
 ( #30508, #61399 ),
 ( #92351, #46184 ),
 ( #77103, #7706 ),
 ( #69503, #90368 ),
 ( #59392, #20947 ),
 ( #82770, #13337 ),
 ( #5715, #36604 ),
 ( #94348, #71030 ),
 ( #9212, #93855 ),
 ( #2122, #39083 ),
 ( #87292, #93342 ),
 ( #79155, #31493 ),
 ( #24902, #24410 ),
 ( #9736, #40591 ),
 ( #48724, #85252 ),
 ( #611, #23392 ),
 ( #8711, #86266 ),
 ( #32516, #69996 ),
 ( #8213, #71530 ),
 ( #63409, #54282 ),
 ( #33004, #63905 ),
 ( #15797, #55286 ),
 ( #1116, #47199 ) ),
 .UNSPECIFIED., .F., .F., .F.,
 ( 4, 3, 3, 3, 3, 3, 3, 3, 3, 3, 4 ),
 ( 2, 2 ),
 ( 0.000000000000000000, 0.1122669598086777354, 0.2243161639709747579, 0.3396355846219261121, 0.4553962076585106877, 0.5677860799922511692, 0.6749047109689668700, 0.7773884377078540409, 0.8775581155834283331, 0.9782364162377975569, 1.000000000000000000 ),
 ( 0.000000000000000000, 1.000000000000000000 ),
 .UNSPECIFIED. ) ;
#89459=LINE ( 'NONE', #42287, #92684 ) ;
#89465=CARTESIAN_POINT ( 'NONE',  ( 3.631266576971075910, 20.83478043621385467, -8.090169943749479842 ) ) ;
#89471=VERTEX_POINT ( 'NONE', #72636 ) ;
#89472=CARTESIAN_POINT ( 'NONE',  ( 78.86792953187128319, 59.60067377931095933, 16.50582274385373438 ) ) ;
#89473=DIRECTION ( 'NONE',  ( 0.5000000000000013323, -0.8660254037844378194, 0.000000000000000000 ) ) ;
#89475=CARTESIAN_POINT ( 'NONE',  ( 74.72875307343204554, 53.51675845243507723, 16.07614988730082928 ) ) ;
#89476=EDGE_LOOP ( 'NONE', ( #71407, #38072, #63754, #36754 ) ) ;
#89488=CARTESIAN_POINT ( 'NONE',  ( 76.00560383303448475, 63.90649832781891604, 14.64634901227351449 ) ) ;
#89489=CARTESIAN_POINT ( 'NONE',  ( 89.84776793077681134, 45.10341964059156794, 0.3078307376628255376 ) ) ;
#89490=ORIENTED_EDGE ( 'NONE', *, *, #93781, .F. ) ;
#89493=CARTESIAN_POINT ( 'NONE',  ( 82.09195791283381993, 41.10995726237445069, 3.277656812944607090 ) ) ;
#89497=CARTESIAN_POINT ( 'NONE',  ( 18.88643602551048417, 33.83705186507754092, 3.090169943749475401 ) ) ;
#89504=ADVANCED_FACE ( 'NONE', ( #1090 ), #24385, .T. ) ;
#89513=CARTESIAN_POINT ( 'NONE',  ( 70.97534519514762508, 61.01255604146208356, 14.53188312944952543 ) ) ;
#89515=CARTESIAN_POINT ( 'NONE',  ( 86.23748403073643942, 43.56198212328983033, 3.817419489612863703 ) ) ;
#89516=CARTESIAN_POINT ( 'NONE',  ( 88.26483236760812190, 44.33866273282983173, -2.345556310904765684 ) ) ;
#89519=ORIENTED_EDGE ( 'NONE', *, *, #93904, .F. ) ;
#89527=CARTESIAN_POINT ( 'NONE',  ( 88.28417999105286640, 44.35115056094939234, 2.384166010199538110 ) ) ;
#89530=VERTEX_POINT ( 'NONE', #53762 ) ;
#89531=CARTESIAN_POINT ( 'NONE',  ( 76.91358264944020107, 60.84600432610378107, -15.73813892003315651 ) ) ;
#89534=CARTESIAN_POINT ( 'NONE',  ( 69.86610170196659908, 66.23337933603376371, -10.74216025327337931 ) ) ;
#89535=CARTESIAN_POINT ( 'NONE',  ( 67.09968926803097133, 66.79733971661106295, -9.013546469615247858 ) ) ;
#89537=CARTESIAN_POINT ( 'NONE',  ( 80.95554863947107549, 43.36305847308316430, -9.979587924406191135 ) ) ;
#89544=CARTESIAN_POINT ( 'NONE',  ( 77.94050277262006432, 51.16694309523679607, 15.34650497222302334 ) ) ;
#89545=AXIS2_PLACEMENT_3D ( 'NONE', #48030, #64238, #9560 ) ;
#89546=CARTESIAN_POINT ( 'NONE',  ( 75.82794950087699704, 51.68186498792067596, 15.74941689662516531 ) ) ;
#89549=CARTESIAN_POINT ( 'NONE',  ( 84.57934031330240998, 50.64028946732422298, 13.68816099377781015 ) ) ;
#89555=CARTESIAN_POINT ( 'NONE',  ( 88.07426949318437437, 43.62472922332415237, 0.07787791115677746012 ) ) ;
#89556=EDGE_CURVE ( 'NONE', #38703, #32075, #23870, .T. ) ;
#89563=CARTESIAN_POINT ( 'NONE',  ( 86.70600090578749075, 46.44620277030321631, -9.070728233001970509 ) ) ;
#89565=CARTESIAN_POINT ( 'NONE',  ( 26.56574046957052460, 17.19860640527293327, 2.839279412974134775 ) ) ;
#89567=CARTESIAN_POINT ( 'NONE',  ( 29.54281338067077911, 40.55466486950702176, -1.111400068045478839E-16 ) ) ;
#89570=B_SPLINE_CURVE_WITH_KNOTS ( 'NONE', 3,
 ( #57866, #74598, #51254, #82718, #34572, #20888, #67457, #59336, #19888, #50759, #88845, #81712, #75081, #50267, #81220, #11796, #12285, #98385, #12793, #42651, #5173, #36052, #43656, #73585, #43145, #4678, #35568, #89809, #28976, #20382, #82220 ),
 .UNSPECIFIED., .F., .F.,
 ( 4, 3, 3, 3, 3, 3, 3, 3, 3, 3, 4 ),
 ( 0.000000000000000000, 0.1333490885032311002, 0.3007194338854346505, 0.4699862290245186980, 0.5844252810809363874, 0.6686540514502655741, 0.7354980260655468172, 0.8028463152565521455, 0.8633854507757170449, 0.9437142632667351316, 1.000000000000000000 ),
 .UNSPECIFIED. ) ;
#89572=CARTESIAN_POINT ( 'NONE',  ( 70.92847601347175157, 61.07039847582737480, 15.02503073586101934 ) ) ;
#89578=CARTESIAN_POINT ( 'NONE',  ( 75.44698045856164015, 53.24411920270586762, 16.49076459687135809 ) ) ;
#89584=CARTESIAN_POINT ( 'NONE',  ( 84.98597642252352102, 42.67336299467312699, 3.100190142275117022 ) ) ;
#89586=CARTESIAN_POINT ( 'NONE',  ( 86.09173314450353587, 43.00402348852082923, 1.099162958027281034 ) ) ;
#89592=CARTESIAN_POINT ( 'NONE',  ( 83.59149176045259821, 49.15513213620079824, 13.56910806411459980 ) ) ;
#89594=CARTESIAN_POINT ( 'NONE',  ( 34.69977369993910798, 22.96004757982091959, -5.678558825948275768 ) ) ;
#89595=CARTESIAN_POINT ( 'NONE',  ( 73.35648102757406264, 60.49408656809458051, -15.23552882400795028 ) ) ;
#89600=ORIENTED_EDGE ( 'NONE', *, *, #10980, .F. ) ;
#89601=CARTESIAN_POINT ( 'NONE',  ( 81.39623687408305841, 42.43901693502521510, 7.471974766692582648 ) ) ;
#89605=CARTESIAN_POINT ( 'NONE',  ( 85.70209702422732789, 48.64685655562228561, 12.37813881961889528 ) ) ;
#89607=AXIS2_PLACEMENT_3D ( 'NONE', #16474, #277, #63075 ) ;
#89620=ORIENTED_EDGE ( 'NONE', *, *, #24343, .T. ) ;
#89621=CARTESIAN_POINT ( 'NONE',  ( 86.98925081226386169, 46.40596221211884398, -8.809588356812486865 ) ) ;
#89630=VERTEX_POINT ( 'NONE', #83050 ) ;
#89633=CARTESIAN_POINT ( 'NONE',  ( 82.18459391862934638, 44.45332069473768399, 9.672573637705005112 ) ) ;
#89635=CARTESIAN_POINT ( 'NONE',  ( 69.71517978252398962, 62.25915488727545721, -13.58123164448667985 ) ) ;
#89637=ORIENTED_EDGE ( 'NONE', *, *, #61593, .F. ) ;
#89639=CARTESIAN_POINT ( 'NONE',  ( 71.67038792483674570, 63.34331654576415360, 13.62529284351906078 ) ) ;
#89644=CARTESIAN_POINT ( 'NONE',  ( 76.07161074972545123, 51.48760201263585401, -16.16757060908070898 ) ) ;
#89647=CARTESIAN_POINT ( 'NONE',  ( 80.26331314844821918, 51.25704456883815396, 15.00005997246581835 ) ) ;
#89650=CARTESIAN_POINT ( 'NONE',  ( 73.08094384907833785, 54.14441083166272506, 0.000000000000000000 ) ) ;
#89655=CARTESIAN_POINT ( 'NONE',  ( 68.42965730954357184, 70.07997676687871547, -1.242414669626054957 ) ) ;
#89659=CARTESIAN_POINT ( 'NONE',  ( 34.97582608256301739, 32.14441083166263979, 10.00000000000000533 ) ) ;
#89663=CARTESIAN_POINT ( 'NONE',  ( 81.92870213848958372, 43.19805473905109494, -8.210944645206849302 ) ) ;
#89668=AXIS2_PLACEMENT_3D ( 'NONE', #91441, #76231, #29124 ) ;
#89669=CARTESIAN_POINT ( 'NONE',  ( 86.82393771405537564, 45.90093866298671799, 8.916403221032373594 ) ) ;
#89672=CARTESIAN_POINT ( 'NONE',  ( 72.07067459802226495, 72.25717277724338317, -1.547674812006160305 ) ) ;
#89674=CARTESIAN_POINT ( 'NONE',  ( 86.79998443407272646, 45.86195168027221314, 8.882059948630848467 ) ) ;
#89677=CARTESIAN_POINT ( 'NONE',  ( 4.462289544239296468, 25.68290643055184574, 3.479690158560446702E-15 ) ) ;
#89682=DIRECTION ( 'NONE',  ( 0.2649596321166021728, -0.4589235447807153423, -0.8480480961564252906 ) ) ;
#89684=CARTESIAN_POINT ( 'NONE',  ( 87.10573541114747798, 46.00189626469253312, -8.174982887696250700 ) ) ;
#89701=CARTESIAN_POINT ( 'NONE',  ( 30.77620441319551503, 35.95586893147757479, 7.433330006724141015 ) ) ;
#89706=CARTESIAN_POINT ( 'NONE',  ( 19.86064915544625009, 12.26216523072493914, -2.296566073217252530E-15 ) ) ;
#89707=CARTESIAN_POINT ( 'NONE',  ( 68.42452078367514900, 64.50266422004676770, 12.17129190631728441 ) ) ;
#89711=CARTESIAN_POINT ( 'NONE',  ( 76.65983718867957464, 54.53321319951793811, 16.54430215486172528 ) ) ;
#89714=VERTEX_POINT ( 'NONE', #46489 ) ;
#89715=ADVANCED_FACE ( 'NONE', ( #9525 ), #31787, .T. ) ;
#89720=CARTESIAN_POINT ( 'NONE',  ( 66.27921550192024824, 69.23555237665273410, -2.128515666495896852 ) ) ;
#89722=CARTESIAN_POINT ( 'NONE',  ( 81.90070505019525626, 55.28399500932853528, 16.25061773925407493 ) ) ;
#89723=CARTESIAN_POINT ( 'NONE',  ( 78.12682272674805972, 61.49995998885079729, -16.15539878443392396 ) ) ;
#89732=CARTESIAN_POINT ( 'NONE',  ( 75.10797937051889051, 66.37172067175724521, -13.15131572357236323 ) ) ;
#89735=CARTESIAN_POINT ( 'NONE',  ( 81.71596569511639530, 55.69046771286013353, 16.33797717450969955 ) ) ;
#89738=CARTESIAN_POINT ( 'NONE',  ( 87.37622458635497935, 44.94434973981049808, 6.879737256407633339 ) ) ;
#89740=CARTESIAN_POINT ( 'NONE',  ( 69.12672858200174630, 64.33651235087042153, -11.97836756590942997 ) ) ;
#89754=ORIENTED_EDGE ( 'NONE', *, *, #1566, .F. ) ;
#89756=CARTESIAN_POINT ( 'NONE',  ( 72.03003869383933022, 67.53192604503671248, -11.37324896331792345 ) ) ;
#89761=CARTESIAN_POINT ( 'NONE',  ( 76.51707580940211528, 54.71355426065986194, 16.11649618684974428 ) ) ;
#89768=CARTESIAN_POINT ( 'NONE',  ( 16.25994779760269182, 31.16126292948895227, -6.180339887498951690 ) ) ;
#89780=CARTESIAN_POINT ( 'NONE',  ( 85.49770414599811375, 44.29146548767710101, 7.659876876720736583 ) ) ;
#89781=CARTESIAN_POINT ( 'NONE',  ( 23.12210336471560623, 25.30066082961422325, -10.00000000000000533 ) ) ;
#89782=CARTESIAN_POINT ( 'NONE',  ( 85.39369755680034757, 48.58767798792116821, 12.46940421135661481 ) ) ;
#89784=CARTESIAN_POINT ( 'NONE',  ( 72.06656620204616104, 72.31304997165260318, -3.465063205002326452 ) ) ;
#89785=CARTESIAN_POINT ( 'NONE',  ( 74.11229751948719979, 55.49134365809288028, -16.11695285934779065 ) ) ;
#89799=CARTESIAN_POINT ( 'NONE',  ( 78.72005499730052236, 59.93730459920318765, 16.11786052172796957 ) ) ;
#89800=CARTESIAN_POINT ( 'NONE',  ( 36.75658403392715456, 24.14754757982092315, -5.678558825948276656 ) ) ;
#89804=CARTESIAN_POINT ( 'NONE',  ( 66.31795133315472413, 69.20145725301702555, 2.477662600322605879 ) ) ;
#89808=CARTESIAN_POINT ( 'NONE',  ( 11.81506597172265316, 27.79752408145591502, -5.678558825948271327 ) ) ;
#89809=CARTESIAN_POINT ( 'NONE',  ( 71.51113537273407417, 72.37632541024542832, 1.045464050329073080 ) ) ;
#89810=CARTESIAN_POINT ( 'NONE',  ( 82.30806329515122854, 54.25783888570826718, 15.62849564502622535 ) ) ;
#89815=CARTESIAN_POINT ( 'NONE',  ( 27.68909066282341058, 16.39040679176984128, 1.333680081654574804E-15 ) ) ;
#89816=CARTESIAN_POINT ( 'NONE',  ( 75.07322640240430189, 53.47801449719656830, -16.05294907914215585 ) ) ;
#89817=CARTESIAN_POINT ( 'NONE',  ( 81.09886180088987828, 42.51057861825624684, 7.870722850269344484 ) ) ;
#89820=CARTESIAN_POINT ( 'NONE',  ( 67.20229271573394669, 69.31781426814865199, 1.387273778539772628 ) ) ;
#89821=CARTESIAN_POINT ( 'NONE',  ( 66.40550710205239682, 68.63594664406403467, 4.834922236012838326 ) ) ;
#89823=ORIENTED_EDGE ( 'NONE', *, *, #76170, .F. ) ;
#89829=CARTESIAN_POINT ( 'NONE',  ( 88.39284856500222531, 43.98633817645592359, -2.257003550805378733 ) ) ;
#89830=CARTESIAN_POINT ( 'NONE',  ( 80.09948508391848065, 57.43746099958096352, -16.59413991463535964 ) ) ;
#89833=CARTESIAN_POINT ( 'NONE',  ( 78.09472128404415514, 61.02041436207807834, -15.89733411056267975 ) ) ;
#89834=CARTESIAN_POINT ( 'NONE',  ( 78.58954130030575413, 50.31985150518112704, -14.97515835093867409 ) ) ;
#89837=CARTESIAN_POINT ( 'NONE',  ( 81.04951158705246428, 43.05756051927024686, 9.551121383308712964 ) ) ;
#89843=EDGE_LOOP ( 'NONE', ( #36358, #67467, #5868, #3218 ) ) ;
#89859=CARTESIAN_POINT ( 'NONE',  ( 77.52349842883717201, 56.82266075537747696, -16.19943627310666656 ) ) ;
#89867=CARTESIAN_POINT ( 'NONE',  ( 81.22979812886450190, 55.45288652294036069, -16.34461090620092349 ) ) ;
#89873=ORIENTED_EDGE ( 'NONE', *, *, #90378, .F. ) ;
#89881=DIRECTION ( 'NONE',  ( -0.3782958374750610142, 0.000000000000000000, 0.9256847516023164468 ) ) ;
#89890=CARTESIAN_POINT ( 'NONE',  ( 74.43609056695282788, 68.34186375642043743, -11.37380148218260523 ) ) ;
#89891=CARTESIAN_POINT ( 'NONE',  ( 71.74212438849298223, 71.89688598250658913, -2.523334318048504166 ) ) ;
#89892=CARTESIAN_POINT ( 'NONE',  ( 76.38701104150307231, 51.11410097943224429, 16.04685272891217807 ) ) ;
#89893=CARTESIAN_POINT ( 'NONE',  ( 81.85212985314085188, 41.17943844758806193, -5.658149982800025235 ) ) ;
#89898=ORIENTED_EDGE ( 'NONE', *, *, #4916, .T. ) ;
#89904=CARTESIAN_POINT ( 'NONE',  ( 72.52865609843787809, 57.51546068812135815, 16.29679984377914437 ) ) ;
#89905=CARTESIAN_POINT ( 'NONE',  ( 71.52927238475341198, 59.05921948282066580, -15.82638290425087213 ) ) ;
#89906=CARTESIAN_POINT ( 'NONE',  ( 66.41141984641225804, 68.22144906810552811, -4.374511944796394047 ) ) ;
#89911=CARTESIAN_POINT ( 'NONE',  ( 69.30365146289868505, 68.49145811655579053, 7.529959361284295660 ) ) ;
#89912=CARTESIAN_POINT ( 'NONE',  ( 66.18968672750138182, 68.49487770620631011, -4.881532527428047885 ) ) ;
#89918=CARTESIAN_POINT ( 'NONE',  ( 29.31840136419365805, 25.43085787977764056, -9.188101187500008038 ) ) ;
#89922=CARTESIAN_POINT ( 'NONE',  ( 81.98377181849168949, 58.72426045759348057, 0.1209609477998357385 ) ) ;
#89925=CARTESIAN_POINT ( 'NONE',  ( 68.53556746510957964, 64.33380229643456971, 11.71290893539683076 ) ) ;
#89932=ORIENTED_EDGE ( 'NONE', *, *, #29628, .T. ) ;
#89933=CARTESIAN_POINT ( 'NONE',  ( 69.27429168244785274, 67.49347697646621214, 8.920200208771037254 ) ) ;
#89936=CARTESIAN_POINT ( 'NONE',  ( 82.41914487369291464, 41.31337197830497132, 3.340431838514237750 ) ) ;
#89938=B_SPLINE_CURVE_WITH_KNOTS ( 'NONE', 3,
 ( #64567, #11390, #40739, #64060, #25053, #25565, #49360, #65058, #18983, #73179, #17978, #87445, #55430, #95524, #16947, #48872, #86419, #79806, #9360, #2789, #40238, #41240, #71180, #72178, #1776, #26069, #75169, #36137, #59422, #52336, #28045, #5743, #66057, #19495, #29062, #13365, #20466, #67039, #35651, #68041, #97006, #97964, #4769, #89891, #27068, #75656 ),
 .UNSPECIFIED., .F., .F.,
 ( 4, 1, 1, 1, 2, 2, 1, 1, 1, 2, 2, 1, 1, 2, 2, 1, 1, 2, 2, 1, 1, 2, 2, 1, 2, 2, 1, 2, 2, 4 ),
 ( 0.000000000000000000, 0.06250000000001762479, 0.09375000000002652045, 0.1093750000000299621, 0.1171875000000316969, 0.1250000000000334177, 0.1875000000000454359, 0.2187500000000504596, 0.2343750000000519862, 0.2421875000000517919, 0.2500000000000515699, 0.3125000000000497935, 0.3437500000000499600, 0.3593750000000500711, 0.3750000000000501266, 0.4375000000000536793, 0.4687500000000536238, 0.4843750000000536238, 0.5000000000000535127, 0.5625000000000512923, 0.5937500000000489608, 0.6093750000000478506, 0.6250000000000466294, 0.6875000000000398570, 0.7187500000000370814, 0.7500000000000341949, 0.8125000000000272005, 0.8437500000000224265, 0.8750000000000176525, 1.000000000000000000 ),
 .UNSPECIFIED. ) ;
#89941=CARTESIAN_POINT ( 'NONE',  ( 68.88895345938509251, 70.13622972219421570, 2.764439259769861934 ) ) ;
#89943=CARTESIAN_POINT ( 'NONE',  ( 2.403541337051680493, 23.16126292948892740, -6.180339887498951690 ) ) ;
#89946=CARTESIAN_POINT ( 'NONE',  ( 73.65799801046682660, 55.43801576298897515, 16.58642910536338633 ) ) ;
#89955=ORIENTED_EDGE ( 'NONE', *, *, #40532, .T. ) ;
#89959=CARTESIAN_POINT ( 'NONE',  ( 81.21547345588363953, 42.27537644322796950, -7.379875351412039208 ) ) ;
#89964=CARTESIAN_POINT ( 'NONE',  ( 80.42949956019809576, 46.69659513737585144, 12.58869027114300820 ) ) ;
#89968=ORIENTED_EDGE ( 'NONE', *, *, #95173, .T. ) ;
#89974=CARTESIAN_POINT ( 'NONE',  ( 73.90428922879758034, 67.91979487962545647, -11.48018831094223025 ) ) ;
#89977=CARTESIAN_POINT ( 'NONE',  ( 66.00998368741205979, 68.68708060386751413, -0.4081457534283032262 ) ) ;
#89978=CARTESIAN_POINT ( 'NONE',  ( 13.91516400911260298, 10.96004757982088584, -5.678558825948276656 ) ) ;
#89987=ADVANCED_FACE ( 'NONE', ( #5406 ), #70290, .T. ) ;
#89990=CARTESIAN_POINT ( 'NONE',  ( 70.35604517217940668, 61.15948129931610566, 14.31845027234643375 ) ) ;
#89994=CARTESIAN_POINT ( 'NONE',  ( 88.29571403098292137, 44.29400929412249610, -2.002076236142582122 ) ) ;
#89997=CARTESIAN_POINT ( 'NONE',  ( 77.10839581433575063, 61.44820719566746448, -15.66518503319612066 ) ) ;
#89998=ORIENTED_EDGE ( 'NONE', *, *, #54891, .T. ) ;
#90003=CARTESIAN_POINT ( 'NONE',  ( 81.11634633033922626, 44.85415553531951360, -10.71945838295695808 ) ) ;
#90006=CARTESIAN_POINT ( 'NONE',  ( 88.07864672190808619, 43.84249974723677212, 2.482382391715414194 ) ) ;
#90009=AXIS2_PLACEMENT_3D ( 'NONE', #56702, #64814, #22922 ) ;
#90010=ORIENTED_EDGE ( 'NONE', *, *, #28697, .F. ) ;
#90014=EDGE_CURVE ( 'NONE', #73177, #83882, #37240, .T. ) ;
#90018=CARTESIAN_POINT ( 'NONE',  ( 70.57121147093401703, 70.14490917978909579, 6.900396944493546236 ) ) ;
#90024=CARTESIAN_POINT ( 'NONE',  ( 78.82063543606528810, 55.18920479240949817, 16.06735020332761721 ) ) ;
#90030=CARTESIAN_POINT ( 'NONE',  ( 84.22641972556617418, 50.60946249816755227, 13.78776958506131933 ) ) ;
#90035=EDGE_CURVE ( 'NONE', #46807, #27838, #21106, .T. ) ;
#90044=CARTESIAN_POINT ( 'NONE',  ( 75.84977083960791333, 65.49147256048033228, 14.30114164871030979 ) ) ;
#90045=CARTESIAN_POINT ( 'NONE',  ( 79.96041668311714545, 44.45513045632799276, 11.65481888797057053 ) ) ;
#90047=CARTESIAN_POINT ( 'NONE',  ( 40.90268743793880901, 35.56628583063844218, 9.188101187500006262 ) ) ;
#90051=CARTESIAN_POINT ( 'NONE',  ( 23.42942861845947178, 22.03085787977762777, 9.188101187500006262 ) ) ;
#90052=CARTESIAN_POINT ( 'NONE',  ( 16.96546585850747491, 10.76426979415088603, 3.090169943749476733 ) ) ;
#90056=ADVANCED_FACE ( 'NONE', ( #70120 ), #24531, .T. ) ;
#90060=CARTESIAN_POINT ( 'NONE',  ( 70.54892256928862082, 60.87711404068373611, 14.48624038529373692 ) ) ;
#90061=CARTESIAN_POINT ( 'NONE',  ( 76.03323602888910671, 65.53324422044475739, -14.33394004605309036 ) ) ;
#90070=CARTESIAN_POINT ( 'NONE',  ( 83.74409828966761893, 41.70414196250850836, 1.316375386105367973 ) ) ;
#90077=CARTESIAN_POINT ( 'NONE',  ( 88.05604604623943032, 44.30204071979397185, -4.408624695025144646 ) ) ;
#90079=LINE ( 'NONE', #68219, #7595 ) ;
#90080=CIRCLE ( 'NONE', #78700, 15.60714546451156970 ) ;
#90082=CARTESIAN_POINT ( 'NONE',  ( 76.92488294255016967, 59.33389770090989401, -15.98887582225194315 ) ) ;
#90091=CARTESIAN_POINT ( 'NONE',  ( 85.35998281785300890, 48.55136375776380930, 12.45655298324007632 ) ) ;
#90096=CARTESIAN_POINT ( 'NONE',  ( 76.93764771006534886, 63.33963654317832948, -15.47180374620822008 ) ) ;
#90097=CARTESIAN_POINT ( 'NONE',  ( 78.94581588320816934, 59.75573664777502358, 16.49495449398541425 ) ) ;
#90104=CARTESIAN_POINT ( 'NONE',  ( 87.09255433220386067, 46.36910785074704933, -8.684712773181464840 ) ) ;
#90107=CARTESIAN_POINT ( 'NONE',  ( 34.45917901495312208, 20.86426979415091765, -3.090169943749474069 ) ) ;
#90112=VERTEX_POINT ( 'NONE', #94984 ) ;
#90115=CARTESIAN_POINT ( 'NONE',  ( 24.58352123714976045, 26.14441083166261848, 10.00000000000000533 ) ) ;
#90116=CARTESIAN_POINT ( 'NONE',  ( 66.76298077169236933, 68.73162322739956664, -3.360950600179818615 ) ) ;
#90118=CARTESIAN_POINT ( 'NONE',  ( 69.40417236955050839, 62.75999532108927781, -13.75910047794655888 ) ) ;
#90123=CARTESIAN_POINT ( 'NONE',  ( 82.55658783523657007, 52.19925090473437024, 14.89975261573945353 ) ) ;
#90124=CARTESIAN_POINT ( 'NONE',  ( 82.37981659293198788, 40.82262905711825596, -3.714377343554210675 ) ) ;
#90129=CARTESIAN_POINT ( 'NONE',  ( 72.14978007694548978, 72.25075206688683238, 3.885827817524732275 ) ) ;
#90130=EDGE_CURVE ( 'NONE', #52772, #90841, #96984, .T. ) ;
#90134=CARTESIAN_POINT ( 'NONE',  ( 79.91228614544331776, 49.76825289431341304, 14.47702846840523883 ) ) ;
#90145=CARTESIAN_POINT ( 'NONE',  ( 16.11573996861870128, 9.708529653044783103, 1.583844403245364907 ) ) ;
#90146=CARTESIAN_POINT ( 'NONE',  ( 34.80818111321084274, 38.83478043621391151, -8.090169943749479842 ) ) ;
#90148=CARTESIAN_POINT ( 'NONE',  ( 82.33860354803769610, 54.25881085800082104, 15.62396609633239386 ) ) ;
#90150=CARTESIAN_POINT ( 'NONE',  ( 71.93253201618666992, 72.27632922802737880, 3.295383250428983946 ) ) ;
#90162=CARTESIAN_POINT ( 'NONE',  ( 31.84840506572257723, 40.16126292948897003, -6.180339887498951690 ) ) ;
#90167=CARTESIAN_POINT ( 'NONE',  ( 5.558032429380089567, 24.18502408145590010, 5.678558825948277544 ) ) ;
#90172=CARTESIAN_POINT ( 'NONE',  ( 73.05076519265766422, 63.10628205629707566, 14.17491965763273853 ) ) ;
#90181=ORIENTED_EDGE ( 'NONE', *, *, #218, .F. ) ;
#90189=CARTESIAN_POINT ( 'NONE',  ( 27.20206195878591870, 37.74646525600392266, 2.839279412974139660 ) ) ;
#90191=CARTESIAN_POINT ( 'NONE',  ( 86.53588498072504365, 47.33349044025582231, -10.24843137454403674 ) ) ;
#90196=CARTESIAN_POINT ( 'NONE',  ( 22.39139443204644664, 24.87878583063842086, -9.188101187500006262 ) ) ;
#90197=CARTESIAN_POINT ( 'NONE',  ( 22.59275855922847498, 34.81751292744058190, -6.180339887498951690 ) ) ;
#90200=ORIENTED_EDGE ( 'NONE', *, *, #15660, .F. ) ;
#90204=B_SPLINE_CURVE_WITH_KNOTS ( 'NONE', 3,
 ( #4727, #70490, #54786, #68988, #53774, #54270, #24398, #55273, #69492, #63396, #99912, #46172, #15277, #38074, #1104, #23381, #596, #93844, #47188, #84736, #30498, #86252, #8698, #7188 ),
 .UNSPECIFIED., .F., .F.,
 ( 4, 2, 2, 2, 2, 2, 2, 2, 2, 2, 2, 4 ),
 ( 0.000000000000000000, 0.1250000000000101308, 0.2500000000000202616, 0.3750000000000304201, 0.4375000000000273670, 0.5000000000000243139, 0.5625000000000213163, 0.6250000000000182077, 0.6875000000000152101, 0.7500000000000121014, 0.8750000000000061062, 1.000000000000000000 ),
 .UNSPECIFIED. ) ;
#90215=B_SPLINE_CURVE_WITH_KNOTS ( 'NONE', 3,
 ( #80458, #64208, #56606, #41902, #26713, #32306, #63208, #71329, #88574, #57093, #96149, #33307, #11029, #1920, #39881, #40389 ),
 .UNSPECIFIED., .F., .F.,
 ( 4, 1, 2, 2, 2, 1, 2, 2, 4 ),
 ( 0.000000000000000000, 0.1249999999999978351, 0.1874999999999980294, 0.2499999999999982236, 0.5000000000000008882, 0.6250000000000035527, 0.6875000000000035527, 0.7500000000000034417, 1.000000000000000000 ),
 .UNSPECIFIED. ) ;
#90216=ADVANCED_FACE ( 'NONE', ( #82780 ), #29043, .T. ) ;
#90220=EDGE_LOOP ( 'NONE', ( #80237, #66769, #75785, #79397 ) ) ;
#90259=EDGE_CURVE ( 'NONE', #81326, #45691, #54796, .T. ) ;
#90263=CARTESIAN_POINT ( 'NONE',  ( 76.19782269962939836, 53.23845936708418947, 15.97715781805315949 ) ) ;
#90265=CARTESIAN_POINT ( 'NONE',  ( 80.85980389730832485, 50.83193235690592360, 14.69879135629361500 ) ) ;
#90275=CARTESIAN_POINT ( 'NONE',  ( 13.14225634397871367, 29.36126292948895156, 6.180339887498949913 ) ) ;
#90278=CARTESIAN_POINT ( 'NONE',  ( 22.83062064355499032, 21.38052372038641380, 10.00000000000000533 ) ) ;
#90282=ADVANCED_FACE ( 'NONE', ( #83259 ), #63674, .T. ) ;
#90287=CARTESIAN_POINT ( 'NONE',  ( 66.52985639494735892, 67.77629683309557151, -6.953963155367802074 ) ) ;
#90291=CARTESIAN_POINT ( 'NONE',  ( 24.00897855452593888, 29.56454794089042082, 10.00000000000000355 ) ) ;
#90292=CARTESIAN_POINT ( 'NONE',  ( 85.66514145605599140, 48.89467697360638709, 12.11710310453397099 ) ) ;
#90295=CARTESIAN_POINT ( 'NONE',  ( 85.51062282364698319, 48.96702101389664108, -12.23238128493630583 ) ) ;
#90296=CARTESIAN_POINT ( 'NONE',  ( 73.85266254684545117, 55.03492225557787521, -16.12802322512867548 ) ) ;
#90299=CARTESIAN_POINT ( 'NONE',  ( 75.48012123268173923, 53.33211347945791658, 16.49774674168797617 ) ) ;
#90306=CARTESIAN_POINT ( 'NONE',  ( 72.82956929615318131, 70.88121797294114401, -7.877017184599606203 ) ) ;
#90308=CARTESIAN_POINT ( 'NONE',  ( 40.31210609084968866, 28.98920272979929535, 7.433330006724137462 ) ) ;
#90314=EDGE_CURVE ( 'NONE', #31643, #83325, #55297, .T. ) ;
#90315=CARTESIAN_POINT ( 'NONE',  ( 15.13723537722347778, 17.24335787977762280, -9.188101187500008038 ) ) ;
#90317=CARTESIAN_POINT ( 'NONE',  ( 82.78605335669568888, 53.79744310428999654, 15.41452286606368283 ) ) ;
#90326=CARTESIAN_POINT ( 'NONE',  ( 67.56996644992010204, 69.57760016826152594, 0.9047167175399849492 ) ) ;
#90327=CARTESIAN_POINT ( 'NONE',  ( 66.69731441546797157, 68.33447113151889596, 4.530513419427100175 ) ) ;
#90329=VERTEX_POINT ( 'NONE', #18832 ) ;
#90337=CARTESIAN_POINT ( 'NONE',  ( 80.42785451945398734, 57.51445601405281138, -16.58998511169260937 ) ) ;
#90340=CARTESIAN_POINT ( 'NONE',  ( 87.69605122943771391, 45.27158203283479310, -6.304490442501953673 ) ) ;
#90355=CARTESIAN_POINT ( 'NONE',  ( 73.66300103671132149, 69.67160076658454670, 9.549075820628328160 ) ) ;
#90364=CARTESIAN_POINT ( 'NONE',  ( 73.30040493051414785, 58.25693415237071804, -15.77479770186053898 ) ) ;
#90365=CARTESIAN_POINT ( 'NONE',  ( 31.25301259707286050, 39.81751292744058901, -6.180339887498951690 ) ) ;
#90368=CARTESIAN_POINT ( 'NONE',  ( 67.22111511317197596, 66.59540578004832412, 8.496167826198702144 ) ) ;
#90373=ORIENTED_EDGE ( 'NONE', *, *, #12801, .F. ) ;
#90375=CARTESIAN_POINT ( 'NONE',  ( 77.89973555931712212, 53.60260371492954334, -15.91514005743381155 ) ) ;
#90377=CARTESIAN_POINT ( 'NONE',  ( 79.53682116969469007, 45.82036653282950311, 12.91785852832784265 ) ) ;
#90378=EDGE_CURVE ( 'NONE', #78755, #47892, #59640, .T. ) ;
#90384=CARTESIAN_POINT ( 'NONE',  ( 83.89296645697339727, 43.48164506579582422, 7.866080993069674676 ) ) ;
#90401=CARTESIAN_POINT ( 'NONE',  ( 88.22316733864592209, 44.26875609612613971, 2.029272769359137474 ) ) ;
#90402=CARTESIAN_POINT ( 'NONE',  ( 82.07381172419997029, 41.42616999410403622, -5.934122665073511271 ) ) ;
#90403=CARTESIAN_POINT ( 'NONE',  ( 14.09675671201943992, 9.108019796199272378, 3.090169943749476733 ) ) ;
#90407=AXIS2_PLACEMENT_3D ( 'NONE', #87936, #88940, #19500 ) ;
#90408=ORIENTED_EDGE ( 'NONE', *, *, #3460, .F. ) ;
#90418=CARTESIAN_POINT ( 'NONE',  ( 6.499975723459110455, 22.49103043416547010, -8.090169943749479842 ) ) ;
#90419=CARTESIAN_POINT ( 'NONE',  ( 79.27712787825650764, 45.82676469203064329, -12.41914995154098911 ) ) ;
#90421=CARTESIAN_POINT ( 'NONE',  ( 66.71234638643888104, 68.39628657080208995, -4.370994838407439964 ) ) ;
#90425=CARTESIAN_POINT ( 'NONE',  ( 70.20553746537656536, 69.89474460070350403, 5.933681650480220782 ) ) ;
#90426=CARTESIAN_POINT ( 'NONE',  ( 66.38800753050692549, 68.05348521546564200, -4.839280302337260586 ) ) ;
#90432=CARTESIAN_POINT ( 'NONE',  ( 26.18025557360336464, 27.06628583063842797, -9.188101187500006262 ) ) ;
#90437=CARTESIAN_POINT ( 'NONE',  ( 74.92881689719639837, 67.14644430943499742, 12.99852016367276875 ) ) ;
#90448=CARTESIAN_POINT ( 'NONE',  ( 68.43551180206651452, 65.84368784619988446, 10.25479611292870885 ) ) ;
#90450=CARTESIAN_POINT ( 'NONE',  ( 71.94311743993219466, 72.25799473628046599, 0.6149828437083229016 ) ) ;
#90454=CARTESIAN_POINT ( 'NONE',  ( 69.20334762877976686, 70.41346677573686463, 2.281924207914373781 ) ) ;
#90458=CARTESIAN_POINT ( 'NONE',  ( 16.97222724706318076, 11.92755873383624632, 6.180339887498953466 ) ) ;
#90473=CARTESIAN_POINT ( 'NONE',  ( 73.09452573934707686, 69.60050248057373778, -9.839270276345128963 ) ) ;
#90485=CARTESIAN_POINT ( 'NONE',  ( 82.63495489645998759, 40.85464596424811390, 3.248838194811724200 ) ) ;
#90490=CARTESIAN_POINT ( 'NONE',  ( 71.06913592625164711, 68.39894819183987806, -9.182066607298049021 ) ) ;
#90493=CARTESIAN_POINT ( 'NONE',  ( 77.12841425132344852, 62.56755827935163694, 15.36159490606874556 ) ) ;
#90494=CARTESIAN_POINT ( 'NONE',  ( 9.401013375279877238, 17.37878583063838889, 9.188101187500006262 ) ) ;
#90503=CARTESIAN_POINT ( 'NONE',  ( 70.36532766715068021, 61.07443295118657289, 14.35799568614401345 ) ) ;
#90510=CARTESIAN_POINT ( 'NONE',  ( 68.90560621877192204, 63.79076715805910425, -12.30144644517788421 ) ) ;
#90519=CARTESIAN_POINT ( 'NONE',  ( 76.06516313603486878, 65.42396348981594656, 14.39793886682782187 ) ) ;
#90526=CARTESIAN_POINT ( 'NONE',  ( 68.12913145924295577, 66.36538084368893919, -9.493516625238422435 ) ) ;
#90527=CARTESIAN_POINT ( 'NONE',  ( 67.04719753439840702, 66.82148211118030190, -8.940350841082095101 ) ) ;
#90528=CARTESIAN_POINT ( 'NONE',  ( 86.73093147390520130, 43.68969761139900498, 3.372955308790926754 ) ) ;
#90529=CARTESIAN_POINT ( 'NONE',  ( 84.55460127224613132, 47.09886495345954671, 11.09894356431207818 ) ) ;
#90535=CARTESIAN_POINT ( 'NONE',  ( 78.51615055793223519, 53.63995692175274854, 15.85712610117593080 ) ) ;
#90539=DIRECTION ( 'NONE',  ( 0.8116583814955234955, 0.01378320505841451778, 0.5839697723396178874 ) ) ;
#90542=CARTESIAN_POINT ( 'NONE',  ( 70.60537956472130361, 60.95729775083580648, -14.46506356667156190 ) ) ;
#90543=CARTESIAN_POINT ( 'NONE',  ( 84.85964987685913741, 50.19146562821751445, 13.75030272624154470 ) ) ;
#90550=CARTESIAN_POINT ( 'NONE',  ( 8.859747497914600700, 17.06628583063839599, -9.188101187500006262 ) ) ;
#90555=CARTESIAN_POINT ( 'NONE',  ( 83.93039057805418679, 42.25368239170656182, -3.699647659905914931 ) ) ;
#90560=CARTESIAN_POINT ( 'NONE',  ( 42.48198750171711424, 33.03085787977767041, 9.188101187500006262 ) ) ;
#90562=FACE_BOUND ( 'NONE', #34009, .T. ) ;
#90564=CARTESIAN_POINT ( 'NONE',  ( 24.44820476603448611, 26.06628583063842086, -9.188101187500006262 ) ) ;
#90565=AXIS2_PLACEMENT_3D ( 'NONE', #39230, #31633, #84396 ) ;
#90569=VERTEX_POINT ( 'NONE', #17942 ) ;
#90570=CARTESIAN_POINT ( 'NONE',  ( 70.58551217508033915, 60.91456802530846915, 15.00778779846412192 ) ) ;
#90579=DIRECTION ( 'NONE',  ( -0.8660254037844378194, -0.5000000000000014433, -0.000000000000000000 ) ) ;
#90581=ORIENTED_EDGE ( 'NONE', *, *, #80604, .T. ) ;
#90583=CARTESIAN_POINT ( 'NONE',  ( 83.66501680638440064, 41.65036927881936890, 1.209882539926571354 ) ) ;
#90584=ADVANCED_FACE ( 'NONE', ( #41204 ), #86886, .T. ) ;
#90585=ORIENTED_EDGE ( 'NONE', *, *, #49000, .F. ) ;
#90587=VERTEX_POINT ( 'NONE', #31604 ) ;
#90588=DIRECTION ( 'NONE',  ( 0.3213938048432692374, -0.5566703992264209200, -0.7660444431189770143 ) ) ;
#90589=CARTESIAN_POINT ( 'NONE',  ( 3.297978757390601423, 24.83705186507751606, 3.090169943749475401 ) ) ;
#90594=CARTESIAN_POINT ( 'NONE',  ( 39.98734656443052415, 28.80170272979929535, 7.433330006724137462 ) ) ;
#90595=CARTESIAN_POINT ( 'NONE',  ( 78.02766155223862654, 58.91636306235935905, -16.12600223474660410 ) ) ;
#90597=CARTESIAN_POINT ( 'NONE',  ( 87.55848707468658176, 45.50985013822432990, 6.922438743303467312 ) ) ;
#90598=ORIENTED_EDGE ( 'NONE', *, *, #64639, .T. ) ;
#90604=CARTESIAN_POINT ( 'NONE',  ( 77.57770355975000598, 59.80217626084218097, -16.01913283567768076 ) ) ;
#90607=CARTESIAN_POINT ( 'NONE',  ( 76.86986466358051473, 64.04458250793000218, -15.20481942635857742 ) ) ;
#90617=CARTESIAN_POINT ( 'NONE',  ( 87.04951863019347513, 45.82536234993809643, -8.629913247614998895 ) ) ;
#90631=CARTESIAN_POINT ( 'NONE',  ( 67.95642171729713255, 69.05834527840744386, -4.640993296857849337 ) ) ;
#90633=CARTESIAN_POINT ( 'NONE',  ( 69.40753887930063115, 62.89835586300766579, -13.67854514043513525 ) ) ;
#90639=CARTESIAN_POINT ( 'NONE',  ( 71.14846176242140530, 61.60121696541033742, 14.32671748640477460 ) ) ;
#90644=CARTESIAN_POINT ( 'NONE',  ( 71.78913936505468030, 72.20160104369585952, 3.260718063500199548 ) ) ;
#90645=CARTESIAN_POINT ( 'NONE',  ( 83.26766257861952170, 43.36122241240380504, 7.252070224612332972 ) ) ;
#90648=CARTESIAN_POINT ( 'NONE',  ( 79.65794105133953451, 48.82961183344457368, 14.10136067249946024 ) ) ;
#90649=CARTESIAN_POINT ( 'NONE',  ( 68.03078532392423483, 69.75226796743223190, -1.878725101587667146 ) ) ;
#90652=DIRECTION ( 'NONE',  ( 0.8660254037844399289, 0.4999999999999977240, -0.000000000000000000 ) ) ;
#90654=CARTESIAN_POINT ( 'NONE',  ( 66.63322413591409088, 67.62875759604085601, 6.186734474800332784 ) ) ;
#90660=CARTESIAN_POINT ( 'NONE',  ( 70.80322137413752159, 60.50400129575321273, -14.70302039727343413 ) ) ;
#90661=CARTESIAN_POINT ( 'NONE',  ( 35.07028576228009342, 43.18080186712595747, 3.090169943749475401 ) ) ;
#90664=CARTESIAN_POINT ( 'NONE',  ( 82.43809236625457970, 54.24053208071835286, 15.60321882952343842 ) ) ;
#90665=CARTESIAN_POINT ( 'NONE',  ( 72.10617024684211174, 72.18421392457028674, 4.031754617348227043 ) ) ;
#90668=CARTESIAN_POINT ( 'NONE',  ( 46.74164954608104949, 27.39040679176987325, -6.890680421881970419E-14 ) ) ;
#90669=CARTESIAN_POINT ( 'NONE',  ( 77.53589688945717739, 51.31089695689070851, -15.44518354484521083 ) ) ;
#90670=CARTESIAN_POINT ( 'NONE',  ( 72.00459748831643481, 72.21134089809413581, -1.634945730901812722 ) ) ;
#90673=CARTESIAN_POINT ( 'NONE',  ( 19.57800816787531062, 26.70171378149919050, -9.188101187500004485 ) ) ;
#90676=CARTESIAN_POINT ( 'NONE',  ( 3.278110179240818045, 23.93396525600387648, 2.839279412974139660 ) ) ;
#90678=CARTESIAN_POINT ( 'NONE',  ( 75.83332386201834652, 58.24149532073650448, 16.46778979864901160 ) ) ;
#90680=CARTESIAN_POINT ( 'NONE',  ( 82.21717897060236169, 40.84507121292054421, -1.199451623573249970 ) ) ;
#90681=CARTESIAN_POINT ( 'NONE',  ( 71.08662668937095930, 67.82508006278297330, -9.836311824178357810 ) ) ;
#90700=CARTESIAN_POINT ( 'NONE',  ( 86.40862467444883066, 43.51472063525788059, 4.903409472307490802 ) ) ;
#90701=FACE_OUTER_BOUND ( 'NONE', #8046, .T. ) ;
#90704=CARTESIAN_POINT ( 'NONE',  ( 17.01121839442928163, 30.79752408145592568, -5.678558825948271327 ) ) ;
#90705=CARTESIAN_POINT ( 'NONE',  ( 76.13725175568590942, 60.79812444030506668, 15.65525560863753896 ) ) ;
#90706=CARTESIAN_POINT ( 'NONE',  ( 72.54520184348785961, 70.27380328412901633, -7.860630163369380696 ) ) ;
#90707=CARTESIAN_POINT ( 'NONE',  ( 75.28634535225387481, 66.86406054372800156, -12.88709815648634383 ) ) ;
#90710=CARTESIAN_POINT ( 'NONE',  ( 76.87300970902636266, 55.60219541319754200, 16.60077664465815417 ) ) ;
#90714=VECTOR ( 'NONE', #28530, 1000.000000000000227 ) ;
#90716=CARTESIAN_POINT ( 'NONE',  ( 70.82117999291602928, 62.89421842260256312, 14.15644170336123153 ) ) ;
#90719=CARTESIAN_POINT ( 'NONE',  ( 66.41647611861264977, 68.75673559357331044, -2.143700313894566278 ) ) ;
#90721=CARTESIAN_POINT ( 'NONE',  ( 84.68093819348166562, 42.16537887657799644, 0.2499978311480390847 ) ) ;
#90737=CARTESIAN_POINT ( 'NONE',  ( 73.05863210132505969, 69.60576123971951290, -9.808587366596233537 ) ) ;
#90744=CARTESIAN_POINT ( 'NONE',  ( 66.38217553272322391, 68.79393763757845193, -4.316952526664222134 ) ) ;
#90747=CARTESIAN_POINT ( 'NONE',  ( 76.05851436047953484, 51.43505017026153325, -16.15825921707162394 ) ) ;
#90756=EDGE_CURVE ( 'NONE', #94179, #64640, #88265, .T. ) ;
#90761=CARTESIAN_POINT ( 'NONE',  ( 71.35329583521033214, 67.64943209593164397, -10.88520583469783887 ) ) ;
#90763=CARTESIAN_POINT ( 'NONE',  ( 72.99046944781451884, 70.71697578006111939, 8.277156641257130687 ) ) ;
#90766=CARTESIAN_POINT ( 'NONE',  ( 76.39332965939082953, 54.12380165434665003, 16.07031247584009392 ) ) ;
#90769=CARTESIAN_POINT ( 'NONE',  ( 72.62522464330835703, 71.47837554186844500, -5.665107215650756700 ) ) ;
#90770=CARTESIAN_POINT ( 'NONE',  ( 81.68759648889933089, 55.58869686435339474, 15.96161034574013904 ) ) ;
#90776=CARTESIAN_POINT ( 'NONE',  ( 28.02677306626161879, 24.38052372038642091, 10.00000000000000533 ) ) ;
#90777=CARTESIAN_POINT ( 'NONE',  ( 82.07265110639774264, 53.99302234254209054, 15.59308437138325587 ) ) ;
#90782=CARTESIAN_POINT ( 'NONE',  ( 71.88142767616335504, 71.70553083785841864, -3.832731862061182326 ) ) ;
#90786=CARTESIAN_POINT ( 'NONE',  ( 67.15201250546462575, 67.74620447341509077, -6.543367556292805531 ) ) ;
#90787=CARTESIAN_POINT ( 'NONE',  ( 73.08131391382630682, 70.69050563043288093, -7.679366471979098385 ) ) ;
#90791=CARTESIAN_POINT ( 'NONE',  ( 22.17733255989135088, 35.73705186507754661, -3.090169943749475845 ) ) ;
#90792=CARTESIAN_POINT ( 'NONE',  ( 85.29796244568555608, 48.43343408700369679, 12.39349753750686034 ) ) ;
#90794=CARTESIAN_POINT ( 'NONE',  ( 72.03718002748324523, 71.77198201402653410, -3.924036090042733349 ) ) ;
#90801=CARTESIAN_POINT ( 'NONE',  ( 69.81582973455007846, 63.14295414310246457, -13.67321376818635059 ) ) ;
#90806=CARTESIAN_POINT ( 'NONE',  ( 43.17480782474465428, 33.43085787977766898, -9.188101187500008038 ) ) ;
#90813=SHAPE_DEFINITION_REPRESENTATION ( #87215, #46310 ) ;
#90814=CARTESIAN_POINT ( 'NONE',  ( 16.25825050073692069, 15.10170272979925876, -7.433330006724141015 ) ) ;
#90816=CARTESIAN_POINT ( 'NONE',  ( 82.98423510826575011, 53.52344736239028578, 15.67380116644084076 ) ) ;
#90817=CARTESIAN_POINT ( 'NONE',  ( 71.40044295081541748, 59.41588353585593296, 15.70283061017000925 ) ) ;
#90820=CARTESIAN_POINT ( 'NONE',  ( 85.97213429613141500, 45.53948383454844873, -8.355993802508837831 ) ) ;
#90822=CARTESIAN_POINT ( 'NONE',  ( 81.40724292810348572, 41.99019188331313757, 7.748015485544303971 ) ) ;
#90823=EDGE_CURVE ( 'NONE', #78334, #11388, #63241, .T. ) ;
#90838=CARTESIAN_POINT ( 'NONE',  ( 31.70419723673859025, 18.70852965304479909, 1.583844403245330712 ) ) ;
#90841=VERTEX_POINT ( 'NONE', #44573 ) ;
#90842=CARTESIAN_POINT ( 'NONE',  ( 87.43441255672811963, 45.02171211745687884, -6.109614425055893250 ) ) ;
#90844=CARTESIAN_POINT ( 'NONE',  ( 81.11499192049835472, 43.08689460941847926, 9.540678225713152827 ) ) ;
#90847=CARTESIAN_POINT ( 'NONE',  ( 74.96484514675771038, 65.34853496422127250, 13.65623017033944997 ) ) ;
#90848=ORIENTED_EDGE ( 'NONE', *, *, #19494, .F. ) ;
#90859=CARTESIAN_POINT ( 'NONE',  ( 73.65729962767424865, 69.49757902785616182, 9.740712345197151123 ) ) ;
#90861=CARTESIAN_POINT ( 'NONE',  ( 82.56035143084491779, 53.86840602817222390, 15.84327991562211757 ) ) ;
#90862=CARTESIAN_POINT ( 'NONE',  ( 19.62422909362874535, 11.73415679381821342, 1.333680081654574804E-15 ) ) ;
#90868=CARTESIAN_POINT ( 'NONE',  ( 73.48578390778760649, 58.20067181093861564, -15.80716316672890009 ) ) ;
#90869=CARTESIAN_POINT ( 'NONE',  ( 30.67947171958994090, 41.21091486745863364, -1.111400068045478839E-16 ) ) ;
#90871=CARTESIAN_POINT ( 'NONE',  ( 67.88685699899777148, 70.31731532184431899, 0.4175378299487736422 ) ) ;
#90878=CARTESIAN_POINT ( 'NONE',  ( 76.09838423539584085, 54.19830694069673171, -16.08845863169665336 ) ) ;
#90881=CARTESIAN_POINT ( 'NONE',  ( 79.70171752247047436, 45.99846658741579120, 12.97553337965657860 ) ) ;
#90901=CARTESIAN_POINT ( 'NONE',  ( 81.66730501177755741, 41.57387089987508944, -5.459456342607252211 ) ) ;
#90904=CARTESIAN_POINT ( 'NONE',  ( 68.59321919598859552, 64.61334443947949069, -12.16043161807688300 ) ) ;
#90913=CARTESIAN_POINT ( 'NONE',  ( 4.767924915890233706, 21.49103043416546654, -8.090169943749479842 ) ) ;
#90915=CARTESIAN_POINT ( 'NONE',  ( 71.75564132893636327, 58.72497181799866439, -15.45604496957676233 ) ) ;
#90916=CARTESIAN_POINT ( 'NONE',  ( 73.23925880138965283, 69.80348372919694100, 9.104443575153400303 ) ) ;
#90921=CARTESIAN_POINT ( 'NONE',  ( 70.30840464414876578, 70.04154225169172321, 5.745843947021113785 ) ) ;
#90929=CARTESIAN_POINT ( 'NONE',  ( 27.58635055662477953, 24.43085787977765122, -9.188101187500008038 ) ) ;
#90931=CARTESIAN_POINT ( 'NONE',  ( 83.63562430374231838, 51.63275018564552710, -14.84107497619760174 ) ) ;
#90933=CARTESIAN_POINT ( 'NONE',  ( 88.42823867725131493, 44.01048851461693801, 2.280060627005670248 ) ) ;
#90934=CARTESIAN_POINT ( 'NONE',  ( 74.86935717915280009, 67.14205582119099347, 12.97785457704837775 ) ) ;
#90935=CARTESIAN_POINT ( 'NONE',  ( 69.07388362541929894, 64.21813251217939467, 12.04565015971650510 ) ) ;
#90937=CARTESIAN_POINT ( 'NONE',  ( 81.70340159412396019, 53.68629051274507447, 15.93867609236433758 ) ) ;
#90939=CARTESIAN_POINT ( 'NONE',  ( 70.23041638060261960, 67.14587595898601080, -10.73806474816264434 ) ) ;
#90942=VERTEX_POINT ( 'NONE', #98819 ) ;
#90943=CARTESIAN_POINT ( 'NONE',  ( 69.72231879373730123, 68.30382478307210192, 8.176497125895556550 ) ) ;
#90952=CARTESIAN_POINT ( 'NONE',  ( 9.678154728840961951, 27.36126292948894090, 6.180339887498949913 ) ) ;
#90956=CARTESIAN_POINT ( 'NONE',  ( 86.40784109447328376, 47.52432272822921533, -11.05097720836333330 ) ) ;
#90957=CARTESIAN_POINT ( 'NONE',  ( 80.45391135454320874, 45.63592357980512304, -11.76834192579569915 ) ) ;
#90960=CARTESIAN_POINT ( 'NONE',  ( 79.31708208686119121, 59.64451620468177140, -16.52545681491536556 ) ) ;
#90966=CARTESIAN_POINT ( 'NONE',  ( 68.10710844971850975, 70.39465110784678359, 1.444126812255956516 ) ) ;
#90967=CARTESIAN_POINT ( 'NONE',  ( 81.82036482997024507, 42.35048943659092657, -7.944650131497826173 ) ) ;
#90979=CARTESIAN_POINT ( 'NONE',  ( 82.68215287466908592, 53.55713939286302150, -15.73562046651999857 ) ) ;
#90983=CARTESIAN_POINT ( 'NONE',  ( 17.99030130830579566, 16.10170272979926054, -7.433330006724141015 ) ) ;
#90987=ORIENTED_EDGE ( 'NONE', *, *, #72048, .F. ) ;
#90997=CARTESIAN_POINT ( 'NONE',  ( 72.74372184067405556, 62.96568689615059355, -14.16853096237499798 ) ) ;
#91008=ORIENTED_EDGE ( 'NONE', *, *, #67834, .T. ) ;
#91024=CARTESIAN_POINT ( 'NONE',  ( 80.00195504689109782, 53.61111274759718981, -15.70840541018166725 ) ) ;
#91029=CARTESIAN_POINT ( 'NONE',  ( 85.04793144752866851, 49.76842598555752062, 13.42690168825988373 ) ) ;
#91036=CARTESIAN_POINT ( 'NONE',  ( 2.730238736670422384, 24.68290643055184574, 3.479690158560446702E-15 ) ) ;
#91041=CARTESIAN_POINT ( 'NONE',  ( 83.30611589712688669, 42.09688407475692884, -4.353475907038308890 ) ) ;
#91044=CARTESIAN_POINT ( 'NONE',  ( 80.55977923466276991, 44.53388773495298381, 11.41474457630165062 ) ) ;
#91045=CARTESIAN_POINT ( 'NONE',  ( 40.97001837269192492, 24.44966523072497466, -2.296566073217252530E-15 ) ) ;
#91049=CARTESIAN_POINT ( 'NONE',  ( 18.86656744736070124, 32.93396525600390845, 2.839279412974139660 ) ) ;
#91054=( BOUNDED_CURVE ( )  B_SPLINE_CURVE ( 2, ( #74154, #34147, #34629, #97457, #42710, #4746, #35630, #67018, #96479, #66530, #27047, #96982, #80283 ),
 .UNSPECIFIED., .F., .T. ) 
 B_SPLINE_CURVE_WITH_KNOTS ( ( 3, 2, 2, 2, 2, 2, 3 ),
 ( 0.1875000000000000000, 0.1900000000000000022, 0.1950000000000000067, 0.2000000000000000111, 0.2049999999999999878, 0.2099999999999999922, 0.2124999999999999944 ),
 .UNSPECIFIED. ) 
 CURVE ( )  GEOMETRIC_REPRESENTATION_ITEM ( )  RATIONAL_B_SPLINE_CURVE ( ( 0.9755282581475768211, 0.9755282581475768211, 1.000000000000000000, 0.9510565162951535312, 1.000000000000000000, 0.9510565162951535312, 1.000000000000000000, 0.9510565162951535312, 1.000000000000000000, 0.9510565162951535312, 1.000000000000000000, 0.9755282581475768211, 0.9755282581475768211 ) ) 
 REPRESENTATION_ITEM ( '' )  );
#91056=CARTESIAN_POINT ( 'NONE',  ( 70.96429761874149733, 61.15374941682173926, 14.99935025261083688 ) ) ;
#91058=CARTESIAN_POINT ( 'NONE',  ( 73.72587696377917155, 59.63361033315440807, 16.00582498373660556 ) ) ;
#91063=CARTESIAN_POINT ( 'NONE',  ( 71.62510740771190854, 67.51121758376429227, 11.15861874543539400 ) ) ;
#91066=CARTESIAN_POINT ( 'NONE',  ( 84.39844661083043320, 42.18200899752556410, 2.226954688809204885 ) ) ;
#91076=CARTESIAN_POINT ( 'NONE',  ( 35.86231599663030067, 42.74646525600393687, 2.839279412974139660 ) ) ;
#91078=CARTESIAN_POINT ( 'NONE',  ( 77.42588836629299465, 61.59288719192012707, -16.04997787272938936 ) ) ;
#91079=CARTESIAN_POINT ( 'NONE',  ( 85.93470712620026575, 48.23248545518190866, 11.93606436224419376 ) ) ;
#91083=DIRECTION ( 'NONE',  ( 0.7713975076906463002, 0.000000000000000000, 0.6363535849892411056 ) ) ;
#91091=CARTESIAN_POINT ( 'NONE',  ( 77.31293068221884823, 63.17731889312780424, -15.23105203122446838 ) ) ;
#91094=CARTESIAN_POINT ( 'NONE',  ( 83.67416965427615594, 41.61942911856458949, 0.1873010706438003881 ) ) ;
#91095=CARTESIAN_POINT ( 'NONE',  ( 27.02885687802902837, 37.64646525600391413, -2.839279412974133887 ) ) ;
#91099=CARTESIAN_POINT ( 'NONE',  ( 74.05204724713870235, 68.33764315531155376, -11.67956189741113349 ) ) ;
#91104=CARTESIAN_POINT ( 'NONE',  ( 27.28458541428561901, 34.49103043416550918, -8.090169943749479842 ) ) ;
#91116=CARTESIAN_POINT ( 'NONE',  ( 67.79268864257714711, 69.02054886865253991, -4.467901244201882172 ) ) ;
#91117=CARTESIAN_POINT ( 'NONE',  ( 65.82437655349816907, 69.12761348810168727, -0.3171013769033966812 ) ) ;
#91118=CARTESIAN_POINT ( 'NONE',  ( 70.00592750416963383, 62.80307869517519492, -13.36220121966311858 ) ) ;
#91121=B_SPLINE_SURFACE_WITH_KNOTS ( 'NONE', 3, 1, ( 
 ( #33354, #71875 ),
 ( #78989, #31348 ),
 ( #63756, #16154 ),
 ( #54632, #16650 ),
 ( #2473, #94689 ),
 ( #92690, #24748 ),
 ( #17148, #23241 ),
 ( #47052, #39428 ),
 ( #48046, #54128 ),
 ( #56133, #15637 ),
 ( #40438, #62738 ),
 ( #17663, #8065 ),
 ( #62231, #93183 ),
 ( #94194, #93694 ),
 ( #71373, #70347 ),
 ( #47545, #31835 ),
 ( #85091, #32352 ),
 ( #24257, #46534 ),
 ( #69845, #1962 ),
 ( #87131, #86120 ),
 ( #32847, #1471 ),
 ( #55134, #39926 ),
 ( #12564, #2990 ),
 ( #33880, #66255 ),
 ( #56649, #58144 ),
 ( #96692, #4446 ),
 ( #3953, #34836 ),
 ( #27261, #43439 ),
 ( #64765, #97190 ),
 ( #89124, #4964 ),
 ( #25774, #35346 ) ),
 .UNSPECIFIED., .F., .F., .F.,
 ( 4, 3, 3, 3, 3, 3, 3, 3, 3, 3, 4 ),
 ( 2, 2 ),
 ( 0.000000000000000000, 0.1122669598086739884, 0.2243161639709730926, 0.3396355846219151764, 0.4553962076585294505, 0.5677860799922427315, 0.6749047109689578772, 0.7773884377078319474, 0.8775581155834339953, 0.9782364162377981120, 1.000000000000000000 ),
 ( 0.000000000000000000, 1.000000000000000000 ),
 .UNSPECIFIED. ) ;
#91122=CARTESIAN_POINT ( 'NONE',  ( 82.15383659063220989, 50.27708431210408691, 14.14486460422176073 ) ) ;
#91123=CARTESIAN_POINT ( 'NONE',  ( 82.24301957861473511, 40.72317291277653339, -3.636295274160996183 ) ) ;
#91126=CARTESIAN_POINT ( 'NONE',  ( 72.10617024684209753, 72.18421392457030095, 4.031754617348218162 ) ) ;
#91130=CARTESIAN_POINT ( 'NONE',  ( 70.48822326768343771, 61.33110110675399085, -14.80687757298846918 ) ) ;
#91131=CARTESIAN_POINT ( 'NONE',  ( 82.61614429202859355, 53.50419195261176242, -15.73127852458025266 ) ) ;
#91137=CARTESIAN_POINT ( 'NONE',  ( 66.43435659019957029, 67.91024671103048149, 6.587328651168637528 ) ) ;
#91142=CARTESIAN_POINT ( 'NONE',  ( 38.46077748372666605, 37.90829794293884447, 10.00000000000000355 ) ) ;
#91143=CARTESIAN_POINT ( 'NONE',  ( 75.04467193377834633, 57.90891680148014586, -16.45096375161649149 ) ) ;
#91144=CARTESIAN_POINT ( 'NONE',  ( 82.76645177422848576, 53.88639560009900009, 15.44535535711801977 ) ) ;
#91145=CARTESIAN_POINT ( 'NONE',  ( 72.27859001089517221, 72.07364561169796957, 3.260268701118359758 ) ) ;
#91148=CARTESIAN_POINT ( 'NONE',  ( 79.78357408300404074, 50.66639049700688702, -14.85564821779047229 ) ) ;
#91149=CARTESIAN_POINT ( 'NONE',  ( 71.67602448659575032, 72.02732272969839755, -1.570697476799420844 ) ) ;
#91151=CARTESIAN_POINT ( 'NONE',  ( 17.68238808236222326, 31.18502408145591787, 5.678558825948276656 ) ) ;
#91153=CARTESIAN_POINT ( 'NONE',  ( 6.414422030351863313, 19.10171378149916421, 9.188101187500008038 ) ) ;
#91156=CARTESIAN_POINT ( 'NONE',  ( 76.05950007140947378, 59.49804724808203815, 16.31946239994518777 ) ) ;
#91157=EDGE_LOOP ( 'NONE', ( #11328, #17676, #48019, #13658 ) ) ;
#91158=CARTESIAN_POINT ( 'NONE',  ( 72.64134535439403351, 61.55457294482811648, 14.72326246863772781 ) ) ;
#91171=ADVANCED_FACE ( 'NONE', ( #74781 ), #97751, .T. ) ;
#91176=ORIENTED_EDGE ( 'NONE', *, *, #12283, .T. ) ;
#91177=AXIS2_PLACEMENT_3D ( 'NONE', #59363, #4705, #21879 ) ;
#91179=CARTESIAN_POINT ( 'NONE',  ( 79.20708015383932832, 46.31796976865181392, -12.77997348381888187 ) ) ;
#91181=CARTESIAN_POINT ( 'NONE',  ( 73.03195784919465439, 70.41880241001356922, -8.079853440356906447 ) ) ;
#91184=EDGE_LOOP ( 'NONE', ( #79005, #63941, #15323, #96280 ) ) ;
#91185=CARTESIAN_POINT ( 'NONE',  ( 24.50893013558248157, 16.01110640527292261, 2.839279412974134775 ) ) ;
#91186=CARTESIAN_POINT ( 'NONE',  ( 66.93954981368713675, 69.16002812685212575, -1.529596994131542154 ) ) ;
#91187=CARTESIAN_POINT ( 'NONE',  ( 75.18619828000903738, 66.99152146615374193, -12.75634951131107364 ) ) ;
#91188=ORIENTED_EDGE ( 'NONE', *, *, #51324, .T. ) ;
#91198=CYLINDRICAL_SURFACE ( 'NONE', #14083, 16.60714546451156792 ) ;
#91199=CARTESIAN_POINT ( 'NONE',  ( 81.50373498261929228, 55.81176558511297969, 16.37496158676513858 ) ) ;
#91205=CARTESIAN_POINT ( 'NONE',  ( 79.22258912688209875, 45.79454436770367920, 13.02573821740452864 ) ) ;
#91206=ORIENTED_EDGE ( 'NONE', *, *, #4821, .T. ) ;
#91207=CARTESIAN_POINT ( 'NONE',  ( 72.52865609843787809, 57.51546068812135815, 16.29679984377914437 ) ) ;
#91210=CARTESIAN_POINT ( 'NONE',  ( 76.16027975956328078, 65.34306562879338287, 14.46508190410746764 ) ) ;
#91211=CARTESIAN_POINT ( 'NONE',  ( 66.84894034102782712, 67.93781524052256771, 6.996449262558990689 ) ) ;
#91212=DIRECTION ( 'NONE',  ( -0.5000000000000082157, 0.8660254037844338226, 0.000000000000000000 ) ) ;
#91220=EDGE_LOOP ( 'NONE', ( #36334, #88904, #97570, #42542 ) ) ;
#91228=CARTESIAN_POINT ( 'NONE',  ( 69.13511649644314616, 71.04256955909853843, 2.869324681485878275E-06 ) ) ;
#91231=CARTESIAN_POINT ( 'NONE',  ( 87.84403297180379866, 44.29423158952226203, 4.754374079557552868 ) ) ;
#91232=CARTESIAN_POINT ( 'NONE',  ( 85.71285599281509349, 43.91756893743614398, 5.655568829977952738 ) ) ;
#91235=CARTESIAN_POINT ( 'NONE',  ( 79.52110638078222848, 59.35728171255717456, -16.21327867740588857 ) ) ;
#91237=CARTESIAN_POINT ( 'NONE',  ( 71.22189038257839400, 67.26187328387359798, -10.54518486082646511 ) ) ;
#91238=ORIENTED_EDGE ( 'NONE', *, *, #34423, .T. ) ;
#91239=CARTESIAN_POINT ( 'NONE',  ( 76.47762942987780832, 54.52376294675376300, 16.10255537987762153 ) ) ;
#91242=CARTESIAN_POINT ( 'NONE',  ( 82.57480368249606784, 41.04376301281222794, 1.111617510708536205 ) ) ;
#91253=CARTESIAN_POINT ( 'NONE',  ( 23.52344096658253747, 21.78052372038641238, -10.00000000000000355 ) ) ;
#91257=CARTESIAN_POINT ( 'NONE',  ( 66.82849716633455728, 68.92242650857625108, -4.723788943350095693 ) ) ;
#91258=B_SPLINE_CURVE_WITH_KNOTS ( 'NONE', 3,
 ( #43598, #20322, #12734, #83645, #67905, #98825, #89756, #90761, #37480, #5114, #97828, #22296, #68392, #59277, #82663, #20827 ),
 .UNSPECIFIED., .F., .F.,
 ( 4, 1, 2, 2, 2, 1, 2, 2, 4 ),
 ( 0.000000000000000000, 0.1249999999999970024, 0.1874999999999956424, 0.2499999999999942824, 0.4999999999999977796, 0.6249999999999977796, 0.6874999999999976685, 0.7499999999999976685, 1.000000000000000000 ),
 .UNSPECIFIED. ) ;
#91264=CARTESIAN_POINT ( 'NONE',  ( 66.95873798537226662, 67.67772264583786068, -6.456423497743614348 ) ) ;
#91265=CARTESIAN_POINT ( 'NONE',  ( 72.83785029587782844, 70.28570241188594991, -8.113289319485218698 ) ) ;
#91269=CARTESIAN_POINT ( 'NONE',  ( 26.39215011307057424, 23.43677371833802425, -10.00000000000000355 ) ) ;
#91270=CARTESIAN_POINT ( 'NONE',  ( 85.05422843502101671, 48.88568976824796408, 12.38837144396399381 ) ) ;
#91274=EDGE_CURVE ( 'NONE', #97853, #57975, #99497, .T. ) ;
#91284=CARTESIAN_POINT ( 'NONE',  ( 43.77620770598743150, 30.98920272979930601, 7.433330006724137462 ) ) ;
#91292=CARTESIAN_POINT ( 'NONE',  ( 14.66813190280496570, 26.65586893147755276, -7.433330006724137462 ) ) ;
#91294=CARTESIAN_POINT ( 'NONE',  ( 71.88182444303143370, 59.07920979518379312, 15.87605134362294734 ) ) ;
#91301=CARTESIAN_POINT ( 'NONE',  ( 88.02595808552065648, 44.67474554292944333, 4.297255302186842485 ) ) ;
#91302=CARTESIAN_POINT ( 'NONE',  ( 81.36830186270630350, 42.43310981303259410, 7.489272701115289088 ) ) ;
#91309=ORIENTED_EDGE ( 'NONE', *, *, #2788, .T. ) ;
#91315=CARTESIAN_POINT ( 'NONE',  ( 29.42770338693789967, 22.15404122711134960, 8.090169943749479842 ) ) ;
#91316=CARTESIAN_POINT ( 'NONE',  ( 80.74762043199122274, 57.32811249769932260, 16.57232535949601626 ) ) ;
#91317=CARTESIAN_POINT ( 'NONE',  ( 68.29143555172046831, 69.60586533063577974, -5.163910978133268159 ) ) ;
#91320=AXIS2_PLACEMENT_3D ( 'NONE', #51033, #97189, #91083 ) ;
#91325=EDGE_LOOP ( 'NONE', ( #72625, #21803, #47344, #8746 ) ) ;
#91336=CARTESIAN_POINT ( 'NONE',  ( 73.20149111268449360, 69.78470516290340697, 9.100743165113243549 ) ) ;
#91344=CARTESIAN_POINT ( 'NONE',  ( 76.92044504429365759, 57.04706196720093914, -16.17893565157367775 ) ) ;
#91345=CARTESIAN_POINT ( 'NONE',  ( 71.87575657461835021, 71.09473384654326367, 5.547135274974943187 ) ) ;
#91349=CARTESIAN_POINT ( 'NONE',  ( 78.54767433042584912, 47.93402356940807607, 13.94239611146432445 ) ) ;
#91352=CARTESIAN_POINT ( 'NONE',  ( 72.33612429178343461, 70.29735357913294536, 7.619994811607423202 ) ) ;
#91354=CARTESIAN_POINT ( 'NONE',  ( 79.22767783863193358, 46.14077938263190504, 12.65241577235085124 ) ) ;
#91360=CARTESIAN_POINT ( 'NONE',  ( 82.87158540007671093, 42.03325885046006505, 6.269962817432972457 ) ) ;
#91361=CARTESIAN_POINT ( 'NONE',  ( 72.60487375326179915, 71.50102857937403655, 5.576306808341180421 ) ) ;
#91367=CARTESIAN_POINT ( 'NONE',  ( 84.15726348823297087, 50.51978324134979204, 13.75935458598990557 ) ) ;
#91380=CARTESIAN_POINT ( 'NONE',  ( 75.75493378409400691, 65.86437009324525604, -14.07593894684414693 ) ) ;
#91386=VECTOR ( 'NONE', #98381, 1000.000000000000114 ) ;
#91390=CARTESIAN_POINT ( 'NONE',  ( 15.23341505093859816, 9.764269794150882475, 3.090169943749476733 ) ) ;
#91392=CARTESIAN_POINT ( 'NONE',  ( 71.62383979505139564, 59.52605231305792444, -15.70840275671411845 ) ) ;
#91397=CARTESIAN_POINT ( 'NONE',  ( 73.16773116491842188, 57.32667411120098677, 16.38412366264992315 ) ) ;
#91398=CARTESIAN_POINT ( 'NONE',  ( 69.75017563541113930, 66.23009299845347186, 11.34195834197200625 ) ) ;
#91399=CARTESIAN_POINT ( 'NONE',  ( 66.43953443436693362, 68.06212878376058484, -4.898982275787033380 ) ) ;
#91401=EDGE_CURVE ( 'NONE', #66291, #80464, #80712, .T. ) ;
#91405=CARTESIAN_POINT ( 'NONE',  ( 25.24326406500046360, 20.28920272979927475, -7.433330006724141015 ) ) ;
#91407=CARTESIAN_POINT ( 'NONE',  ( 83.83095627921952087, 51.88776739408810812, -14.90233955705620694 ) ) ;
#91409=CARTESIAN_POINT ( 'NONE',  ( 72.69493809724967548, 71.16443809380129437, -7.267007365939463170 ) ) ;
#91411=CARTESIAN_POINT ( 'NONE',  ( 74.66818547213321722, 67.01009517369644186, 12.98877810528426835 ) ) ;
#91412=EDGE_CURVE ( 'NONE', #38035, #90841, #35418, .T. ) ;
#91413=CARTESIAN_POINT ( 'NONE',  ( 69.13686587061594935, 64.31895405193962745, 11.99662287724233067 ) ) ;
#91415=CARTESIAN_POINT ( 'NONE',  ( 81.53593397896733563, 52.71546265156933941, 15.68299913778540500 ) ) ;
#91418=CARTESIAN_POINT ( 'NONE',  ( 67.53167658295855347, 67.09922345392760690, 8.942594108559751120 ) ) ;
#91419=ORIENTED_EDGE ( 'NONE', *, *, #1818, .F. ) ;
#91431=B_SPLINE_CURVE_WITH_KNOTS ( 'NONE', 3,
 ( #649, #15838, #48250, #32032, #16348, #85819, #39121, #85293, #24939, #54836, #78664, #40128, #55816, #47242, #78161, #48762, #8749, #56334, #1669, #39620, #86809, #17342, #79196, #9770 ),
 .UNSPECIFIED., .F., .F.,
 ( 4, 2, 2, 2, 2, 2, 2, 2, 2, 2, 2, 4 ),
 ( 0.000000000000000000, 0.1250000000000026090, 0.2500000000000052180, 0.3750000000000078271, 0.4375000000000070499, 0.5000000000000063283, 0.5625000000000056621, 0.6250000000000048850, 0.6875000000000042188, 0.7500000000000035527, 0.8750000000000017764, 1.000000000000000000 ),
 .UNSPECIFIED. ) ;
#91433=CARTESIAN_POINT ( 'NONE',  ( 15.90241741327948866, 17.38052372038639248, 10.00000000000000533 ) ) ;
#91441=CARTESIAN_POINT ( 'NONE',  ( 87.04122873496829982, 46.31593380912285340, -9.298662157179387933 ) ) ;
#91443=CARTESIAN_POINT ( 'NONE',  ( 74.98280371995244309, 53.54625940471802892, -16.54205200350763505 ) ) ;
#91444=CARTESIAN_POINT ( 'NONE',  ( 69.72103949949544699, 62.67904974704494236, 13.91083112788282072 ) ) ;
#91449=CARTESIAN_POINT ( 'NONE',  ( 81.80218481495317917, 42.34898084214702152, -7.958921281150827198 ) ) ;
#91452=VERTEX_POINT ( 'NONE', #3993 ) ;
#91453=CARTESIAN_POINT ( 'NONE',  ( 81.26485967175177905, 49.45078135016260745, 13.98408766788312896 ) ) ;
#91462=CARTESIAN_POINT ( 'NONE',  ( 82.49266829201729934, 54.25868459827957935, -15.95543171357395629 ) ) ;
#91465=CARTESIAN_POINT ( 'NONE',  ( 65.97950814763213145, 68.67089519182323443, -0.3204388555221999724 ) ) ;
#91466=CARTESIAN_POINT ( 'NONE',  ( 19.11131643181922968, 13.96004757982089473, -5.678558825948276656 ) ) ;
#91468=CARTESIAN_POINT ( 'NONE',  ( 80.68870194293324971, 57.51412305112833678, 16.58365939551019608 ) ) ;
#91480=CARTESIAN_POINT ( 'NONE',  ( 83.82827945288542537, 51.88092520783234818, 14.50189114860043205 ) ) ;
#91487=CARTESIAN_POINT ( 'NONE',  ( 72.13241438359672486, 72.32265461515862626, 1.126504182728680803 ) ) ;
#91488=CARTESIAN_POINT ( 'NONE',  ( 72.78673888116644264, 70.95540242780744222, 7.715912594624930065 ) ) ;
#91490=CARTESIAN_POINT ( 'NONE',  ( 24.92020183544706668, 36.16126292948897003, -6.180339887498951690 ) ) ;
#91502=EDGE_CURVE ( 'NONE', #69479, #88281, #99197, .T. ) ;
#91503=CARTESIAN_POINT ( 'NONE',  ( 83.42066707790206692, 44.47267527468968495, 8.844408096855449486 ) ) ;
#91509=LINE ( 'NONE', #52969, #9234 ) ;
#91511=CARTESIAN_POINT ( 'NONE',  ( 81.66084985466937951, 53.00684753587499642, -15.33431951212414646 ) ) ;
#91523=B_SPLINE_CURVE_WITH_KNOTS ( 'NONE', 3,
 ( #23880, #60872, #68486, #85235, #31478, #7184, #38071, #103, #77088, #53771, #14301, #39067, #45188, #46687, #6198, #69979, #68984, #593, #52780, #84733, #61383, #69489, #15273, #53291 ),
 .UNSPECIFIED., .F., .F.,
 ( 4, 2, 2, 2, 2, 2, 2, 2, 2, 2, 2, 4 ),
 ( 0.000000000000000000, 0.1249999999999943379, 0.2499999999999886757, 0.3749999999999830136, 0.4374999999999846789, 0.4999999999999863443, 0.5624999999999880096, 0.6249999999999897859, 0.6874999999999914513, 0.7499999999999932276, 0.8749999999999965583, 1.000000000000000000 ),
 .UNSPECIFIED. ) ;
#91525=CARTESIAN_POINT ( 'NONE',  ( 13.11890841201833169, 13.28920272979925166, -7.433330006724141015 ) ) ;
#91530=CARTESIAN_POINT ( 'NONE',  ( 85.07585738814579202, 42.60566994075947633, -2.415354379879502300 ) ) ;
#91534=CARTESIAN_POINT ( 'NONE',  ( 34.28181963472369631, 41.83396525600392835, -2.839279412974133887 ) ) ;
#91538=CARTESIAN_POINT ( 'NONE',  ( 24.17276070933917609, 32.14336893147756768, 7.433330006724141015 ) ) ;
#91543=CARTESIAN_POINT ( 'NONE',  ( 70.69455434939749239, 60.85083930861275547, 14.53159835427401880 ) ) ;
#91547=CARTESIAN_POINT ( 'NONE',  ( 75.16643821786686885, 52.89298839225886439, -15.99447471506349672 ) ) ;
#91550=CARTESIAN_POINT ( 'NONE',  ( 73.61926920126447271, 69.75873974038962899, 10.00767910897496193 ) ) ;
#91553=CARTESIAN_POINT ( 'NONE',  ( 88.00349997577261263, 44.64923112938743088, 4.253506518527973235 ) ) ;
#91555=DIRECTION ( 'NONE',  ( -0.3037402332698226903, -0.8935232438716340653, 0.3306933373297776257 ) ) ;
#91561=CARTESIAN_POINT ( 'NONE',  ( 40.09738740370236343, 25.01110640527295104, 2.839279412974134775 ) ) ;
#91563=CARTESIAN_POINT ( 'NONE',  ( 77.77867966053455007, 61.43039905302717330, -16.12786080876372807 ) ) ;
#91564=CARTESIAN_POINT ( 'NONE',  ( 87.39465943033326312, 45.50146518389362171, 7.088208788914807101 ) ) ;
#91571=DIRECTION ( 'NONE',  ( 0.8660254037844378194, 0.5000000000000015543, 0.000000000000000000 ) ) ;
#91574=CARTESIAN_POINT ( 'NONE',  ( 72.92438617816932833, 61.44597022494355798, -14.84684155615548740 ) ) ;
#91575=CARTESIAN_POINT ( 'NONE',  ( 82.09534214412946085, 40.77824446403596426, 1.263644830401252861 ) ) ;
#91577=CARTESIAN_POINT ( 'NONE',  ( 76.99381129068922291, 63.91386138922637628, -15.28064156999390732 ) ) ;
#91580=ORIENTED_EDGE ( 'NONE', *, *, #60172, .T. ) ;
#91582=CARTESIAN_POINT ( 'NONE',  ( 43.01361757626971638, 27.76004757982093452, 5.678558825948272215 ) ) ;
#91584=EDGE_LOOP ( 'NONE', ( #7963, #34040, #18061, #693 ) ) ;
#91588=CARTESIAN_POINT ( 'NONE',  ( 86.86990765421666083, 45.77415147683691288, -8.704208088459520098 ) ) ;
#91598=VERTEX_POINT ( 'NONE', #55063 ) ;
#91603=CARTESIAN_POINT ( 'NONE',  ( 82.43642368079662219, 44.97063798659471701, 10.10360692900326995 ) ) ;
#91615=CARTESIAN_POINT ( 'NONE',  ( 84.67330385480828170, 45.84957715147402268, 9.683287886809928580 ) ) ;
#91617=CARTESIAN_POINT ( 'NONE',  ( 20.05933935144479108, 19.78052372038640527, -10.00000000000000355 ) ) ;
#91619=B_SPLINE_CURVE_WITH_KNOTS ( 'NONE', 3,
 ( #79822, #95024, #55947, #96518, #18492, #73194, #65076, #56473, #79329, #9897, #33694, #48385, #2806, #2298, #57971, #27087 ),
 .UNSPECIFIED., .F., .F.,
 ( 4, 1, 2, 2, 2, 1, 2, 2, 4 ),
 ( 0.000000000000000000, 0.1250000000000056066, 0.1875000000000069111, 0.2500000000000082157, 0.5000000000000036637, 0.6250000000000013323, 0.6875000000000004441, 0.7499999999999994449, 1.000000000000000000 ),
 .UNSPECIFIED. ) ;
#91620=CARTESIAN_POINT ( 'NONE',  ( 82.59012279121988342, 53.49374897786832150, -15.73261944071848539 ) ) ;
#91621=EDGE_CURVE ( 'NONE', #69104, #43232, #20717, .T. ) ;
#91632=CARTESIAN_POINT ( 'NONE',  ( 73.34072767760012823, 69.17406821459752564, -9.926094365178592227 ) ) ;
#91637=CARTESIAN_POINT ( 'NONE',  ( 82.07790669499631520, 54.04471111898705260, 15.60661167468746591 ) ) ;
#91638=VECTOR ( 'NONE', #55515, 1000.000000000000114 ) ;
#91639=CARTESIAN_POINT ( 'NONE',  ( 71.98582063699875278, 72.29727681381652360, 3.337216071139561979 ) ) ;
#91643=CARTESIAN_POINT ( 'NONE',  ( 77.66081197416168891, 51.27534508892328802, -15.41764112584265334 ) ) ;
#91646=B_SPLINE_CURVE_WITH_KNOTS ( 'NONE', 3,
 ( #85979, #83963, #61600, #39285, #77319, #91550, #75844, #55000, #93036, #62090, #14527, #313, #46908, #31201, #23592, #30215, #6431, #76810, #62591, #77830, #31685, #8413, #93547, #84459, #53011, #7925, #37308, #29719, #14999, #37799, #68208 ),
 .UNSPECIFIED., .F., .F.,
 ( 4, 3, 3, 3, 3, 3, 3, 3, 3, 3, 4 ),
 ( 0.000000000000000000, 0.1333490885032317663, 0.3007194338854262683, 0.4699862290245025997, 0.5844252810809391629, 0.6686540514502795629, 0.7354980260655534785, 0.8028463152565619154, 0.8633854507757232621, 0.9437142632667340214, 1.000000000000000000 ),
 .UNSPECIFIED. ) ;
#91647=CARTESIAN_POINT ( 'NONE',  ( 21.31005897544419625, 27.70171378149919050, -9.188101187500004485 ) ) ;
#91650=CARTESIAN_POINT ( 'NONE',  ( 44.67827877960949223, 26.76426979415094110, 3.090169943749476733 ) ) ;
#91652=CARTESIAN_POINT ( 'NONE',  ( 76.62811072403027879, 63.82025679357946046, 14.86655239196480771 ) ) ;
#91653=CARTESIAN_POINT ( 'NONE',  ( 76.34415836482729389, 61.31935459807998967, 15.96335647903723221 ) ) ;
#91654=VECTOR ( 'NONE', #55566, 999.9999999999998863 ) ;
#91656=CARTESIAN_POINT ( 'NONE',  ( 82.11871479691291142, 40.77613790009904449, -1.068313329471679562 ) ) ;
#91660=CARTESIAN_POINT ( 'NONE',  ( 87.68255615283939619, 45.40041221884136746, -6.563636875042941021 ) ) ;
#91666=ORIENTED_EDGE ( 'NONE', *, *, #26037, .T. ) ;
#91672=CARTESIAN_POINT ( 'NONE',  ( 72.10617024684209753, 72.18421392457030095, 4.031754617348218162 ) ) ;
#91673=LINE ( 'NONE', #23227, #79834 ) ;
#91675=CARTESIAN_POINT ( 'NONE',  ( 85.75842679711398375, 42.78537197811905202, 3.771247107581231717 ) ) ;
#91680=CARTESIAN_POINT ( 'NONE',  ( 20.33338779993010803, 20.24335787977762990, -9.188101187500008038 ) ) ;
#91688=CARTESIAN_POINT ( 'NONE',  ( 80.08925426792347935, 49.88496243973265365, -14.48658023246625604 ) ) ;
#91690=PLANE ( 'NONE',  #62108 ) ;
#91692=CARTESIAN_POINT ( 'NONE',  ( 1.830000459568766003, 24.55466486950697202, 1.000260061240931054E-15 ) ) ;
#91702=CARTESIAN_POINT ( 'NONE',  ( 72.93270222632347100, 70.75261854202813083, -7.421515863126944446 ) ) ;
#91705=ORIENTED_EDGE ( 'NONE', *, *, #58039, .T. ) ;
#91710=CARTESIAN_POINT ( 'NONE',  ( 66.51083587138683129, 67.82564551438169076, 6.839597181675368454 ) ) ;
#91712=B_SPLINE_CURVE_WITH_KNOTS ( 'NONE', 3,
 ( #43637, #74577, #50738, #81693, #27473, #19871, #58341, #36036, #44130, #75064, #42635, #11285, #49758, #43125, #26470, #28437, #73077, #82202, #80709, #3675, #5157, #26961, #66936, #34553 ),
 .UNSPECIFIED., .F., .F.,
 ( 4, 2, 2, 2, 2, 2, 2, 2, 2, 2, 2, 4 ),
 ( 0.000000000000000000, 0.1249999999999972522, 0.2499999999999945044, 0.3749999999999917843, 0.4374999999999891753, 0.4999999999999865663, 0.5624999999999840128, 0.6249999999999813483, 0.6874999999999787947, 0.7499999999999762412, 0.8749999999999881206, 1.000000000000000000 ),
 .UNSPECIFIED. ) ;
#91715=CARTESIAN_POINT ( 'NONE',  ( 81.01777758920067640, 56.07228383068083843, 16.10439022756407468 ) ) ;
#91716=CARTESIAN_POINT ( 'NONE',  ( 73.62250635243424313, 69.55784274833359859, 10.23584637956792776 ) ) ;
#91718=CARTESIAN_POINT ( 'NONE',  ( 70.29920436004088913, 63.58999502166589934, 12.99331325176316376 ) ) ;
#91722=CARTESIAN_POINT ( 'NONE',  ( 76.13978442645490929, 51.56145741272602834, -16.17442695369989281 ) ) ;
#91729=VERTEX_POINT ( 'NONE', #77390 ) ;
#91731=CARTESIAN_POINT ( 'NONE',  ( 87.88540012852695327, 44.32205958948441094, 4.765779035299133604 ) ) ;
#91732=CARTESIAN_POINT ( 'NONE',  ( 86.48644980920353476, 45.02549005842475083, 7.069432882560119147 ) ) ;
#91734=CARTESIAN_POINT ( 'NONE',  ( 79.89247370868126552, 44.63210057524135266, -11.16478091168645470 ) ) ;
#91736=CARTESIAN_POINT ( 'NONE',  ( 72.85564822012069897, 70.83604795162270307, 7.235281746655774171 ) ) ;
#91752=CARTESIAN_POINT ( 'NONE',  ( 29.85841906089621389, 18.20801979619929867, -3.090169943749474069 ) ) ;
#91755=CARTESIAN_POINT ( 'NONE',  ( 67.75058886435806471, 69.10744749125690589, -5.632754406238772660 ) ) ;
#91760=CARTESIAN_POINT ( 'NONE',  ( 66.46435720904777611, 67.83184248247579262, -6.775977428004711811 ) ) ;
#91761=CARTESIAN_POINT ( 'NONE',  ( 72.77745277708218907, 70.81288354178653321, -7.938184674006797614 ) ) ;
#91764=VECTOR ( 'NONE', #67549, 1000.000000000000114 ) ;
#91767=CARTESIAN_POINT ( 'NONE',  ( 22.59275855922847498, 34.81751292744058190, -6.180339887498951690 ) ) ;
#91768=CARTESIAN_POINT ( 'NONE',  ( 85.06235871598175891, 48.90491807502699828, 12.39955041771802691 ) ) ;
#91771=VECTOR ( 'NONE', #45657, 1000.000000000000114 ) ;
#91781=CARTESIAN_POINT ( 'NONE',  ( 72.60008616680404714, 70.69752196365911345, -7.958780822297746305 ) ) ;
#91782=CARTESIAN_POINT ( 'NONE',  ( 72.58458169156800466, 71.41452113280901415, 5.739636480442070088 ) ) ;
#91783=CARTESIAN_POINT ( 'NONE',  ( 38.30461122658549300, 34.06628583063844928, -9.188101187500006262 ) ) ;
#91787=CARTESIAN_POINT ( 'NONE',  ( 79.14312167556931854, 57.64441083166269664, 0.000000000000000000 ) ) ;
#91790=CARTESIAN_POINT ( 'NONE',  ( 24.50893013558248157, 16.01110640527292261, 2.839279412974134775 ) ) ;
#91792=CARTESIAN_POINT ( 'NONE',  ( 72.02510489751692546, 59.23144522310215621, 15.35746550185032255 ) ) ;
#91798=CARTESIAN_POINT ( 'NONE',  ( 81.10000394050406669, 45.98558232817099878, -12.37583392106304458 ) ) ;
#91799=CARTESIAN_POINT ( 'NONE',  ( 75.36487073175837281, 53.53173320265494795, -16.04382577248123809 ) ) ;
#91800=CARTESIAN_POINT ( 'NONE',  ( 81.71275118201126020, 42.05154519778324129, 7.556033175796731172 ) ) ;
#91801=PLANE ( 'NONE',  #86690 ) ;
#91804=DIRECTION ( 'NONE',  ( 0.2347357813929421555, -0.4065742997269585213, 0.8829475928589297640 ) ) ;
#91805=CARTESIAN_POINT ( 'NONE',  ( 72.39195994751899832, 71.88450172447629427, -5.391213119607743742 ) ) ;
#91806=CARTESIAN_POINT ( 'NONE',  ( 77.20977722794761178, 63.51083823537270945, 15.08832032918205357 ) ) ;
#91808=ORIENTED_EDGE ( 'NONE', *, *, #96460, .F. ) ;
#91812=CARTESIAN_POINT ( 'NONE',  ( 87.85430303351097336, 43.89859490532884223, 0.3596698246726173775 ) ) ;
#91813=B_SPLINE_CURVE_WITH_KNOTS ( 'NONE', 3,
 ( #34315, #20125, #26718, #34799, #73329, #88580, #4929, #19142, #65701, #96655, #27225, #58108, #50499, #50016, #57098, #81453 ),
 .UNSPECIFIED., .F., .F.,
 ( 4, 1, 2, 2, 2, 1, 2, 2, 4 ),
 ( 0.000000000000000000, 0.1250000000000047462, 0.1875000000000061062, 0.2500000000000074940, 0.5000000000000091038, 0.6250000000000103251, 0.6875000000000094369, 0.7500000000000085487, 1.000000000000000000 ),
 .UNSPECIFIED. ) ;
#91816=CARTESIAN_POINT ( 'NONE',  ( 26.31557204471864253, 27.14441083166262203, 10.00000000000000533 ) ) ;
#91817=CARTESIAN_POINT ( 'NONE',  ( 80.07172880487748046, 57.71088839156738715, 16.60216399474093762 ) ) ;
#91820=EDGE_CURVE ( 'NONE', #8542, #54050, #63044, .T. ) ;
#91828=CARTESIAN_POINT ( 'NONE',  ( 78.37926235792471630, 47.32821374589490659, -14.23582365648701575 ) ) ;
#91829=ORIENTED_EDGE ( 'NONE', *, *, #35429, .F. ) ;
#91832=CARTESIAN_POINT ( 'NONE',  ( 42.14088959202413776, 24.73415679381825427, -6.890680421881970419E-14 ) ) ;
#91838=CARTESIAN_POINT ( 'NONE',  ( 88.22316733864592209, 44.26875609612613971, 2.029272769359137474 ) ) ;
#91840=CARTESIAN_POINT ( 'NONE',  ( 82.35193903712398367, 53.76144841737798430, 15.84691369965402963 ) ) ;
#91847=B_SPLINE_CURVE_WITH_KNOTS ( 'NONE', 3,
 ( #19833, #29415, #97837, #6108, #28926, #90769, #58793, #52197, #67914, #50705, #83146, #37004, #98834, #51203, #12743, #43607, #28406, #59286, #14211, #29904, #7100, #6616, #85664, #47095 ),
 .UNSPECIFIED., .F., .F.,
 ( 4, 2, 2, 2, 2, 2, 2, 2, 2, 2, 2, 4 ),
 ( 0.000000000000000000, 0.1250000000000033029, 0.2500000000000066058, 0.3750000000000098810, 0.4375000000000053291, 0.5000000000000007772, 0.5624999999999962252, 0.6249999999999916733, 0.6874999999999871214, 0.7499999999999824585, 0.8749999999999912292, 1.000000000000000000 ),
 .UNSPECIFIED. ) ;
#91849=CARTESIAN_POINT ( 'NONE',  ( 69.91676562038409770, 67.50422961795942456, 9.414007674835353612 ) ) ;
#91854=CARTESIAN_POINT ( 'NONE',  ( 78.13762852215380406, 47.61987223718105611, 14.45360562616755828 ) ) ;
#91856=ORIENTED_EDGE ( 'NONE', *, *, #72937, .T. ) ;
#91859=CARTESIAN_POINT ( 'NONE',  ( 74.94274948198699349, 54.56384823593326416, -16.13558687890323995 ) ) ;
#91862=CARTESIAN_POINT ( 'NONE',  ( 79.56664545794562571, 45.84018632621341283, 12.91967758877038897 ) ) ;
#91871=CARTESIAN_POINT ( 'NONE',  ( 72.56680254073343406, 71.38637538794350235, 5.777867564336604644 ) ) ;
#91875=EDGE_CURVE ( 'NONE', #85355, #52772, #25555, .T. ) ;
#91877=DIRECTION ( 'NONE',  ( 0.5000000000000013323, -0.8660254037844378194, 0.000000000000000000 ) ) ;
#91882=ORIENTED_EDGE ( 'NONE', *, *, #35886, .F. ) ;
#91885=FACE_OUTER_BOUND ( 'NONE', #70147, .T. ) ;
#91889=CARTESIAN_POINT ( 'NONE',  ( 81.86592541406376711, 41.15561125584435587, -5.581452205721086024 ) ) ;
#91891=CARTESIAN_POINT ( 'NONE',  ( 68.55042658866229033, 64.21781301378140938, -12.45171015595362540 ) ) ;
#91897=CARTESIAN_POINT ( 'NONE',  ( 78.60735446187601383, 47.91558663937575346, -14.46554739992949834 ) ) ;
#91899=CARTESIAN_POINT ( 'NONE',  ( 6.588875291771465470, 26.73705186507752174, -3.090169943749475845 ) ) ;
#91901=CARTESIAN_POINT ( 'NONE',  ( 71.49043722402748813, 59.12641653362435079, -15.80154365645430836 ) ) ;
#91902=FACE_OUTER_BOUND ( 'NONE', #41036, .T. ) ;
#91906=CARTESIAN_POINT ( 'NONE',  ( 73.58947491971605359, 55.55901669400043374, 16.10573162174744155 ) ) ;
#91908=CARTESIAN_POINT ( 'NONE',  ( 66.31978875953279839, 68.10230444367267921, -4.579799779162929241 ) ) ;
#91909=B_SPLINE_CURVE_WITH_KNOTS ( 'NONE', 3,
 ( #66743, #73862, #66258, #81496, #27760, #12065, #59119, #98172, #28750, #65741 ),
 .UNSPECIFIED., .F., .F.,
 ( 4, 2, 2, 2, 4 ),
 ( 0.000000000000000000, 0.2500000000000000000, 0.5000000000000000000, 0.7500000000000000000, 1.000000000000000000 ),
 .UNSPECIFIED. ) ;
#91915=CARTESIAN_POINT ( 'NONE',  ( 28.07469292777547309, 37.18502408145594273, 5.678558825948277544 ) ) ;
#91917=CARTESIAN_POINT ( 'NONE',  ( 66.43953443436691941, 68.06212878376058484, -4.898982275787033380 ) ) ;
#91922=ORIENTED_EDGE ( 'NONE', *, *, #15013, .T. ) ;
#91924=DIRECTION ( 'NONE',  ( 0.000000000000000000, 0.000000000000000000, 1.000000000000000000 ) ) ;
#91929=ORIENTED_EDGE ( 'NONE', *, *, #57812, .F. ) ;
#91944=CARTESIAN_POINT ( 'NONE',  ( 18.14948940725119897, 10.28848085856230377, 1.475505719884397138E-15 ) ) ;
#91945=CARTESIAN_POINT ( 'NONE',  ( 86.46048006423903587, 47.32182001325401899, 10.26516935212321258 ) ) ;
#91948=CARTESIAN_POINT ( 'NONE',  ( 86.46734690923850053, 47.05374834302038067, -10.53985889464876458 ) ) ;
#91949=CARTESIAN_POINT ( 'NONE',  ( 80.52777769245514605, 45.62452705624884430, -11.72524612028085222 ) ) ;
#91956=CARTESIAN_POINT ( 'NONE',  ( 74.92809311542137607, 53.46823265460128738, -16.53855748461180752 ) ) ;
#91957=CARTESIAN_POINT ( 'NONE',  ( 69.40575591891894192, 62.79509274011370223, 13.16381358185486405 ) ) ;
#91961=CARTESIAN_POINT ( 'NONE',  ( 73.32155222933093341, 69.66094733087366819, -9.921889652296787432 ) ) ;
#91962=CARTESIAN_POINT ( 'NONE',  ( 81.80835978698212330, 42.34965515190965846, -7.954336405571433843 ) ) ;
#91963=B_SPLINE_SURFACE_WITH_KNOTS ( 'NONE', 3, 1, ( 
 ( #72582, #73559 ),
 ( #65943, #57341 ),
 ( #58336, #10764 ),
 ( #5151, #42140 ),
 ( #34548, #73072 ),
 ( #95415, #49752 ),
 ( #41639, #66446 ),
 ( #89312, #20360 ),
 ( #58822, #34071 ),
 ( #80704, #25971 ),
 ( #89784, #95907 ),
 ( #50733, #81688 ),
 ( #3670, #65446 ),
 ( #57839, #88819 ),
 ( #13737, #66932 ),
 ( #28433, #39385 ),
 ( #44617, #29440 ),
 ( #16604, #53234 ),
 ( #21837, #83682 ),
 ( #93649, #60810 ),
 ( #21346, #14243 ),
 ( #8516, #90794 ),
 ( #24214, #75552 ),
 ( #9009, #55095 ),
 ( #47503, #20864 ),
 ( #75060, #52722 ),
 ( #37522, #67942 ),
 ( #83175, #59315 ),
 ( #86082, #60314 ),
 ( #84186, #29933 ),
 ( #62693, #45129 ) ),
 .UNSPECIFIED., .F., .F., .F.,
 ( 4, 3, 3, 3, 3, 3, 3, 3, 3, 3, 4 ),
 ( 2, 2 ),
 ( 0.000000000000000000, 0.1333490885032340423, 0.3007194338854312643, 0.4699862290245129803, 0.5844252810809342780, 0.6686540514502644639, 0.7354980260655447077, 0.8028463152565625816, 0.8633854507757121599, 0.9437142632667110398, 1.000000000000000000 ),
 ( 0.000000000000000000, 1.000000000000000000 ),
 .UNSPECIFIED. ) ;
#91965=EDGE_CURVE ( 'NONE', #49112, #19562, #70205, .T. ) ;
#91968=EDGE_LOOP ( 'NONE', ( #30755, #85386, #92827, #69363 ) ) ;
#91969=CARTESIAN_POINT ( 'NONE',  ( 81.27747349237425567, 49.50046732535272298, 14.00627724909530691 ) ) ;
#91971=CARTESIAN_POINT ( 'NONE',  ( 68.17307502523176765, 68.36170032566508326, 6.558107242125284841 ) ) ;
#91974=AXIS2_PLACEMENT_3D ( 'NONE', #36635, #97482, #13848 ) ;
#91978=CARTESIAN_POINT ( 'NONE',  ( 70.30291785998953458, 68.43742151735528978, -8.517849549379890917 ) ) ;
#91980=CARTESIAN_POINT ( 'NONE',  ( 80.07214027775873433, 55.25082771389860170, -16.41292865798596878 ) ) ;
#91981=CARTESIAN_POINT ( 'NONE',  ( 21.59269996301512862, 13.26216523072493914, -2.296566073217252530E-15 ) ) ;
#91984=CARTESIAN_POINT ( 'NONE',  ( 74.14312167556930433, 66.30466486950707861, 1.224646799147354045E-15 ) ) ;
#91990=CARTESIAN_POINT ( 'NONE',  ( 81.43726257051942241, 46.06824199903791595, -11.66015455581693061 ) ) ;
#91996=CARTESIAN_POINT ( 'NONE',  ( 74.79855439552166274, 62.33245921625753994, -14.96095770982128847 ) ) ;
#92000=CARTESIAN_POINT ( 'NONE',  ( 82.83316871194540454, 53.40219886645672176, -15.30257817068320847 ) ) ;
#92002=EDGE_CURVE ( 'NONE', #56559, #2820, #28054, .T. ) ;
#92005=CARTESIAN_POINT ( 'NONE',  ( 72.08719088798999053, 72.32551850972336638, 0.8194835739893685522 ) ) ;
#92009=FACE_OUTER_BOUND ( 'NONE', #27504, .T. ) ;
#92014=VERTEX_POINT ( 'NONE', #88521 ) ;
#92028=CARTESIAN_POINT ( 'NONE',  ( 78.82139251731592822, 54.02149238465010939, -15.89892391852131048 ) ) ;
#92035=CARTESIAN_POINT ( 'NONE',  ( 70.32692526124142773, 70.56678268892162009, 4.342815048252711918 ) ) ;
#92036=CARTESIAN_POINT ( 'NONE',  ( 70.54960841692590634, 71.60126540147106766, 2.719701375183281034 ) ) ;
#92038=EDGE_LOOP ( 'NONE', ( #73716, #72175, #44556, #58889 ) ) ;
#92044=CARTESIAN_POINT ( 'NONE',  ( 3.278110179240818045, 23.93396525600387648, 2.839279412974139660 ) ) ;
#92047=FACE_OUTER_BOUND ( 'NONE', #77502, .T. ) ;
#92052=AXIS2_PLACEMENT_3D ( 'NONE', #9762, #46342, #15443 ) ;
#92053=CARTESIAN_POINT ( 'NONE',  ( 36.29711636232130445, 39.14336893147758900, 7.433330006724141015 ) ) ;
#92054=CARTESIAN_POINT ( 'NONE',  ( 33.00691499580853616, 42.55466486950702887, 7.012934429366973338E-14 ) ) ;
#92057=CARTESIAN_POINT ( 'NONE',  ( 34.04181514241641082, 20.44966523072496756, -2.296566073217252530E-15 ) ) ;
#92058=CARTESIAN_POINT ( 'NONE',  ( 74.41527144631503177, 63.48680199517529843, -14.86167820946030815 ) ) ;
#92062=CARTESIAN_POINT ( 'NONE',  ( 84.55094438110296551, 49.89265462440669552, -13.67900519688966021 ) ) ;
#92063=CARTESIAN_POINT ( 'NONE',  ( 76.01570425163725986, 65.59347775405139203, -14.29814048726880316 ) ) ;
#92066=CARTESIAN_POINT ( 'NONE',  ( 75.07854663334262568, 53.00102994419008695, -16.48764564530848631 ) ) ;
#92071=CARTESIAN_POINT ( 'NONE',  ( 37.04286019156342746, 27.10170272979929607, -7.433330006724141015 ) ) ;
#92078=CARTESIAN_POINT ( 'NONE',  ( 86.50941216119214516, 47.42513861390694530, -10.35655363221832737 ) ) ;
#92085=CARTESIAN_POINT ( 'NONE',  ( 31.21403501649406209, 38.99752408145594273, 5.678558825948276656 ) ) ;
#92086=CYLINDRICAL_SURFACE ( 'NONE', #94772, 10.00000000000001066 ) ;
#92094=VERTEX_POINT ( 'NONE', #21552 ) ;
#92095=CARTESIAN_POINT ( 'NONE',  ( 72.12409258116959165, 72.31950243486284080, -1.088631527110781594 ) ) ;
#92105=CARTESIAN_POINT ( 'NONE',  ( 77.19405137238244663, 62.95358206284149105, -15.28408875821778423 ) ) ;
#92118=ORIENTED_EDGE ( 'NONE', *, *, #67667, .T. ) ;
#92128=CARTESIAN_POINT ( 'NONE',  ( 81.69252017841917279, 43.53081715963432430, 8.862045408265887048 ) ) ;
#92130=CARTESIAN_POINT ( 'NONE',  ( 69.66079769549185130, 63.13740578632653921, -13.62281212579674161 ) ) ;
#92134=CARTESIAN_POINT ( 'NONE',  ( 72.02948279518248853, 64.51453867759187233, 13.07310271355176390 ) ) ;
#92135=CARTESIAN_POINT ( 'NONE',  ( 82.62760750629610129, 40.94168765461595427, -3.622589341579083300 ) ) ;
#92139=CARTESIAN_POINT ( 'NONE',  ( 82.63082945135448654, 42.48621489691582553, 6.270187774756061039 ) ) ;
#92143=CARTESIAN_POINT ( 'NONE',  ( 82.51639823017981712, 53.47659673923356394, -15.74004163755323304 ) ) ;
#92156=CARTESIAN_POINT ( 'NONE',  ( 42.57599984984017993, 32.78052372038644791, -10.00000000000000355 ) ) ;
#92159=CARTESIAN_POINT ( 'NONE',  ( 71.83668398922712583, 71.91439960379638308, 2.874141227818668654 ) ) ;
#92162=EDGE_CURVE ( 'NONE', #95962, #99249, #99308, .T. ) ;
#92166=CARTESIAN_POINT ( 'NONE',  ( 82.36450559414066674, 49.91219489361158423, -13.90160499203291522 ) ) ;
#92170=CARTESIAN_POINT ( 'NONE',  ( 22.39019813391814751, 21.43085787977763701, -9.188101187500008038 ) ) ;
#92173=CARTESIAN_POINT ( 'NONE',  ( 14.98925625915878079, 9.449665230724930254, -2.296566073217252530E-15 ) ) ;
#92174=CARTESIAN_POINT ( 'NONE',  ( 24.67121952831112353, 36.01751292744057764, 6.180339887498949913 ) ) ;
#92175=CARTESIAN_POINT ( 'NONE',  ( 77.03033377257250436, 63.66679109869721742, 15.37730549896620147 ) ) ;
#92185=CARTESIAN_POINT ( 'NONE',  ( 77.23115344012272487, 49.25751081205777382, 15.36283045010027948 ) ) ;
#92186=ORIENTED_EDGE ( 'NONE', *, *, #11475, .T. ) ;
#92192=CARTESIAN_POINT ( 'NONE',  ( 79.08118623426810245, 45.97885358038440273, -12.60247831142608987 ) ) ;
#92194=CARTESIAN_POINT ( 'NONE',  ( 73.09164847706512091, 70.51859621836145209, -7.974784385355167871 ) ) ;
#92195=PLANE ( 'NONE',  #38530 ) ;
#92197=CARTESIAN_POINT ( 'NONE',  ( 15.62557774837418023, 29.99752408145591431, 5.678558825948276656 ) ) ;
#92202=EDGE_CURVE ( 'NONE', #25358, #184, #69128, .T. ) ;
#92204=ADVANCED_FACE ( 'NONE', ( #68135 ), #67640, .T. ) ;
#92205=ORIENTED_EDGE ( 'NONE', *, *, #36678, .T. ) ;
#92208=CARTESIAN_POINT ( 'NONE',  ( 68.06446806950627604, 66.09146943954503683, -10.51449895684611491 ) ) ;
#92211=EDGE_CURVE ( 'NONE', #52319, #86732, #69138, .T. ) ;
#92220=EDGE_LOOP ( 'NONE', ( #39494, #22999, #31707, #69392, #30537 ) ) ;
#92223=CARTESIAN_POINT ( 'NONE',  ( 79.46553399343461876, 45.78194281441977864, 12.91977081584364662 ) ) ;
#92229=CARTESIAN_POINT ( 'NONE',  ( 66.96658208328462081, 68.04499853430465350, 6.922779954623445420 ) ) ;
#92231=CARTESIAN_POINT ( 'NONE',  ( 90.04477061917849312, 44.76220097505219542, 0.000000000000000000 ) ) ;
#92232=CARTESIAN_POINT ( 'NONE',  ( 81.17013726474981183, 56.17602725108039152, 16.10664853823880804 ) ) ;
#92234=CARTESIAN_POINT ( 'NONE',  ( 71.55041901307521357, 67.02176819343763725, 10.94176416068171953 ) ) ;
#92238=B_SPLINE_SURFACE_WITH_KNOTS ( 'NONE', 3, 1, ( 
 ( #63749, #86114 ),
 ( #40428, #54623 ),
 ( #71362, #25240 ),
 ( #1953, #56125 ),
 ( #87121, #71868 ),
 ( #33346, #64245 ),
 ( #95195, #25767 ),
 ( #56642, #87625 ),
 ( #18154, #49053 ),
 ( #79989, #10557 ),
 ( #78341, #69718 ),
 ( #8923, #54498 ),
 ( #8426, #62102 ),
 ( #93049, #78847 ),
 ( #70212, #63622 ),
 ( #17521, #94559 ),
 ( #48428, #79376 ),
 ( #48933, #79872 ),
 ( #10432, #64635 ),
 ( #72249, #4840 ),
 ( #80883, #95587 ),
 ( #34717, #49925 ),
 ( #10943, #66121 ),
 ( #65616, #41306 ),
 ( #80372, #35220 ),
 ( #11452, #42308 ),
 ( #4317, #35720 ),
 ( #58506, #97070 ),
 ( #73239, #3832 ),
 ( #96573, #57513 ),
 ( #66618, #97548 ) ),
 .UNSPECIFIED., .F., .F., .F.,
 ( 4, 3, 3, 3, 3, 3, 3, 3, 3, 3, 4 ),
 ( 2, 2 ),
 ( 0.000000000000000000, 0.1333490885032359574, 0.3007194338854340954, 0.4699862290245186980, 0.5844252810809413834, 0.6686540514502794519, 0.7354980260655689106, 0.8028463152565833427, 0.8633854507757432462, 0.9437142632667659958, 1.000000000000000000 ),
 ( 0.000000000000000000, 1.000000000000000000 ),
 .UNSPECIFIED. ) ;
#92242=CARTESIAN_POINT ( 'NONE',  ( 76.20470709868462222, 65.28062994224386273, -14.10576654135921437 ) ) ;
#92248=CARTESIAN_POINT ( 'NONE',  ( 87.82600437409995209, 44.28008912978396694, 4.743525404917310340 ) ) ;
#92252=( BOUNDED_CURVE ( )  B_SPLINE_CURVE ( 2, ( #92054, #53488, #70181, #84440, #15477, #69690, #15995, #77818, #47388, #22600, #38279, #93535, #8893 ),
 .UNSPECIFIED., .F., .T. ) 
 B_SPLINE_CURVE_WITH_KNOTS ( ( 3, 2, 2, 2, 2, 2, 3 ),
 ( 0.9125000000000000888, 0.9150000000000000355, 0.9200000000000000400, 0.9250000000000000444, 0.9300000000000000488, 0.9350000000000000533, 0.9375000000000000000 ),
 .UNSPECIFIED. ) 
 CURVE ( )  GEOMETRIC_REPRESENTATION_ITEM ( )  RATIONAL_B_SPLINE_CURVE ( ( 0.9755282581475767101, 0.9755282581475772652, 1.000000000000000000, 0.9510565162951535312, 1.000000000000000000, 0.9510565162951535312, 1.000000000000000000, 0.9510565162951535312, 1.000000000000000000, 0.9510565162951535312, 1.000000000000000000, 0.9755282581475768211, 0.9755282581475768211 ) ) 
 REPRESENTATION_ITEM ( '' )  );
#92253=CARTESIAN_POINT ( 'NONE',  ( 73.06677152903225192, 70.63173304288399379, 7.751455205043641605 ) ) ;
#92254=CARTESIAN_POINT ( 'NONE',  ( 69.73018707955242235, 67.40416580934164870, -9.399663619568531914 ) ) ;
#92259=CARTESIAN_POINT ( 'NONE',  ( 80.80154134310006953, 50.59177401893971648, 14.61214521119545751 ) ) ;
#92260=FACE_OUTER_BOUND ( 'NONE', #59114, .T. ) ;
#92264=EDGE_CURVE ( 'NONE', #19562, #72450, #8339, .T. ) ;
#92267=CARTESIAN_POINT ( 'NONE',  ( 73.87609383058843093, 55.21511341151430230, 16.12190632378065303 ) ) ;
#92268=CARTESIAN_POINT ( 'NONE',  ( 24.58352123714976045, 26.14441083166261848, 10.00000000000000533 ) ) ;
#92276=VECTOR ( 'NONE', #50683, 1000.000000000000000 ) ;
#92278=CARTESIAN_POINT ( 'NONE',  ( 72.49337063691618255, 70.67504402769610294, -7.896386945446492334 ) ) ;
#92279=CARTESIAN_POINT ( 'NONE',  ( 81.60564328118654487, 41.73995806223437199, 5.932757990861635022 ) ) ;
#92281=CARTESIAN_POINT ( 'NONE',  ( 23.90938336746022586, 36.73705186507755371, -3.090169943749475845 ) ) ;
#92282=CARTESIAN_POINT ( 'NONE',  ( 85.20962068992432137, 42.51169701653922317, -1.264518624749869868 ) ) ;
#92285=DIRECTION ( 'NONE',  ( -0.4999999999999974465, 0.8660254037844402619, 0.000000000000000000 ) ) ;
#92288=CARTESIAN_POINT ( 'NONE',  ( 34.47489329363036603, 42.83705186507756935, 3.090169943749475401 ) ) ;
#92291=CARTESIAN_POINT ( 'NONE',  ( 72.54816569808836846, 70.68207713539274550, -7.935695741106854051 ) ) ;
#92292=CARTESIAN_POINT ( 'NONE',  ( 36.94473716931751284, 21.73415679381824361, -6.890680421881970419E-14 ) ) ;
#92293=CARTESIAN_POINT ( 'NONE',  ( 43.88624854525928498, 27.19860640527296169, 2.839279412974134775 ) ) ;
#92301=CARTESIAN_POINT ( 'NONE',  ( 23.18645373101242413, 19.10170272979927120, -7.433330006724141015 ) ) ;
#92303=CARTESIAN_POINT ( 'NONE',  ( 72.03863647653309954, 59.27131230149748831, 15.84878527872051279 ) ) ;
#92305=ORIENTED_EDGE ( 'NONE', *, *, #92211, .T. ) ;
#92306=CARTESIAN_POINT ( 'NONE',  ( 79.57426776854913442, 46.24084366570346560, -13.18946159588284139 ) ) ;
#92308=CARTESIAN_POINT ( 'NONE',  ( 81.82544566900152461, 42.13177917682811824, 7.581690138153514447 ) ) ;
#92311=CARTESIAN_POINT ( 'NONE',  ( 72.37288529989473318, 71.73372848700918780, -5.731447342215284735 ) ) ;
#92313=CARTESIAN_POINT ( 'NONE',  ( 76.59502500117768875, 63.79608208629903032, 14.86840811388221439 ) ) ;
#92318=B_SPLINE_CURVE_WITH_KNOTS ( 'NONE', 3,
 ( #18228, #42493, #34898, #19250, #65798, #73426, #10628, #11142, #40990, #87196 ),
 .UNSPECIFIED., .F., .F.,
 ( 4, 2, 2, 2, 4 ),
 ( 0.000000000000000000, 0.2500000000000000000, 0.5000000000000000000, 0.7500000000000000000, 1.000000000000000000 ),
 .UNSPECIFIED. ) ;
#92322=CARTESIAN_POINT ( 'NONE',  ( 71.81093420572706520, 69.41658505044310346, 9.148441192301559610 ) ) ;
#92324=CARTESIAN_POINT ( 'NONE',  ( 71.59204759908475069, 69.79570777427565531, -8.447857603145788374 ) ) ;
#92330=CARTESIAN_POINT ( 'NONE',  ( 74.90805568670471359, 65.07985694792712650, 13.78103290621842270 ) ) ;
#92332=FACE_OUTER_BOUND ( 'NONE', #75636, .T. ) ;
#92333=CARTESIAN_POINT ( 'NONE',  ( 78.19421406511375494, 47.63508073124027220, -14.44498547994805016 ) ) ;
#92337=CARTESIAN_POINT ( 'NONE',  ( 41.50110961350213046, 24.36477965099642873, 1.583844403245330712 ) ) ;
#92348=CARTESIAN_POINT ( 'NONE',  ( 71.02066284800852713, 69.66031639842336176, 7.328838084737518521 ) ) ;
#92351=CARTESIAN_POINT ( 'NONE',  ( 67.01638591644868370, 66.89576277548633243, 8.813849967855754031 ) ) ;
#92353=CARTESIAN_POINT ( 'NONE',  ( 78.53005147510766903, 47.90408355870507506, 13.93219832960360094 ) ) ;
#92357=CARTESIAN_POINT ( 'NONE',  ( 83.62483622648333892, 41.61889388988494431, -1.100529281121362501 ) ) ;
#92358=CARTESIAN_POINT ( 'NONE',  ( 87.77948443791279942, 45.22530890134208903, -6.970560438077714416 ) ) ;
#92359=CARTESIAN_POINT ( 'NONE',  ( 79.29099298814826113, 45.77971119220809015, 12.98826949500056926 ) ) ;
#92364=ORIENTED_EDGE ( 'NONE', *, *, #74921, .T. ) ;
#92376=CARTESIAN_POINT ( 'NONE',  ( 85.74825148587619594, 48.61567592689142003, -12.33318615817162645 ) ) ;
#92377=VERTEX_POINT ( 'NONE', #54926 ) ;
#92379=CARTESIAN_POINT ( 'NONE',  ( 74.14452735224477919, 67.86235095172764886, -11.65459263701698234 ) ) ;
#92383=ADVANCED_FACE ( 'NONE', ( #17954 ), #70629, .T. ) ;
#92386=B_SPLINE_CURVE_WITH_KNOTS ( 'NONE', 3,
 ( #81450, #66699, #90045, #5902, #52005, #97634, #66214, #74337, #5413, #91044 ),
 .UNSPECIFIED., .F., .F.,
 ( 4, 2, 2, 2, 4 ),
 ( 0.000000000000000000, 0.0002622400424272520970, 0.0005244800848545041940, 0.0007867201272817562910, 0.001048960169709008388 ),
 .UNSPECIFIED. ) ;
#92394=CARTESIAN_POINT ( 'NONE',  ( 73.03321427718370273, 68.50884256177610609, -10.98349909054766549 ) ) ;
#92401=CARTESIAN_POINT ( 'NONE',  ( 72.90605544040717234, 57.09015056262271059, 16.39620496795493665 ) ) ;
#92403=CARTESIAN_POINT ( 'NONE',  ( 66.42322958073232542, 68.80919999086530936, -4.344013851444929131 ) ) ;
#92404=ORIENTED_EDGE ( 'NONE', *, *, #56831, .T. ) ;
#92408=CARTESIAN_POINT ( 'NONE',  ( 33.90351810284484202, 25.28920272979928896, -7.433330006724141015 ) ) ;
#92412=CARTESIAN_POINT ( 'NONE',  ( 68.98401675473516548, 68.40627949866706103, 8.275036679873185363 ) ) ;
#92414=CARTESIAN_POINT ( 'NONE',  ( 68.56394572365037732, 64.18846526882273906, 11.84148672416030124 ) ) ;
#92419=CARTESIAN_POINT ( 'NONE',  ( 14.85095921958720666, 14.28920272979925699, -7.433330006724141015 ) ) ;
#92423=CARTESIAN_POINT ( 'NONE',  ( 69.69525977227351632, 62.53367147251394442, 13.41414775225847755 ) ) ;
#92425=CARTESIAN_POINT ( 'NONE',  ( 71.71459329694582152, 72.12586688595882833, 0.6178152589126062466 ) ) ;
#92435=ORIENTED_EDGE ( 'NONE', *, *, #63166, .T. ) ;
#92438=CARTESIAN_POINT ( 'NONE',  ( 81.37277742391516711, 45.49914513073889566, -11.21303457981032103 ) ) ;
#92445=CARTESIAN_POINT ( 'NONE',  ( 69.41441713838028704, 62.72891755904008448, 13.20643227790562335 ) ) ;
#92450=CARTESIAN_POINT ( 'NONE',  ( 81.68042570781203437, 42.31879938090973070, -8.022231220700685839 ) ) ;
#92454=CARTESIAN_POINT ( 'NONE',  ( 73.95930103172710801, 63.91830289297120515, 14.08246017068975142 ) ) ;
#92456=EDGE_LOOP ( 'NONE', ( #20059, #59126, #42414, #14785 ) ) ;
#92457=CARTESIAN_POINT ( 'NONE',  ( 67.75555162469370885, 67.74667152934745218, 7.221070002596457371 ) ) ;
#92460=CARTESIAN_POINT ( 'NONE',  ( 81.98865867772765625, 45.57652215286253750, 10.94910104189580657 ) ) ;
#92463=CARTESIAN_POINT ( 'NONE',  ( 82.53793375827495993, 54.22719885510827709, -15.94096427280454442 ) ) ;
#92465=CARTESIAN_POINT ( 'NONE',  ( 17.47068606603513530, 15.80170272979925628, 7.433330006724137462 ) ) ;
#92467=CARTESIAN_POINT ( 'NONE',  ( 78.75297625639956323, 47.66336229257159118, 14.29739783539339371 ) ) ;
#92468=CARTESIAN_POINT ( 'NONE',  ( 79.14312167556931854, 57.64441083166269664, 0.000000000000000000 ) ) ;
#92473=CARTESIAN_POINT ( 'NONE',  ( 79.48876273271771709, 46.38894273206648222, -12.71961528548989406 ) ) ;
#92478=CARTESIAN_POINT ( 'NONE',  ( 72.59700804457577306, 63.00543003063684466, -14.10603509414891654 ) ) ;
#92489=ORIENTED_EDGE ( 'NONE', *, *, #34876, .F. ) ;
#92493=CARTESIAN_POINT ( 'NONE',  ( 83.03036255845053404, 46.46437440478001690, -11.26726318583448183 ) ) ;
#92497=CARTESIAN_POINT ( 'NONE',  ( 82.03292314450337130, 42.28330721560684680, 6.570821834211296952 ) ) ;
#92506=CARTESIAN_POINT ( 'NONE',  ( 76.56057136519696371, 54.76627436849224750, -16.10539304684806083 ) ) ;
#92525=CARTESIAN_POINT ( 'NONE',  ( 9.022134044517839513, 26.18502408145589655, 5.678558825948277544 ) ) ;
#92527=CARTESIAN_POINT ( 'NONE',  ( 81.30975366074838462, 56.24313983998633404, -16.44754541364716971 ) ) ;
#92529=CARTESIAN_POINT ( 'NONE',  ( 86.80939509573987323, 43.35552860557069010, -0.1859311002499181298 ) ) ;
#92538=CARTESIAN_POINT ( 'NONE',  ( 25.99623195869281744, 35.98502408145594700, -5.678558825948271327 ) ) ;
#92539=CARTESIAN_POINT ( 'NONE',  ( 71.96639307748559133, 71.49757472301891426, -5.734781593071442529 ) ) ;
#92544=B_SPLINE_SURFACE_WITH_KNOTS ( 'NONE', 3, 1, ( 
 ( #59993, #75728 ),
 ( #99524, #45300 ),
 ( #61494, #6808 ),
 ( #69096, #91957 ),
 ( #68105, #14895 ),
 ( #37204, #92445 ),
 ( #22990, #62477 ),
 ( #8309, #30107 ),
 ( #47291, #100023 ),
 ( #77723, #38180 ),
 ( #53882, #69599 ),
 ( #37690, #29613 ),
 ( #54893, #204 ),
 ( #76234, #30609 ),
 ( #15380, #99026 ),
 ( #16400, #77203 ),
 ( #78217, #70090 ),
 ( #23995, #84842 ),
 ( #91444, #700 ),
 ( #76705, #83852 ),
 ( #46277, #14418 ),
 ( #7808, #45784 ),
 ( #68600, #22505 ),
 ( #61977, #85347 ),
 ( #31090, #85873 ),
 ( #92931, #7299 ),
 ( #23483, #84348 ),
 ( #60990, #38694 ),
 ( #53399, #54373 ),
 ( #93442, #39173 ),
 ( #15894, #60485 ) ),
 .UNSPECIFIED., .F., .F., .F.,
 ( 4, 3, 3, 3, 3, 3, 3, 3, 3, 3, 4 ),
 ( 2, 2 ),
 ( 0.000000000000000000, 0.1122669598086646486, 0.2243161639709356503, 0.3396355846218876984, 0.4553962076585064134, 0.5677860799922357371, 0.6749047109689600976, 0.7773884377078469354, 0.8775581155834195624, 0.9782364162377885641, 1.000000000000000000 ),
 ( 0.000000000000000000, 1.000000000000000000 ),
 .UNSPECIFIED. ) ;
#92545=CARTESIAN_POINT ( 'NONE',  ( 84.44631528110988938, 49.90853024617071299, -13.72425691458318475 ) ) ;
#92546=CARTESIAN_POINT ( 'NONE',  ( 85.51825389741982519, 45.42935502215924259, 9.290761976430086833 ) ) ;
#92553=CARTESIAN_POINT ( 'NONE',  ( 38.16387531507685793, 24.96004757982092315, -5.678558825948276656 ) ) ;
#92555=CARTESIAN_POINT ( 'NONE',  ( 66.52662661294374402, 68.71800325113713370, 4.800704629298682136 ) ) ;
#92559=CARTESIAN_POINT ( 'NONE',  ( 86.55235766077406367, 47.22292317728852140, -10.66532192617879637 ) ) ;
#92562=CARTESIAN_POINT ( 'NONE',  ( 85.05685448785742153, 49.86430017123296210, 13.48384481714161787 ) ) ;
#92567=DIRECTION ( 'NONE',  ( 0.5000000000000013323, -0.8660254037844378194, 0.000000000000000000 ) ) ;
#92573=ORIENTED_EDGE ( 'NONE', *, *, #88127, .F. ) ;
#92575=CARTESIAN_POINT ( 'NONE',  ( 79.81870009848962866, 57.67573475680517703, 16.25934251437179512 ) ) ;
#92576=ORIENTED_EDGE ( 'NONE', *, *, #83409, .F. ) ;
#92586=CARTESIAN_POINT ( 'NONE',  ( 70.43138065582230922, 60.95397308647202550, -14.95463465097626354 ) ) ;
#92587=CARTESIAN_POINT ( 'NONE',  ( 37.18479240120036167, 39.65586893147759895, -7.433330006724137462 ) ) ;
#92590=CARTESIAN_POINT ( 'NONE',  ( 86.81792973151222270, 45.86417987983289635, -8.215134288092611925 ) ) ;
#92591=CARTESIAN_POINT ( 'NONE',  ( 74.16718187723988365, 63.24922278397193764, -14.42629137139557827 ) ) ;
#92592=DIRECTION ( 'NONE',  ( -0.8660254037844378194, -0.5000000000000013323, -0.000000000000000000 ) ) ;
#92594=CARTESIAN_POINT ( 'NONE',  ( 72.00815872078212010, 61.71914051830567161, 14.51550446260311134 ) ) ;
#92620=CARTESIAN_POINT ( 'NONE',  ( 82.21690911714624406, 41.97360749678824732, 5.658590786372603709 ) ) ;
#92623=CARTESIAN_POINT ( 'NONE',  ( 72.17187393125894346, 66.23161324361963409, -12.52721847853723247 ) ) ;
#92633=CARTESIAN_POINT ( 'NONE',  ( 73.48070833180072725, 69.95435187952867295, -9.683457271946362965 ) ) ;
#92634=CARTESIAN_POINT ( 'NONE',  ( 76.43143940513256496, 51.47447208219396231, 15.62944959062109440 ) ) ;
#92636=EDGE_CURVE ( 'NONE', #12691, #58645, #91054, .T. ) ;
#92645=CARTESIAN_POINT ( 'NONE',  ( 88.10161777267849459, 43.64076697146427364, 0.1132407729617423420 ) ) ;
#92646=CARTESIAN_POINT ( 'NONE',  ( 82.09089402055167284, 49.99296431688566145, -14.01874078344520669 ) ) ;
#92650=CARTESIAN_POINT ( 'NONE',  ( 25.00689474275853286, 16.29860640527292759, -2.839279412974138328 ) ) ;
#92653=CARTESIAN_POINT ( 'NONE',  ( 14.85095921958720666, 14.28920272979925699, -7.433330006724141015 ) ) ;
#92665=CARTESIAN_POINT ( 'NONE',  ( 77.09205440684367261, 49.43085972797705097, 15.45120731324600349 ) ) ;
#92670=CARTESIAN_POINT ( 'NONE',  ( 71.37166012509962343, 68.88869991590640041, -8.754280617899828698 ) ) ;
#92674=ADVANCED_FACE ( 'NONE', ( #12856 ), #88880, .T. ) ;
#92679=CARTESIAN_POINT ( 'NONE',  ( 23.56475526289127842, 35.64646525600391413, -2.839279412974133887 ) ) ;
#92680=CARTESIAN_POINT ( 'NONE',  ( 27.68909066282341058, 16.39040679176984128, 1.333680081654574804E-15 ) ) ;
#92682=CARTESIAN_POINT ( 'NONE',  ( 75.03771487841179066, 67.29470115673240116, -12.93936238812017514 ) ) ;
#92684=VECTOR ( 'NONE', #35195, 1000.000000000000000 ) ;
#92685=ORIENTED_EDGE ( 'NONE', *, *, #94357, .T. ) ;
#92686=PLANE ( 'NONE',  #83850 ) ;
#92690=CARTESIAN_POINT ( 'NONE',  ( 67.64135108386106765, 65.79995805064302772, 10.56434706573462634 ) ) ;
#92691=CARTESIAN_POINT ( 'NONE',  ( 67.97241529915037006, 65.50463755924691611, -10.32544819515218038 ) ) ;
#92701=VERTEX_POINT ( 'NONE', #37603 ) ;
#92708=CARTESIAN_POINT ( 'NONE',  ( 66.69662207783855479, 67.50385436546183371, 6.505031878347596219 ) ) ;
#92713=CARTESIAN_POINT ( 'NONE',  ( 72.10474246843376989, 68.41231093896740845, 9.878068674442724628 ) ) ;
#92717=CARTESIAN_POINT ( 'NONE',  ( 15.84452179826556417, 32.08080186712592763, -3.090169943749475845 ) ) ;
#92721=CARTESIAN_POINT ( 'NONE',  ( 18.12000580879176326, 26.16454794089041513, -10.00000000000000355 ) ) ;
#92729=CARTESIAN_POINT ( 'NONE',  ( 42.94622797204061726, 25.76426979415093044, 3.090169943749476733 ) ) ;
#92731=CARTESIAN_POINT ( 'NONE',  ( 72.57700935610729687, 70.89248372566723333, 7.619130926959992500 ) ) ;
#92736=FACE_OUTER_BOUND ( 'NONE', #30489, .T. ) ;
#92738=CARTESIAN_POINT ( 'NONE',  ( 83.61138909378800577, 52.00041238365411544, 15.00249647689079424 ) ) ;
#92740=ORIENTED_EDGE ( 'NONE', *, *, #3657, .T. ) ;
#92741=EDGE_CURVE ( 'NONE', #40803, #90112, #1640, .T. ) ;
#92745=CARTESIAN_POINT ( 'NONE',  ( 73.66703090666727860, 55.44584689847431491, 16.58622807595889270 ) ) ;
#92748=CARTESIAN_POINT ( 'NONE',  ( 24.60437102317565206, 29.90829794293881960, 10.00000000000000355 ) ) ;
#92750=CARTESIAN_POINT ( 'NONE',  ( 87.35668359673078953, 44.84080960044052944, -6.701380392922970053 ) ) ;
#92757=VECTOR ( 'NONE', #38158, 1000.000000000000000 ) ;
#92758=CARTESIAN_POINT ( 'NONE',  ( 66.74743652013738426, 67.50578830241221340, -6.557104418870829399 ) ) ;
#92759=CARTESIAN_POINT ( 'NONE',  ( 73.05894514279327723, 70.71455386244217323, -7.616028886072077064 ) ) ;
#92763=CARTESIAN_POINT ( 'NONE',  ( 35.77580382318486585, 22.78380873178790011, -6.180339887498949025 ) ) ;
#92764=CARTESIAN_POINT ( 'NONE',  ( 83.57802576903957004, 41.91920785109143566, -3.213770064112233982 ) ) ;
#92766=DIRECTION ( 'NONE',  ( 0.4996954135095463823, -0.8654978445076774163, -0.03489949670249753444 ) ) ;
#92768=CARTESIAN_POINT ( 'NONE',  ( 82.86808232639344851, 43.79884615191943453, 9.160507364924834306 ) ) ;
#92772=CARTESIAN_POINT ( 'NONE',  ( 82.09598787739267323, 41.22586304043770866, 5.427194921701099517 ) ) ;
#92777=CARTESIAN_POINT ( 'NONE',  ( 33.91574581199579086, 27.78052372038643369, -10.00000000000000355 ) ) ;
#92779=CARTESIAN_POINT ( 'NONE',  ( 85.68485941944550177, 48.66523437743575187, 11.91861461389294163 ) ) ;
#92781=DIRECTION ( 'NONE',  ( -0.9532659690011937581, 0.2314883312386630254, -0.1941575258509295188 ) ) ;
#92784=CARTESIAN_POINT ( 'NONE',  ( 21.37261828447143586, 20.84335787977763133, 9.188101187500006262 ) ) ;
#92786=CARTESIAN_POINT ( 'NONE',  ( 72.04273812837081437, 59.28583566120335036, 15.34548535902080246 ) ) ;
#92788=ORIENTED_EDGE ( 'NONE', *, *, #92002, .T. ) ;
#92791=LINE ( 'NONE', #47149, #50099 ) ;
#92792=CARTESIAN_POINT ( 'NONE',  ( 81.89600004460587002, 42.20886894945997625, 7.642739303376051119 ) ) ;
#92796=CARTESIAN_POINT ( 'NONE',  ( 72.40857565946932084, 71.84120774512069829, -5.522868224832428119 ) ) ;
#92797=CARTESIAN_POINT ( 'NONE',  ( 73.09176899391452764, 57.17258086466325295, 16.39964270276630742 ) ) ;
#92803=CARTESIAN_POINT ( 'NONE',  ( 84.69548858147219050, 42.71338583940531208, -3.895673258569514630 ) ) ;
#92804=ORIENTED_EDGE ( 'NONE', *, *, #18984, .T. ) ;
#92807=CYLINDRICAL_SURFACE ( 'NONE', #12729, 16.60714546451156792 ) ;
#92808=CARTESIAN_POINT ( 'NONE',  ( 76.85865272105424140, 63.69649487134743282, 15.33129195839047298 ) ) ;
#92813=ORIENTED_EDGE ( 'NONE', *, *, #71582, .F. ) ;
#92815=LINE ( 'NONE', #16279, #88299 ) ;
#92817=CARTESIAN_POINT ( 'NONE',  ( 31.61033844661487180, 20.11110640527293825, -2.839279412974138328 ) ) ;
#92826=ORIENTED_EDGE ( 'NONE', *, *, #68263, .T. ) ;
#92827=ORIENTED_EDGE ( 'NONE', *, *, #95017, .T. ) ;
#92829=CARTESIAN_POINT ( 'NONE',  ( 82.36003205642018088, 42.70002867508654276, -6.979109086437436105 ) ) ;
#92841=CARTESIAN_POINT ( 'NONE',  ( 75.92693672788908543, 65.58256616235577496, 13.87764565375856662 ) ) ;
#92843=CARTESIAN_POINT ( 'NONE',  ( 78.55383125624311447, 47.44943004927687014, 14.24641143436689816 ) ) ;
#92847=CARTESIAN_POINT ( 'NONE',  ( 70.26774927589852382, 65.27959088349479089, 11.79268299559660349 ) ) ;
#92851=CARTESIAN_POINT ( 'NONE',  ( 83.76909922093737748, 51.72725043056325234, -14.84865573977556075 ) ) ;
#92855=CARTESIAN_POINT ( 'NONE',  ( 72.45582997685151838, 71.59006409230265433, 5.171701996141663926 ) ) ;
#92859=LINE ( 'NONE', #44712, #56146 ) ;
#92863=CARTESIAN_POINT ( 'NONE',  ( 85.70408377067469985, 48.42330189018957043, -11.73456542461740604 ) ) ;
#92865=CARTESIAN_POINT ( 'NONE',  ( 71.45374252289430217, 64.76739115956998205, 12.70080691706103515 ) ) ;
#92866=CARTESIAN_POINT ( 'NONE',  ( 88.07442723472371426, 44.71957171711925838, -4.374393210843437352 ) ) ;
#92870=CARTESIAN_POINT ( 'NONE',  ( 82.08809084460519045, 41.85377707259943492, -5.545080802233028905 ) ) ;
#92871=CARTESIAN_POINT ( 'NONE',  ( 10.49025449741314375, 29.55466486950698624, -1.111400068045478839E-16 ) ) ;
#92876=CARTESIAN_POINT ( 'NONE',  ( 15.42233441037273423, 31.83705186507753382, 3.090169943749475401 ) ) ;
#92882=CARTESIAN_POINT ( 'NONE',  ( 16.70795526530605457, 14.81029122506293483, 8.090169943749479842 ) ) ;
#92885=CARTESIAN_POINT ( 'NONE',  ( 73.06502562637749065, 69.62150218382535627, 9.203196011093488949 ) ) ;
#92889=CARTESIAN_POINT ( 'NONE',  ( 72.61312054461893695, 57.22205865948716763, 15.86921491991221522 ) ) ;
#92890=DIRECTION ( 'NONE',  ( 0.2588190451025306205, 0.9659258262890656477, 0.000000000000000000 ) ) ;
#92891=CARTESIAN_POINT ( 'NONE',  ( 66.76842575320728201, 68.41059621743521291, -4.427724692764615888 ) ) ;
#92897=CARTESIAN_POINT ( 'NONE',  ( 30.51038259252555207, 29.56628583063842441, 9.188101187500006262 ) ) ;
#92903=CARTESIAN_POINT ( 'NONE',  ( 66.43068645214782464, 68.73212257389783986, 2.345923867857303335 ) ) ;
#92905=DIRECTION ( 'NONE',  ( -0.6758705274779386318, -0.2489746672676196315, -0.6936934806855771241 ) ) ;
#92909=CARTESIAN_POINT ( 'NONE',  ( 18.45335787429653251, 11.44966523072493558, -2.296566073217252530E-15 ) ) ;
#92910=VERTEX_POINT ( 'NONE', #72546 ) ;
#92913=CARTESIAN_POINT ( 'NONE',  ( 23.90938336746022586, 36.73705186507755371, -3.090169943749475845 ) ) ;
#92923=CARTESIAN_POINT ( 'NONE',  ( 71.17064988840769502, 70.28013413260883624, 7.276424097237452315 ) ) ;
#92924=CARTESIAN_POINT ( 'NONE',  ( 87.14288108606291416, 44.98988116358240319, -6.378897604470720850 ) ) ;
#92928=CARTESIAN_POINT ( 'NONE',  ( 17.13867093926436169, 10.86426979415088567, -3.090169943749474069 ) ) ;
#92929=CARTESIAN_POINT ( 'NONE',  ( 86.13879346367242817, 46.95025718893441535, -10.63009676298478823 ) ) ;
#92930=EDGE_CURVE ( 'NONE', #93753, #89224, #95382, .T. ) ;
#92931=CARTESIAN_POINT ( 'NONE',  ( 69.91735932814472676, 62.82170394719442896, 13.89425379104851999 ) ) ;
#92941=CARTESIAN_POINT ( 'NONE',  ( 68.42993948008529514, 68.72088526677468678, 6.145480275798111514 ) ) ;
#92944=CARTESIAN_POINT ( 'NONE',  ( 83.59982691654131770, 50.63482651926307909, 13.94564167549828504 ) ) ;
#92948=CARTESIAN_POINT ( 'NONE',  ( 82.75828967192548191, 53.74568045750391576, -15.77735475420663924 ) ) ;
#92952=CARTESIAN_POINT ( 'NONE',  ( 19.48598279363274344, 13.11110640527291693, -2.839279412974138328 ) ) ;
#92954=CARTESIAN_POINT ( 'NONE',  ( 80.73437012277888414, 57.38180594535329249, 16.57560423861647081 ) ) ;
#92960=CARTESIAN_POINT ( 'NONE',  ( 77.14944321224352564, 49.32060529837239926, -15.40190492294266278 ) ) ;
#92961=B_SPLINE_CURVE_WITH_KNOTS ( 'NONE', 3,
 ( #27360, #42048, #97283, #4547, #19770, #66350, #50153, #65352, #90191, #65835, #74966, #57736, #43023, #5548, #26860, #20767, #81105, #18768, #49645, #82099, #58242, #43540, #72982, #74481 ),
 .UNSPECIFIED., .F., .F.,
 ( 4, 2, 2, 2, 2, 2, 2, 2, 2, 2, 2, 4 ),
 ( 0.000000000000000000, 0.1250000000000053568, 0.2500000000000107137, 0.3750000000000160982, 0.4375000000000109912, 0.5000000000000058842, 0.5625000000000007772, 0.6249999999999956701, 0.6874999999999905631, 0.7499999999999854561, 0.8749999999999927836, 1.000000000000000000 ),
 .UNSPECIFIED. ) ;
#92962=CARTESIAN_POINT ( 'NONE',  ( 83.79436218315080964, 45.74912830802215780, -10.11333493852419707 ) ) ;
#92968=CARTESIAN_POINT ( 'NONE',  ( 74.84872400778057511, 66.80276697526575447, -13.19923776164384499 ) ) ;
#92972=CARTESIAN_POINT ( 'NONE',  ( 82.87432691701982890, 53.54933337481561750, -15.33804591960182861 ) ) ;
#92973=CARTESIAN_POINT ( 'NONE',  ( 15.58658660100807580, 11.12755873383624561, -6.180339887498949025 ) ) ;
#92975=DIRECTION ( 'NONE',  ( 0.9659258262890674240, -0.2588190451025239036, 8.659560562355041327E-17 ) ) ;
#92977=CARTESIAN_POINT ( 'NONE',  ( 75.58214075417596689, 65.23491603964201602, 14.35294216029143755 ) ) ;
#92983=EDGE_CURVE ( 'NONE', #57886, #79592, #80666, .T. ) ;
#92988=CARTESIAN_POINT ( 'NONE',  ( 74.02653709664873816, 68.32631449583556105, -11.67658431812981412 ) ) ;
#92996=CARTESIAN_POINT ( 'NONE',  ( 38.51867309874058520, 23.20801979619931643, -3.090169943749474069 ) ) ;
#93000=CARTESIAN_POINT ( 'NONE',  ( 82.31162263179685112, 47.02075270482669112, 12.63320473991187676 ) ) ;
#93002=CARTESIAN_POINT ( 'NONE',  ( 72.12483444493729223, 64.99830324756513278, 13.36562007551493281 ) ) ;
#93005=CARTESIAN_POINT ( 'NONE',  ( 69.77287440015896891, 69.89897948854762433, 5.259387334649119339 ) ) ;
#93012=CARTESIAN_POINT ( 'NONE',  ( 8.675723883004062387, 25.98502408145591147, -5.678558825948271327 ) ) ;
#93014=CARTESIAN_POINT ( 'NONE',  ( 79.86306577577953192, 56.87384565298960126, -16.58767780902013911 ) ) ;
#93015=CARTESIAN_POINT ( 'NONE',  ( 19.29290913472606661, 12.10801979619928126, 3.090169943749476733 ) ) ;
#93025=CARTESIAN_POINT ( 'NONE',  ( 69.28997898220227114, 64.65901494164410224, -12.44462553223597823 ) ) ;
#93029=CARTESIAN_POINT ( 'NONE',  ( 79.21012467913614330, 50.17711341405016867, 14.78417737531875886 ) ) ;
#93032=CARTESIAN_POINT ( 'NONE',  ( 77.08943580299947484, 49.61595851769167353, 15.51385818994994459 ) ) ;
#93033=CARTESIAN_POINT ( 'NONE',  ( 74.95739461836087969, 53.28572374827752611, -16.04297136957062264 ) ) ;
#93036=CARTESIAN_POINT ( 'NONE',  ( 73.53729735990698657, 69.85633680769765874, 9.839233502311348190 ) ) ;
#93037=CARTESIAN_POINT ( 'NONE',  ( 34.67813663163181559, 40.99752408145594273, 5.678558825948277544 ) ) ;
#93043=CARTESIAN_POINT ( 'NONE',  ( 86.13879346367242817, 46.95025718893440825, -10.63009676298480422 ) ) ;
#93046=CARTESIAN_POINT ( 'NONE',  ( 85.87384404189388931, 44.42517650707678456, -7.508811624228250103 ) ) ;
#93049=CARTESIAN_POINT ( 'NONE',  ( 84.81216594078708226, 50.08139507223255293, -13.70157583983569971 ) ) ;
#93055=CARTESIAN_POINT ( 'NONE',  ( 77.23449085028160255, 49.20386544400301432, -14.82971331545884652 ) ) ;
#93060=CARTESIAN_POINT ( 'NONE',  ( 36.34934470066777834, 21.39040679176985194, 1.333680081654574804E-15 ) ) ;
#93062=CARTESIAN_POINT ( 'NONE',  ( 70.22362515028090968, 62.13392031687246941, -13.81625945947303080 ) ) ;
#93069=CARTESIAN_POINT ( 'NONE',  ( 70.39572275625086206, 61.09682404813923995, -14.88543345152358022 ) ) ;
#93070=CARTESIAN_POINT ( 'NONE',  ( 34.67813663163181559, 40.99752408145594273, 5.678558825948277544 ) ) ;
#93072=ORIENTED_EDGE ( 'NONE', *, *, #57154, .F. ) ;
#93073=VECTOR ( 'NONE', #11318, 1000.000000000000114 ) ;
#93078=CARTESIAN_POINT ( 'NONE',  ( 72.08687029594609896, 62.01746031163174422, 14.40919635732520021 ) ) ;
#93079=CARTESIAN_POINT ( 'NONE',  ( 66.27017796984547715, 68.16393141397755073, 4.308032648087416483 ) ) ;
#93084=CARTESIAN_POINT ( 'NONE',  ( 74.85238693809837685, 54.71601908059493269, -16.61539935277903268 ) ) ;
#93086=CARTESIAN_POINT ( 'NONE',  ( 83.37296956034946049, 51.74080471427829053, 14.95189368521467976 ) ) ;
#93087=CARTESIAN_POINT ( 'NONE',  ( 65.98272894656351184, 68.67277586300092196, -0.2982986715729523119 ) ) ;
#93100=EDGE_CURVE ( 'NONE', #89249, #92701, #96271, .T. ) ;
#93101=CARTESIAN_POINT ( 'NONE',  ( 72.47507403108335211, 60.92439914301793635, 15.41744962056277224 ) ) ;
#93107=CARTESIAN_POINT ( 'NONE',  ( 85.30910355950469182, 47.43175382727999079, 10.99938408205740004 ) ) ;
#93110=( BOUNDED_CURVE ( )  B_SPLINE_CURVE ( 2, ( #12755, #7113, #14719, #53221, #83666, #84172, #75536, #90278, #6630, #6121, #21821, #74559, #37017 ),
 .UNSPECIFIED., .F., .T. ) 
 B_SPLINE_CURVE_WITH_KNOTS ( ( 3, 2, 2, 2, 2, 2, 3 ),
 ( 0.4124999999999999778, 0.4149999999999999800, 0.4199999999999999845, 0.4249999999999999889, 0.4299999999999999933, 0.4349999999999999978, 0.4375000000000000000 ),
 .UNSPECIFIED. ) 
 CURVE ( )  GEOMETRIC_REPRESENTATION_ITEM ( )  RATIONAL_B_SPLINE_CURVE ( ( 0.9755282581475768211, 0.9755282581475768211, 1.000000000000000000, 0.9510565162951535312, 1.000000000000000000, 0.9510565162951535312, 1.000000000000000000, 0.9510565162951535312, 1.000000000000000000, 0.9510565162951535312, 1.000000000000000000, 0.9755282581475768211, 0.9755282581475768211 ) ) 
 REPRESENTATION_ITEM ( '' )  );
#93113=CARTESIAN_POINT ( 'NONE',  ( 69.66464655795641647, 66.64923878050555572, -10.89182121580662432 ) ) ;
#93120=EDGE_CURVE ( 'NONE', #61384, #37680, #31435, .T. ) ;
#93121=CARTESIAN_POINT ( 'NONE',  ( 78.60047569677259105, 58.74348153791917326, 16.19982007990188322 ) ) ;
#93122=CARTESIAN_POINT ( 'NONE',  ( 84.78559661328758068, 49.87520375107067849, -13.17027106718964902 ) ) ;
#93124=CARTESIAN_POINT ( 'NONE',  ( 78.31490237461567006, 61.48931456610748825, 15.81469504661664516 ) ) ;
#93125=CARTESIAN_POINT ( 'NONE',  ( 73.44801800142467130, 69.18349203779057177, -9.987627434106716606 ) ) ;
#93126=CARTESIAN_POINT ( 'NONE',  ( 76.16734681154976272, 51.14571779461076773, 16.08280053340072868 ) ) ;
#93137=CARTESIAN_POINT ( 'NONE',  ( 82.21410988452117863, 40.73976263626466476, 3.762362152834610729 ) ) ;
#93138=CARTESIAN_POINT ( 'NONE',  ( 88.24973202300745356, 44.12735596345137168, 0.4777715347392412215 ) ) ;
#93139=CARTESIAN_POINT ( 'NONE',  ( 83.93511005065496988, 49.44454015237737821, -13.15056953514552518 ) ) ;
#93143=CARTESIAN_POINT ( 'NONE',  ( 25.38519627463738715, 32.84336893147757053, -7.433330006724137462 ) ) ;
#93145=CARTESIAN_POINT ( 'NONE',  ( 82.94087190812932420, 47.09133877588998018, -11.82568837119483085 ) ) ;
#93146=CARTESIAN_POINT ( 'NONE',  ( 12.59929316974766955, 12.98920272979924739, 7.433330006724137462 ) ) ;
#93148=CARTESIAN_POINT ( 'NONE',  ( 77.16076033720362659, 63.58031483167507503, 15.43380074518343825 ) ) ;
#93153=B_SPLINE_CURVE_WITH_KNOTS ( 'NONE', 3,
 ( #50624, #81091, #80589, #19756, #35925, #19272, #88202, #11657, #12657, #57722 ),
 .UNSPECIFIED., .F., .F.,
 ( 4, 2, 2, 2, 4 ),
 ( 0.000000000000000000, 0.0002622400424272852736, 0.0005244800848545705472, 0.0007867201272818558208, 0.001048960169709141094 ),
 .UNSPECIFIED. ) ;
#93155=CARTESIAN_POINT ( 'NONE',  ( 75.50969905168113883, 56.69343460978081595, -16.12022845293416751 ) ) ;
#93156=CARTESIAN_POINT ( 'NONE',  ( 87.51070308547132015, 44.87157588833125033, -6.586006751413206572 ) ) ;
#93161=CARTESIAN_POINT ( 'NONE',  ( 77.12302860632740931, 49.36369884983294298, 15.42198964217536528 ) ) ;
#93166=CARTESIAN_POINT ( 'NONE',  ( 67.84800455489335036, 68.64766278059737203, -5.501624410574179613 ) ) ;
#93167=ORIENTED_EDGE ( 'NONE', *, *, #13148, .T. ) ;
#93170=CARTESIAN_POINT ( 'NONE',  ( 79.36831560114676165, 46.38765329515769764, -12.76462913186217030 ) ) ;
#93172=CARTESIAN_POINT ( 'NONE',  ( 82.52530459147394026, 45.85050490410911550, 11.59675866233544106 ) ) ;
#93173=ORIENTED_EDGE ( 'NONE', *, *, #92002, .F. ) ;
#93174=CARTESIAN_POINT ( 'NONE',  ( 31.61033844661487180, 20.11110640527293825, -2.839279412974138328 ) ) ;
#93175=CARTESIAN_POINT ( 'NONE',  ( 75.38962278209211831, 56.66636018296492239, 16.13016272302565213 ) ) ;
#93177=CARTESIAN_POINT ( 'NONE',  ( 74.68932948184824738, 66.80812537921997318, -13.13442079021221609 ) ) ;
#93183=CARTESIAN_POINT ( 'NONE',  ( 67.90965126688126929, 65.44846603141178321, 10.34735008748251595 ) ) ;
#93184=CARTESIAN_POINT ( 'NONE',  ( 68.01698362341183213, 65.55827135151169216, -10.29583288777463679 ) ) ;
#93191=EDGE_CURVE ( 'NONE', #76006, #89530, #94290, .T. ) ;
#93202=CARTESIAN_POINT ( 'NONE',  ( 66.69106175333467945, 67.85483539735206193, 6.981201250520606472 ) ) ;
#93206=CARTESIAN_POINT ( 'NONE',  ( 81.29827136372979624, 55.78681482234479461, 16.38844377500790017 ) ) ;
#93212=ORIENTED_EDGE ( 'NONE', *, *, #86491, .T. ) ;
#93216=CARTESIAN_POINT ( 'NONE',  ( 21.19599769036394932, 20.43677371833801359, -10.00000000000000355 ) ) ;
#93217=CARTESIAN_POINT ( 'NONE',  ( 76.26204961069845467, 64.89063096657046970, -14.31995487015190172 ) ) ;
#93224=CARTESIAN_POINT ( 'NONE',  ( 84.94358975746530405, 43.75860775811098335, -6.241023248769397291 ) ) ;
#93225=CARTESIAN_POINT ( 'NONE',  ( 39.55573625059403753, 31.03677371833805054, 10.00000000000000533 ) ) ;
#93226=CARTESIAN_POINT ( 'NONE',  ( 29.10553579016685077, 39.73705186507756082, -3.090169943749475845 ) ) ;
#93229=CARTESIAN_POINT ( 'NONE',  ( 72.56545876662167416, 70.71212947315848396, 7.162847399348136079 ) ) ;
#93230=CARTESIAN_POINT ( 'NONE',  ( 71.98158595747280231, 67.14350720622732638, -11.10114360595152050 ) ) ;
#93237=CARTESIAN_POINT ( 'NONE',  ( 83.40084016564935609, 52.41263683630168657, 14.84168028052237176 ) ) ;
#93240=ORIENTED_EDGE ( 'NONE', *, *, #80679, .F. ) ;
#93247=CARTESIAN_POINT ( 'NONE',  ( 73.77213256992256163, 55.19446632860606883, 16.59757308087127825 ) ) ;
#93249=EDGE_CURVE ( 'NONE', #96074, #2731, #37538, .T. ) ;
#93250=CARTESIAN_POINT ( 'NONE',  ( 32.18369500442690878, 26.78052372038641948, -10.00000000000000355 ) ) ;
#93253=LINE ( 'NONE', #8128, #97100 ) ;
#93261=CARTESIAN_POINT ( 'NONE',  ( 81.57802524835842917, 41.68064318211084185, 5.833990239057619931 ) ) ;
#93263=CARTESIAN_POINT ( 'NONE',  ( 25.74102936209481385, 30.56454794089042437, 10.00000000000000355 ) ) ;
#93264=CARTESIAN_POINT ( 'NONE',  ( 36.19122982252199705, 21.86426979415092120, -3.090169943749474069 ) ) ;
#93265=CARTESIAN_POINT ( 'NONE',  ( 76.61888230025124358, 51.35972145274618583, 16.07233720520855158 ) ) ;
#93271=CARTESIAN_POINT ( 'NONE',  ( 67.86202049053581220, 66.83700393428978259, -8.676109968774889936 ) ) ;
#93274=CARTESIAN_POINT ( 'NONE',  ( 72.12013178652179590, 70.28500072208976235, -8.194891429308611919 ) ) ;
#93278=B_SPLINE_CURVE_WITH_KNOTS ( 'NONE', 3,
 ( #97535, #28104, #70080, #61970, #14887, #92923, #76698, #86356, #54886, #23476, #77717, #45776, #63495, #1202, #77194, #85866 ),
 .UNSPECIFIED., .F., .F.,
 ( 4, 1, 2, 2, 2, 1, 2, 2, 4 ),
 ( 0.000000000000000000, 0.1250000000000013600, 0.1875000000000028866, 0.2500000000000043854, 0.4999999999999998890, 0.6249999999999976685, 0.6874999999999965583, 0.7499999999999954481, 1.000000000000000000 ),
 .UNSPECIFIED. ) ;
#93280=CARTESIAN_POINT ( 'NONE',  ( 67.32971676510786097, 66.39089803301675374, -8.864210629079892101 ) ) ;
#93284=CARTESIAN_POINT ( 'NONE',  ( 16.26188567080226477, 32.49540643055187417, 3.479690158560446702E-15 ) ) ;
#93286=CARTESIAN_POINT ( 'NONE',  ( 72.03863647653309954, 59.27131230149748831, 15.34878527849881458 ) ) ;
#93289=ORIENTED_EDGE ( 'NONE', *, *, #37013, .F. ) ;
#93290=CARTESIAN_POINT ( 'NONE',  ( 37.76795716069911890, 37.50829794293884589, -10.00000000000000355 ) ) ;
#93292=CARTESIAN_POINT ( 'NONE',  ( 8.697374518098676788, 25.99752408145590366, 5.678558825948276656 ) ) ;
#93293=CARTESIAN_POINT ( 'NONE',  ( 73.37087704974057090, 59.79349537656993618, -15.44674116277980147 ) ) ;
#93294=CARTESIAN_POINT ( 'NONE',  ( 81.89248010131869648, 42.20395449353005546, 7.637921802679397132 ) ) ;
#93297=CARTESIAN_POINT ( 'NONE',  ( 69.27156750288784792, 70.56227451142774498, -1.298478209937802719 ) ) ;
#93304=CARTESIAN_POINT ( 'NONE',  ( 87.13830015243127036, 43.52866481668240084, -0.7691705554832481972 ) ) ;
#93307=CARTESIAN_POINT ( 'NONE',  ( 71.94697066620052794, 72.20377774097838142, -3.624262489285473343 ) ) ;
#93308=CARTESIAN_POINT ( 'NONE',  ( 80.01979875032591849, 57.54866692369599690, 16.59896302490742315 ) ) ;
#93309=CARTESIAN_POINT ( 'NONE',  ( 77.24238159045749796, 63.47610639771342278, 15.48509222746617553 ) ) ;
#93313=VERTEX_POINT ( 'NONE', #423 ) ;
#93319=CARTESIAN_POINT ( 'NONE',  ( 31.84670776885679899, 24.10170272979928541, -7.433330006724141015 ) ) ;
#93321=CARTESIAN_POINT ( 'NONE',  ( 78.19070433545205390, 47.56140015029151868, -14.40966192187991624 ) ) ;
#93322=VERTEX_POINT ( 'NONE', #31312 ) ;
#93325=CARTESIAN_POINT ( 'NONE',  ( 25.26661199696083671, 36.36126292948896577, 6.180339887498949913 ) ) ;
#93327=CARTESIAN_POINT ( 'NONE',  ( 40.62554608437772430, 25.58380873178790083, 6.180339887498953466 ) ) ;
#93340=CARTESIAN_POINT ( 'NONE',  ( 68.70434024268674023, 64.76539896931275564, 11.44226853676074995 ) ) ;
#93342=CARTESIAN_POINT ( 'NONE',  ( 67.44483578933650847, 66.62155022141699590, 8.635578642564382790 ) ) ;
#93343=CARTESIAN_POINT ( 'NONE',  ( 73.51625129091058852, 64.84468117635124429, -13.42585287280998330 ) ) ;
#93344=CARTESIAN_POINT ( 'NONE',  ( 78.56500620533599033, 47.97831951877432743, 13.95998044843349817 ) ) ;
#93346=ORIENTED_EDGE ( 'NONE', *, *, #75481, .F. ) ;
#93348=CARTESIAN_POINT ( 'NONE',  ( 82.81954554793986745, 41.27561870364412755, -2.050892944899044945 ) ) ;
#93351=B_SPLINE_CURVE_WITH_KNOTS ( 'NONE', 3,
 ( #65191, #89546, #59054, #12504, #43375, #20107, #74320, #96635, #89071, #80950 ),
 .UNSPECIFIED., .F., .F.,
 ( 4, 2, 2, 2, 4 ),
 ( 0.000000000000000000, 0.2499999999999991118, 0.4999999999999982236, 0.7499999999999991118, 1.000000000000000000 ),
 .UNSPECIFIED. ) ;
#93353=CARTESIAN_POINT ( 'NONE',  ( 83.83681109075200766, 51.55721269723052558, -14.37373883924508000 ) ) ;
#93354=CARTESIAN_POINT ( 'NONE',  ( 70.15619903503488786, 64.92682878892891551, -12.01717930017344038 ) ) ;
#93355=ORIENTED_EDGE ( 'NONE', *, *, #69288, .F. ) ;
#93358=CARTESIAN_POINT ( 'NONE',  ( 72.48128350488923388, 71.72257018173657173, 5.902110541236717189 ) ) ;
#93368=CARTESIAN_POINT ( 'NONE',  ( 67.41248320326423027, 66.37693208286884783, -8.946798147498746800 ) ) ;
#93369=VERTEX_POINT ( 'NONE', #89567 ) ;
#93370=CARTESIAN_POINT ( 'NONE',  ( 72.47029212360676809, 67.90129717547449673, 10.67585825917434761 ) ) ;
#93377=CARTESIAN_POINT ( 'NONE',  ( 82.09393458893232776, 41.85502508557050305, -5.540192124174895483 ) ) ;
#93388=CARTESIAN_POINT ( 'NONE',  ( 19.28614774617036787, 10.94473085651391386, 1.475505719884397138E-15 ) ) ;
#93392=CARTESIAN_POINT ( 'NONE',  ( 72.24325681757291306, 72.08904859244903207, 3.121326503868123492 ) ) ;
#93398=CARTESIAN_POINT ( 'NONE',  ( 10.48369258086752787, 24.79103043416547791, 8.090169943749478065 ) ) ;
#93408=CARTESIAN_POINT ( 'NONE',  ( 28.93108252874724684, 32.10171378149919974, 9.188101187500008038 ) ) ;
#93414=B_SPLINE_CURVE_WITH_KNOTS ( 'NONE', 3,
 ( #69365, #98292, #44552, #37452, #91205, #53169, #92223, #8080, #83609, #75486 ),
 .UNSPECIFIED., .F., .F.,
 ( 4, 2, 2, 2, 4 ),
 ( 0.000000000000000000, 0.0002622400424272794731, 0.0005244800848545589462, 0.0007867201272818383651, 0.001048960169709117892 ),
 .UNSPECIFIED. ) ;
#93415=CARTESIAN_POINT ( 'NONE',  ( 66.14637081899437021, 69.08478385240519515, 2.576720762024273359 ) ) ;
#93420=CARTESIAN_POINT ( 'NONE',  ( 14.33134397731654630, 13.98920272979924917, 7.433330006724137462 ) ) ;
#93421=ORIENTED_EDGE ( 'NONE', *, *, #45650, .F. ) ;
#93425=CARTESIAN_POINT ( 'NONE',  ( 32.72712820738424000, 19.86426979415091054, -3.090169943749474069 ) ) ;
#93433=CARTESIAN_POINT ( 'NONE',  ( 72.79448081417055505, 70.83012470017415296, 7.186594751207691978 ) ) ;
#93439=CARTESIAN_POINT ( 'NONE',  ( 79.16081066472990813, 59.09338877662139566, -16.21814646735712273 ) ) ;
#93441=CARTESIAN_POINT ( 'NONE',  ( 85.84005213714648619, 47.01912803749855385, -10.88097575854029309 ) ) ;
#93442=CARTESIAN_POINT ( 'NONE',  ( 69.95297458392498413, 62.89479584344802277, 13.86435754852248969 ) ) ;
#93447=CARTESIAN_POINT ( 'NONE',  ( 40.36445127458296867, 23.70852965304482041, 1.583844403245330712 ) ) ;
#93448=EDGE_LOOP ( 'NONE', ( #11192, #40543, #35481, #59386 ) ) ;
#93458=CARTESIAN_POINT ( 'NONE',  ( 83.56215914360431896, 50.45755031246686428, 13.86092672225745837 ) ) ;
#93467=CARTESIAN_POINT ( 'NONE',  ( 15.07770630580378501, 30.74646525600389424, 2.839279412974139660 ) ) ;
#93469=CARTESIAN_POINT ( 'NONE',  ( 80.56456852273207403, 57.68474611512090888, 16.59351620786970116 ) ) ;
#93476=CARTESIAN_POINT ( 'NONE',  ( 79.68797162431192760, 46.35385572848484514, -12.62015847980756611 ) ) ;
#93491=VERTEX_POINT ( 'NONE', #98129 ) ;
#93496=CARTESIAN_POINT ( 'NONE',  ( 81.94645434516804983, 46.66819754834421730, -11.94275014213957675 ) ) ;
#93498=CARTESIAN_POINT ( 'NONE',  ( 82.81707834093893439, 43.43219480169420876, 7.813715050472316292 ) ) ;
#93499=CARTESIAN_POINT ( 'NONE',  ( 74.46912172204532965, 68.18838830983000321, -11.53105533885364231 ) ) ;
#93516=CARTESIAN_POINT ( 'NONE',  ( 84.13204908911602331, 50.42604040346918737, 13.71367173376235371 ) ) ;
#93518=CARTESIAN_POINT ( 'NONE',  ( 71.88630063891508826, 72.11467658586039420, 1.680795692104123162 ) ) ;
#93519=CARTESIAN_POINT ( 'NONE',  ( 75.87525401958798454, 64.72722897157592570, -14.29033900848947169 ) ) ;
#93525=CARTESIAN_POINT ( 'NONE',  ( 15.46199490364264406, 17.43085787977761925, -9.188101187500008038 ) ) ;
#93527=CARTESIAN_POINT ( 'NONE',  ( 71.88281838930642209, 59.56282477439597045, -15.74156321294393024 ) ) ;
#93528=VECTOR ( 'NONE', #45042, 1000.000000000000114 ) ;
#93530=CARTESIAN_POINT ( 'NONE',  ( 86.98157820904661719, 43.44862423325045597, 0.06000229279370256075 ) ) ;
#93535=CARTESIAN_POINT ( 'NONE',  ( 43.82855288972071151, 25.70852965304483462, 1.583844403245364907 ) ) ;
#93536=CARTESIAN_POINT ( 'NONE',  ( 86.26520568890161655, 47.67615905960597900, 10.76369269717137733 ) ) ;
#93539=CARTESIAN_POINT ( 'NONE',  ( 68.91022223105564137, 64.71151235087043574, -12.22836756590942464 ) ) ;
#93542=CARTESIAN_POINT ( 'NONE',  ( 78.98404269576303705, 49.35947893415648480, 14.50012733305994139 ) ) ;
#93547=CARTESIAN_POINT ( 'NONE',  ( 73.13555747811004437, 69.81939941050913490, 9.605153593488003239 ) ) ;
#93548=CARTESIAN_POINT ( 'NONE',  ( 42.37730965384162829, 25.26216523072498532, -2.296566073217252530E-15 ) ) ;
#93552=CARTESIAN_POINT ( 'NONE',  ( 80.96157657440146238, 44.13459223731847914, -10.82752981140125925 ) ) ;
#93554=CARTESIAN_POINT ( 'NONE',  ( 79.41525598906244454, 59.66657864593240390, 16.17364996136696931 ) ) ;
#93557=CARTESIAN_POINT ( 'NONE',  ( 88.33748333995926316, 44.07075497373335793, -2.898134731201833070 ) ) ;
#93558=CARTESIAN_POINT ( 'NONE',  ( 83.42026165063415988, 45.10053359704732401, -10.33714611788759896 ) ) ;
#93563=ORIENTED_EDGE ( 'NONE', *, *, #36832, .F. ) ;
#93564=CARTESIAN_POINT ( 'NONE',  ( 77.18698849263780914, 49.25976772916404656, -14.85955674287117922 ) ) ;
#93567=CARTESIAN_POINT ( 'NONE',  ( 78.33316717312801813, 49.42570397860901465, 14.68581309318566497 ) ) ;
#93573=CARTESIAN_POINT ( 'NONE',  ( 82.75615910393362640, 40.58425042732405785, 0.9307152221985128815 ) ) ;
#93580=CARTESIAN_POINT ( 'NONE',  ( 70.64661241052995422, 60.59469274283073048, -14.62924882204517729 ) ) ;
#93581=CARTESIAN_POINT ( 'NONE',  ( 38.84587710395076954, 34.37878583063844218, 9.188101187500006262 ) ) ;
#93584=CARTESIAN_POINT ( 'NONE',  ( 28.83231091828818649, 21.81029122506295792, 8.090169943749479842 ) ) ;
#93592=B_SPLINE_CURVE_WITH_KNOTS ( 'NONE', 3,
 ( #34838, #28243, #80503, #12064, #89126, #97676, #97192, #72888, #88617, #57641, #65251, #19185, #3955, #81013, #81993, #12566, #73861, #50539, #4448, #41442, #43441, #11077, #42921, #3480 ),
 .UNSPECIFIED., .F., .F.,
 ( 4, 2, 2, 2, 2, 2, 2, 2, 2, 2, 2, 4 ),
 ( 0.000000000000000000, 0.1249999999999925060, 0.2499999999999850120, 0.3749999999999775180, 0.4374999999999797384, 0.4999999999999820144, 0.5624999999999842348, 0.6249999999999864553, 0.6874999999999887867, 0.7499999999999910072, 0.8749999999999954481, 1.000000000000000000 ),
 .UNSPECIFIED. ) ;
#93611=CARTESIAN_POINT ( 'NONE',  ( 72.89767165371587510, 62.52605430883413362, 14.90584116256920133 ) ) ;
#93616=CARTESIAN_POINT ( 'NONE',  ( 73.85129109314340212, 68.53037146055885387, 11.40305250113367741 ) ) ;
#93625=CARTESIAN_POINT ( 'NONE',  ( 78.14015596324891533, 47.79605781560270117, 14.53813849190288465 ) ) ;
#93626=CIRCLE ( 'NONE', #24020, 16.60714546451156082 ) ;
#93627=EDGE_CURVE ( 'NONE', #57243, #45703, #77403, .T. ) ;
#93628=CARTESIAN_POINT ( 'NONE',  ( 77.89337869297911254, 54.04621959010322740, 15.98457785149147092 ) ) ;
#93632=CARTESIAN_POINT ( 'NONE',  ( 76.45858476847112684, 51.15202837745678721, 16.04606878625051536 ) ) ;
#93646=CARTESIAN_POINT ( 'NONE',  ( 88.50685567279400345, 43.87431988399859506, -0.03150979628302791324 ) ) ;
#93649=CARTESIAN_POINT ( 'NONE',  ( 71.87942950353104266, 72.15877716270880171, -3.647418342425857052 ) ) ;
#93653=CARTESIAN_POINT ( 'NONE',  ( 24.06271987006732616, 35.93396525600390845, 2.839279412974139660 ) ) ;
#93656=CARTESIAN_POINT ( 'NONE',  ( 16.72130706672765754, 10.44966523072493203, -2.296566073217252530E-15 ) ) ;
#93662=CARTESIAN_POINT ( 'NONE',  ( 74.31686216695912606, 67.90482052775791999, 11.67503013858854466 ) ) ;
#93664=CARTESIAN_POINT ( 'NONE',  ( 82.21393801928418554, 54.22668391568882384, -15.61295444237038232 ) ) ;
#93669=ORIENTED_EDGE ( 'NONE', *, *, #96063, .F. ) ;
#93670=CARTESIAN_POINT ( 'NONE',  ( 77.10732452059650655, 49.39774977627229191, 15.43680315855346663 ) ) ;
#93672=ORIENTED_EDGE ( 'NONE', *, *, #12122, .F. ) ;
#93675=CARTESIAN_POINT ( 'NONE',  ( 68.54420489956650897, 68.75802437611594087, -6.174013142999687176 ) ) ;
#93682=CONICAL_SURFACE ( 'NONE', #25688, 16.60714546451156082, 0.7853981633974407295 ) ;
#93684=CARTESIAN_POINT ( 'NONE',  ( 24.44940106416278169, 29.51421378149920116, -9.188101187500004485 ) ) ;
#93685=CARTESIAN_POINT ( 'NONE',  ( 79.74649121193665735, 44.83324031607526194, 11.42014051431522681 ) ) ;
#93687=CARTESIAN_POINT ( 'NONE',  ( 74.87331927037789114, 66.80950769484921636, -13.20416362156882961 ) ) ;
#93690=LINE ( 'NONE', #16148, #93528 ) ;
#93694=CARTESIAN_POINT ( 'NONE',  ( 67.93934924601143166, 65.44133490301047118, 10.37202260051014058 ) ) ;
#93695=CARTESIAN_POINT ( 'NONE',  ( 67.93406655831707042, 65.27944798580912789, -10.53696878470477571 ) ) ;
#93696=CARTESIAN_POINT ( 'NONE',  ( 81.47677896408023912, 55.16251862595696309, -15.92532667734195329 ) ) ;
#93698=CARTESIAN_POINT ( 'NONE',  ( 32.98506340464172837, 40.81751292744058901, -6.180339887498951690 ) ) ;
#93709=EDGE_LOOP ( 'NONE', ( #2462, #35877, #31184, #51523 ) ) ;
#93712=ORIENTED_EDGE ( 'NONE', *, *, #46504, .T. ) ;
#93713=EDGE_CURVE ( 'NONE', #42456, #48590, #95584, .T. ) ;
#93714=CARTESIAN_POINT ( 'NONE',  ( 80.43640818173928153, 44.73695621425903113, -11.66065100600888549 ) ) ;
#93716=CARTESIAN_POINT ( 'NONE',  ( 67.12382456020034738, 67.68358546754156180, 6.632048820649145249 ) ) ;
#93718=CARTESIAN_POINT ( 'NONE',  ( 81.06903993398350394, 56.12834176912372186, 16.10816894976702685 ) ) ;
#93719=CARTESIAN_POINT ( 'NONE',  ( 78.77411331422680973, 48.77619312070567759, -14.30298268893856140 ) ) ;
#93722=B_SPLINE_CURVE_WITH_KNOTS ( 'NONE', 3,
 ( #92306, #52261, #5668, #91798, #22855, #38547, #84213, #45158, #44153, #44645, #60341, #6670, #68453, #76569, #7150, #84699 ),
 .UNSPECIFIED., .F., .F.,
 ( 4, 1, 2, 2, 2, 1, 2, 2, 4 ),
 ( 0.000000000000000000, 0.1250000000000017764, 0.1875000000000028033, 0.2500000000000038303, 0.5000000000000042188, 0.6250000000000029976, 0.6875000000000041078, 0.7500000000000052180, 1.000000000000000000 ),
 .UNSPECIFIED. ) ;
#93729=CARTESIAN_POINT ( 'NONE',  ( 15.09101445147005727, 32.21091486745859811, -1.111400068045478839E-16 ) ) ;
#93735=CARTESIAN_POINT ( 'NONE',  ( 87.73298548431469612, 44.18903561216111342, 4.633618514853093728 ) ) ;
#93737=CARTESIAN_POINT ( 'NONE',  ( 82.53511752467487383, 43.65719814951889077, -8.367179187669531615 ) ) ;
#93742=B_SPLINE_CURVE_WITH_KNOTS ( 'NONE', 3,
 ( #30163, #5876, #53452, #98091, #83407, #84403, #74805, #99579, #21100, #90018, #20590, #22066, #76760, #38239, #82440, #67672 ),
 .UNSPECIFIED., .F., .F.,
 ( 4, 1, 2, 2, 2, 1, 2, 2, 4 ),
 ( 0.000000000000000000, 0.1250000000000024980, 0.1875000000000030254, 0.2500000000000035527, 0.5000000000000019984, 0.6250000000000015543, 0.6875000000000027756, 0.7500000000000038858, 1.000000000000000000 ),
 .UNSPECIFIED. ) ;
#93744=LINE ( 'NONE', #86657, #76153 ) ;
#93749=CARTESIAN_POINT ( 'NONE',  ( 86.49003203920455007, 46.12064888256469430, 8.834558565304289957 ) ) ;
#93751=CARTESIAN_POINT ( 'NONE',  ( 83.71675958367757175, 52.25485864705834160, 14.69809135895772201 ) ) ;
#93753=VERTEX_POINT ( 'NONE', #82354 ) ;
#93759=CARTESIAN_POINT ( 'NONE',  ( 73.67134723356205939, 55.40687185882725174, 16.58795594256350725 ) ) ;
#93762=CARTESIAN_POINT ( 'NONE',  ( 27.18159744850307291, 27.64441083166262203, -10.00000000000000533 ) ) ;
#93772=CARTESIAN_POINT ( 'NONE',  ( 13.35896364390118052, 31.21091486745859811, -1.111400068045478839E-16 ) ) ;
#93776=CARTESIAN_POINT ( 'NONE',  ( 26.05686017436622137, 36.81751292744056769, -6.180339887498951690 ) ) ;
#93777=CARTESIAN_POINT ( 'NONE',  ( 78.35917589421563889, 60.43990711353329459, 16.37966976287263421 ) ) ;
#93779=CARTESIAN_POINT ( 'NONE',  ( 81.07801343454443099, 56.14216831447085099, 16.10939811578601066 ) ) ;
#93781=EDGE_CURVE ( 'NONE', #86588, #75472, #75705, .T. ) ;
#93785=CARTESIAN_POINT ( 'NONE',  ( 71.83360485995035560, 66.53127591888950576, -11.52825921822993038 ) ) ;
#93788=CARTESIAN_POINT ( 'NONE',  ( 72.76037481019558584, 70.79492043649185007, -7.951079947203126608 ) ) ;
#93793=CARTESIAN_POINT ( 'NONE',  ( 79.14312167556931854, 57.64441083166269664, 0.000000000000000000 ) ) ;
#93797=CARTESIAN_POINT ( 'NONE',  ( 19.79331822069313418, 23.37878583063840665, 9.188101187500006262 ) ) ;
#93803=CARTESIAN_POINT ( 'NONE',  ( 7.739928672529463149, 22.65586893147754211, -7.433330006724137462 ) ) ;
#93805=CARTESIAN_POINT ( 'NONE',  ( 72.08846993314111273, 60.16552014367059797, -15.10313558536819123 ) ) ;
#93806=CARTESIAN_POINT ( 'NONE',  ( 88.10649794555163794, 44.30893306230427697, 2.763757158845316475 ) ) ;
#93810=CARTESIAN_POINT ( 'NONE',  ( 70.74702872844959245, 71.14896229169289654, -3.171960569837653399 ) ) ;
#93814=ORIENTED_EDGE ( 'NONE', *, *, #12143, .F. ) ;
#93817=CARTESIAN_POINT ( 'NONE',  ( 85.17596481923946783, 42.83503000546589590, -3.343520128603064023 ) ) ;
#93821=CARTESIAN_POINT ( 'NONE',  ( 80.09463153584134432, 58.13915816355183352, 16.26729705550203420 ) ) ;
#93822=CARTESIAN_POINT ( 'NONE',  ( 76.80413851785759505, 63.68367294747309870, 15.32454931363362149 ) ) ;
#93834=CARTESIAN_POINT ( 'NONE',  ( 29.64555348686941016, 32.51421378149920827, -9.188101187500004485 ) ) ;
#93839=ORIENTED_EDGE ( 'NONE', *, *, #26867, .F. ) ;
#93840=CARTESIAN_POINT ( 'NONE',  ( 74.39841895140679640, 68.21392270468032848, 11.95628786500076934 ) ) ;
#93844=CARTESIAN_POINT ( 'NONE',  ( 86.78238304187964047, 46.46655037883369488, 9.077226469069437087 ) ) ;
#93847=ORIENTED_EDGE ( 'NONE', *, *, #60933, .T. ) ;
#93855=CARTESIAN_POINT ( 'NONE',  ( 67.37618507725385086, 66.59842348624097497, 8.613459505069345212 ) ) ;
#93856=CARTESIAN_POINT ( 'NONE',  ( 75.88312381431275355, 64.11863994377948472, -14.52687401886447027 ) ) ;
#93859=ORIENTED_EDGE ( 'NONE', *, *, #38058, .T. ) ;
#93861=CARTESIAN_POINT ( 'NONE',  ( 83.54264106503212872, 41.58140769794766811, -1.200180926444211149 ) ) ;
#93864=CARTESIAN_POINT ( 'NONE',  ( 83.44578961920555571, 51.64149152686551503, -14.89211022975658949 ) ) ;
#93870=CARTESIAN_POINT ( 'NONE',  ( 74.64154962151783934, 66.95428888261444911, 13.01658699031521849 ) ) ;
#93878=CARTESIAN_POINT ( 'NONE',  ( 76.91089219145437994, 60.33774281596894440, -16.24596170531351902 ) ) ;
#93883=CARTESIAN_POINT ( 'NONE',  ( 72.19109158906036328, 71.10838548458626462, -5.953967166465967686 ) ) ;
#93885=CARTESIAN_POINT ( 'NONE',  ( 74.14312167556930433, 66.30466486950707861, 1.224646799147354045E-15 ) ) ;
#93896=CARTESIAN_POINT ( 'NONE',  ( 13.57497413706089517, 16.03677371833800436, 10.00000000000000533 ) ) ;
#93899=CARTESIAN_POINT ( 'NONE',  ( 72.28819773863641274, 72.03526396437469259, 3.423969264441562466 ) ) ;
#93904=EDGE_CURVE ( 'NONE', #51277, #37680, #48665, .T. ) ;
#93906=CARTESIAN_POINT ( 'NONE',  ( 15.30702494462977192, 17.03677371833800791, 10.00000000000000533 ) ) ;
#93907=EDGE_LOOP ( 'NONE', ( #94092, #51423, #10346, #90598 ) ) ;
#93913=CARTESIAN_POINT ( 'NONE',  ( 31.37640799630998956, 30.06628583063843507, -9.188101187500006262 ) ) ;
#93919=CARTESIAN_POINT ( 'NONE',  ( 66.30824103392255608, 68.65941448300486627, 2.357034909269177358 ) ) ;
#93921=CARTESIAN_POINT ( 'NONE',  ( 79.98829826350832661, 44.59498145193617802, 11.76229303994366582 ) ) ;
#93922=CARTESIAN_POINT ( 'NONE',  ( 4.275827057391709651, 20.65586893147753500, -7.433330006724137462 ) ) ;
#93924=CARTESIAN_POINT ( 'NONE',  ( 11.61057445305848823, 22.10171378149917487, 9.188101187500008038 ) ) ;
#93929=LINE ( 'NONE', #86347, #88267 ) ;
#93933=VERTEX_POINT ( 'NONE', #77180 ) ;
#93936=DIRECTION ( 'NONE',  ( 0.6270036013472576331, 0.3336146661356737542, -0.7039657224870771168 ) ) ;
#93943=CARTESIAN_POINT ( 'NONE',  ( 79.21141449090154651, 59.45940664425069144, -16.53580481313994710 ) ) ;
#93945=CARTESIAN_POINT ( 'NONE',  ( 80.61419007678392745, 43.44355932592966241, 9.504397039665120062 ) ) ;
#93950=CARTESIAN_POINT ( 'NONE',  ( 36.68702710410600076, 29.38052372038643867, 10.00000000000000533 ) ) ;
#93955=CARTESIAN_POINT ( 'NONE',  ( 74.41922904744917844, 66.10598066252020999, 13.04199649849176978 ) ) ;
#93958=VECTOR ( 'NONE', #86163, 1000.000000000000227 ) ;
#93961=CARTESIAN_POINT ( 'NONE',  ( 81.41038491292694346, 44.34486577817341413, 10.01861531637363001 ) ) ;
#93968=CARTESIAN_POINT ( 'NONE',  ( 18.65184876021338312, 28.95586893147755703, 7.433330006724141015 ) ) ;
#93972=ORIENTED_EDGE ( 'NONE', *, *, #90130, .F. ) ;
#93977=EDGE_CURVE ( 'NONE', #23731, #97425, #48148, .T. ) ;
#93979=CARTESIAN_POINT ( 'NONE',  ( 71.48241248555748939, 59.13619044504650901, 15.79769907036114596 ) ) ;
#93988=CARTESIAN_POINT ( 'NONE',  ( 82.33681322515650436, 40.36000428313853661, -1.174226880687108565 ) ) ;
#93993=CARTESIAN_POINT ( 'NONE',  ( 75.52860420788245222, 65.41786526994388851, 13.84462426059885232 ) ) ;
#93997=ORIENTED_EDGE ( 'NONE', *, *, #90314, .T. ) ;
#93999=CARTESIAN_POINT ( 'NONE',  ( 83.81405641344784385, 46.32409837379321260, -10.73277976188174598 ) ) ;
#94000=CARTESIAN_POINT ( 'NONE',  ( 83.14518538925494795, 42.42924448188458086, 5.540143244992730587 ) ) ;
#94010=CARTESIAN_POINT ( 'NONE',  ( 38.10324709940346111, 24.12755873383628469, -6.180339887498949025 ) ) ;
#94012=CARTESIAN_POINT ( 'NONE',  ( 68.83964938300935898, 63.80711696496913987, -12.26050211274642265 ) ) ;
#94022=EDGE_LOOP ( 'NONE', ( #98070, #36712, #87003, #58256 ) ) ;
#94028=CARTESIAN_POINT ( 'NONE',  ( 11.93836421708519779, 28.93396525600389069, 2.839279412974139660 ) ) ;
#94034=CARTESIAN_POINT ( 'NONE',  ( 30.06092144891428930, 17.75978393459166682, -1.583844403245396437 ) ) ;
#94038=CARTESIAN_POINT ( 'NONE',  ( 85.88548993935545184, 47.52640722116844785, 10.83458574080284187 ) ) ;
#94039=ORIENTED_EDGE ( 'NONE', *, *, #54563, .T. ) ;
#94045=CARTESIAN_POINT ( 'NONE',  ( 84.15543808568007478, 42.98865946211766698, 6.707866528308588094 ) ) ;
#94048=CARTESIAN_POINT ( 'NONE',  ( 74.96538493238443834, 53.10769796979874258, -16.50489419803275837 ) ) ;
#94050=ORIENTED_EDGE ( 'NONE', *, *, #75362, .T. ) ;
#94051=EDGE_CURVE ( 'NONE', #45703, #52319, #91673, .T. ) ;
#94053=CARTESIAN_POINT ( 'NONE',  ( 36.57375671714491006, 36.51421378149921537, -9.188101187500004485 ) ) ;
#94054=CARTESIAN_POINT ( 'NONE',  ( 73.06817150023823615, 70.46971108366265923, -8.031831301699734027 ) ) ;
#94060=CARTESIAN_POINT ( 'NONE',  ( 86.40901846424877419, 47.04753287972406639, -10.02754009819726733 ) ) ;
#94063=CARTESIAN_POINT ( 'NONE',  ( 88.05624235485146301, 44.55787864911079765, -5.145732200269208967 ) ) ;
#94066=CARTESIAN_POINT ( 'NONE',  ( 80.41490723808537666, 44.37095382489257389, 11.34173964343496621 ) ) ;
#94072=DIRECTION ( 'NONE',  ( 0.5000000000000014433, -0.8660254037844378194, 0.000000000000000000 ) ) ;
#94074=CARTESIAN_POINT ( 'NONE',  ( 74.88642528495033446, 58.21203573159304767, 15.94079607396144560 ) ) ;
#94075=CARTESIAN_POINT ( 'NONE',  ( 78.71449943708836372, 50.90750488496149018, 15.15446692355688896 ) ) ;
#94081=LINE ( 'NONE', #55514, #61215 ) ;
#94083=CARTESIAN_POINT ( 'NONE',  ( 76.97203077703174756, 62.91777711518242455, -15.25263661455074171 ) ) ;
#94087=CARTESIAN_POINT ( 'NONE',  ( 70.62612002322232740, 60.62352525996839603, -14.61234695924068205 ) ) ;
#94088=CARTESIAN_POINT ( 'NONE',  ( 37.50955192761952617, 39.84336893147759184, -7.433330006724137462 ) ) ;
#94089=ADVANCED_FACE ( 'NONE', ( #22235 ), #51633, .T. ) ;
#94092=ORIENTED_EDGE ( 'NONE', *, *, #31161, .F. ) ;
#94097=CARTESIAN_POINT ( 'NONE',  ( 73.72578271399891037, 68.22897723188711439, 11.11049049714292991 ) ) ;
#94110=CARTESIAN_POINT ( 'NONE',  ( 86.78549426258132371, 45.83013854792883279, 8.849882187839877901 ) ) ;
#94117=CARTESIAN_POINT ( 'NONE',  ( 73.83053071202353124, 66.06161260281930936, 13.30051256284848904 ) ) ;
#94119=CARTESIAN_POINT ( 'NONE',  ( 87.88902802526534686, 43.91876200309240375, 0.4180276961671919311 ) ) ;
#94122=CARTESIAN_POINT ( 'NONE',  ( 73.86986929274216607, 68.54753403896816621, 11.39714278534122549 ) ) ;
#94123=CARTESIAN_POINT ( 'NONE',  ( 74.33743881423829691, 68.50532701121755963, 11.17712573888744920 ) ) ;
#94124=CARTESIAN_POINT ( 'NONE',  ( 70.52490725396940263, 71.27080261044798704, -1.937046345266181024 ) ) ;
#94131=CARTESIAN_POINT ( 'NONE',  ( 77.84067285015417781, 53.77961970061534203, 15.94779701496784696 ) ) ;
#94133=CARTESIAN_POINT ( 'NONE',  ( 67.00432206419098691, 66.89247057574091571, 8.809205559600117752 ) ) ;
#94134=CARTESIAN_POINT ( 'NONE',  ( 75.87085204095464519, 51.53938293317272468, 15.71483405503507136 ) ) ;
#94141=DIRECTION ( 'NONE',  ( -0.3715724127386920705, 0.6435822975543701308, -0.6691306063588670083 ) ) ;
#94142=ADVANCED_FACE ( 'NONE', ( #87112 ), #86599, .T. ) ;
#94144=EDGE_CURVE ( 'NONE', #93491, #51674, #85688, .T. ) ;
#94148=CARTESIAN_POINT ( 'NONE',  ( 88.34978748912247681, 44.19151614600375666, -0.08427336824597120302 ) ) ;
#94150=CARTESIAN_POINT ( 'NONE',  ( 79.36263291408793918, 45.67866562566761957, -12.88899626193393999 ) ) ;
#94151=CARTESIAN_POINT ( 'NONE',  ( 77.63584588586775226, 49.30200881430058502, 15.29451607107652222 ) ) ;
#94153=CARTESIAN_POINT ( 'NONE',  ( 22.53213034355507460, 33.98502408145593279, -5.678558825948271327 ) ) ;
#94156=CARTESIAN_POINT ( 'NONE',  ( 6.742211794378569323, 25.93396525600388003, 2.839279412974139660 ) ) ;
#94158=CARTESIAN_POINT ( 'NONE',  ( 80.87517248313827167, 58.64441083166272506, 0.000000000000000000 ) ) ;
#94161=CARTESIAN_POINT ( 'NONE',  ( 69.47037063557095848, 62.62442318441491551, -13.85991542342858018 ) ) ;
#94164=CARTESIAN_POINT ( 'NONE',  ( 77.84895608869516082, 55.91079568154652435, -16.15415909428238095 ) ) ;
#94165=CARTESIAN_POINT ( 'NONE',  ( 87.60351575088976972, 45.13338919493600798, -6.137684345434423427 ) ) ;
#94167=CARTESIAN_POINT ( 'NONE',  ( 82.66777534753497036, 40.88273136530058594, 3.288167606880421090 ) ) ;
#94170=CARTESIAN_POINT ( 'NONE',  ( 77.45223888989086447, 49.57236342607031787, 14.91341569047779281 ) ) ;
#94176=CARTESIAN_POINT ( 'NONE',  ( 69.72007715475741918, 68.87520295995811637, -7.276862800964089217 ) ) ;
#94177=VERTEX_POINT ( 'NONE', #62722 ) ;
#94179=VERTEX_POINT ( 'NONE', #39912 ) ;
#94180=CARTESIAN_POINT ( 'NONE',  ( 79.46801687855551677, 46.39187830138592972, -12.72948678403309053 ) ) ;
#94184=CARTESIAN_POINT ( 'NONE',  ( 20.10065364775352847, 33.64646525600390703, -2.839279412974133887 ) ) ;
#94185=CARTESIAN_POINT ( 'NONE',  ( 79.74133107861359804, 44.86189080207443425, 11.44794314671259627 ) ) ;
#94187=CARTESIAN_POINT ( 'NONE',  ( 75.32434183498538971, 66.62165581190093633, -13.06803771652694834 ) ) ;
#94188=CARTESIAN_POINT ( 'NONE',  ( 78.66149435155034553, 49.46989482002797445, -14.61922007752083452 ) ) ;
#94194=CARTESIAN_POINT ( 'NONE',  ( 67.80686942989439103, 65.67079667550257227, 10.79604664877636289 ) ) ;
#94195=CARTESIAN_POINT ( 'NONE',  ( 67.95186835949662907, 65.47617292293909941, -10.34303067525367226 ) ) ;
#94196=CARTESIAN_POINT ( 'NONE',  ( 81.76515281898197429, 55.59664093367394599, -15.96652640277710766 ) ) ;
#94198=CARTESIAN_POINT ( 'NONE',  ( 41.38738224522862907, 24.86426979415093186, -3.090169943749474069 ) ) ;
#94202=CARTESIAN_POINT ( 'NONE',  ( 79.04010335995445757, 59.81086823702358402, 16.49488376190979366 ) ) ;
#94206=CARTESIAN_POINT ( 'NONE',  ( 78.17919853682799669, 61.76234676664309120, -16.10619035535653509 ) ) ;
#94208=ORIENTED_EDGE ( 'NONE', *, *, #64950, .T. ) ;
#94211=CARTESIAN_POINT ( 'NONE',  ( 80.35890605665858288, 44.73641450380378615, -11.69935222326590640 ) ) ;
#94212=CARTESIAN_POINT ( 'NONE',  ( 67.16327201103491973, 67.73731889023999031, 6.573435314091262249 ) ) ;
#94215=CARTESIAN_POINT ( 'NONE',  ( 37.16144446923997435, 23.58380873178789727, 6.180339887498953466 ) ) ;
#94216=CARTESIAN_POINT ( 'NONE',  ( 84.05270344386845238, 47.46752220604140859, -11.66933861446510079 ) ) ;
#94218=ORIENTED_EDGE ( 'NONE', *, *, #14534, .F. ) ;
#94220=ORIENTED_EDGE ( 'NONE', *, *, #44208, .F. ) ;
#94224=VERTEX_POINT ( 'NONE', #71862 ) ;
#94226=CARTESIAN_POINT ( 'NONE',  ( 76.17858836466767514, 64.76715759548049789, -14.35676355172211238 ) ) ;
#94231=CARTESIAN_POINT ( 'NONE',  ( 85.75565660721923678, 43.84343610033825200, -5.420381390687177614 ) ) ;
#94237=DIRECTION ( 'NONE',  ( 0.3782958374750613473, 0.000000000000000000, -0.9256847516023162248 ) ) ;
#94241=CARTESIAN_POINT ( 'NONE',  ( 85.92630256486899043, 44.97195868260131846, 7.553312411822113326 ) ) ;
#94243=CARTESIAN_POINT ( 'NONE',  ( 83.67285453873573431, 52.00132685099405450, 14.98825055830738329 ) ) ;
#94249=CARTESIAN_POINT ( 'NONE',  ( 74.87853038332181654, 63.73010615337872053, -14.43890213384147003 ) ) ;
#94251=FACE_BOUND ( 'NONE', #2228, .T. ) ;
#94252=CARTESIAN_POINT ( 'NONE',  ( 69.81243019392553606, 62.22010195957141576, -13.63492759933605392 ) ) ;
#94254=CARTESIAN_POINT ( 'NONE',  ( 22.35729902920393997, 37.00034080476290654, -1.878358725466461243E-16 ) ) ;
#94260=CARTESIAN_POINT ( 'NONE',  ( 81.67192807023319290, 46.29478322961348624, 11.76198625675847431 ) ) ;
#94262=EDGE_CURVE ( 'NONE', #7411, #26733, #55468, .T. ) ;
#94267=CIRCLE ( 'NONE', #97520, 16.60714546451156082 ) ;
#94269=CARTESIAN_POINT ( 'NONE',  ( 29.53625146412516500, 35.79103043416551344, 8.090169943749478065 ) ) ;
#94272=CARTESIAN_POINT ( 'NONE',  ( 72.87667924365860017, 65.01085463311059698, 13.62852699864587969 ) ) ;
#94273=CARTESIAN_POINT ( 'NONE',  ( 81.42628347097989661, 41.97763379937408956, 7.709395309255075546 ) ) ;
#94278=CARTESIAN_POINT ( 'NONE',  ( 68.69958519936569985, 66.83058884119587617, -9.320282762443202529 ) ) ;
#94285=CARTESIAN_POINT ( 'NONE',  ( 67.35308227982150697, 66.38192671655097854, -8.894446999883845351 ) ) ;
#94287=VECTOR ( 'NONE', #26921, 1000.000000000000114 ) ;
#94290=B_SPLINE_CURVE_WITH_KNOTS ( 'NONE', 3,
 ( #53607, #45011, #76441, #37408, #52115, #6533, #36918, #83566, #30324, #83062, #98752, #91158, #13635, #61212, #84566, #75956, #15104, #35920, #97749, #59196, #28317, #90172, #5529, #20745, #51631, #13146, #98245, #44509, #59714, #29332, #60198, #21724, #52608, #87092, #39894, #54099, #70828, #25216, #86093, #38909, #23702, #9543, #77936, #17629, #93662, #85055 ),
 .UNSPECIFIED., .F., .F.,
 ( 4, 1, 1, 1, 2, 2, 1, 1, 1, 2, 2, 1, 1, 2, 2, 1, 1, 2, 2, 1, 1, 2, 2, 1, 2, 2, 1, 2, 2, 4 ),
 ( 0.000000000000000000, 0.06249999999998047395, 0.09374999999997075950, 0.1093749999999649170, 0.1171874999999624883, 0.1249999999999600597, 0.1874999999999578670, 0.2187499999999581446, 0.2343749999999596989, 0.2421874999999613365, 0.2499999999999629741, 0.3124999999999686362, 0.3437499999999719669, 0.3593749999999722444, 0.3749999999999725220, 0.4374999999999828471, 0.4687499999999875100, 0.4843749999999880096, 0.4999999999999884537, 0.5624999999999913403, 0.5937499999999945599, 0.6093749999999962252, 0.6249999999999978906, 0.6875000000000027756, 0.7187500000000056621, 0.7500000000000085487, 0.8125000000000102141, 0.8437500000000092149, 0.8750000000000082157, 1.000000000000000000 ),
 .UNSPECIFIED. ) ;
#94293=CARTESIAN_POINT ( 'NONE',  ( 27.77157046966360809, 18.96004757982091249, -5.678558825948276656 ) ) ;
#94298=CARTESIAN_POINT ( 'NONE',  ( 34.69457829350510281, 43.52903772873360566, -1.583844403245329602 ) ) ;
#94299=CARTESIAN_POINT ( 'NONE',  ( 4.795442299662375341, 20.95586893147752861, 7.433330006724141015 ) ) ;
#94301=CARTESIAN_POINT ( 'NONE',  ( 74.84764555390079011, 59.32158413457844404, -15.77185916182937575 ) ) ;
#94302=CARTESIAN_POINT ( 'NONE',  ( 71.72790558683757922, 72.47596629505412125, -1.350878852920679662 ) ) ;
#94307=CARTESIAN_POINT ( 'NONE',  ( 85.47555641224485612, 49.06903847834369969, 12.34201857654865542 ) ) ;
#94316=CARTESIAN_POINT ( 'NONE',  ( 72.75640829328646930, 57.27960352001080224, -15.87147226852406234 ) ) ;
#94322=ORIENTED_EDGE ( 'NONE', *, *, #64364, .T. ) ;
#94325=CARTESIAN_POINT ( 'NONE',  ( 22.55378097864968012, 33.99752408145592852, 5.678558825948277544 ) ) ;
#94327=CARTESIAN_POINT ( 'NONE',  ( 78.32185800947360121, 47.85121949867834701, -14.51427106730122141 ) ) ;
#94330=CARTESIAN_POINT ( 'NONE',  ( 73.86986929274216607, 68.54753403896816621, 10.89714278534122549 ) ) ;
#94340=CARTESIAN_POINT ( 'NONE',  ( 68.23957855939767114, 69.39062747421131405, -4.093039667954597505 ) ) ;
#94345=CIRCLE ( 'NONE', #74882, 10.00000000000001066 ) ;
#94346=CARTESIAN_POINT ( 'NONE',  ( 82.96854302488638666, 41.23096503478176089, -0.6813192392769399364 ) ) ;
#94347=CARTESIAN_POINT ( 'NONE',  ( 81.82036482989325066, 42.35048943672428834, -7.944650131338358179 ) ) ;
#94348=CARTESIAN_POINT ( 'NONE',  ( 67.18318263371854471, 66.87162863476784480, 8.978259895924134426 ) ) ;
#94349=CARTESIAN_POINT ( 'NONE',  ( 71.00065756275667184, 65.38050944624951910, -12.04497808108590817 ) ) ;
#94354=CARTESIAN_POINT ( 'NONE',  ( 69.42144788871625849, 62.89730317705431872, 13.10748580973936939 ) ) ;
#94355=AXIS2_PLACEMENT_3D ( 'NONE', #62043, #32163, #33172 ) ;
#94357=EDGE_CURVE ( 'NONE', #12913, #75751, #76818, .T. ) ;
#94359=CARTESIAN_POINT ( 'NONE',  ( 87.62133583293774564, 45.31115884160843876, -7.293173845241961217 ) ) ;
#94362=CARTESIAN_POINT ( 'NONE',  ( 80.39015929397758953, 57.47250276623566378, -16.58917374605577777 ) ) ;
#94365=CARTESIAN_POINT ( 'NONE',  ( 74.63372323989780455, 66.93453420673688470, 13.02704161780705938 ) ) ;
#94372=CARTESIAN_POINT ( 'NONE',  ( 85.37572018521500183, 48.32884972269767587, -12.27680401939018751 ) ) ;
#94373=CARTESIAN_POINT ( 'NONE',  ( 87.90135287304421752, 44.47855560518080154, -3.950668869199154720 ) ) ;
#94374=ADVANCED_FACE ( 'NONE', ( #14533 ), #38304, .T. ) ;
#94382=CARTESIAN_POINT ( 'NONE',  ( 84.27862564753039010, 50.65054004415126343, -13.76907720482496700 ) ) ;
#94384=EDGE_CURVE ( 'NONE', #64537, #80050, #22626, .T. ) ;
#94386=CARTESIAN_POINT ( 'NONE',  ( 71.86256228778262312, 72.60615528678948749, -0.5650332253008888417 ) ) ;
#94388=CARTESIAN_POINT ( 'NONE',  ( 13.42817895373461390, 26.49103043416548076, -8.090169943749479842 ) ) ;
#94391=CARTESIAN_POINT ( 'NONE',  ( 83.42542119994749328, 51.64995580955419996, -14.90072893730333270 ) ) ;
#94395=CARTESIAN_POINT ( 'NONE',  ( 3.720166145283430925, 25.08080186712590276, -3.090169943749475845 ) ) ;
#94404=CARTESIAN_POINT ( 'NONE',  ( 34.45502471548058310, 41.93396525600392977, 2.839279412974139660 ) ) ;
#94408=CARTESIAN_POINT ( 'NONE',  ( 35.22599450741489591, 22.19860640527294393, 2.839279412974134775 ) ) ;
#94411=CARTESIAN_POINT ( 'NONE',  ( 65.90510710696692342, 68.96474564273314911, 2.468420138682963394 ) ) ;
#94417=CARTESIAN_POINT ( 'NONE',  ( 15.62556418158687244, 11.94754757982088123, 5.678558825948272215 ) ) ;
#94424=CARTESIAN_POINT ( 'NONE',  ( 66.06796213254585837, 68.60782010546279253, 4.332213670276926720 ) ) ;
#94427=EDGE_LOOP ( 'NONE', ( #73108, #62247, #3226 ) ) ;
#94428=ORIENTED_EDGE ( 'NONE', *, *, #92983, .F. ) ;
#94430=VECTOR ( 'NONE', #63593, 1000.000000000000227 ) ;
#94431=CARTESIAN_POINT ( 'NONE',  ( 86.27668453731669729, 47.22199995466520761, 10.82669603042141304 ) ) ;
#94436=CARTESIAN_POINT ( 'NONE',  ( 79.48002332306521112, 59.20369081482913742, -16.22437187204984710 ) ) ;
#94438=CARTESIAN_POINT ( 'NONE',  ( 80.74974841597983755, 43.27611110042440146, 10.01619596034499260 ) ) ;
#94441=CARTESIAN_POINT ( 'NONE',  ( 69.46659797204442555, 64.04447920839335495, -12.97926778662067093 ) ) ;
#94445=ORIENTED_EDGE ( 'NONE', *, *, #87882, .T. ) ;
#94450=CARTESIAN_POINT ( 'NONE',  ( 73.61601042510409343, 62.36123447726389202, 14.66634685749964184 ) ) ;
#94454=CARTESIAN_POINT ( 'NONE',  ( 83.06160119771897143, 48.50967694913268247, 12.83647970848521425 ) ) ;
#94463=CARTESIAN_POINT ( 'NONE',  ( 16.80975711337266176, 31.74646525600390135, 2.839279412974139660 ) ) ;
#94482=CARTESIAN_POINT ( 'NONE',  ( 82.49906311289566929, 40.47457387647443738, -1.406446948987077006 ) ) ;
#94486=CARTESIAN_POINT ( 'NONE',  ( 75.58778754766929353, 65.52267137415682896, 13.80857608998921116 ) ) ;
#94487=VECTOR ( 'NONE', #80598, 1000.000000000000114 ) ;
#94489=ORIENTED_EDGE ( 'NONE', *, *, #60564, .F. ) ;
#94491=CARTESIAN_POINT ( 'NONE',  ( 87.86298961015023679, 44.89260222163544256, 6.207647304897665919 ) ) ;
#94493=CARTESIAN_POINT ( 'NONE',  ( 79.17490018547003672, 47.23354819373627578, -13.38294009737406043 ) ) ;
#94494=CARTESIAN_POINT ( 'NONE',  ( 85.14296776498849795, 45.57912900884821283, 9.070685772083578513 ) ) ;
#94496=LINE ( 'NONE', #1778, #13975 ) ;
#94498=CARTESIAN_POINT ( 'NONE',  ( 74.19835002362358978, 68.51042020854130499, -11.60174470505228150 ) ) ;
#94505=CARTESIAN_POINT ( 'NONE',  ( 82.15438889958460322, 43.42002399553825853, 8.329187321006108036 ) ) ;
#94506=ADVANCED_FACE ( 'NONE', ( #75349 ), #19267, .T. ) ;
#94510=CARTESIAN_POINT ( 'NONE',  ( 29.49842587079848855, 40.52903772873359856, -1.583844403245363575 ) ) ;
#94515=ADVANCED_FACE ( 'NONE', ( #85471 ), #96123, .T. ) ;
#94517=CARTESIAN_POINT ( 'NONE',  ( 73.62250635243425734, 69.55784274833358438, 10.23584637956793308 ) ) ;
#94524=CARTESIAN_POINT ( 'NONE',  ( 18.97660828663255117, 29.14336893147755703, 7.433330006724141015 ) ) ;
#94525=CARTESIAN_POINT ( 'NONE',  ( 74.03931459348295618, 60.54867073305699421, -15.82834853898143912 ) ) ;
#94534=CARTESIAN_POINT ( 'NONE',  ( 85.86469242221521370, 47.48580584220093925, 10.80557080686977933 ) ) ;
#94539=CARTESIAN_POINT ( 'NONE',  ( 71.96852905813886991, 72.61068693531510121, 1.394764389614196354 ) ) ;
#94540=CARTESIAN_POINT ( 'NONE',  ( 85.86494630647001713, 46.28363073764573699, 10.08731117762910046 ) ) ;
#94541=CARTESIAN_POINT ( 'NONE',  ( 83.91613728284298190, 51.81858503665881699, -14.46596598907902909 ) ) ;
#94546=CARTESIAN_POINT ( 'NONE',  ( 39.98734656443052415, 28.80170272979929535, 7.433330006724137462 ) ) ;
#94554=CARTESIAN_POINT ( 'NONE',  ( 86.52735458038128513, 47.21746853903349006, -10.13408089075210050 ) ) ;
#94555=CARTESIAN_POINT ( 'NONE',  ( 77.32817876982272765, 63.13942984521013813, 15.61058464551962111 ) ) ;
#94556=CARTESIAN_POINT ( 'NONE',  ( 87.02903784321956948, 44.46201794666647800, -6.348227258070155088 ) ) ;
#94557=DIRECTION ( 'NONE',  ( -0.4924038765061016787, 0.8528685319524424990, -0.1736481776669404342 ) ) ;
#94558=CARTESIAN_POINT ( 'NONE',  ( 81.82083194927301406, 45.30039977485242275, -11.45098190420846862 ) ) ;
#94559=CARTESIAN_POINT ( 'NONE',  ( 84.83269492062768791, 49.93259165162010760, -13.18831682406798400 ) ) ;
#94565=CARTESIAN_POINT ( 'NONE',  ( 77.38344707993300631, 49.10671604804453239, -15.27628165703247198 ) ) ;
#94568=CARTESIAN_POINT ( 'NONE',  ( 88.31205481598105678, 44.17345802399140098, -0.1934329303017474633 ) ) ;
#94576=CARTESIAN_POINT ( 'NONE',  ( 79.11275361910446691, 46.11146926033848814, 13.27945046499837112 ) ) ;
#94585=CARTESIAN_POINT ( 'NONE',  ( 20.61848683307935914, 34.83705186507754803, 3.090169943749475401 ) ) ;
#94586=ORIENTED_EDGE ( 'NONE', *, *, #98906, .T. ) ;
#94591=CARTESIAN_POINT ( 'NONE',  ( 71.50240432004942193, 72.40933122983058468, 5.654570818603106787E-06 ) ) ;
#94602=VERTEX_POINT ( 'NONE', #13909 ) ;
#94620=CARTESIAN_POINT ( 'NONE',  ( 67.77025216284080500, 69.60538277264423357, 1.930950847018320982 ) ) ;
#94625=CARTESIAN_POINT ( 'NONE',  ( 88.08080417645612670, 44.69611168586961014, -4.296359715587334094 ) ) ;
#94627=CARTESIAN_POINT ( 'NONE',  ( 78.51571825418398021, 47.42707193263058230, 14.24622496894903634 ) ) ;
#94628=CARTESIAN_POINT ( 'NONE',  ( 77.56166335470948070, 52.46047131205113345, 15.73022103520029980 ) ) ;
#94630=CARTESIAN_POINT ( 'NONE',  ( 78.27096424623380244, 61.69037436829221122, 15.77147391507759799 ) ) ;
#94637=CARTESIAN_POINT ( 'NONE',  ( 72.95830788359974406, 56.77128196665827176, -15.96545419981962333 ) ) ;
#94640=CARTESIAN_POINT ( 'NONE',  ( 73.63798764345266079, 69.67310094948797428, 10.11710443556177275 ) ) ;
#94646=CARTESIAN_POINT ( 'NONE',  ( 88.54283264841694745, 43.89585489789003248, -0.1669414168386815500 ) ) ;
#94652=CARTESIAN_POINT ( 'NONE',  ( 25.24689923506580769, 37.68290643055188838, 3.479690158560446702E-15 ) ) ;
#94653=CARTESIAN_POINT ( 'NONE',  ( 81.66039725905243074, 47.34856834791166591, 13.14074354680314372 ) ) ;
#94654=CARTESIAN_POINT ( 'NONE',  ( 79.06313471345563926, 47.89260127994747762, -13.77394454897267728 ) ) ;
#94655=ORIENTED_EDGE ( 'NONE', *, *, #58612, .F. ) ;
#94656=CARTESIAN_POINT ( 'NONE',  ( 21.91745948943428601, 13.44966523072494269, -2.296566073217252530E-15 ) ) ;
#94658=CARTESIAN_POINT ( 'NONE',  ( 82.65022647498227570, 54.02725688527395675, -15.50106321898839923 ) ) ;
#94660=CARTESIAN_POINT ( 'NONE',  ( 69.73646959995419081, 63.15839211331632441, -13.63664433904350481 ) ) ;
#94667=CARTESIAN_POINT ( 'NONE',  ( 84.13622801036203214, 43.12737274679144406, 5.841038043053070616 ) ) ;
#94672=CARTESIAN_POINT ( 'NONE',  ( 68.77965372826733415, 68.78927433938119407, -6.398530390328347472 ) ) ;
#94675=EDGE_LOOP ( 'NONE', ( #10710, #8930, #85358, #68112 ) ) ;
#94676=CARTESIAN_POINT ( 'NONE',  ( 72.35414581608256412, 71.76618622507949397, 5.628474724962954312 ) ) ;
#94681=CARTESIAN_POINT ( 'NONE',  ( 23.84800118292001159, 31.95586893147756058, 7.433330006724141015 ) ) ;
#94682=CARTESIAN_POINT ( 'NONE',  ( 74.67000616351417364, 66.81477949400927230, -13.12245706047551508 ) ) ;
#94683=CARTESIAN_POINT ( 'NONE',  ( 78.96527083864563679, 49.39199274328564115, -14.51843862548532904 ) ) ;
#94684=CYLINDRICAL_SURFACE ( 'NONE', #96723, 16.60714546451156792 ) ;
#94686=EDGE_LOOP ( 'NONE', ( #47450, #32744, #93712, #29978 ) ) ;
#94689=CARTESIAN_POINT ( 'NONE',  ( 67.76997328886733385, 65.59689072950045841, 10.11017479253558626 ) ) ;
#94691=CARTESIAN_POINT ( 'NONE',  ( 81.75866452494919656, 55.62065470240971621, -15.97060719759759628 ) ) ;
#94695=CARTESIAN_POINT ( 'NONE',  ( 72.96253058994859941, 62.41371533620014134, -14.96910879617931656 ) ) ;
#94705=CARTESIAN_POINT ( 'NONE',  ( 80.11135166060731194, 44.61021142565198261, -11.71391964968389132 ) ) ;
#94706=CARTESIAN_POINT ( 'NONE',  ( 80.87517248313827167, 58.64441083166272506, 0.000000000000000000 ) ) ;
#94708=CARTESIAN_POINT ( 'NONE',  ( 79.89582544085288873, 48.49195324432764664, -13.86380691270739440 ) ) ;
#94715=B_SPLINE_SURFACE_WITH_KNOTS ( 'NONE', 3, 1, ( 
 ( #64306, #64813 ),
 ( #95259, #65788 ),
 ( #95761, #26313 ),
 ( #49597, #80552 ),
 ( #48616, #11128 ),
 ( #25825, #79555 ),
 ( #42482, #73416 ),
 ( #96747, #33928 ),
 ( #96245, #41999 ),
 ( #17195, #57689 ),
 ( #26806, #72935 ),
 ( #58196, #71921 ),
 ( #94737, #88667 ),
 ( #19234, #18217 ),
 ( #48098, #79039 ),
 ( #10110, #40975 ),
 ( #2523, #33405 ),
 ( #56701, #87682 ),
 ( #80046, #82045 ),
 ( #37380, #20211 ),
 ( #75411, #52581 ),
 ( #36889, #51599 ),
 ( #12110, #27805 ),
 ( #82553, #13118 ),
 ( #97720, #43485 ),
 ( #58678, #74429 ),
 ( #4499, #35893 ),
 ( #66795, #36384 ),
 ( #28288, #6503 ),
 ( #67288, #98215 ),
 ( #28799, #59679 ) ),
 .UNSPECIFIED., .F., .F., .F.,
 ( 4, 3, 3, 3, 3, 3, 3, 3, 3, 3, 4 ),
 ( 2, 2 ),
 ( 0.000000000000000000, 0.1333490885032345696, 0.3007194338854333737, 0.4699862290245237495, 0.5844252810809289489, 0.6686540514502742338, 0.7354980260655397117, 0.8028463152565420424, 0.8633854507756993923, 0.9437142632667149256, 1.000000000000000000 ),
 ( 0.000000000000000000, 1.000000000000000000 ),
 .UNSPECIFIED. ) ;
#94716=FACE_OUTER_BOUND ( 'NONE', #67774, .T. ) ;
#94721=CARTESIAN_POINT ( 'NONE',  ( 22.61461015039527922, 36.55466486950700755, 7.012934429366973338E-14 ) ) ;
#94722=CARTESIAN_POINT ( 'NONE',  ( 70.00660573506930007, 69.36680803441663556, -6.749214270069086474 ) ) ;
#94723=CARTESIAN_POINT ( 'NONE',  ( 88.08546139208640113, 44.41188104239807188, 4.690966480777962744 ) ) ;
#94725=CARTESIAN_POINT ( 'NONE',  ( 81.23259876005273838, 43.67848304645094970, -9.361027865139382342 ) ) ;
#94726=CARTESIAN_POINT ( 'NONE',  ( 80.33508072308801218, 44.92307697338561212, 11.19555900290710326 ) ) ;
#94728=CARTESIAN_POINT ( 'NONE',  ( 38.08139550823666042, 22.39040679176985904, -6.890680421881970419E-14 ) ) ;
#94735=CARTESIAN_POINT ( 'NONE',  ( 82.15463706511577868, 40.84277258114416043, 1.595534587534165549 ) ) ;
#94737=CARTESIAN_POINT ( 'NONE',  ( 78.08661669030729513, 61.77574478846858597, 16.09152831843414688 ) ) ;
#94746=CARTESIAN_POINT ( 'NONE',  ( 26.99866280452971878, 37.36126292948897287, 6.180339887498949913 ) ) ;
#94755=CARTESIAN_POINT ( 'NONE',  ( 82.13016512221932430, 47.61428595633086758, 12.58464463784943987 ) ) ;
#94759=CARTESIAN_POINT ( 'NONE',  ( 82.09831584080588129, 41.83606685967262706, 5.488894909882152895 ) ) ;
#94762=CARTESIAN_POINT ( 'NONE',  ( 32.55392312662736032, 19.76426979415091267, 3.090169943749476733 ) ) ;
#94763=CARTESIAN_POINT ( 'NONE',  ( 38.89349527680885643, 24.58380873178789727, 6.180339887498953466 ) ) ;
#94768=CARTESIAN_POINT ( 'NONE',  ( 81.17617732377340189, 56.17678352023477117, 16.10626194070232131 ) ) ;
#94770=CARTESIAN_POINT ( 'NONE',  ( 84.91076779388347973, 49.09221707277423974, 13.05056290568177779 ) ) ;
#94771=CARTESIAN_POINT ( 'NONE',  ( 83.67285453873573431, 52.00132685099406160, 14.98825055830738151 ) ) ;
#94772=AXIS2_PLACEMENT_3D ( 'NONE', #61613, #77843, #92567 ) ;
#94775=CARTESIAN_POINT ( 'NONE',  ( 74.65546376004118656, 65.88439924513853896, -13.23886940964006520 ) ) ;
#94785=CARTESIAN_POINT ( 'NONE',  ( 66.27113406421898389, 69.38871762109552321, 0.1120879072176016594 ) ) ;
#94789=CARTESIAN_POINT ( 'NONE',  ( 25.52954022263672940, 23.24335787977764411, -9.188101187500008038 ) ) ;
#94794=CARTESIAN_POINT ( 'NONE',  ( 8.860943796042899834, 20.51421378149916919, -9.188101187500004485 ) ) ;
#94797=CARTESIAN_POINT ( 'NONE',  ( 87.80398682648640829, 44.12684940286039392, 2.720675826359043370 ) ) ;
#94799=CARTESIAN_POINT ( 'NONE',  ( 72.22232072300009520, 71.11120588350317462, -5.989663598951492141 ) ) ;
#94801=CARTESIAN_POINT ( 'NONE',  ( 85.56434759925559774, 49.01624254635854783, 12.26054419347457092 ) ) ;
#94804=ORIENTED_EDGE ( 'NONE', *, *, #21934, .F. ) ;
#94808=ORIENTED_EDGE ( 'NONE', *, *, #25109, .F. ) ;
#94809=CARTESIAN_POINT ( 'NONE',  ( 45.60499120716188060, 26.73415679381826138, -6.890680421881970419E-14 ) ) ;
#94811=CARTESIAN_POINT ( 'NONE',  ( 72.98918101599892339, 57.62492086428549243, -16.32278002199753075 ) ) ;
#94816=VECTOR ( 'NONE', #638, 1000.000000000000000 ) ;
#94820=CARTESIAN_POINT ( 'NONE',  ( 26.18145187173165311, 30.51421378149920116, -9.188101187500004485 ) ) ;
#94822=CARTESIAN_POINT ( 'NONE',  ( 67.73131330550826590, 69.99787020178199271, -2.592847403169493692 ) ) ;
#94824=CARTESIAN_POINT ( 'NONE',  ( 74.39896838111268096, 68.39356553035000275, 11.80479640254016083 ) ) ;
#94827=AXIS2_PLACEMENT_3D ( 'NONE', #39980, #55184, #24308 ) ;
#94829=ORIENTED_EDGE ( 'NONE', *, *, #1510, .F. ) ;
#94830=CARTESIAN_POINT ( 'NONE',  ( 76.81910699536521747, 57.83062468730825856, -16.12375912510302101 ) ) ;
#94831=CARTESIAN_POINT ( 'NONE',  ( 84.65917736194083432, 42.99992238498651886, -4.794713744061861682 ) ) ;
#94841=CARTESIAN_POINT ( 'NONE',  ( 83.33466500116428222, 41.42342953991349219, -0.2387503505471941512 ) ) ;
#94842=CARTESIAN_POINT ( 'NONE',  ( 85.82824564990275462, 42.91066052166247147, -4.076138561270094662 ) ) ;
#94843=CARTESIAN_POINT ( 'NONE',  ( 76.17367474885168122, 65.32298633591217651, 14.07450646204639355 ) ) ;
#94845=DIRECTION ( 'NONE',  ( -0.8660254037844379305, -0.5000000000000015543, -0.000000000000000000 ) ) ;
#94849=CARTESIAN_POINT ( 'NONE',  ( 83.98760013881610575, 42.11425398099174089, 2.993173605489666933 ) ) ;
#94853=CARTESIAN_POINT ( 'NONE',  ( 83.73048316204189234, 51.68689211301329323, -14.84080274415373069 ) ) ;
#94854=CARTESIAN_POINT ( 'NONE',  ( 76.38896655220229093, 51.63588879817334742, -15.66987219493312367 ) ) ;
#94856=CARTESIAN_POINT ( 'NONE',  ( 80.46893305712502809, 57.11762031667031891, -16.22953243887947039 ) ) ;
#94863=B_SPLINE_CURVE_WITH_KNOTS ( 'NONE', 3,
 ( #37728, #28648, #99558, #98580, #59530, #30141, #61026, #84382, #45819, #76743, #21083, #62016, #7847, #17442, #86906, #8346, #78757, #24534, #62517, #55912, #40218, #46839, #54933, #92968, #48348, #38731, #16932, #71670, #23522, #47332, #24033 ),
 .UNSPECIFIED., .F., .F.,
 ( 4, 3, 3, 3, 3, 3, 3, 3, 3, 3, 4 ),
 ( 0.000000000000000000, 0.1333490885032361239, 0.3007194338854258242, 0.4699862290245113705, 0.5844252810809250631, 0.6686540514502664623, 0.7354980260655568092, 0.8028463152565741279, 0.8633854507757309227, 0.9437142632667492315, 1.000000000000000000 ),
 .UNSPECIFIED. ) ;
#94867=CARTESIAN_POINT ( 'NONE',  ( 71.22183910690829123, 62.20025648080263636, -14.61908299792422561 ) ) ;
#94869=CARTESIAN_POINT ( 'NONE',  ( 88.01747121012718367, 44.57676444843377794, -4.047986979593448886 ) ) ;
#94870=CARTESIAN_POINT ( 'NONE',  ( 69.36155480510052485, 70.48406901999045715, -2.430337453229784561 ) ) ;
#94872=CARTESIAN_POINT ( 'NONE',  ( 81.56932236973577233, 41.66854487856439704, 5.818248598875920052 ) ) ;
#94877=CARTESIAN_POINT ( 'NONE',  ( 25.03708881625784244, 16.58380873178787596, 6.180339887498953466 ) ) ;
#94880=CARTESIAN_POINT ( 'NONE',  ( 10.22618198766610575, 28.83705186507752671, 3.090169943749475401 ) ) ;
#94882=EDGE_CURVE ( 'NONE', #9557, #99079, #1137, .T. ) ;
#94884=CARTESIAN_POINT ( 'NONE',  ( 18.77112655976752009, 19.03677371833801502, 10.00000000000000533 ) ) ;
#94885=CARTESIAN_POINT ( 'NONE',  ( 68.18482425360609511, 65.67105585894155695, -10.27890673059631510 ) ) ;
#94902=CARTESIAN_POINT ( 'NONE',  ( 38.86330120330953974, 24.29860640527295246, -2.839279412974138328 ) ) ;
#94907=CARTESIAN_POINT ( 'NONE',  ( 33.90351810284484202, 25.28920272979928896, -7.433330006724141015 ) ) ;
#94914=CARTESIAN_POINT ( 'NONE',  ( 9.991594722369004700, 23.95586893147753926, 7.433330006724141015 ) ) ;
#94916=CARTESIAN_POINT ( 'NONE',  ( 16.72494223679300873, 27.84336893147755987, -7.433330006724137462 ) ) ;
#94928=CARTESIAN_POINT ( 'NONE',  ( 87.79538347886169447, 45.10662587206182650, 6.725936807544239393 ) ) ;
#94932=CARTESIAN_POINT ( 'NONE',  ( 86.18930939419189485, 47.16029689842823558, 10.81535065263619622 ) ) ;
#94934=CARTESIAN_POINT ( 'NONE',  ( 77.97772543808913781, 58.87949468740131209, 16.12526282269577393 ) ) ;
#94940=CARTESIAN_POINT ( 'NONE',  ( 80.51198428680064012, 43.68793065238016737, 9.861687463089005234 ) ) ;
#94944=DIRECTION ( 'NONE',  ( -0.8660254037844377084, -0.5000000000000014433, -0.000000000000000000 ) ) ;
#94947=EDGE_CURVE ( 'NONE', #30622, #56696, #8169, .T. ) ;
#94950=CARTESIAN_POINT ( 'NONE',  ( 39.11189823470242999, 30.78052372038643725, -10.00000000000000355 ) ) ;
#94954=VERTEX_POINT ( 'NONE', #27006 ) ;
#94958=DIRECTION ( 'NONE',  ( 0.000000000000000000, 0.6788029332000728999, 0.7343204871709473336 ) ) ;
#94961=CARTESIAN_POINT ( 'NONE',  ( 72.11625326144877590, 70.64305112490642102, 6.725456730032719932 ) ) ;
#94963=CARTESIAN_POINT ( 'NONE',  ( 82.77886453090131624, 53.33514393157792455, -15.29216242284640437 ) ) ;
#94968=CARTESIAN_POINT ( 'NONE',  ( 22.77687932801360660, 15.01110640527292261, 2.839279412974134775 ) ) ;
#94969=VECTOR ( 'NONE', #33288, 1000.000000000000114 ) ;
#94975=ORIENTED_EDGE ( 'NONE', *, *, #83937, .T. ) ;
#94980=DIRECTION ( 'NONE',  ( 0.5000000000000013323, -0.8660254037844378194, 0.000000000000000000 ) ) ;
#94981=VECTOR ( 'NONE', #28015, 1000.000000000000114 ) ;
#94984=CARTESIAN_POINT ( 'NONE',  ( 84.47860975560725194, 49.82577972120142817, -13.24615549146050952 ) ) ;
#94992=CARTESIAN_POINT ( 'NONE',  ( 82.16210765379520353, 40.80679471695141558, -1.129513917607761542 ) ) ;
#95001=ORIENTED_EDGE ( 'NONE', *, *, #11528, .T. ) ;
#95005=B_SPLINE_CURVE_WITH_KNOTS ( 'NONE', 3,
 ( #9116, #48626, #63310, #64820, #47106, #79561, #10118, #64314, #8618, #95767, #26323, #66799, #11628, #97726, #65794, #12625 ),
 .UNSPECIFIED., .F., .F.,
 ( 4, 1, 2, 2, 2, 1, 2, 2, 4 ),
 ( 0.000000000000000000, 0.1250000000000013878, 0.1875000000000020817, 0.2500000000000027756, 0.5000000000000042188, 0.6250000000000046629, 0.6875000000000039968, 0.7500000000000032196, 1.000000000000000000 ),
 .UNSPECIFIED. ) ;
#95006=CARTESIAN_POINT ( 'NONE',  ( 82.65244178817603427, 41.86818416018829936, 4.798348907845769062 ) ) ;
#95009=CARTESIAN_POINT ( 'NONE',  ( 68.89470241882965240, 64.09230978405759060, 12.06256359161597125 ) ) ;
#95010=CARTESIAN_POINT ( 'NONE',  ( 74.07678436671264421, 68.35284689741969544, -11.67875583378132198 ) ) ;
#95015=CARTESIAN_POINT ( 'NONE',  ( 82.69279102287485728, 44.35692915535365444, 9.190022298575403426 ) ) ;
#95017=EDGE_CURVE ( 'NONE', #96205, #63867, #96633, .T. ) ;
#95019=CARTESIAN_POINT ( 'NONE',  ( 68.49778638537657116, 64.30983983548141225, -12.35708682889201171 ) ) ;
#95024=CARTESIAN_POINT ( 'NONE',  ( 67.23469673426404825, 68.21886821911095922, -6.894059962813373410 ) ) ;
#95031=CARTESIAN_POINT ( 'NONE',  ( 14.85459438965255607, 31.68290643055187061, 3.479690158560446702E-15 ) ) ;
#95032=CARTESIAN_POINT ( 'NONE',  ( 75.29614551415185986, 66.72342768736930907, 13.41754944753248502 ) ) ;
#95046=LINE ( 'NONE', #25609, #60220 ) ;
#95051=B_SPLINE_SURFACE_WITH_KNOTS ( 'NONE', 3, 1, ( 
 ( #42893, #79971 ),
 ( #34812, #3929 ),
 ( #19652, #18137 ),
 ( #49037, #2963 ),
 ( #95177, #80983 ),
 ( #97168, #34330 ),
 ( #4422, #65713 ),
 ( #49524, #58602 ),
 ( #87609, #56626 ),
 ( #73833, #96668 ),
 ( #27236, #65226 ),
 ( #33857, #66231 ),
 ( #95691, #89102 ),
 ( #96169, #26730 ),
 ( #11549, #26238 ),
 ( #79476, #88593 ),
 ( #42408, #19155 ),
 ( #50514, #81466 ),
 ( #12040, #17639 ),
 ( #48537, #10040 ),
 ( #71851, #2448 ),
 ( #33330, #25747 ),
 ( #64227, #99007 ),
 ( #68085, #29591 ),
 ( #6293, #12538 ),
 ( #89578, #43411 ),
 ( #37185, #74358 ),
 ( #20141, #51012 ),
 ( #81963, #61812 ),
 ( #95153, #34303 ),
 ( #23317, #54204 ) ),
 .UNSPECIFIED., .F., .F., .F.,
 ( 4, 3, 3, 3, 3, 3, 3, 3, 3, 3, 4 ),
 ( 2, 2 ),
 ( 0.000000000000000000, 0.1122669598086755566, 0.2243161639709691235, 0.3396355846219065722, 0.4553962076585197916, 0.5677860799922422874, 0.6749047109689728652, 0.7773884377078309482, 0.8775581155834237812, 0.9782364162377977790, 1.000000000000000000 ),
 ( 0.000000000000000000, 1.000000000000000000 ),
 .UNSPECIFIED. ) ;
#95054=CARTESIAN_POINT ( 'NONE',  ( 83.82265501036586386, 51.54306753207543323, -14.37114190926680557 ) ) ;
#95055=CARTESIAN_POINT ( 'NONE',  ( 72.26191451101281871, 71.91445694603925176, -5.118044210176695863 ) ) ;
#95061=CARTESIAN_POINT ( 'NONE',  ( 35.86231599663030067, 42.74646525600393687, 2.839279412974139660 ) ) ;
#95068=CARTESIAN_POINT ( 'NONE',  ( 78.72187027071313992, 59.93413112120518349, 16.11827352649737222 ) ) ;
#95070=CARTESIAN_POINT ( 'NONE',  ( 88.44601041138486153, 44.07807065378580802, -2.614235559790803798 ) ) ;
#95073=CARTESIAN_POINT ( 'NONE',  ( 80.19020872641095821, 44.76014306349777883, 11.12255406994323792 ) ) ;
#95080=FACE_OUTER_BOUND ( 'NONE', #53840, .T. ) ;
#95084=ORIENTED_EDGE ( 'NONE', *, *, #8362, .F. ) ;
#95085=ADVANCED_FACE ( 'NONE', ( #97907 ), #19911, .T. ) ;
#95096=CARTESIAN_POINT ( 'NONE',  ( 70.97972651378927367, 61.11640933415372245, -14.48974805571130098 ) ) ;
#95097=CARTESIAN_POINT ( 'NONE',  ( 4.275827057391709651, 20.65586893147753500, -7.433330006724137462 ) ) ;
#95099=EDGE_CURVE ( 'NONE', #83325, #75846, #27514, .T. ) ;
#95100=CARTESIAN_POINT ( 'NONE',  ( 82.92857491607050235, 43.40443588184567147, -8.571747185156002757 ) ) ;
#95113=CARTESIAN_POINT ( 'NONE',  ( 6.430760413625676186, 27.21091486745858390, -1.111400068045478839E-16 ) ) ;
#95126=CARTESIAN_POINT ( 'NONE',  ( 74.38266378283655911, 61.70959607653536239, -15.06044949738370065 ) ) ;
#95128=CARTESIAN_POINT ( 'NONE',  ( 72.85736843160729848, 65.69469193138741048, -12.66355394330495976 ) ) ;
#95133=CARTESIAN_POINT ( 'NONE',  ( 70.35209472271311881, 71.19767260777499018, -1.695128100752382849 ) ) ;
#95136=CARTESIAN_POINT ( 'NONE',  ( 87.93887446415499198, 44.76116579897428949, -4.704258403839746805 ) ) ;
#95145=CARTESIAN_POINT ( 'NONE',  ( 76.48451822609287376, 51.58183040335976699, 15.64690190214837173 ) ) ;
#95149=CARTESIAN_POINT ( 'NONE',  ( 79.28496812781699532, 45.69181762706666916, -12.92980226288132251 ) ) ;
#95150=CARTESIAN_POINT ( 'NONE',  ( 73.36774340952439388, 69.90371635966560859, 9.665654898056800448 ) ) ;
#95153=CARTESIAN_POINT ( 'NONE',  ( 75.47830877820287299, 53.32463629016104534, 16.49710431891617901 ) ) ;
#95158=CARTESIAN_POINT ( 'NONE',  ( 13.25914332478948410, 9.783808731787853930, -6.180339887498949025 ) ) ;
#95162=CARTESIAN_POINT ( 'NONE',  ( 22.33066906249845118, 34.93396525600390845, 2.839279412974139660 ) ) ;
#95166=CARTESIAN_POINT ( 'NONE',  ( 15.60392711327956761, 29.98502408145592213, -5.678558825948271327 ) ) ;
#95168=CARTESIAN_POINT ( 'NONE',  ( 76.62156306105930526, 63.43458379359962152, 15.37592086074862685 ) ) ;
#95173=EDGE_CURVE ( 'NONE', #89471, #94179, #53948, .T. ) ;
#95177=CARTESIAN_POINT ( 'NONE',  ( 74.83378613555646552, 53.36200798387709909, 16.53431728583301208 ) ) ;
#95189=CARTESIAN_POINT ( 'NONE',  ( 81.29539683296886210, 43.25976067974499273, 9.624898955577574355 ) ) ;
#95190=AXIS2_PLACEMENT_3D ( 'NONE', #79176, #2648, #9755 ) ;
#95191=EDGE_LOOP ( 'NONE', ( #96709, #19438, #34187, #13212 ) ) ;
#95192=CARTESIAN_POINT ( 'NONE',  ( 38.19650550196953986, 40.79103043416552765, 8.090169943749478065 ) ) ;
#95194=CARTESIAN_POINT ( 'NONE',  ( 38.91320803870388545, 23.26216523072497466, -2.296566073217252530E-15 ) ) ;
#95195=CARTESIAN_POINT ( 'NONE',  ( 84.78734842081532008, 50.40784050611168965, -13.89907628984690113 ) ) ;
#95196=CARTESIAN_POINT ( 'NONE',  ( 85.21227539605295931, 47.84198382932485316, -11.42607603513809877 ) ) ;
#95197=PLANE ( 'NONE',  #62746 ) ;
#95209=CARTESIAN_POINT ( 'NONE',  ( 71.30420826232683851, 72.17422640967487268, -1.921222099538757666 ) ) ;
#95213=AXIS2_PLACEMENT_3D ( 'NONE', #6728, #84759, #22421 ) ;
#95224=CARTESIAN_POINT ( 'NONE',  ( 80.20857768024397672, 44.93227668248793094, -11.26798599081711139 ) ) ;
#95229=CARTESIAN_POINT ( 'NONE',  ( 80.48961952429826283, 48.34260169403606255, -13.60942759726339268 ) ) ;
#95236=CARTESIAN_POINT ( 'NONE',  ( 27.18159744850307291, 27.64441083166262203, -10.00000000000000533 ) ) ;
#95240=CARTESIAN_POINT ( 'NONE',  ( 87.84239280846571774, 44.77947472371889148, 4.964184461739159282 ) ) ;
#95244=CARTESIAN_POINT ( 'NONE',  ( 81.14562047329557970, 46.93173235953988609, 12.45778470005855354 ) ) ;
#95247=CARTESIAN_POINT ( 'NONE',  ( 71.49943747925016169, 59.40683841810739807, -15.72255559731668129 ) ) ;
#95255=CARTESIAN_POINT ( 'NONE',  ( 86.12973485563841791, 45.34942800271429775, 7.988429100487741685 ) ) ;
#95257=CARTESIAN_POINT ( 'NONE',  ( 22.49950015666239622, 18.15404122711133539, 8.090169943749479842 ) ) ;
#95259=CARTESIAN_POINT ( 'NONE',  ( 78.44787846840736734, 61.26446607870955319, 16.23792605971963354 ) ) ;
#95261=EDGE_CURVE ( 'NONE', #29839, #99059, #32337, .T. ) ;
#95264=AXIS2_PLACEMENT_3D ( 'NONE', #93793, #46639, #33451 ) ;
#95265=B_SPLINE_CURVE_WITH_KNOTS ( 'NONE', 3,
 ( #43706, #13333, #5712, #97931, #12334, #28506, #58890, #66518, #98933, #60389, #44691, #97443, #74648, #73632, #89384, #35113, #96973, #19938, #89859, #67505, #20434, #91344, #51300, #44198, #66024, #75135, #21904, #74143, #82273, #98438, #52793, #82767, #75620, #5224, #29028, #59900, #36103, #27540, #90868, #90364, #58409, #21419, #59387, #52305, #13810, #50810 ),
 .UNSPECIFIED., .F., .F.,
 ( 4, 1, 2, 2, 1, 2, 2, 1, 1, 2, 2, 1, 1, 2, 2, 1, 1, 2, 2, 1, 1, 1, 2, 2, 1, 1, 1, 2, 2, 4 ),
 ( 0.000000000000000000, 0.06250000000000124900, 0.09375000000000187350, 0.1250000000000024980, 0.1875000000000036360, 0.2187500000000061340, 0.2500000000000086042, 0.3125000000000096589, 0.3437500000000101585, 0.3593750000000088263, 0.3750000000000075495, 0.4375000000000063283, 0.4687500000000042188, 0.4843750000000027756, 0.5000000000000013323, 0.5625000000000027756, 0.5937500000000034417, 0.6093750000000038858, 0.6250000000000042188, 0.6875000000000037748, 0.7187500000000018874, 0.7343750000000011102, 0.7421875000000006661, 0.7500000000000001110, 0.8124999999999923395, 0.8437499999999882316, 0.8593749999999862332, 0.8671874999999853451, 0.8749999999999844569, 1.000000000000000000 ),
 .UNSPECIFIED. ) ;
#95272=CARTESIAN_POINT ( 'NONE',  ( 22.77272502854106762, 36.08080186712593473, -3.090169943749475845 ) ) ;
#95273=CARTESIAN_POINT ( 'NONE',  ( 77.93060254874920645, 48.03996307830335155, 14.17289077042660139 ) ) ;
#95277=CARTESIAN_POINT ( 'NONE',  ( 82.89640184790823696, 43.22043319592323485, -7.394312023068621009 ) ) ;
#95281=CARTESIAN_POINT ( 'NONE',  ( 81.93937120068478919, 47.03835499581510504, 12.23552757480724118 ) ) ;
#95283=CARTESIAN_POINT ( 'NONE',  ( 87.32537421964468649, 46.00455475262659633, 8.658505635391252397 ) ) ;
#95286=CARTESIAN_POINT ( 'NONE',  ( 81.69623217530381964, 41.61371471569898262, 5.513057524364318063 ) ) ;
#95289=CARTESIAN_POINT ( 'NONE',  ( 30.56436172585706146, 22.81029122506296147, 8.090169943749479842 ) ) ;
#95290=CARTESIAN_POINT ( 'NONE',  ( 43.53485905213462104, 24.94473085651396005, 1.475505719884397138E-15 ) ) ;
#95300=EDGE_CURVE ( 'NONE', #10592, #93322, #14217, .T. ) ;
#95308=ADVANCED_FACE ( 'NONE', ( #82327 ), #58873, .T. ) ;
#95315=DIRECTION ( 'NONE',  ( -0.4145187862775162602, 0.7179675985244458047, -0.5591929034707565638 ) ) ;
#95317=CARTESIAN_POINT ( 'NONE',  ( 30.25295400085950703, 18.26216523072495690, -2.296566073217252530E-15 ) ) ;
#95322=CARTESIAN_POINT ( 'NONE',  ( 7.821713311501573784, 19.91421378149916421, 9.188101187500008038 ) ) ;
#95325=B_SPLINE_CURVE_WITH_KNOTS ( 'NONE', 3,
 ( #80347, #40277, #72223, #79351, #65097, #18018, #41281, #79845, #48910, #3326, #65593, #57482, #88466, #96050, #19027, #41790 ),
 .UNSPECIFIED., .F., .F.,
 ( 4, 1, 2, 2, 2, 1, 2, 2, 4 ),
 ( 0.000000000000000000, 0.1250000000000003608, 0.1874999999999987232, 0.2499999999999971134, 0.4999999999999960587, 0.6249999999999973355, 0.6874999999999978906, 0.7499999999999983347, 1.000000000000000000 ),
 .UNSPECIFIED. ) ;
#95327=CARTESIAN_POINT ( 'NONE',  ( 72.38706308606541029, 71.16596677985461383, -6.083085609279689443 ) ) ;
#95328=CARTESIAN_POINT ( 'NONE',  ( 85.53100213312241351, 49.04015438577492603, 12.29448614360842207 ) ) ;
#95329=DIRECTION ( 'NONE',  ( 0.5000000000000013323, -0.8660254037844378194, 0.000000000000000000 ) ) ;
#95330=DIRECTION ( 'NONE',  ( -0.8660254037844378194, -0.5000000000000014433, -0.000000000000000000 ) ) ;
#95339=AXIS2_PLACEMENT_3D ( 'NONE', #26930, #18839, #80675 ) ;
#95341=CARTESIAN_POINT ( 'NONE',  ( 72.92456211408232036, 57.41452964202046161, -15.86517170058079529 ) ) ;
#95342=CARTESIAN_POINT ( 'NONE',  ( 78.06822720212770150, 61.43946511097403373, -16.16087495820213960 ) ) ;
#95348=ORIENTED_EDGE ( 'NONE', *, *, #89022, .F. ) ;
#95351=ORIENTED_EDGE ( 'NONE', *, *, #76521, .F. ) ;
#95352=CARTESIAN_POINT ( 'NONE',  ( 31.21403501649405854, 38.99752408145594273, 5.678558825948277544 ) ) ;
#95354=CARTESIAN_POINT ( 'NONE',  ( 72.16990512472445118, 70.69651720998999167, -7.560285414252116531 ) ) ;
#95356=CARTESIAN_POINT ( 'NONE',  ( 74.07459009150333884, 68.62600853808264389, 10.93350474783683701 ) ) ;
#95361=VECTOR ( 'NONE', #16394, 1000.000000000000114 ) ;
#95362=CARTESIAN_POINT ( 'NONE',  ( 76.86653180887425663, 57.81399073350881679, -16.12744706992745947 ) ) ;
#95363=CARTESIAN_POINT ( 'NONE',  ( 84.36170811391946245, 42.94765869660285063, -5.099173484137480727 ) ) ;
#95368=CARTESIAN_POINT ( 'NONE',  ( 67.37375070832676727, 69.12700154216180692, -3.154838971303389528 ) ) ;
#95370=DIRECTION ( 'NONE',  ( -0.8660254037844378194, -0.5000000000000014433, -0.000000000000000000 ) ) ;
#95382=LINE ( 'NONE', #25934, #37615 ) ;
#95384=CARTESIAN_POINT ( 'NONE',  ( 74.07698310468663294, 57.69947640214264339, 15.94728086577454285 ) ) ;
#95387=CARTESIAN_POINT ( 'NONE',  ( 80.12177396824181130, 57.42895151072963955, -16.59339316893575145 ) ) ;
#95396=CARTESIAN_POINT ( 'NONE',  ( 85.61005001132002690, 48.37664482377094544, -12.20733655019926189 ) ) ;
#95398=CARTESIAN_POINT ( 'NONE',  ( 67.82635223848771489, 69.76632902677688719, -0.4661708874699829752 ) ) ;
#95405=CARTESIAN_POINT ( 'NONE',  ( 81.35671934171772079, 51.65773188628860169, -14.92242472238318385 ) ) ;
#95412=CARTESIAN_POINT ( 'NONE',  ( 23.30503800868896391, 15.58380873178786885, 6.180339887498953466 ) ) ;
#95415=CARTESIAN_POINT ( 'NONE',  ( 72.09323793696012217, 72.40190342410335234, -3.152634433464706287 ) ) ;
#95417=CARTESIAN_POINT ( 'NONE',  ( 72.22324980102312963, 72.08985755953557373, 3.071982638949906086 ) ) ;
#95424=EDGE_CURVE ( 'NONE', #56685, #27648, #13862, .T. ) ;
#95431=CARTESIAN_POINT ( 'NONE',  ( 34.56506555475243658, 38.14336893147758900, 7.433330006724141015 ) ) ;
#95436=CARTESIAN_POINT ( 'NONE',  ( 28.07469292777547309, 37.18502408145594273, 5.678558825948277544 ) ) ;
#95439=CARTESIAN_POINT ( 'NONE',  ( 80.82369704674587751, 43.25674710424449643, -9.944928983646200038 ) ) ;
#95440=CARTESIAN_POINT ( 'NONE',  ( 35.94483945213000453, 39.49103043416551628, -8.090169943749479842 ) ) ;
#95442=CARTESIAN_POINT ( 'NONE',  ( 9.471979480098337234, 23.65586893147754566, -7.433330006724137462 ) ) ;
#95444=CARTESIAN_POINT ( 'NONE',  ( 13.34262526062736676, 23.10171378149917487, 9.188101187500008038 ) ) ;
#95447=DIRECTION ( 'NONE',  ( 0.000000000000000000, -0.7457702847286216130, 0.6662031840330625565 ) ) ;
#95450=ORIENTED_EDGE ( 'NONE', *, *, #59890, .T. ) ;
#95453=CARTESIAN_POINT ( 'NONE',  ( 66.26747146336929006, 68.17285859727699915, 4.275621689475024745 ) ) ;
#95454=CARTESIAN_POINT ( 'NONE',  ( 87.74082335983182190, 45.11567895962653552, 6.804767787324426997 ) ) ;
#95459=CARTESIAN_POINT ( 'NONE',  ( 86.61846192408904699, 47.19909516036467068, 10.60101820161781561 ) ) ;
#95461=CARTESIAN_POINT ( 'NONE',  ( 77.08070689000365405, 54.07734400991444801, 16.01987238285506976 ) ) ;
#95464=CARTESIAN_POINT ( 'NONE',  ( 27.85515008297419826, 39.58029201028043076, 1.583844403245397769 ) ) ;
#95476=VERTEX_POINT ( 'NONE', #46229 ) ;
#95481=CARTESIAN_POINT ( 'NONE',  ( 84.09736312987760698, 50.03755393994106271, -13.91877743777747511 ) ) ;
#95491=CARTESIAN_POINT ( 'NONE',  ( 24.30746885452586525, 16.96004757982090183, -5.678558825948276656 ) ) ;
#95492=ADVANCED_FACE ( 'NONE', ( #77153 ), #83801, .T. ) ;
#95497=ORIENTED_EDGE ( 'NONE', *, *, #84131, .T. ) ;
#95500=CARTESIAN_POINT ( 'NONE',  ( 40.44261144040436307, 35.30066082961425167, -10.00000000000000533 ) ) ;
#95502=B_SPLINE_CURVE_WITH_KNOTS ( 'NONE', 3,
 ( #37577, #68485, #99413, #85234, #29990, #60871, #38582, #84242, #14791, #45673 ),
 .UNSPECIFIED., .F., .F.,
 ( 4, 2, 2, 2, 4 ),
 ( 0.000000000000000000, 0.0002622400424272710705, 0.0005244800848545421411, 0.0007867201272818132116, 0.001048960169709084282 ),
 .UNSPECIFIED. ) ;
#95503=ADVANCED_FACE ( 'NONE', ( #91902 ), #84793, .T. ) ;
#95514=CARTESIAN_POINT ( 'NONE',  ( 82.45152879043666871, 40.98320966393081477, -1.227003583139177234 ) ) ;
#95524=CARTESIAN_POINT ( 'NONE',  ( 68.06957118741028978, 69.65128302599352139, 2.634141232969352764 ) ) ;
#95525=CARTESIAN_POINT ( 'NONE',  ( 84.37164395270971795, 44.14120688093528599, 7.575032260828749919 ) ) ;
#95532=CARTESIAN_POINT ( 'NONE',  ( 83.57287430471535572, 46.19826479596613922, 10.70837057327410236 ) ) ;
#95535=CARTESIAN_POINT ( 'NONE',  ( 68.63161566428617277, 64.63521157819846508, -12.16067767049918302 ) ) ;
#95548=EDGE_CURVE ( 'NONE', #31346, #65907, #21586, .T. ) ;
#95549=CARTESIAN_POINT ( 'NONE',  ( 16.96131155903493593, 31.83396525600390348, -2.839279412974133887 ) ) ;
#95550=CARTESIAN_POINT ( 'NONE',  ( 75.29548954665729354, 66.77148020061324019, 13.38688763123640868 ) ) ;
#95552=EDGE_CURVE ( 'NONE', #67404, #69466, #73437, .T. ) ;
#95562=CARTESIAN_POINT ( 'NONE',  ( 81.64250830485353561, 55.19057895047647122, -15.91435995628795474 ) ) ;
#95563=ORIENTED_EDGE ( 'NONE', *, *, #54261, .F. ) ;
#95567=CARTESIAN_POINT ( 'NONE',  ( 71.94676095904019064, 72.61122666528672198, 1.254485733363779998 ) ) ;
#95570=CARTESIAN_POINT ( 'NONE',  ( 70.94111402853239667, 71.65689097173488165, -0.4145321067673689575 ) ) ;
#95573=ORIENTED_EDGE ( 'NONE', *, *, #80105, .F. ) ;
#95575=CARTESIAN_POINT ( 'NONE',  ( 12.62681055351980497, 12.45404122711131656, -8.090169943749478065 ) ) ;
#95584=B_SPLINE_CURVE_WITH_KNOTS ( 'NONE', 3,
 ( #98517, #6292, #51388, #5788, #36676, #74725, #83328, #20010, #58962, #29590 ),
 .UNSPECIFIED., .F., .F.,
 ( 4, 2, 2, 2, 4 ),
 ( 0.3032312338214309122, 0.6516156169107113483, 0.7387117126830333724, 0.8258078084553553966, 1.000000000000000000 ),
 .UNSPECIFIED. ) ;
#95586=CARTESIAN_POINT ( 'NONE',  ( 81.62548137452107255, 50.83754634041029163, -14.55613181760977604 ) ) ;
#95587=CARTESIAN_POINT ( 'NONE',  ( 84.73310270403948152, 49.83751242549850247, -13.16584697690378469 ) ) ;
#95590=ORIENTED_EDGE ( 'NONE', *, *, #80172, .T. ) ;
#95598=CARTESIAN_POINT ( 'NONE',  ( 82.55774480658821801, 40.79923812737882116, 3.201402393612977626 ) ) ;
#95603=CARTESIAN_POINT ( 'NONE',  ( 86.64367300647309378, 42.83085291352504242, -0.9951962297809489044 ) ) ;
#95606=CARTESIAN_POINT ( 'NONE',  ( 70.50084764297432116, 61.32838242238358362, -14.81127601099039381 ) ) ;
#95607=VERTEX_POINT ( 'NONE', #79701 ) ;
#95614=CARTESIAN_POINT ( 'NONE',  ( 75.92077897862843372, 64.70916915221214083, -14.31233127451968024 ) ) ;
#95615=CARTESIAN_POINT ( 'NONE',  ( 79.36263291408793918, 45.67866562566761957, -12.88899626193393999 ) ) ;
#95618=FACE_OUTER_BOUND ( 'NONE', #2896, .T. ) ;
#95624=CARTESIAN_POINT ( 'NONE',  ( 77.99518601148065500, 61.05539905302716619, -15.87786080876372274 ) ) ;
#95636=CARTESIAN_POINT ( 'NONE',  ( 70.85377919256794144, 62.62944324200850588, -13.74144414313397000 ) ) ;
#95639=CARTESIAN_POINT ( 'NONE',  ( 69.63879362503037385, 66.25765348761015616, -10.58390212558767374 ) ) ;
#95640=EDGE_CURVE ( 'NONE', #78334, #54308, #1674, .T. ) ;
#95643=CARTESIAN_POINT ( 'NONE',  ( 80.65610391127596301, 43.47179147593435289, -9.508242589467984729 ) ) ;
#95644=CARTESIAN_POINT ( 'NONE',  ( 66.53768955469421087, 68.51814803147433963, 3.669749247662600133 ) ) ;
#95648=CARTESIAN_POINT ( 'NONE',  ( 88.06347939733042551, 44.64227011997218142, -4.166356787718118682 ) ) ;
#95652=CARTESIAN_POINT ( 'NONE',  ( 75.39279733249207993, 55.13144413046544656, -16.13680074438373069 ) ) ;
#95655=CARTESIAN_POINT ( 'NONE',  ( 76.48640248419296483, 51.58918322513654431, 15.64831315713032645 ) ) ;
#95657=ADVANCED_FACE ( 'NONE', ( #25451 ), #27343, .T. ) ;
#95659=CARTESIAN_POINT ( 'NONE',  ( 74.97172962767024273, 56.14972995073008377, -16.13536416545135666 ) ) ;
#95660=CARTESIAN_POINT ( 'NONE',  ( 82.84414721460336750, 52.67170891611750250, -15.43689080123882640 ) ) ;
#95661=CARTESIAN_POINT ( 'NONE',  ( 73.33758058659837786, 69.90254644623917102, 9.645949167502998023 ) ) ;
#95664=CARTESIAN_POINT ( 'NONE',  ( 77.08113471857714671, 63.57880127914461355, -15.41835532793242791 ) ) ;
#95667=ADVANCED_FACE ( 'NONE', ( #52231 ), #30432, .T. ) ;
#95673=CARTESIAN_POINT ( 'NONE',  ( 38.58005528328081368, 27.98920272979929535, 7.433330006724137462 ) ) ;
#95674=CARTESIAN_POINT ( 'NONE',  ( 82.20333476588919552, 49.18919034555798930, 14.05466216932103229 ) ) ;
#95675=CARTESIAN_POINT ( 'NONE',  ( 85.07790208279682531, 46.70498825579053914, -10.39314567700957248 ) ) ;
#95677=CARTESIAN_POINT ( 'NONE',  ( 16.72494223679300873, 27.84336893147755987, -7.433330006724137462 ) ) ;
#95685=ORIENTED_EDGE ( 'NONE', *, *, #93904, .T. ) ;
#95691=CARTESIAN_POINT ( 'NONE',  ( 75.02805439306581547, 53.11903014810299339, 16.50248075768144318 ) ) ;
#95699=CARTESIAN_POINT ( 'NONE',  ( 77.29458184488724726, 63.35267271352311269, -15.16560563611173507 ) ) ;
#95703=B_SPLINE_CURVE_WITH_KNOTS ( 'NONE', 3,
 ( #68995, #30506, #91345, #61397, #77101, #54280, #84256, #8211, #21905, #31491, #83753, #6713, #92348, #22409, #38596, #85250, #45200, #45685, #68503, #15795, #76139, #99425, #30002, #60887, #16304, #115, #85774, #91849, #46700, #53302, #69994, #22898, #30999, #61887, #78120, #8709, #53783, #39577, #14803, #7198, #77627, #39081, #609, #62383, #93340, #41085 ),
 .UNSPECIFIED., .F., .F.,
 ( 4, 1, 2, 2, 1, 2, 2, 1, 1, 2, 2, 1, 1, 2, 2, 1, 1, 2, 2, 1, 1, 1, 2, 2, 1, 1, 1, 2, 2, 4 ),
 ( 0.000000000000000000, 0.06249999999998988309, 0.09374999999998481770, 0.1249999999999797662, 0.1874999999999709677, 0.2187499999999666656, 0.2499999999999623634, 0.3124999999999550915, 0.3437499999999521494, 0.3593749999999485967, 0.3749999999999450440, 0.4374999999999310552, 0.4687499999999235056, 0.4843749999999204525, 0.4999999999999173439, 0.5624999999999097389, 0.5937499999999078515, 0.6093749999999069633, 0.6249999999999059641, 0.6874999999999060751, 0.7187499999999081846, 0.7343749999999101830, 0.7421874999999107381, 0.7499999999999111822, 0.8124999999999258371, 0.8437499999999352740, 0.8593749999999390488, 0.8671874999999417133, 0.8749999999999442668, 1.000000000000000000 ),
 .UNSPECIFIED. ) ;
#95704=CARTESIAN_POINT ( 'NONE',  ( 83.54554058275616057, 48.97625582294687518, 13.47504863331772107 ) ) ;
#95706=CARTESIAN_POINT ( 'NONE',  ( 31.05164846989082506, 29.87878583063843507, -9.188101187500006262 ) ) ;
#95707=CARTESIAN_POINT ( 'NONE',  ( 81.59934002536490993, 48.72548848104391084, -13.46818898573163459 ) ) ;
#95711=VECTOR ( 'NONE', #22095, 1000.000000000000114 ) ;
#95716=CARTESIAN_POINT ( 'NONE',  ( 85.33961507832758286, 48.52663690637297123, 12.44665103731247235 ) ) ;
#95722=LINE ( 'NONE', #25782, #12724 ) ;
#95728=ORIENTED_EDGE ( 'NONE', *, *, #95261, .T. ) ;
#95729=CARTESIAN_POINT ( 'NONE',  ( 80.07107477179017962, 44.27104509910737562, -11.43245809723916828 ) ) ;
#95740=CARTESIAN_POINT ( 'NONE',  ( 75.96894176838442547, 64.70234315684297144, -14.32931214104222839 ) ) ;
#95745=CARTESIAN_POINT ( 'NONE',  ( 87.76670979354591395, 44.75042847539244661, 5.006797044073166170 ) ) ;
#95747=CARTESIAN_POINT ( 'NONE',  ( 87.36419812053318878, 44.11474433763744685, -3.583216742975352087 ) ) ;
#95748=CARTESIAN_POINT ( 'NONE',  ( 81.16897067834024426, 46.99626341444099609, 12.49506798774365812 ) ) ;
#95749=CARTESIAN_POINT ( 'NONE',  ( 81.99805462481849361, 40.98459159741175029, -2.988575740387717339 ) ) ;
#95750=CARTESIAN_POINT ( 'NONE',  ( 80.80672984637854483, 43.46007305841095558, 9.388711751469632105 ) ) ;
#95754=CARTESIAN_POINT ( 'NONE',  ( 88.86175791728626905, 45.81123908072883921, 1.850091733736755357E-15 ) ) ;
#95759=CARTESIAN_POINT ( 'NONE',  ( 83.29111138074479470, 41.74013809017890964, 3.135737421875423259 ) ) ;
#95761=CARTESIAN_POINT ( 'NONE',  ( 78.44279992643997446, 61.32017871564067946, 16.22697472196325208 ) ) ;
#95765=CARTESIAN_POINT ( 'NONE',  ( 75.15176481940822839, 63.63400548413613933, -14.55503147312456846 ) ) ;
#95767=CARTESIAN_POINT ( 'NONE',  ( 79.14863538599044546, 51.66069612159751046, 15.78305943820313573 ) ) ;
#95768=CARTESIAN_POINT ( 'NONE',  ( 30.11635425815369871, 39.16126292948897003, -6.180339887498951690 ) ) ;
#95772=CARTESIAN_POINT ( 'NONE',  ( 86.48029715743111012, 43.63525664527010406, -3.689685108413566450 ) ) ;
#95776=CARTESIAN_POINT ( 'NONE',  ( 81.02962758293600132, 44.75529754875908139, 10.68588457171068029 ) ) ;
#95778=ADVANCED_FACE ( 'NONE', ( #38522 ), #15216, .T. ) ;
#95779=CARTESIAN_POINT ( 'NONE',  ( 87.12517199902879383, 46.36582989257513532, 8.660211133915520776 ) ) ;
#95782=CARTESIAN_POINT ( 'NONE',  ( 82.10268951128394121, 41.23340284509138343, 5.436379245411558259 ) ) ;
#95784=CARTESIAN_POINT ( 'NONE',  ( 87.10076192357585967, 46.06401709681040302, 8.920816893773267253 ) ) ;
#95786=CARTESIAN_POINT ( 'NONE',  ( 34.21278864456112956, 38.49103043416551628, -8.090169943749479842 ) ) ;
#95796=( BOUNDED_CURVE ( )  B_SPLINE_CURVE ( 2, ( #72505, #55742, #63872, #88236, #64884, #79116, #95830, #18291, #9698, #40558, #49185, #16767, #94809 ),
 .UNSPECIFIED., .F., .T. ) 
 B_SPLINE_CURVE_WITH_KNOTS ( ( 3, 2, 2, 2, 2, 2, 3 ),
 ( 0.9625000000000000222, 0.9649999999999999689, 0.9699999999999999734, 0.9749999999999999778, 0.9799999999999999822, 0.9849999999999999867, 0.9875000000000000444 ),
 .UNSPECIFIED. ) 
 CURVE ( )  GEOMETRIC_REPRESENTATION_ITEM ( )  RATIONAL_B_SPLINE_CURVE ( ( 0.9755282581475767101, 0.9755282581475772652, 1.000000000000000000, 0.9510565162951535312, 1.000000000000000000, 0.9510565162951535312, 1.000000000000000000, 0.9510565162951535312, 1.000000000000000000, 0.9510565162951535312, 1.000000000000000000, 0.9755282581475761550, 0.9755282581475767101 ) ) 
 REPRESENTATION_ITEM ( '' )  );
#95798=CARTESIAN_POINT ( 'NONE',  ( 29.86737195101775200, 39.01751292744058475, 6.180339887498949913 ) ) ;
#95800=CARTESIAN_POINT ( 'NONE',  ( 85.33699565288863198, 48.33901173460943568, -12.30238903177782284 ) ) ;
#95804=CARTESIAN_POINT ( 'NONE',  ( 67.14715456163476404, 67.13714923225593623, -8.580159373155410663 ) ) ;
#95809=CARTESIAN_POINT ( 'NONE',  ( 82.09429624515669843, 46.55866185173159977, -12.38170325825488405 ) ) ;
#95810=CARTESIAN_POINT ( 'NONE',  ( 31.32709252658613508, 23.80170272979928114, 7.433330006724137462 ) ) ;
#95815=CARTESIAN_POINT ( 'NONE',  ( 17.03285546273658113, 12.76004757982088655, 5.678558825948272215 ) ) ;
#95820=CARTESIAN_POINT ( 'NONE',  ( 72.16236457449060993, 71.55515601828724925, -5.863900035885150075 ) ) ;
#95829=ORIENTED_EDGE ( 'NONE', *, *, #31753, .F. ) ;
#95830=CARTESIAN_POINT ( 'NONE',  ( 40.17197850526964942, 35.14441083166263979, 10.00000000000000533 ) ) ;
#95832=CARTESIAN_POINT ( 'NONE',  ( 72.89289663045832413, 57.39945837237475246, -15.86463492901048511 ) ) ;
#95833=CARTESIAN_POINT ( 'NONE',  ( 78.38767366332245956, 61.45523861435393798, -15.84040300007290014 ) ) ;
#95841=CARTESIAN_POINT ( 'NONE',  ( 34.84170590957603508, 35.51421378149921537, -9.188101187500004485 ) ) ;
#95843=CARTESIAN_POINT ( 'NONE',  ( 78.19399585541323461, 47.86142559180260037, -14.00782581797713355 ) ) ;
#95845=CARTESIAN_POINT ( 'NONE',  ( 73.83553503644242255, 68.51229284434135991, 11.41127707145446379 ) ) ;
#95857=EDGE_CURVE ( 'NONE', #71488, #77470, #54714, .T. ) ;
#95861=CARTESIAN_POINT ( 'NONE',  ( 75.53717334121844829, 65.45021734152629733, 13.83070122522489775 ) ) ;
#95866=CARTESIAN_POINT ( 'NONE',  ( 83.88071297790835956, 44.16974053325726146, -8.051342648303378979 ) ) ;
#95867=CARTESIAN_POINT ( 'NONE',  ( 83.90573916032475665, 42.04407056160079037, 2.878155474715036188 ) ) ;
#95869=EDGE_CURVE ( 'NONE', #54902, #6127, #7035, .T. ) ;
#95875=CARTESIAN_POINT ( 'NONE',  ( 80.36956643484273854, 57.45342863445996784, -16.58888403658913901 ) ) ;
#95882=CARTESIAN_POINT ( 'NONE',  ( 67.41238942065514550, 68.07228407881235910, 6.202831302144204528 ) ) ;
#95886=B_SPLINE_SURFACE_WITH_KNOTS ( 'NONE', 3, 1, ( 
 ( #99766, #16155 ),
 ( #37932, #7051 ),
 ( #46030, #47546 ),
 ( #54633, #68845 ),
 ( #77472, #77967 ),
 ( #22763, #30857 ),
 ( #76947, #1472 ),
 ( #15133, #93695 ),
 ( #8066, #38941 ),
 ( #8562, #53640 ),
 ( #45539, #85092 ),
 ( #47053, #69353 ),
 ( #39927, #76471 ),
 ( #31349, #46535 ),
 ( #84595, #94195 ),
 ( #38439, #92691 ),
 ( #23242, #62232 ),
 ( #39429, #93184 ),
 ( #62739, #55135 ),
 ( #85612, #69846 ),
 ( #30357, #61742 ),
 ( #86121, #61242 ),
 ( #70348, #23738 ),
 ( #960, #9060 ),
 ( #24258, #16651 ),
 ( #31836, #78473 ),
 ( #92208, #7547 ),
 ( #70864, #84111 ),
 ( #54129, #32353 ),
 ( #63254, #24749 ),
 ( #14663, #100272 ) ),
 .UNSPECIFIED., .F., .F., .F.,
 ( 4, 3, 3, 3, 3, 3, 3, 3, 3, 3, 4 ),
 ( 2, 2 ),
 ( 0.000000000000000000, 0.1122669598086744880, 0.2243161639709676802, 0.3396355846218965246, 0.4553962076584930907, 0.5677860799922345159, 0.6749047109689415569, 0.7773884377078037478, 0.8775581155834019098, 0.9782364162377737982, 1.000000000000000000 ),
 ( 0.000000000000000000, 1.000000000000000000 ),
 .UNSPECIFIED. ) ;
#95887=CARTESIAN_POINT ( 'NONE',  ( 15.94411698533127542, 24.90829794293879473, 10.00000000000000355 ) ) ;
#95889=CARTESIAN_POINT ( 'NONE',  ( 81.62374368218522136, 41.76230689378201788, 5.959470817902202455 ) ) ;
#95893=EDGE_CURVE ( 'NONE', #15371, #46807, #52970, .T. ) ;
#95895=CARTESIAN_POINT ( 'NONE',  ( 81.59595212483856130, 51.57806399716481138, -14.84616350707865706 ) ) ;
#95904=CARTESIAN_POINT ( 'NONE',  ( 22.23522817490527714, 21.03677371833801857, 10.00000000000000533 ) ) ;
#95907=CARTESIAN_POINT ( 'NONE',  ( 72.27382559518491689, 71.95406617239038383, -3.744659656737702846 ) ) ;
#95909=CARTESIAN_POINT ( 'NONE',  ( 73.84282566857962138, 55.27273555838809216, -16.11958282414678933 ) ) ;
#95918=CARTESIAN_POINT ( 'NONE',  ( 32.72297390791170812, 40.93396525600392977, 2.839279412974139660 ) ) ;
#95921=CARTESIAN_POINT ( 'NONE',  ( 38.48863484149602954, 25.14754757982092670, -5.678558825948276656 ) ) ;
#95922=CARTESIAN_POINT ( 'NONE',  ( 16.82306525903893046, 33.21091486745860522, -1.111400068045478839E-16 ) ) ;
#95928=CARTESIAN_POINT ( 'NONE',  ( 13.91516400911260298, 10.96004757982088584, -5.678558825948276656 ) ) ;
#95930=CARTESIAN_POINT ( 'NONE',  ( 9.658441966945924051, 28.68290643055185996, 3.479690158560446702E-15 ) ) ;
#95933=CARTESIAN_POINT ( 'NONE',  ( 19.12865694409072148, 32.81751292744056769, -6.180339887498951690 ) ) ;
#95936=VERTEX_POINT ( 'NONE', #66839 ) ;
#95939=CARTESIAN_POINT ( 'NONE',  ( 66.28997097015012230, 68.26748065702538781, 4.019969198947881850 ) ) ;
#95945=CARTESIAN_POINT ( 'NONE',  ( 86.17334730086119521, 47.14257514812162952, 10.80675504988608715 ) ) ;
#95947=CARTESIAN_POINT ( 'NONE',  ( 76.71053421761779134, 52.48524597020742988, 15.80685200372052357 ) ) ;
#95950=CARTESIAN_POINT ( 'NONE',  ( 78.31205730182037428, 61.08770274336716710, -15.90934363462768708 ) ) ;
#95951=CARTESIAN_POINT ( 'NONE',  ( 88.54283264841694745, 43.89585489789003248, -0.1669414168386812725 ) ) ;
#95953=CARTESIAN_POINT ( 'NONE',  ( 80.00967963870645860, 48.43740759703016607, -14.32305472254445355 ) ) ;
#95954=CARTESIAN_POINT ( 'NONE',  ( 80.53863348453982951, 43.47454295502769384, 9.594131698209025672 ) ) ;
#95955=EDGE_LOOP ( 'NONE', ( #32651, #16395, #77486, #52810 ) ) ;
#95961=VECTOR ( 'NONE', #91804, 999.9999999999998863 ) ;
#95962=VERTEX_POINT ( 'NONE', #5056 ) ;
#95971=CARTESIAN_POINT ( 'NONE',  ( 70.39481278435968647, 67.27897370780323172, 9.975814553134231488 ) ) ;
#95978=CARTESIAN_POINT ( 'NONE',  ( 26.65055534615017763, 21.10170272979927830, -7.433330006724141015 ) ) ;
#95980=CARTESIAN_POINT ( 'NONE',  ( 77.52911305372531103, 49.76152791203366377, -14.96532194459484089 ) ) ;
#95986=CARTESIAN_POINT ( 'NONE',  ( 43.20833262110986084, 30.11029122506297995, -8.090169943749478065 ) ) ;
#95994=DIRECTION ( 'NONE',  ( 0.5295078238379082869, 0.5024823063052964445, -0.6834712842135746147 ) ) ;
#96000=CARTESIAN_POINT ( 'NONE',  ( 72.10617024684209753, 72.18421392457030095, 4.031754617348218162 ) ) ;
#96001=CARTESIAN_POINT ( 'NONE',  ( 20.76744934909352125, 17.15404122711133184, 8.090169943749479842 ) ) ;
#96005=ORIENTED_EDGE ( 'NONE', *, *, #9028, .F. ) ;
#96008=FACE_OUTER_BOUND ( 'NONE', #44306, .T. ) ;
#96017=CARTESIAN_POINT ( 'NONE',  ( 82.28690965751638942, 43.63874554170867270, 8.536804570166234285 ) ) ;
#96021=CARTESIAN_POINT ( 'NONE',  ( 68.72674373419405924, 63.90649084318997097, -12.13465469835461086 ) ) ;
#96035=CARTESIAN_POINT ( 'NONE',  ( 26.36427918851389407, 18.14754757982090894, -5.678558825948276656 ) ) ;
#96048=CARTESIAN_POINT ( 'NONE',  ( 81.61641279696441131, 55.18026415975641186, -15.91513574126469877 ) ) ;
#96050=CARTESIAN_POINT ( 'NONE',  ( 75.38995058909416969, 64.62150842440080112, -14.61153521280294143 ) ) ;
#96055=FACE_OUTER_BOUND ( 'NONE', #31590, .T. ) ;
#96059=CARTESIAN_POINT ( 'NONE',  ( 12.95333698454457760, 7.288480858562293996, 1.475505719884397138E-15 ) ) ;
#96062=CARTESIAN_POINT ( 'NONE',  ( 78.17252251050902601, 61.73722341659915713, 16.11086890919063919 ) ) ;
#96063=EDGE_CURVE ( 'NONE', #34200, #69466, #52625, .T. ) ;
#96067=CARTESIAN_POINT ( 'NONE',  ( 79.19031144066791228, 60.01104784500377320, 16.13641150400241386 ) ) ;
#96070=CARTESIAN_POINT ( 'NONE',  ( 80.33501951744612768, 51.27104759306554627, -14.99191532815999928 ) ) ;
#96071=CARTESIAN_POINT ( 'NONE',  ( 73.48070833180072725, 69.95435187952867295, -9.683457271946362965 ) ) ;
#96072=FACE_OUTER_BOUND ( 'NONE', #89476, .T. ) ;
#96074=VERTEX_POINT ( 'NONE', #83583 ) ;
#96077=PLANE ( 'NONE',  #57899 ) ;
#96081=( BOUNDED_CURVE ( )  B_SPLINE_CURVE ( 2, ( #9953, #1849, #71759, #23615, #32731, #48441, #77341, #69731, #77853, #336, #832, #39310, #93060 ),
 .UNSPECIFIED., .F., .T. ) 
 B_SPLINE_CURVE_WITH_KNOTS ( ( 3, 2, 2, 2, 2, 2, 3 ),
 ( 0.6625000000000000888, 0.6650000000000000355, 0.6700000000000000400, 0.6750000000000000444, 0.6800000000000000488, 0.6850000000000000533, 0.6875000000000000000 ),
 .UNSPECIFIED. ) 
 CURVE ( )  GEOMETRIC_REPRESENTATION_ITEM ( )  RATIONAL_B_SPLINE_CURVE ( ( 0.9755282581475767101, 0.9755282581475772652, 1.000000000000000000, 0.9510565162951535312, 1.000000000000000000, 0.9510565162951535312, 1.000000000000000000, 0.9510565162951535312, 1.000000000000000000, 0.9510565162951535312, 1.000000000000000000, 0.9755282581475768211, 0.9755282581475768211 ) ) 
 REPRESENTATION_ITEM ( '' )  );
#96084=CARTESIAN_POINT ( 'NONE',  ( 81.96547941067910870, 41.17040324926905726, 3.814626384468423392 ) ) ;
#96093=CARTESIAN_POINT ( 'NONE',  ( 75.43135263623493358, 53.72653608919682711, 16.05972988992205686 ) ) ;
#96098=CARTESIAN_POINT ( 'NONE',  ( 78.47445242937311605, 48.02372130040763665, -14.00813393920220662 ) ) ;
#96099=CARTESIAN_POINT ( 'NONE',  ( 76.23413744742458675, 64.83205629739494213, -14.34075561390215015 ) ) ;
#96102=( BOUNDED_CURVE ( )  B_SPLINE_CURVE ( 2, ( #62367, #84731, #78103, #93325, #23878, #86248, #16786, #63391, #17286, #15271, #7690, #71012, #9194 ),
 .UNSPECIFIED., .F., .T. ) 
 B_SPLINE_CURVE_WITH_KNOTS ( ( 3, 2, 2, 2, 2, 2, 3 ),
 ( 0.6625000000000000888, 0.6650000000000000355, 0.6700000000000000400, 0.6750000000000000444, 0.6800000000000000488, 0.6850000000000000533, 0.6875000000000000000 ),
 .UNSPECIFIED. ) 
 CURVE ( )  GEOMETRIC_REPRESENTATION_ITEM ( )  RATIONAL_B_SPLINE_CURVE ( ( 0.9755282581475767101, 0.9755282581475772652, 1.000000000000000000, 0.9510565162951535312, 1.000000000000000000, 0.9510565162951535312, 1.000000000000000000, 0.9510565162951535312, 1.000000000000000000, 0.9510565162951535312, 1.000000000000000000, 0.9755282581475768211, 0.9755282581475768211 ) ) 
 REPRESENTATION_ITEM ( '' )  );
#96105=CARTESIAN_POINT ( 'NONE',  ( 83.67416965427615594, 41.61942911856458949, 0.1873010706438003881 ) ) ;
#96106=CARTESIAN_POINT ( 'NONE',  ( 88.18231713977282027, 44.19070851116610754, -1.765747973715714236 ) ) ;
#96110=CARTESIAN_POINT ( 'NONE',  ( 66.10352841413255476, 68.74164459769689017, 0.05599916294954376816 ) ) ;
#96116=DIRECTION ( 'NONE',  ( 0.3782958374750531316, 0.000000000000000000, 0.9256847516023195555 ) ) ;
#96117=CARTESIAN_POINT ( 'NONE',  ( 82.19428834490943814, 44.75703489301101712, -9.991791377543423280 ) ) ;
#96120=CARTESIAN_POINT ( 'NONE',  ( 88.40933139567989940, 44.00655032011064094, 2.323659332633148722 ) ) ;
#96123=B_SPLINE_SURFACE_WITH_KNOTS ( 'NONE', 3, 1, ( 
 ( #70202, #8916 ),
 ( #39292, #9422 ),
 ( #31692, #46916 ),
 ( #39784, #93554 ),
 ( #40297, #71239 ),
 ( #17517, #48423 ),
 ( #71743, #72755 ),
 ( #4307, #33219 ),
 ( #11934, #42790 ),
 ( #87501, #96067 ),
 ( #26625, #81853 ),
 ( #80877, #50904 ),
 ( #3348, #42301 ),
 ( #19046, #73725 ),
 ( #49919, #56513 ),
 ( #2848, #73234 ),
 ( #41808, #34223 ),
 ( #40798, #79866 ),
 ( #33737, #66114 ),
 ( #64629, #41300 ),
 ( #3826, #2336 ),
 ( #81365, #64117 ),
 ( #97063, #35212 ),
 ( #88484, #27634 ),
 ( #58499, #11448 ),
 ( #34709, #65118 ),
 ( #10428, #95068 ),
 ( #80364, #87986 ),
 ( #89472, #25629 ),
 ( #18036, #65610 ),
 ( #10936, #96563 ) ),
 .UNSPECIFIED., .F., .F., .F.,
 ( 4, 3, 3, 3, 3, 3, 3, 3, 3, 3, 4 ),
 ( 2, 2 ),
 ( 0.000000000000000000, 0.1333490885032346807, 0.3007194338854402571, 0.4699862290245250818, 0.5844252810809306142, 0.6686540514502837818, 0.7354980260655518132, 0.8028463152565542549, 0.8633854507757066088, 0.9437142632667097075, 1.000000000000000000 ),
 ( 0.000000000000000000, 1.000000000000000000 ),
 .UNSPECIFIED. ) ;
#96124=CARTESIAN_POINT ( 'NONE',  ( 72.86930352181153125, 62.14391970216223626, -14.54723569203636124 ) ) ;
#96125=CARTESIAN_POINT ( 'NONE',  ( 80.01857661193632509, 58.13192459411606450, 16.26806844874244362 ) ) ;
#96126=CARTESIAN_POINT ( 'NONE',  ( 73.99930017925848347, 65.38118273369227040, -13.31775726196476661 ) ) ;
#96128=CARTESIAN_POINT ( 'NONE',  ( 80.93613592876508278, 42.95327845838396286, -9.503115154746584636 ) ) ;
#96134=CARTESIAN_POINT ( 'NONE',  ( 88.02334914385743048, 44.75692394554157261, -4.561185668002573301 ) ) ;
#96136=FACE_OUTER_BOUND ( 'NONE', #50896, .T. ) ;
#96142=CARTESIAN_POINT ( 'NONE',  ( 79.18557317608008361, 54.66583532628084896, -15.99631523082424600 ) ) ;
#96149=CARTESIAN_POINT ( 'NONE',  ( 83.65470120645571228, 42.99590864647574051, -7.250413499812092155 ) ) ;
#96153=CARTESIAN_POINT ( 'NONE',  ( 33.82173346387272517, 28.03085787977764909, 9.188101187500006262 ) ) ;
#96154=CARTESIAN_POINT ( 'NONE',  ( 81.52443553237245055, 48.71771659309563063, -14.02210268134143512 ) ) ;
#96155=CARTESIAN_POINT ( 'NONE',  ( 85.79712387213245961, 46.58647785539236708, -9.836184165120874567 ) ) ;
#96157=CARTESIAN_POINT ( 'NONE',  ( 19.08966579672462061, 13.94754757982089188, 5.678558825948272215 ) ) ;
#96169=CARTESIAN_POINT ( 'NONE',  ( 75.06334566771610639, 53.10221114767903572, 16.49884716248028838 ) ) ;
#96178=CARTESIAN_POINT ( 'NONE',  ( 77.00525802853118762, 62.90742007320628204, -15.26276671481578973 ) ) ;
#96180=VERTEX_POINT ( 'NONE', #75457 ) ;
#96184=CARTESIAN_POINT ( 'NONE',  ( 80.25178558894602077, 57.14685393251872370, -16.23521980932009612 ) ) ;
#96187=CARTESIAN_POINT ( 'NONE',  ( 34.79119414172389213, 25.80170272979928470, 7.433330006724137462 ) ) ;
#96188=CARTESIAN_POINT ( 'NONE',  ( 83.16021335601298858, 48.33887568228013976, -12.68239118580088132 ) ) ;
#96197=CARTESIAN_POINT ( 'NONE',  ( 85.63218110832043806, 48.66108713908771932, 12.42024371201311972 ) ) ;
#96205=VERTEX_POINT ( 'NONE', #51134 ) ;
#96206=CARTESIAN_POINT ( 'NONE',  ( 74.15479259499207387, 55.62765001666249276, -16.59030973340311022 ) ) ;
#96209=ORIENTED_EDGE ( 'NONE', *, *, #4754, .T. ) ;
#96211=CARTESIAN_POINT ( 'NONE',  ( 87.15508732983295204, 45.91009000376428872, -8.663677684674611967 ) ) ;
#96217=EDGE_LOOP ( 'NONE', ( #39747, #86217, #40659, #79512 ) ) ;
#96222=CARTESIAN_POINT ( 'NONE',  ( 22.77272502854106762, 36.08080186712593473, -3.090169943749475845 ) ) ;
#96226=CARTESIAN_POINT ( 'NONE',  ( 69.46471525646846601, 62.64179866298621846, -13.84787601622161901 ) ) ;
#96233=CARTESIAN_POINT ( 'NONE',  ( 82.17119170860053146, 40.62002387180137220, -3.389656615904392378 ) ) ;
#96242=CARTESIAN_POINT ( 'NONE',  ( 80.31687802057754766, 51.50889260389730140, 15.08045506871916608 ) ) ;
#96243=CARTESIAN_POINT ( 'NONE',  ( 67.93311001602360477, 69.70947576764457665, -1.762602472474833926 ) ) ;
#96245=CARTESIAN_POINT ( 'NONE',  ( 78.26458253827964029, 61.66843869688886315, 16.13698506349214412 ) ) ;
#96249=CARTESIAN_POINT ( 'NONE',  ( 71.79577640164012564, 64.60757656470461541, -12.94397184867940176 ) ) ;
#96252=CARTESIAN_POINT ( 'NONE',  ( 36.35590661721340666, 26.15404122711136026, 8.090169943749479842 ) ) ;
#96256=CARTESIAN_POINT ( 'NONE',  ( 85.74962510757818279, 43.49686255595008078, -4.555259895190277852 ) ) ;
#96258=CARTESIAN_POINT ( 'NONE',  ( 82.57639827720844039, 49.19050994824535650, 13.45810755646198409 ) ) ;
#96260=CARTESIAN_POINT ( 'NONE',  ( 86.84204249716189850, 45.92435628226732547, 8.934002094794735171 ) ) ;
#96262=CARTESIAN_POINT ( 'NONE',  ( 82.03687330897646746, 41.20536659497016529, 5.461263348486533609 ) ) ;
#96266=CARTESIAN_POINT ( 'NONE',  ( 86.96880057233924788, 46.02321981727299516, 8.968744825131210519 ) ) ;
#96268=CARTESIAN_POINT ( 'NONE',  ( 34.71711421221060334, 41.81751292744059612, -6.180339887498951690 ) ) ;
#96271=LINE ( 'NONE', #81568, #97541 ) ;
#96274=EDGE_CURVE ( 'NONE', #54157, #55257, #43059, .T. ) ;
#96280=ORIENTED_EDGE ( 'NONE', *, *, #56808, .T. ) ;
#96284=CARTESIAN_POINT ( 'NONE',  ( 67.27543762298243735, 66.59126356583220741, -8.544430691054564875 ) ) ;
#96289=CARTESIAN_POINT ( 'NONE',  ( 28.99364183777449000, 25.24335787977764767, -9.188101187500008038 ) ) ;
#96294=CARTESIAN_POINT ( 'NONE',  ( 12.79778405566451482, 30.49540643055186351, 3.479690158560446702E-15 ) ) ;
#96298=ORIENTED_EDGE ( 'NONE', *, *, #5153, .F. ) ;
#96307=ORIENTED_EDGE ( 'NONE', *, *, #11654, .F. ) ;
#96311=ORIENTED_EDGE ( 'NONE', *, *, #91965, .F. ) ;
#96312=CARTESIAN_POINT ( 'NONE',  ( 66.09342489060131243, 68.50075773664546830, -2.578996081064114598 ) ) ;
#96314=CARTESIAN_POINT ( 'NONE',  ( 72.65506221629649986, 57.10929429594364137, -16.37270640794472598 ) ) ;
#96315=CARTESIAN_POINT ( 'NONE',  ( 78.06091359999885526, 61.03177674231440619, -15.89086307328630276 ) ) ;
#96321=ORIENTED_EDGE ( 'NONE', *, *, #39740, .F. ) ;
#96324=CARTESIAN_POINT ( 'NONE',  ( 36.96107555259132482, 29.84335787977765619, 9.188101187500006262 ) ) ;
#96326=CARTESIAN_POINT ( 'NONE',  ( 78.17699230315889736, 47.82979171855502187, -13.99723441571071980 ) ) ;
#96334=DIRECTION ( 'NONE',  ( -0.4635919272833941562, 0.8029647720336182681, 0.3746065934159032440 ) ) ;
#96335=CARTESIAN_POINT ( 'NONE',  ( 87.53652538659707716, 43.81626475740009141, -1.345572693404142983 ) ) ;
#96336=CARTESIAN_POINT ( 'NONE',  ( 87.49661283931372679, 43.54010870773999642, 2.689214756758103508 ) ) ;
#96338=CARTESIAN_POINT ( 'NONE',  ( 73.43762515466688967, 73.52662068827324049, 2.033788753608857291E-15 ) ) ;
#96340=DIRECTION ( 'NONE',  ( -0.8660254037844377084, -0.5000000000000014433, -0.000000000000000000 ) ) ;
#96358=CARTESIAN_POINT ( 'NONE',  ( 75.06845965858576619, 62.64932666483513657, 14.91362258529271756 ) ) ;
#96370=CARTESIAN_POINT ( 'NONE',  ( 24.48906155743269508, 15.10801979619929014, 3.090169943749476733 ) ) ;
#96379=CARTESIAN_POINT ( 'NONE',  ( 79.91325939341504636, 52.13032348250509784, -15.32992361654147828 ) ) ;
#96388=CARTESIAN_POINT ( 'NONE',  ( 18.79197634579341525, 22.80066082961421614, 10.00000000000000533 ) ) ;
#96394=CARTESIAN_POINT ( 'NONE',  ( 73.87485074719697309, 55.34240436449581324, -16.11747225289941099 ) ) ;
#96403=CARTESIAN_POINT ( 'NONE',  ( 31.19238438139944947, 38.98502408145593989, -5.678558825948271327 ) ) ;
#96406=CARTESIAN_POINT ( 'NONE',  ( 40.59535201087842182, 25.29860640527295601, -2.839279412974138328 ) ) ;
#96410=CARTESIAN_POINT ( 'NONE',  ( 81.03765089968891289, 43.40990969291960511, -9.978953348122514555 ) ) ;
#96414=CARTESIAN_POINT ( 'NONE',  ( 6.417452267959404821, 25.74646525600388003, 2.839279412974139660 ) ) ;
#96416=CARTESIAN_POINT ( 'NONE',  ( 13.12254358208367577, 30.68290643055186706, 3.479690158560446702E-15 ) ) ;
#96422=CARTESIAN_POINT ( 'NONE',  ( 74.95119442303548851, 53.20651566882768435, -16.03659100943698945 ) ) ;
#96430=CARTESIAN_POINT ( 'NONE',  ( 66.34027612997587653, 68.16670350466722539, 4.419308956821091705 ) ) ;
#96435=CARTESIAN_POINT ( 'NONE',  ( 75.28650001057752661, 66.67572118895705557, 13.44401380721711270 ) ) ;
#96437=CARTESIAN_POINT ( 'NONE',  ( 86.57431924022760938, 47.22157117268152149, 10.65071021778218352 ) ) ;
#96439=CARTESIAN_POINT ( 'NONE',  ( 77.04668223076443212, 53.92430565998370184, 16.00320842628551787 ) ) ;
#96444=CARTESIAN_POINT ( 'NONE',  ( 81.04805182755087856, 43.65517749199150188, 9.457138610966682180 ) ) ;
#96456=VECTOR ( 'NONE', #59177, 1000.000000000000114 ) ;
#96460=EDGE_CURVE ( 'NONE', #62465, #86376, #55496, .T. ) ;
#96468=VERTEX_POINT ( 'NONE', #94555 ) ;
#96470=CARTESIAN_POINT ( 'NONE',  ( 28.14623683147711830, 18.11110640527293114, -2.839279412974138328 ) ) ;
#96473=ORIENTED_EDGE ( 'NONE', *, *, #76491, .F. ) ;
#96476=CARTESIAN_POINT ( 'NONE',  ( 69.92928646124981640, 62.82442351299641103, 13.89675756931289641 ) ) ;
#96477=ADVANCED_FACE ( 'NONE', ( #86482 ), #87987, .T. ) ;
#96479=CARTESIAN_POINT ( 'NONE',  ( 11.69612814616573893, 25.49103043416548076, -8.090169943749479842 ) ) ;
#96490=CARTESIAN_POINT ( 'NONE',  ( 15.94411698533127542, 24.90829794293879473, 10.00000000000000355 ) ) ;
#96495=ORIENTED_EDGE ( 'NONE', *, *, #34630, .T. ) ;
#96498=CARTESIAN_POINT ( 'NONE',  ( 80.53589555931883126, 46.94866704237161770, -12.72290194427851517 ) ) ;
#96505=CARTESIAN_POINT ( 'NONE',  ( 73.97927654802940367, 68.30869415006648637, -11.66811813765111516 ) ) ;
#96510=CARTESIAN_POINT ( 'NONE',  ( 79.31084698818212075, 59.85625551150462087, -16.50595436643997260 ) ) ;
#96513=CARTESIAN_POINT ( 'NONE',  ( 72.93270222632345678, 70.75261854202811662, -7.421515863126949775 ) ) ;
#96515=VECTOR ( 'NONE', #52968, 1000.000000000000000 ) ;
#96518=CARTESIAN_POINT ( 'NONE',  ( 68.21857645778533197, 68.29686920240547465, -7.752314361411196231 ) ) ;
#96520=CARTESIAN_POINT ( 'NONE',  ( 68.32831816981907025, 66.75461077405910260, 9.160816392852566992 ) ) ;
#96526=CARTESIAN_POINT ( 'NONE',  ( 74.39841895140679640, 68.21392270468032848, 11.95628786500076934 ) ) ;
#96528=CARTESIAN_POINT ( 'NONE',  ( 22.39019813391814751, 21.43085787977763701, -9.188101187500008038 ) ) ;
#96529=CARTESIAN_POINT ( 'NONE',  ( 74.76437051368166919, 67.10386306624577912, 12.96231939749656448 ) ) ;
#96533=DIRECTION ( 'NONE',  ( 0.5000000000000014433, -0.8660254037844378194, 0.000000000000000000 ) ) ;
#96537=CARTESIAN_POINT ( 'NONE',  ( 34.73896580337741113, 43.55466486950702887, 7.012934429366973338E-14 ) ) ;
#96539=CARTESIAN_POINT ( 'NONE',  ( 81.54227884105102930, 55.16382101384258618, -15.91942278333091920 ) ) ;
#96540=EDGE_LOOP ( 'NONE', ( #20090, #65369, #5375, #46949 ) ) ;
#96542=CARTESIAN_POINT ( 'NONE',  ( 80.28753194487839551, 45.30207178207673735, 12.22351710471137665 ) ) ;
#96543=CARTESIAN_POINT ( 'NONE',  ( 71.85125637137586807, 72.20757445900991911, 0.5766358698793758730 ) ) ;
#96545=CARTESIAN_POINT ( 'NONE',  ( 83.06094347246988718, 41.92204296775934580, 4.233641397788413308 ) ) ;
#96546=CARTESIAN_POINT ( 'NONE',  ( 80.56202954020663753, 57.53823600680942718, 16.23110421993949259 ) ) ;
#96549=CARTESIAN_POINT ( 'NONE',  ( 72.06693479607845632, 71.51559350784613400, -5.828149303013867133 ) ) ;
#96555=CARTESIAN_POINT ( 'NONE',  ( 5.363317384539951327, 21.83478043621385822, -8.090169943749479842 ) ) ;
#96563=CARTESIAN_POINT ( 'NONE',  ( 78.70150085959762976, 59.83202584994827333, 16.12694553795979502 ) ) ;
#96565=CARTESIAN_POINT ( 'NONE',  ( 75.06725799386214248, 52.99710587067458079, -16.48800421929521676 ) ) ;
#96570=CARTESIAN_POINT ( 'NONE',  ( 80.48237008273157755, 51.22225194333302767, -14.94672880192676523 ) ) ;
#96572=CARTESIAN_POINT ( 'NONE',  ( 73.44884507967250897, 69.80860085198864340, -9.835095417347671898 ) ) ;
#96573=CARTESIAN_POINT ( 'NONE',  ( 84.44631528110988938, 49.90853024617071299, -13.72425691458318475 ) ) ;
#96579=ORIENTED_EDGE ( 'NONE', *, *, #11902, .T. ) ;
#96590=DIRECTION ( 'NONE',  ( 0.5000000000000013323, -0.8660254037844378194, 0.000000000000000000 ) ) ;
#96594=CARTESIAN_POINT ( 'NONE',  ( 70.76287552252175317, 61.08876315251507805, -14.44714046989205691 ) ) ;
#96595=CARTESIAN_POINT ( 'NONE',  ( 7.821713311501573784, 19.91421378149916421, 9.188101187500008038 ) ) ;
#96596=ORIENTED_EDGE ( 'NONE', *, *, #78944, .F. ) ;
#96598=ORIENTED_EDGE ( 'NONE', *, *, #91502, .F. ) ;
#96607=CARTESIAN_POINT ( 'NONE',  ( 84.64118529441607564, 42.23213341487252848, 1.449458229959814881 ) ) ;
#96608=CARTESIAN_POINT ( 'NONE',  ( 88.29906409831174585, 44.33258913401337509, -2.209727062603330516 ) ) ;
#96611=CARTESIAN_POINT ( 'NONE',  ( 66.01596945876833900, 69.23916865775863982, 0.2712613576453007935 ) ) ;
#96619=CARTESIAN_POINT ( 'NONE',  ( 88.21232870727821762, 44.34776898565001346, 2.631490070295979145 ) ) ;
#96622=CARTESIAN_POINT ( 'NONE',  ( 76.82263189186275554, 60.88017539376242837, -15.71791450812036395 ) ) ;
#96623=CARTESIAN_POINT ( 'NONE',  ( 80.47309446435835412, 57.88546628059901167, 16.25201728225186315 ) ) ;
#96624=CARTESIAN_POINT ( 'NONE',  ( 71.79012238242354726, 65.93304147633399737, -12.01195568269040947 ) ) ;
#96630=CARTESIAN_POINT ( 'NONE',  ( 87.77887691218910504, 44.16646017302762317, -4.484802941535590115 ) ) ;
#96633=B_SPLINE_CURVE_WITH_KNOTS ( 'NONE', 3,
 ( #50290, #17394, #56887, #41686, #87870, #48306, #25499, #40684, #48814, #33099, #63996, #79747, #56391, #87387, #10309, #18416, #72629, #3230, #95950, #66490, #43170, #89833, #59875, #27512 ),
 .UNSPECIFIED., .F., .F.,
 ( 4, 2, 2, 2, 2, 2, 2, 2, 2, 2, 2, 4 ),
 ( 0.000000000000000000, 0.1250000000000107692, 0.2500000000000215383, 0.3750000000000323075, 0.4375000000000291434, 0.5000000000000259792, 0.5625000000000227596, 0.6250000000000196509, 0.6875000000000164313, 0.7500000000000133227, 0.8750000000000066613, 1.000000000000000000 ),
 .UNSPECIFIED. ) ;
#96635=CARTESIAN_POINT ( 'NONE',  ( 76.40735639740501028, 51.42921241913779085, 15.62223202341787598 ) ) ;
#96640=CARTESIAN_POINT ( 'NONE',  ( 84.32075484545329402, 50.66451156707553594, 13.78810211404426411 ) ) ;
#96642=CARTESIAN_POINT ( 'NONE',  ( 75.82692561157452360, 55.11882190618480593, -16.59949335850286545 ) ) ;
#96647=CARTESIAN_POINT ( 'NONE',  ( 84.55537670905214043, 50.62155581810768012, -14.09136642048690291 ) ) ;
#96651=CARTESIAN_POINT ( 'NONE',  ( 75.58214075417596689, 65.23491603964200181, 14.35294216029142333 ) ) ;
#96653=CARTESIAN_POINT ( 'NONE',  ( 32.78250297933140445, 27.43085787977765122, -9.188101187500008038 ) ) ;
#96655=CARTESIAN_POINT ( 'NONE',  ( 75.63520882045094140, 61.37380848085838636, 15.84745159558423744 ) ) ;
#96657=CARTESIAN_POINT ( 'NONE',  ( 13.78045586392592092, 26.14336893147754282, 7.433330006724141015 ) ) ;
#96661=CARTESIAN_POINT ( 'NONE',  ( 86.57431924022760938, 47.22157117268152149, 10.65071021778218352 ) ) ;
#96663=CARTESIAN_POINT ( 'NONE',  ( 72.09375247312608792, 71.41439723707200926, 5.090740936595467225 ) ) ;
#96664=CARTESIAN_POINT ( 'NONE',  ( 87.28672817441044174, 44.98879080050047463, -6.213673670119491454 ) ) ;
#96668=CARTESIAN_POINT ( 'NONE',  ( 74.82815960207534545, 53.36537385475131856, 16.05773697466056404 ) ) ;
#96677=CARTESIAN_POINT ( 'NONE',  ( 89.11175791728626905, 45.37822637883662225, 1.911324073694122932E-15 ) ) ;
#96679=CARTESIAN_POINT ( 'NONE',  ( 71.94643353573427191, 71.53214566342799685, 5.625104812542565114 ) ) ;
#96680=CARTESIAN_POINT ( 'NONE',  ( 13.83268420227240014, 8.390406791769812855, -2.889640176918245968E-15 ) ) ;
#96684=CARTESIAN_POINT ( 'NONE',  ( 25.67147243227365649, 35.79752408145593989, -5.678558825948271327 ) ) ;
#96685=CARTESIAN_POINT ( 'NONE',  ( 79.97511216739995632, 58.10444404117469475, -16.24719292606884125 ) ) ;
#96689=ORIENTED_EDGE ( 'NONE', *, *, #82701, .T. ) ;
#96690=VERTEX_POINT ( 'NONE', #74246 ) ;
#96692=CARTESIAN_POINT ( 'NONE',  ( 68.17866407165988107, 65.83321247030521306, 10.84866537784224327 ) ) ;
#96694=CARTESIAN_POINT ( 'NONE',  ( 85.88643775857894980, 48.50416193104786799, 12.18167088616390537 ) ) ;
#96698=B_SPLINE_CURVE_WITH_KNOTS ( 'NONE', 3,
 ( #2909, #56570, #33803, #95636, #88045, #18089, #79923, #18593, #64686, #50962, #66178, #72813, #58560, #64177, #10483, #41361, #96124, #73783, #80936, #65174, #9991, #97122, #26678, #95126, #88539, #19102, #49981, #87557, #11505, #72302, #42359, #3883, #11990, #27690, #26185, #49471, #96622, #89531, #27187, #40852, #58075, #89056, #19606, #50466, #81418, #42847 ),
 .UNSPECIFIED., .F., .F.,
 ( 4, 1, 1, 1, 2, 2, 1, 1, 1, 2, 2, 1, 1, 2, 2, 1, 1, 2, 2, 1, 1, 2, 2, 1, 2, 2, 1, 2, 2, 4 ),
 ( 0.000000000000000000, 0.06250000000003216871, 0.09375000000004683753, 0.1093750000000559830, 0.1171875000000583283, 0.1250000000000606737, 0.1875000000000799083, 0.2187500000000895950, 0.2343750000000944522, 0.2421875000000950351, 0.2500000000000955902, 0.3125000000001050271, 0.3437500000001079137, 0.3593750000001077471, 0.3750000000001075806, 0.4375000000000972000, 0.4687500000000917599, 0.4843750000000913158, 0.5000000000000908162, 0.5625000000000797140, 0.5937500000000740519, 0.6093750000000709433, 0.6250000000000678346, 0.6875000000000563993, 0.7187500000000501821, 0.7500000000000439648, 0.8125000000000323075, 0.8437500000000265343, 0.8750000000000206501, 1.000000000000000000 ),
 .UNSPECIFIED. ) ;
#96708=AXIS2_PLACEMENT_3D ( 'NONE', #94158, #24711, #55594 ) ;
#96709=ORIENTED_EDGE ( 'NONE', *, *, #58865, .F. ) ;
#96710=CARTESIAN_POINT ( 'NONE',  ( 87.09644473823584576, 45.85687564672072369, -8.636203292310963064 ) ) ;
#96712=B_SPLINE_SURFACE_WITH_KNOTS ( 'NONE', 3, 1, ( 
 ( #40166, #32588 ),
 ( #10801, #95939 ),
 ( #94424, #40672 ),
 ( #41169, #71610 ),
 ( #18402, #2710 ),
 ( #41674, #87376 ),
 ( #63984, #25487 ),
 ( #72107, #33597 ),
 ( #64492, #95453 ),
 ( #49294, #26005 ),
 ( #80234, #72618 ),
 ( #3220, #34105 ),
 ( #80746, #96430 ),
 ( #58371, #73596 ),
 ( #59351, #82232 ),
 ( #26994, #50771 ),
 ( #66478, #5674 ),
 ( #57879, #88857 ),
 ( #35583, #89347 ),
 ( #4177, #19423 ),
 ( #81722, #35076 ),
 ( #89821, #43158 ),
 ( #12299, #82729 ),
 ( #36067, #66966 ),
 ( #74098, #90327 ),
 ( #18911, #50279 ),
 ( #81231, #58851 ),
 ( #96934, #65981 ),
 ( #27501, #19900 ),
 ( #97404, #74612 ),
 ( #27973, #20397 ) ),
 .UNSPECIFIED., .F., .F., .F.,
 ( 4, 3, 3, 3, 3, 3, 3, 3, 3, 3, 4 ),
 ( 2, 2 ),
 ( 0.000000000000000000, 0.1122669598086711712, 0.2243161639709570498, 0.3396355846219037966, 0.4553962076585047480, 0.5677860799922284096, 0.6749047109689546575, 0.7773884377078235097, 0.8775581155834147884, 0.9782364162377757966, 1.000000000000000000 ),
 ( 0.000000000000000000, 1.000000000000000000 ),
 .UNSPECIFIED. ) ;
#96722=ORIENTED_EDGE ( 'NONE', *, *, #75024, .T. ) ;
#96723=AXIS2_PLACEMENT_3D ( 'NONE', #48041, #86116, #79495 ) ;
#96725=CARTESIAN_POINT ( 'NONE',  ( 29.09658290004530556, 18.92755873383627119, 6.180339887498953466 ) ) ;
#96729=CARTESIAN_POINT ( 'NONE',  ( 69.81243019392555027, 62.22010195957142287, -13.63492759933605036 ) ) ;
#96735=CARTESIAN_POINT ( 'NONE',  ( 82.67311241900212337, 40.57720724764539000, -1.428110901475119432 ) ) ;
#96736=CARTESIAN_POINT ( 'NONE',  ( 80.47598030042951223, 43.56226889263761848, 9.740817512588815674 ) ) ;
#96742=DIRECTION ( 'NONE',  ( -0.8660254037844379305, -0.5000000000000014433, -0.000000000000000000 ) ) ;
#96743=CARTESIAN_POINT ( 'NONE',  ( 80.50140447660758980, 52.45483312604073234, 15.35925353569622942 ) ) ;
#96747=CARTESIAN_POINT ( 'NONE',  ( 78.31186438638634684, 61.61641173835174357, 16.15355831358047922 ) ) ;
#96751=CARTESIAN_POINT ( 'NONE',  ( 36.34934470066777834, 21.39040679176985194, 1.333680081654574804E-15 ) ) ;
#96752=CARTESIAN_POINT ( 'NONE',  ( 74.26908450914415027, 55.21978062604117099, 16.60372121789527355 ) ) ;
#96753=CARTESIAN_POINT ( 'NONE',  ( 9.015913755055775525, 20.90829794293878763, 10.00000000000000355 ) ) ;
#96754=CARTESIAN_POINT ( 'NONE',  ( 36.70787689013189947, 33.14441083166263979, 10.00000000000000533 ) ) ;
#96757=CARTESIAN_POINT ( 'NONE',  ( 85.64394211879633190, 43.47961218390750560, -4.674786408818643935 ) ) ;
#96761=ORIENTED_EDGE ( 'NONE', *, *, #92636, .F. ) ;
#96767=CARTESIAN_POINT ( 'NONE',  ( 82.30672826452196489, 41.36268747567339688, 5.465017951912414240 ) ) ;
#96772=CARTESIAN_POINT ( 'NONE',  ( 28.69010979082973023, 40.65659080271451842, -1.878358725466461243E-16 ) ) ;
#96777=CARTESIAN_POINT ( 'NONE',  ( 72.79498119441143444, 67.60180456977322194, -11.11215744783703308 ) ) ;
#96781=EDGE_CURVE ( 'NONE', #81326, #83225, #88997, .T. ) ;
#96787=CARTESIAN_POINT ( 'NONE',  ( 36.09163463545626627, 29.03677371833803988, 10.00000000000000533 ) ) ;
#96790=ORIENTED_EDGE ( 'NONE', *, *, #36113, .T. ) ;
#96793=CARTESIAN_POINT ( 'NONE',  ( 67.00800788680665221, 66.91027394849365351, -8.787034667612781291 ) ) ;
#96794=ADVANCED_FACE ( 'NONE', ( #4308 ), #27635, .T. ) ;
#96799=CARTESIAN_POINT ( 'NONE',  ( 25.29680607046014984, 36.64646525600391413, -2.839279412974133887 ) ) ;
#96804=CARTESIAN_POINT ( 'NONE',  ( 19.64056747690256088, 19.84335787977762777, 9.188101187500006262 ) ) ;
#96807=CARTESIAN_POINT ( 'NONE',  ( 11.58252532646001498, 30.18528772668517135, -1.583844403245363575 ) ) ;
#96813=VERTEX_POINT ( 'NONE', #20032 ) ;
#96821=CARTESIAN_POINT ( 'NONE',  ( 77.96041703586088545, 62.15569039082562597, -15.98643159653562940 ) ) ;
#96829=CARTESIAN_POINT ( 'NONE',  ( 30.25658917092484756, 35.65586893147758474, -7.433330006724137462 ) ) ;
#96831=CARTESIAN_POINT ( 'NONE',  ( 75.16089758350406669, 66.39091360267232744, -13.15879276033818535 ) ) ;
#96837=ORIENTED_EDGE ( 'NONE', *, *, #55293, .T. ) ;
#96838=CARTESIAN_POINT ( 'NONE',  ( 82.41933087055697627, 40.38430946167127189, -0.8419157719606927825 ) ) ;
#96847=CARTESIAN_POINT ( 'NONE',  ( 79.05688537879109390, 48.64051310273040230, 14.69164152319516425 ) ) ;
#96857=CARTESIAN_POINT ( 'NONE',  ( 83.38112233772677939, 44.18327968967634689, -8.473636281462212594 ) ) ;
#96859=ADVANCED_FACE ( 'NONE', ( #31087 ), #6806, .T. ) ;
#96862=CARTESIAN_POINT ( 'NONE',  ( 73.81300068619336230, 56.52063054796119701, 16.05668348448922345 ) ) ;
#96865=CARTESIAN_POINT ( 'NONE',  ( 77.05652628499306900, 57.63148023862245850, 16.16682221975541722 ) ) ;
#96876=CARTESIAN_POINT ( 'NONE',  ( 18.32728854387591610, 18.78052372038640172, -10.00000000000000355 ) ) ;
#96893=CARTESIAN_POINT ( 'NONE',  ( 22.75024936130811426, 12.94473085651391742, 1.475505719884397138E-15 ) ) ;
#96894=CARTESIAN_POINT ( 'NONE',  ( 67.91028321870373929, 65.38586328950580651, -10.41284464168438006 ) ) ;
#96898=CARTESIAN_POINT ( 'NONE',  ( 73.89677966998817737, 55.37416586069887359, -16.11664339955940761 ) ) ;
#96904=ADVANCED_FACE ( 'NONE', ( #60483 ), #64514, .T. ) ;
#96911=CARTESIAN_POINT ( 'NONE',  ( 32.83301474718356161, 37.14336893147758900, 7.433330006724141015 ) ) ;
#96915=EDGE_CURVE ( 'NONE', #66013, #91598, #16397, .T. ) ;
#96920=CARTESIAN_POINT ( 'NONE',  ( 6.618913549016022912, 24.79752408145590081, -5.678558825948271327 ) ) ;
#96922=CARTESIAN_POINT ( 'NONE',  ( 20.82171660429349558, 14.94754757982089366, 5.678558825948272215 ) ) ;
#96928=CARTESIAN_POINT ( 'NONE',  ( 24.66009930550170282, 22.43677371833801715, -10.00000000000000355 ) ) ;
#96934=CARTESIAN_POINT ( 'NONE',  ( 66.55830361311562626, 68.75215758827378920, 4.754528328751027821 ) ) ;
#96935=CARTESIAN_POINT ( 'NONE',  ( 87.57478309584621456, 45.08285526713719094, 6.924932389716523140 ) ) ;
#96940=CARTESIAN_POINT ( 'NONE',  ( 80.93613592869992601, 42.95327845849681836, -9.503115154567232992 ) ) ;
#96942=EDGE_LOOP ( 'NONE', ( #22622, #48856, #3611, #6191 ) ) ;
#96943=CARTESIAN_POINT ( 'NONE',  ( 77.06387632225415985, 54.00152061585258423, 16.01168232074038400 ) ) ;
#96946=CARTESIAN_POINT ( 'NONE',  ( 31.53257425345116260, 33.90829794293883026, 10.00000000000000355 ) ) ;
#96947=CARTESIAN_POINT ( 'NONE',  ( 88.53016884517781193, 43.88792164385783678, -0.09627500500477675915 ) ) ;
#96949=VECTOR ( 'NONE', #75044, 1000.000000000000114 ) ;
#96954=CARTESIAN_POINT ( 'NONE',  ( 73.42974959722798189, 58.60376009667394470, 15.71314503368921223 ) ) ;
#96959=EDGE_LOOP ( 'NONE', ( #15852, #18913, #30603, #73724 ) ) ;
#96969=B_SPLINE_CURVE_WITH_KNOTS ( 'NONE', 3,
 ( #39746, #33559, #18364, #41638, #87825, #49259, #80195, #3187 ),
 .UNSPECIFIED., .F., .F.,
 ( 4, 2, 2, 4 ),
 ( 0.0003401861652890088511, 0.0006945731674992995652, 0.0008717666686044522406, 0.001048960169709604916 ),
 .UNSPECIFIED. ) ;
#96973=CARTESIAN_POINT ( 'NONE',  ( 78.05978962947867217, 56.61574962749410389, -16.20259432744737538 ) ) ;
#96978=ORIENTED_EDGE ( 'NONE', *, *, #73160, .F. ) ;
#96982=CARTESIAN_POINT ( 'NONE',  ( 9.850474518891140008, 29.18528772668516424, -1.583844403245363575 ) ) ;
#96984=LINE ( 'NONE', #50330, #28849 ) ;
#97003=CARTESIAN_POINT ( 'NONE',  ( 14.11247099069668742, 31.08080186712592052, -3.090169943749475845 ) ) ;
#97006=CARTESIAN_POINT ( 'NONE',  ( 71.28802077240882795, 71.71698159252220250, -1.887932162199749575 ) ) ;
#97007=EDGE_CURVE ( 'NONE', #36817, #4740, #36019, .T. ) ;
#97011=CARTESIAN_POINT ( 'NONE',  ( 74.05623475345208817, 67.87786276047000911, -11.59565021290447362 ) ) ;
#97015=CARTESIAN_POINT ( 'NONE',  ( 78.98660877947108361, 59.42842565914680364, -16.52762269555200447 ) ) ;
#97019=CARTESIAN_POINT ( 'NONE',  ( 72.79894534421404728, 70.83549005279604671, -7.921956013610877534 ) ) ;
#97025=CARTESIAN_POINT ( 'NONE',  ( 69.07701453075964082, 68.10981339309213922, 7.918463574440547603 ) ) ;
#97032=CARTESIAN_POINT ( 'NONE',  ( 22.15746398174156440, 34.83396525600390703, -2.839279412974133887 ) ) ;
#97036=CARTESIAN_POINT ( 'NONE',  ( 74.62796085038830540, 66.91441896689961766, 13.03852793085608219 ) ) ;
#97038=CARTESIAN_POINT ( 'NONE',  ( 22.16161828121410338, 13.76426979415089491, 3.090169943749476733 ) ) ;
#97039=ORIENTED_EDGE ( 'NONE', *, *, #65851, .T. ) ;
#97042=CARTESIAN_POINT ( 'NONE',  ( 82.27644995706197051, 41.26364417930392392, -3.466983432302654045 ) ) ;
#97044=CARTESIAN_POINT ( 'NONE',  ( 81.22979812886450190, 55.45288652294036780, -16.34461090620094126 ) ) ;
#97046=CARTESIAN_POINT ( 'NONE',  ( 69.17486568141271164, 67.30733642665069283, 9.082494864214003982 ) ) ;
#97048=EDGE_CURVE ( 'NONE', #23100, #81391, #13094, .T. ) ;
#97049=CARTESIAN_POINT ( 'NONE',  ( 83.07333702396124409, 41.93452038489549949, 4.251322240599892943 ) ) ;
#97050=CARTESIAN_POINT ( 'NONE',  ( 79.60424370460739851, 51.75532430349682755, 15.26378781416301500 ) ) ;
#97052=CARTESIAN_POINT ( 'NONE',  ( 70.46850514343660166, 71.36849393383423035, 0.3238707985676339551 ) ) ;
#97055=CARTESIAN_POINT ( 'NONE',  ( 10.70626499057286196, 14.38052372038638893, 10.00000000000000533 ) ) ;
#97058=CARTESIAN_POINT ( 'NONE',  ( 74.30221102045693726, 55.25029599878391195, 16.60364296989904176 ) ) ;
#97063=CARTESIAN_POINT ( 'NONE',  ( 78.94581588320816934, 59.75573664777502358, 16.49495449398541780 ) ) ;
#97066=ORIENTED_EDGE ( 'NONE', *, *, #47844, .F. ) ;
#97069=CARTESIAN_POINT ( 'NONE',  ( 84.06819687104101035, 49.97680779115592031, -13.47026326439832467 ) ) ;
#97070=CARTESIAN_POINT ( 'NONE',  ( 84.54034743127247964, 49.80906814226769086, -13.21523024495328968 ) ) ;
#97071=CARTESIAN_POINT ( 'NONE',  ( 81.25722694078321240, 42.23628214981317797, -7.275039830697891396 ) ) ;
#97076=CARTESIAN_POINT ( 'NONE',  ( 76.92873890057782660, 49.89429371730488327, 15.13083596839045519 ) ) ;
#97078=CARTESIAN_POINT ( 'NONE',  ( 75.59343510720033521, 61.64003300003175667, 15.32494136272226548 ) ) ;
#97081=EDGE_LOOP ( 'NONE', ( #50275, #59542, #8588, #37910 ) ) ;
#97082=CARTESIAN_POINT ( 'NONE',  ( 82.23229681800175683, 40.64091623807065901, 3.329097291065063136 ) ) ;
#97083=CARTESIAN_POINT ( 'NONE',  ( 81.04961468568201610, 43.68546784643918812, -9.492462169003031747 ) ) ;
#97090=EDGE_LOOP ( 'NONE', ( #21865, #17387, #66754, #3857 ) ) ;
#97091=CARTESIAN_POINT ( 'NONE',  ( 75.93938602863309484, 55.94919493231355290, 16.15023845270562930 ) ) ;
#97092=CARTESIAN_POINT ( 'NONE',  ( 8.259543914800127951, 22.95586893147753571, 7.433330006724141015 ) ) ;
#97094=AXIS2_PLACEMENT_3D ( 'NONE', #62172, #61682, #79441 ) ;
#97100=VECTOR ( 'NONE', #53700, 1000.000000000000114 ) ;
#97101=CARTESIAN_POINT ( 'NONE',  ( 76.22863942704391604, 65.23707805566866114, -14.13549428706411781 ) ) ;
#97105=CARTESIAN_POINT ( 'NONE',  ( 84.90109790862749151, 42.41940689311433488, 1.808878322148949280 ) ) ;
#97106=CARTESIAN_POINT ( 'NONE',  ( 88.35080703960181836, 43.95228889933407856, -2.194260235337642140 ) ) ;
#97109=CARTESIAN_POINT ( 'NONE',  ( 66.40060581361414904, 68.91289971205782194, 0.07367910596505218568 ) ) ;
#97118=CARTESIAN_POINT ( 'NONE',  ( 88.23123598884963315, 44.35170718015631053, 2.587891364668495342 ) ) ;
#97122=CARTESIAN_POINT ( 'NONE',  ( 73.74770275411985665, 61.89915078644302326, -14.85475798109034606 ) ) ;
#97123=CARTESIAN_POINT ( 'NONE',  ( 80.24843660680971880, 58.09750880718839028, 16.26407653974109024 ) ) ;
#97127=CARTESIAN_POINT ( 'NONE',  ( 67.16990927169524639, 66.79708245693809943, -9.067759095298582039 ) ) ;
#97130=CARTESIAN_POINT ( 'NONE',  ( 80.76990913474571698, 43.05389971685210782, -9.742651082411008190 ) ) ;
#97134=DIRECTION ( 'NONE',  ( -0.2503889871761760255, -0.9681453171404016400, 0.000000000000000000 ) ) ;
#97140=CARTESIAN_POINT ( 'NONE',  ( 84.98383346588632037, 50.06751842512129258, 13.63401461718180485 ) ) ;
#97151=CARTESIAN_POINT ( 'NONE',  ( 84.75337437632948934, 42.49783821425369723, -2.788419914845409853 ) ) ;
#97152=CARTESIAN_POINT ( 'NONE',  ( 76.11661262897267477, 65.38883171293761620, 14.43021505105784819 ) ) ;
#97154=CARTESIAN_POINT ( 'NONE',  ( 38.69009612255265296, 24.19860640527295104, 2.839279412974134775 ) ) ;
#97158=CARTESIAN_POINT ( 'NONE',  ( 21.85012855468117721, 24.56628583063841376, 9.188101187500006262 ) ) ;
#97162=CARTESIAN_POINT ( 'NONE',  ( 70.62351716309591154, 60.91279443485260714, 15.01748476286653933 ) ) ;
#97168=CARTESIAN_POINT ( 'NONE',  ( 74.84467759388789432, 53.32343055176874458, 16.53062654614232230 ) ) ;
#97170=CARTESIAN_POINT ( 'NONE',  ( 85.58519120388885426, 46.64559940333228383, 10.07285853436253120 ) ) ;
#97173=CARTESIAN_POINT ( 'NONE',  ( 86.46877025260693017, 44.29843151041793448, 5.647966490367202219 ) ) ;
#97177=CARTESIAN_POINT ( 'NONE',  ( 72.27003297432077034, 71.75159315020286499, 5.546042747704600373 ) ) ;
#97183=CARTESIAN_POINT ( 'NONE',  ( 27.40352323984253857, 36.79752408145593279, -5.678558825948271327 ) ) ;
#97189=DIRECTION ( 'NONE',  ( -0.5778974349098243701, -0.4186690413702435221, 0.7005360722495073134 ) ) ;
#97190=CARTESIAN_POINT ( 'NONE',  ( 68.34875839458671010, 65.66236861316339457, 10.38748295948464140 ) ) ;
#97192=CARTESIAN_POINT ( 'NONE',  ( 85.74188846148156529, 48.75224078981592157, -11.97363005349371079 ) ) ;
#97201=ORIENTED_EDGE ( 'NONE', *, *, #88805, .T. ) ;
#97219=CARTESIAN_POINT ( 'NONE',  ( 82.23427998234210179, 44.55295170538099114, 9.756742293097531160 ) ) ;
#97226=CARTESIAN_POINT ( 'NONE',  ( 82.52124186608902789, 40.48930152589419862, -1.425869482907266450 ) ) ;
#97230=DIRECTION ( 'NONE',  ( 0.2033683215378999376, -0.3522442655536480172, -0.9135454576426004225 ) ) ;
#97233=CARTESIAN_POINT ( 'NONE',  ( 80.51961122738369170, 52.55551232112726012, 15.38693572438338464 ) ) ;
#97240=CARTESIAN_POINT ( 'NONE',  ( 31.78235740255998820, 30.30066082961423746, -10.00000000000000533 ) ) ;
#97241=CARTESIAN_POINT ( 'NONE',  ( 80.06694460085255116, 44.56748078928367818, -11.69919935169422764 ) ) ;
#97243=CARTESIAN_POINT ( 'NONE',  ( 7.614983434379491101, 23.13478043621386249, 8.090169943749478065 ) ) ;
#97244=CARTESIAN_POINT ( 'NONE',  ( 36.68702710410599366, 29.38052372038643867, 10.00000000000000533 ) ) ;
#97248=CARTESIAN_POINT ( 'NONE',  ( 84.59746252465258465, 43.34080150004616883, -5.792757565574923717 ) ) ;
#97254=CARTESIAN_POINT ( 'NONE',  ( 87.36774593059779193, 45.94567951850589083, 8.539250186115692642 ) ) ;
#97255=CARTESIAN_POINT ( 'NONE',  ( 23.89366908878298190, 14.76426979415089846, 3.090169943749476733 ) ) ;
#97257=CARTESIAN_POINT ( 'NONE',  ( 86.84204249716189850, 45.92435628226732547, 8.934002094794735171 ) ) ;
#97260=CARTESIAN_POINT ( 'NONE',  ( 39.59743582264582784, 38.56454794089045635, 10.00000000000000355 ) ) ;
#97265=CARTESIAN_POINT ( 'NONE',  ( 67.85574724824152781, 67.82218689132628242, -7.169315664176491687 ) ) ;
#97276=CARTESIAN_POINT ( 'NONE',  ( 67.29236409614540548, 66.61846781487172109, -8.519670054875607690 ) ) ;
#97281=CARTESIAN_POINT ( 'NONE',  ( 29.13557404741141355, 37.79752408145594700, -5.678558825948271327 ) ) ;
#97283=CARTESIAN_POINT ( 'NONE',  ( 86.38615641404119572, 47.55643641724976334, -10.55640884279900327 ) ) ;
#97287=CARTESIAN_POINT ( 'NONE',  ( 14.74991654177707900, 23.91421378149918198, 9.188101187500008038 ) ) ;
#97292=CARTESIAN_POINT ( 'NONE',  ( 76.98982937314906394, 56.23836901630515683, 16.60980887848485921 ) ) ;
#97296=VERTEX_POINT ( 'NONE', #42917 ) ;
#97298=DIRECTION ( 'NONE',  ( -0.2633726137851614135, -0.9634420117996742583, -0.04913609882121805494 ) ) ;
#97300=CARTESIAN_POINT ( 'NONE',  ( 66.28447348300909425, 69.23781496131373103, -2.133696438910710480 ) ) ;
#97302=LINE ( 'NONE', #66861, #61283 ) ;
#97303=CARTESIAN_POINT ( 'NONE',  ( 78.18465668123985779, 61.71620641638569538, -16.11691968629958183 ) ) ;
#97304=ADVANCED_FACE ( 'NONE', ( #81990 ), #43437, .F. ) ;
#97316=CARTESIAN_POINT ( 'NONE',  ( 81.59396048808834223, 55.93895065387218324, 16.03242832552846053 ) ) ;
#97336=ADVANCED_FACE ( 'NONE', ( #28746 ), #83480, .T. ) ;
#97339=CARTESIAN_POINT ( 'NONE',  ( 74.60895917517520104, 60.22888921480863189, 15.54340603921727748 ) ) ;
#97343=CARTESIAN_POINT ( 'NONE',  ( 76.76894470656165481, 55.99379639269752573, 16.17573251806829404 ) ) ;
#97348=EDGE_CURVE ( 'NONE', #26159, #27875, #1047, .T. ) ;
#97349=CARTESIAN_POINT ( 'NONE',  ( 73.38874485642215006, 69.17140463384058080, -9.961793831881072592 ) ) ;
#97352=CARTESIAN_POINT ( 'NONE',  ( 70.15174361226061706, 71.00165729854369090, 2.050894468748571509 ) ) ;
#97355=CARTESIAN_POINT ( 'NONE',  ( 25.07769263752670597, 14.28848085856231798, 1.475505719884397138E-15 ) ) ;
#97370=CARTESIAN_POINT ( 'NONE',  ( 83.86224871339140918, 42.07689945840732548, 4.987215453410938970 ) ) ;
#97371=CARTESIAN_POINT ( 'NONE',  ( 28.83231091828818649, 21.81029122506295792, 8.090169943749479842 ) ) ;
#97372=CARTESIAN_POINT ( 'NONE',  ( 85.30407614177579489, 48.45294084599412088, 12.40582119231524949 ) ) ;
#97375=CARTESIAN_POINT ( 'NONE',  ( 73.83769579401584338, 55.54879188763737830, -16.58599655330451128 ) ) ;
#97383=CARTESIAN_POINT ( 'NONE',  ( 72.76446422349046372, 71.15534465558161514, -7.354170587574377471 ) ) ;
#97384=CARTESIAN_POINT ( 'NONE',  ( 79.11589578886889740, 60.05912704548522640, 16.12809997863940836 ) ) ;
#97385=CARTESIAN_POINT ( 'NONE',  ( 27.72828276626169952, 36.98502408145593989, -5.678558825948271327 ) ) ;
#97391=CARTESIAN_POINT ( 'NONE',  ( 9.708348802340269756, 27.64646525600388571, -2.839279412974133887 ) ) ;
#97393=CARTESIAN_POINT ( 'NONE',  ( 82.92115063973837152, 53.64018987990929332, 15.71948723892795741 ) ) ;
#97396=DIRECTION ( 'NONE',  ( -0.8660254037844378194, -0.5000000000000014433, -0.000000000000000000 ) ) ;
#97399=CARTESIAN_POINT ( 'NONE',  ( 81.10384738341275579, 42.53340397202252632, 7.902204148537900430 ) ) ;
#97404=CARTESIAN_POINT ( 'NONE',  ( 66.56647152974866799, 68.76039119326856053, 4.744323796004452198 ) ) ;
#97412=ORIENTED_EDGE ( 'NONE', *, *, #28697, .T. ) ;
#97414=CARTESIAN_POINT ( 'NONE',  ( 80.41065583177754661, 57.49148768039361812, -16.58946210043120217 ) ) ;
#97416=ORIENTED_EDGE ( 'NONE', *, *, #28447, .T. ) ;
#97420=CARTESIAN_POINT ( 'NONE',  ( 81.05146334655599105, 43.66063824279576266, 9.461398633974173578 ) ) ;
#97425=VERTEX_POINT ( 'NONE', #19675 ) ;
#97428=ORIENTED_EDGE ( 'NONE', *, *, #90756, .T. ) ;
#97429=EDGE_CURVE ( 'NONE', #33116, #84611, #46793, .T. ) ;
#97435=CARTESIAN_POINT ( 'NONE',  ( 87.88857223635071136, 44.01828834560762971, 1.459818322210690189 ) ) ;
#97438=CARTESIAN_POINT ( 'NONE',  ( 19.46611421548295695, 12.20801979619928090, -3.090169943749474069 ) ) ;
#97443=CARTESIAN_POINT ( 'NONE',  ( 78.98411721334434787, 56.24657107981478532, -16.18231381929481572 ) ) ;
#97451=CARTESIAN_POINT ( 'NONE',  ( 13.83268420227240014, 8.390406791769812855, -2.889640176918245968E-15 ) ) ;
#97455=CARTESIAN_POINT ( 'NONE',  ( 82.02356888928309786, 52.10171163115919057, -14.99001706985075622 ) ) ;
#97457=CARTESIAN_POINT ( 'NONE',  ( 18.45529574749610902, 12.78380873178786281, -6.180339887498949025 ) ) ;
#97460=EDGE_LOOP ( 'NONE', ( #92576, #86773, #57381, #75466 ) ) ;
#97471=CARTESIAN_POINT ( 'NONE',  ( 84.40414035640600332, 50.68119616098906022, 13.77015003724606146 ) ) ;
#97479=CARTESIAN_POINT ( 'NONE',  ( 74.46953068837864009, 68.18058761729560047, -11.53831106377694127 ) ) ;
#97482=DIRECTION ( 'NONE',  ( -0.8660254037844379305, -0.5000000000000014433, -0.000000000000000000 ) ) ;
#97485=CARTESIAN_POINT ( 'NONE',  ( 73.80638704669730998, 68.31061168272385942, -11.57820046455322505 ) ) ;
#97489=CARTESIAN_POINT ( 'NONE',  ( 79.28302063466354355, 59.54490948036851705, -16.53220260971268374 ) ) ;
#97494=DIRECTION ( 'NONE',  ( -0.8660254037844378194, -0.5000000000000014433, -0.000000000000000000 ) ) ;
#97495=CARTESIAN_POINT ( 'NONE',  ( 66.30989429470714924, 68.09514072150794561, -4.585047217807751707 ) ) ;
#97498=CARTESIAN_POINT ( 'NONE',  ( 72.50080294041131879, 57.38314053816311855, 15.83417486949919351 ) ) ;
#97499=CARTESIAN_POINT ( 'NONE',  ( 69.20114864676770594, 68.32048725079164342, 7.706386681980674780 ) ) ;
#97505=CARTESIAN_POINT ( 'NONE',  ( 20.05074681235918277, 34.68290643055188127, 3.479690158560446702E-15 ) ) ;
#97509=DIRECTION ( 'NONE',  ( 0.03487823687205911238, -0.06041087834082882468, 0.9975640502598247528 ) ) ;
#97510=CARTESIAN_POINT ( 'NONE',  ( 75.25521838011508180, 66.92519264401985879, 13.27308740013157085 ) ) ;
#97520=AXIS2_PLACEMENT_3D ( 'NONE', #53717, #60317, #92285 ) ;
#97523=CARTESIAN_POINT ( 'NONE',  ( 72.06430047377128290, 72.31697432814085857, 0.7629622467667349639 ) ) ;
#97524=B_SPLINE_SURFACE_WITH_KNOTS ( 'NONE', 3, 1, ( 
 ( #39531, #14267 ),
 ( #1066, #91301 ),
 ( #994, #47580 ),
 ( #2507, #87165 ),
 ( #55662, #88153 ),
 ( #40474, #1996 ),
 ( #40961, #33389 ),
 ( #10097, #55171 ),
 ( #18201, #16689 ),
 ( #47084, #63286 ),
 ( #71906, #26298 ),
 ( #64291, #49095 ),
 ( #70386, #71406 ),
 ( #94723, #24295 ),
 ( #24780, #95240 ),
 ( #17697, #9093 ),
 ( #9611, #25809 ),
 ( #33911, #95745 ),
 ( #48600, #32882 ),
 ( #57173, #79539 ),
 ( #17179, #56684 ),
 ( #64800, #78004 ),
 ( #87667, #31874 ),
 ( #86649, #80030 ),
 ( #1507, #8596 ),
 ( #78508, #39964 ),
 ( #10598, #48081 ),
 ( #41471, #72419 ),
 ( #70900, #3023 ),
 ( #39461, #62777 ),
 ( #93735, #86156 ) ),
 .UNSPECIFIED., .F., .F., .F.,
 ( 4, 3, 3, 3, 3, 3, 3, 3, 3, 3, 4 ),
 ( 2, 2 ),
 ( 0.000000000000000000, 0.1333490885032314888, 0.3007194338854323190, 0.4699862290245113150, 0.5844252810809227316, 0.6686540514502676835, 0.7354980260655422653, 0.8028463152565505911, 0.8633854507757149355, 0.9437142632667404607, 1.000000000000000000 ),
 ( 0.000000000000000000, 1.000000000000000000 ),
 .UNSPECIFIED. ) ;
#97525=CARTESIAN_POINT ( 'NONE',  ( 85.39968305126339487, 44.98980877744030948, 7.996374091334619294 ) ) ;
#97531=CARTESIAN_POINT ( 'NONE',  ( 11.77607482435655051, 8.927558733836240989, 6.180339887498953466 ) ) ;
#97534=CARTESIAN_POINT ( 'NONE',  ( 74.32283972735670829, 55.33658384534070507, 16.60204640374922036 ) ) ;
#97535=CARTESIAN_POINT ( 'NONE',  ( 71.94643353573427191, 71.53214566342799685, 5.625104812542565114 ) ) ;
#97538=EDGE_CURVE ( 'NONE', #49399, #73618, #51640, .T. ) ;
#97541=VECTOR ( 'NONE', #18248, 1000.000000000000227 ) ;
#97543=CARTESIAN_POINT ( 'NONE',  ( 88.42017002704760387, 43.92753743058676719, 1.721442031696316377 ) ) ;
#97544=CARTESIAN_POINT ( 'NONE',  ( 75.14833501749109246, 53.26070039134698675, 16.02921398246552087 ) ) ;
#97548=CARTESIAN_POINT ( 'NONE',  ( 84.47860975560725194, 49.82577972120141396, -13.24615549146050597 ) ) ;
#97556=FACE_OUTER_BOUND ( 'NONE', #81099, .T. ) ;
#97558=CARTESIAN_POINT ( 'NONE',  ( 75.15495416781809013, 59.46171984578271719, 15.76924538335189396 ) ) ;
#97562=CARTESIAN_POINT ( 'NONE',  ( 81.91642347199164931, 41.06807863313601104, 3.527822212322262896 ) ) ;
#97567=CARTESIAN_POINT ( 'NONE',  ( 76.73007396570457672, 60.00601218884718691, 15.86901231296716119 ) ) ;
#97569=CARTESIAN_POINT ( 'NONE',  ( 9.941082954516854642, 14.24335787977761036, -9.188101187500008038 ) ) ;
#97570=ORIENTED_EDGE ( 'NONE', *, *, #21934, .T. ) ;
#97576=CARTESIAN_POINT ( 'NONE',  ( 76.06972881656521679, 64.70592176699422282, -14.35599997814377282 ) ) ;
#97582=ORIENTED_EDGE ( 'NONE', *, *, #97348, .F. ) ;
#97584=CARTESIAN_POINT ( 'NONE',  ( 77.55708701662783255, 61.25438087302521240, -15.77812108083495524 ) ) ;
#97588=EDGE_CURVE ( 'NONE', #89224, #57901, #44260, .T. ) ;
#97594=CARTESIAN_POINT ( 'NONE',  ( 88.22316733864592209, 44.26875609612614682, 2.029272769359140582 ) ) ;
#97603=AXIS2_PLACEMENT_3D ( 'NONE', #48137, #48655, #62318 ) ;
#97611=CARTESIAN_POINT ( 'NONE',  ( 87.79988801543919408, 44.42003386087115757, -3.950855289944771975 ) ) ;
#97613=CARTESIAN_POINT ( 'NONE',  ( 77.87934091665805170, 50.93078553898673988, 15.28564964083246558 ) ) ;
#97614=VECTOR ( 'NONE', #37669, 999.9999999999998863 ) ;
#97615=CARTESIAN_POINT ( 'NONE',  ( 77.04391226188317887, 50.32083652003289842, 15.24994158219132068 ) ) ;
#97619=CARTESIAN_POINT ( 'NONE',  ( 84.20844839706383311, 50.59124878818558813, 13.78330635088765455 ) ) ;
#97628=CARTESIAN_POINT ( 'NONE',  ( 8.064688198948626763, 22.84336893147754211, -7.433330006724137462 ) ) ;
#97633=CARTESIAN_POINT ( 'NONE',  ( 75.76889645089327985, 65.47676480558789081, 14.28475327549652185 ) ) ;
#97634=CARTESIAN_POINT ( 'NONE',  ( 80.22522614674704755, 44.29332910989383265, 11.37138867391942476 ) ) ;
#97635=CARTESIAN_POINT ( 'NONE',  ( 37.36761971798259196, 27.28920272979929607, -7.433330006724141015 ) ) ;
#97638=ORIENTED_EDGE ( 'NONE', *, *, #97843, .T. ) ;
#97639=CARTESIAN_POINT ( 'NONE',  ( 20.70865909420142259, 30.14336893147755703, 7.433330006724141015 ) ) ;
#97645=CARTESIAN_POINT ( 'NONE',  ( 70.37335645893944047, 61.05447394354146695, 14.89803406748600523 ) ) ;
#97650=CARTESIAN_POINT ( 'NONE',  ( 88.24427088181241174, 44.33808775276298775, -2.403621623811780683 ) ) ;
#97652=CARTESIAN_POINT ( 'NONE',  ( 81.53430506435155678, 46.66854249687567346, -12.70094556911029038 ) ) ;
#97655=CARTESIAN_POINT ( 'NONE',  ( 85.39747940901729351, 43.05929300263707660, 3.749131589292365341 ) ) ;
#97656=ORIENTED_EDGE ( 'NONE', *, *, #62450, .F. ) ;
#97657=CARTESIAN_POINT ( 'NONE',  ( 77.09671571037877413, 63.64621968971055566, -15.01522762802964905 ) ) ;
#97665=CARTESIAN_POINT ( 'NONE',  ( 39.54951596113196644, 25.76004757982092741, 5.678558825948272215 ) ) ;
#97666=CARTESIAN_POINT ( 'NONE',  ( 76.63781029191453342, 59.43798239135757910, -15.94570803233245293 ) ) ;
#97669=CARTESIAN_POINT ( 'NONE',  ( 87.57113761115280681, 45.50653608346983248, 6.901679451313498248 ) ) ;
#97673=CARTESIAN_POINT ( 'NONE',  ( 81.31286011338397657, 42.41139741970113164, 7.506920912044924954 ) ) ;
#97676=CARTESIAN_POINT ( 'NONE',  ( 85.72569040894076409, 48.78770323298218869, -12.00764425159951898 ) ) ;
#97681=CARTESIAN_POINT ( 'NONE',  ( 84.14312167556933275, 48.98415679381830756, 0.000000000000000000 ) ) ;
#97690=CARTESIAN_POINT ( 'NONE',  ( 87.20542010897281671, 46.22683608894070062, -9.058801420718495478 ) ) ;
#97700=CARTESIAN_POINT ( 'NONE',  ( 81.30975366074838462, 56.24313983998633404, -16.44754541364717326 ) ) ;
#97702=CARTESIAN_POINT ( 'NONE',  ( 81.96835758032909780, 44.03121486362022807, 9.310397246505914381 ) ) ;
#97708=CARTESIAN_POINT ( 'NONE',  ( 82.00328269441645546, 49.67669804047655902, 13.87900603238908026 ) ) ;
#97713=CARTESIAN_POINT ( 'NONE',  ( 72.08446838866018425, 72.31872904169155447, 3.483634709754478642 ) ) ;
#97715=DIRECTION ( 'NONE',  ( 0.5000000000000014433, -0.8660254037844378194, 0.000000000000000000 ) ) ;
#97716=CARTESIAN_POINT ( 'NONE',  ( 79.65053214023340900, 48.80355187758674873, 14.09044789434124922 ) ) ;
#97717=CARTESIAN_POINT ( 'NONE',  ( 67.98237831623328020, 69.73113656707158725, -1.821194602964219866 ) ) ;
#97720=CARTESIAN_POINT ( 'NONE',  ( 77.77576245277342082, 61.68761876588025217, 16.07113493600748200 ) ) ;
#97724=CARTESIAN_POINT ( 'NONE',  ( 73.34867049892106650, 70.14346970443526175, -9.354907352444854496 ) ) ;
#97725=DIRECTION ( 'NONE',  ( 0.5000000000000014433, -0.8660254037844378194, 0.000000000000000000 ) ) ;
#97726=CARTESIAN_POINT ( 'NONE',  ( 78.60844116473590759, 49.40628642118211644, 15.13497465346012660 ) ) ;
#97727=CARTESIAN_POINT ( 'NONE',  ( 40.15112871924373650, 31.38052372038644933, 10.00000000000000533 ) ) ;
#97728=CARTESIAN_POINT ( 'NONE',  ( 74.42293240810788291, 58.11393764944256191, -16.37586900588139116 ) ) ;
#97730=CARTESIAN_POINT ( 'NONE',  ( 72.29113772080887657, 72.04443532774766368, 3.396961777288337814 ) ) ;
#97733=CARTESIAN_POINT ( 'NONE',  ( 69.98676787869841576, 71.07097491031876757, 3.687581967789058446 ) ) ;
#97740=CARTESIAN_POINT ( 'NONE',  ( 71.61159621314317292, 72.40963678617121957, -1.342178375522450562 ) ) ;
#97742=CARTESIAN_POINT ( 'NONE',  ( 87.37978634506822573, 45.87160741090568905, 8.420816086386249566 ) ) ;
#97745=CARTESIAN_POINT ( 'NONE',  ( 44.43605786102924782, 27.78380873178790722, -6.180339887498949025 ) ) ;
#97749=CARTESIAN_POINT ( 'NONE',  ( 72.94799627050929303, 62.71678750348689846, 14.32205132279771220 ) ) ;
#97750=CARTESIAN_POINT ( 'NONE',  ( 74.02122080984301533, 67.34355054658300332, -11.96938251222216998 ) ) ;
#97751=B_SPLINE_SURFACE_WITH_KNOTS ( 'NONE', 3, 1, ( 
 ( #67147, #34262 ),
 ( #81898, #59023 ),
 ( #43342, #20570 ),
 ( #4358, #89516 ),
 ( #5361, #21079 ),
 ( #34749, #96608 ),
 ( #36241, #27170 ),
 ( #49964, #27675 ),
 ( #43842, #89994 ),
 ( #82895, #3866 ),
 ( #58541, #98069 ),
 ( #73272, #28645 ),
 ( #51448, #65157 ),
 ( #97106, #82416 ),
 ( #59527, #96106 ),
 ( #26663, #57547 ),
 ( #88525, #19085 ),
 ( #73767, #11490 ),
 ( #42343, #58058 ),
 ( #89042, #20074 ),
 ( #19588, #81402 ),
 ( #11972, #42832 ),
 ( #35253, #66159 ),
 ( #50947, #7092 ),
 ( #21800, #37974 ),
 ( #61287, #52685 ),
 ( #45097, #6101 ),
 ( #13228, #66900 ),
 ( #13708, #21312 ),
 ( #99810, #84633 ),
 ( #97829, #83646 ) ),
 .UNSPECIFIED., .F., .F., .F.,
 ( 4, 3, 3, 3, 3, 3, 3, 3, 3, 3, 4 ),
 ( 2, 2 ),
 ( 0.000000000000000000, 0.1333490885032329043, 0.3007194338854308202, 0.4699862290245099827, 0.5844252810809248411, 0.6686540514502534727, 0.7354980260655189506, 0.8028463152565233907, 0.8633854507756654195, 0.9437142632666670750, 1.000000000000000000 ),
 ( 0.000000000000000000, 1.000000000000000000 ),
 .UNSPECIFIED. ) ;
#97753=CARTESIAN_POINT ( 'NONE',  ( 82.41914487369291464, 41.31337197830497132, 3.340431838514237750 ) ) ;
#97755=DIRECTION ( 'NONE',  ( 0.5000000000000014433, -0.8660254037844378194, 0.000000000000000000 ) ) ;
#97762=CARTESIAN_POINT ( 'NONE',  ( 67.33503286408792121, 66.66970121028828089, -8.481744889717480973 ) ) ;
#97767=CARTESIAN_POINT ( 'NONE',  ( 32.78369927745970358, 30.87878583063843863, -9.188101187500006262 ) ) ;
#97772=B_SPLINE_CURVE_WITH_KNOTS ( 'NONE', 3,
 ( #19383, #33558, #49749, #35036, #96894, #33047, #27464, #94885, #10260, #56839 ),
 .UNSPECIFIED., .F., .F.,
 ( 4, 2, 2, 2, 4 ),
 ( 0.000000000000000000, 0.2500000000000000000, 0.5000000000000000000, 0.7500000000000000000, 1.000000000000000000 ),
 .UNSPECIFIED. ) ;
#97773=CARTESIAN_POINT ( 'NONE',  ( 15.13723537722347956, 17.24335787977762280, -9.188101187500008038 ) ) ;
#97776=CARTESIAN_POINT ( 'NONE',  ( 20.18734655506498754, 13.78380873178786459, -6.180339887498949025 ) ) ;
#97778=CARTESIAN_POINT ( 'NONE',  ( 76.19322934838378103, 52.39361190095211640, 16.33354292047609491 ) ) ;
#97791=CARTESIAN_POINT ( 'NONE',  ( 77.77867966053455007, 61.43039905302717330, -16.12786080876373873 ) ) ;
#97796=CARTESIAN_POINT ( 'NONE',  ( 81.70640461168267166, 59.20467455214015473, -0.4951340343707861247 ) ) ;
#97813=CARTESIAN_POINT ( 'NONE',  ( 70.74807497663788070, 64.07295471535329057, -12.85902237599238163 ) ) ;
#97819=CARTESIAN_POINT ( 'NONE',  ( 76.06543009505163866, 51.20229643674512232, -16.10824878130317117 ) ) ;
#97828=CARTESIAN_POINT ( 'NONE',  ( 69.30885647817778761, 67.84364059337893593, -9.314741131470263724 ) ) ;
#97829=CARTESIAN_POINT ( 'NONE',  ( 87.98594423550160570, 43.75089820288620501, -2.253463800273097561 ) ) ;
#97834=CARTESIAN_POINT ( 'NONE',  ( 76.32480335349765710, 53.80613752448550713, 16.04086341519817793 ) ) ;
#97837=CARTESIAN_POINT ( 'NONE',  ( 72.54662768515015614, 71.52720332855409424, -5.424102431521803602 ) ) ;
#97842=CARTESIAN_POINT ( 'NONE',  ( 70.17655873119920784, 71.02233810139671277, 2.012687245299938255 ) ) ;
#97843=EDGE_CURVE ( 'NONE', #5537, #32075, #28670, .T. ) ;
#97844=CARTESIAN_POINT ( 'NONE',  ( 80.01979875032591849, 57.54866692369599690, 16.59896302490740538 ) ) ;
#97845=CARTESIAN_POINT ( 'NONE',  ( 19.38736881444313198, 23.14441083166260782, 10.00000000000000533 ) ) ;
#97853=VERTEX_POINT ( 'NONE', #26529 ) ;
#97859=CARTESIAN_POINT ( 'NONE',  ( 18.71323094475359738, 33.73705186507753950, -3.090169943749475845 ) ) ;
#97860=CARTESIAN_POINT ( 'NONE',  ( 85.41398746878978443, 48.60267188261818916, 12.47190137721841019 ) ) ;
#97875=CARTESIAN_POINT ( 'NONE',  ( 40.03666203415436797, 35.06628583063844928, -9.188101187500006262 ) ) ;
#97879=CARTESIAN_POINT ( 'NONE',  ( 16.77867774916664345, 33.18528772668517490, -1.583844403245363575 ) ) ;
#97883=CARTESIAN_POINT ( 'NONE',  ( 10.08301516415377641, 26.79752408145591147, -5.678558825948271327 ) ) ;
#97889=CARTESIAN_POINT ( 'NONE',  ( 87.27161142932803273, 45.46653660222711579, -7.106486493650752578 ) ) ;
#97894=CARTESIAN_POINT ( 'NONE',  ( 67.05462070971094590, 69.20977875835498594, 1.581595143886974197 ) ) ;
#97904=CARTESIAN_POINT ( 'NONE',  ( 80.16500549515171770, 58.13051307499745235, 16.26618726186349306 ) ) ;
#97907=FACE_OUTER_BOUND ( 'NONE', #49880, .T. ) ;
#97908=EDGE_CURVE ( 'NONE', #13677, #99877, #2739, .T. ) ;
#97912=CARTESIAN_POINT ( 'NONE',  ( 73.78990874245801024, 60.11125809112680685, 15.42103814799846795 ) ) ;
#97925=CARTESIAN_POINT ( 'NONE',  ( 82.95708619573620979, 53.58516627418448053, 15.69712586674409671 ) ) ;
#97930=ORIENTED_EDGE ( 'NONE', *, *, #19483, .F. ) ;
#97931=CARTESIAN_POINT ( 'NONE',  ( 80.66320740626021291, 55.52576771489578533, -16.04266746477125949 ) ) ;
#97933=CARTESIAN_POINT ( 'NONE',  ( 35.24645901769773815, 32.30066082961424456, -10.00000000000000533 ) ) ;
#97942=CARTESIAN_POINT ( 'NONE',  ( 72.42456163296586169, 70.48275826165811964, 7.406847684272648280 ) ) ;
#97943=CARTESIAN_POINT ( 'NONE',  ( 86.16814719413950741, 44.54916269947106144, 7.429840375059775681 ) ) ;
#97950=CARTESIAN_POINT ( 'NONE',  ( 85.56881463994550074, 46.99119872501016459, 11.02191848255706219 ) ) ;
#97958=ADVANCED_FACE ( 'NONE', ( #85884 ), #87403, .T. ) ;
#97959=DIRECTION ( 'NONE',  ( 0.3940053768033583426, -0.6824373310787393843, 0.6156614753256619554 ) ) ;
#97961=EDGE_LOOP ( 'NONE', ( #56633, #39528, #28856, #41702 ) ) ;
#97964=CARTESIAN_POINT ( 'NONE',  ( 71.40111858386666199, 71.76360913945114817, -2.046226491198976039 ) ) ;
#97965=CARTESIAN_POINT ( 'NONE',  ( 82.04258323635852435, 41.40673436471046642, -5.930946022421568209 ) ) ;
#97973=CARTESIAN_POINT ( 'NONE',  ( 73.43762515466688967, 73.52662068827324049, 2.033788753608857291E-15 ) ) ;
#97978=CARTESIAN_POINT ( 'NONE',  ( 14.08999532346373407, 7.944730856513903205, 1.475505719884397138E-15 ) ) ;
#97979=CARTESIAN_POINT ( 'NONE',  ( 79.05889743344327769, 46.07589703579929363, -12.67661131050572720 ) ) ;
#97980=CARTESIAN_POINT ( 'NONE',  ( 71.48056072480412126, 59.16358519354559320, -15.78944119181872452 ) ) ;
#97981=CARTESIAN_POINT ( 'NONE',  ( 73.46727755934470849, 69.83818549023170874, 9.221945012360034610 ) ) ;
#97985=CARTESIAN_POINT ( 'NONE',  ( 71.36111289249075185, 71.40279321753016006, 3.762213664179777428 ) ) ;
#97986=CARTESIAN_POINT ( 'NONE',  ( 66.32789846179778692, 68.06826338654373387, -4.695580419454262966 ) ) ;
#97992=CARTESIAN_POINT ( 'NONE',  ( 26.97531487256933858, 21.28920272979927830, -7.433330006724141015 ) ) ;
#97993=CARTESIAN_POINT ( 'NONE',  ( 77.71695824120645568, 49.45779813244274692, 15.33409790704233977 ) ) ;
#97994=CARTESIAN_POINT ( 'NONE',  ( 83.75130605492059033, 51.70531176359354220, -14.84358514963803977 ) ) ;
#97998=CARTESIAN_POINT ( 'NONE',  ( 69.12867519028084473, 64.30014342229272017, 12.00737124844781967 ) ) ;
#98006=CARTESIAN_POINT ( 'NONE',  ( 71.23450976540344470, 70.68244710050896629, 5.511218535461621215 ) ) ;
#98007=DIRECTION ( 'NONE',  ( -0.8660254037844382635, -0.5000000000000005551, 0.000000000000000000 ) ) ;
#98010=CARTESIAN_POINT ( 'NONE',  ( 85.30253499385175076, 44.82337869870082159, 7.816767979061977734 ) ) ;
#98015=FACE_OUTER_BOUND ( 'NONE', #60339, .T. ) ;
#98019=CARTESIAN_POINT ( 'NONE',  ( 17.31863740857695078, 12.12755873383625271, -6.180339887498949025 ) ) ;
#98041=DIRECTION ( 'NONE',  ( 0.000000000000000000, 0.000000000000000000, -1.000000000000000000 ) ) ;
#98043=CARTESIAN_POINT ( 'NONE',  ( 75.78736691889224630, 62.67330692550549287, 15.04515854727457480 ) ) ;
#98047=CARTESIAN_POINT ( 'NONE',  ( 82.65509249134085223, 40.87170141247805333, 3.272232117641559856 ) ) ;
#98050=CARTESIAN_POINT ( 'NONE',  ( 25.69932979004302709, 23.03677371833802567, 10.00000000000000533 ) ) ;
#98054=CARTESIAN_POINT ( 'NONE',  ( 76.65905396365022284, 59.59921405739184763, 15.92423336072870299 ) ) ;
#98055=CARTESIAN_POINT ( 'NONE',  ( 12.71236424662705566, 15.84335787977761534, 9.188101187500006262 ) ) ;
#98056=ORIENTED_EDGE ( 'NONE', *, *, #64639, .F. ) ;
#98065=CARTESIAN_POINT ( 'NONE',  ( 79.71918192488826094, 50.71085193480788433, -15.38226593809065790 ) ) ;
#98068=CARTESIAN_POINT ( 'NONE',  ( 84.92581716621455712, 42.43763314791823404, 1.843432607090159658 ) ) ;
#98069=CARTESIAN_POINT ( 'NONE',  ( 88.26412553154668217, 44.25805425434632667, -1.894382960065053023 ) ) ;
#98070=ORIENTED_EDGE ( 'NONE', *, *, #81599, .F. ) ;
#98076=CARTESIAN_POINT ( 'NONE',  ( 85.18987148710466784, 44.62537788682696061, -7.596096801918241326 ) ) ;
#98079=CARTESIAN_POINT ( 'NONE',  ( 88.03979860270585789, 44.27742478294888429, 2.803906792406219761 ) ) ;
#98083=VECTOR ( 'NONE', #69287, 1000.000000000000227 ) ;
#98086=CARTESIAN_POINT ( 'NONE',  ( 80.53966528798085278, 57.74330293187745156, 16.24346292769213562 ) ) ;
#98090=CARTESIAN_POINT ( 'NONE',  ( 81.64670023727850889, 42.65128533460878657, -7.584980231169042852 ) ) ;
#98091=CARTESIAN_POINT ( 'NONE',  ( 68.85919161853215087, 67.18729119566384611, 9.802711484835468170 ) ) ;
#98098=CARTESIAN_POINT ( 'NONE',  ( 78.98010352777859566, 56.10884667310566698, 16.15057212009154952 ) ) ;
#98100=CARTESIAN_POINT ( 'NONE',  ( 76.02315037475985093, 54.93625610767154654, -16.12727872574887655 ) ) ;
#98105=CARTESIAN_POINT ( 'NONE',  ( 84.38175156668881982, 50.02035787987339432, 13.81135446509517628 ) ) ;
#98113=CARTESIAN_POINT ( 'NONE',  ( 14.61458989734527947, 10.29860640527290805, -2.839279412974138328 ) ) ;
#98119=CARTESIAN_POINT ( 'NONE',  ( 75.82286285680700644, 65.49053554218845363, 14.29367836297802974 ) ) ;
#98122=CARTESIAN_POINT ( 'NONE',  ( 43.68478726420265446, 28.14754757982094802, -5.678558825948275768 ) ) ;
#98124=CARTESIAN_POINT ( 'NONE',  ( 81.98204644731730184, 41.14170830008083612, -5.380964918418895238 ) ) ;
#98126=CARTESIAN_POINT ( 'NONE',  ( 25.16147942602835386, 23.03085787977763843, 9.188101187500006262 ) ) ;
#98129=CARTESIAN_POINT ( 'NONE',  ( 65.92723761088207368, 68.94945291059251247, -2.624861928015910895 ) ) ;
#98134=CARTESIAN_POINT ( 'NONE',  ( 70.48220200685271664, 60.91291783368861701, 14.45533156906698125 ) ) ;
#98141=ORIENTED_EDGE ( 'NONE', *, *, #34831, .T. ) ;
#98142=CARTESIAN_POINT ( 'NONE',  ( 70.46985782873493065, 64.39753548552634754, 13.11825968515873164 ) ) ;
#98143=ORIENTED_EDGE ( 'NONE', *, *, #16168, .T. ) ;
#98145=CARTESIAN_POINT ( 'NONE',  ( 84.29971156775336283, 42.10555697619372495, 2.085675295296966603 ) ) ;
#98147=CARTESIAN_POINT ( 'NONE',  ( 86.97523469022577558, 43.65653777248807899, 2.440289623876037872 ) ) ;
#98158=CARTESIAN_POINT ( 'NONE',  ( 43.01361757626970928, 27.76004757982093452, 5.678558825948272215 ) ) ;
#98161=EDGE_CURVE ( 'NONE', #62590, #74723, #68489, .T. ) ;
#98172=CARTESIAN_POINT ( 'NONE',  ( 66.40574244791143599, 68.75251593721850440, -2.129884441287897001 ) ) ;
#98173=CARTESIAN_POINT ( 'NONE',  ( 74.70219116882620369, 60.88919038526882588, -15.38845729014155417 ) ) ;
#98174=CARTESIAN_POINT ( 'NONE',  ( 82.43030793700373238, 40.39877996038060814, 0.9710434448888033421 ) ) ;
#98176=CARTESIAN_POINT ( 'NONE',  ( 76.77173841120222164, 63.31185858333683569, -15.44871830894366838 ) ) ;
#98183=CARTESIAN_POINT ( 'NONE',  ( 87.14453225490829880, 46.27907944775106586, -9.173786573548373013 ) ) ;
#98187=CARTESIAN_POINT ( 'NONE',  ( 73.99737204167014681, 54.85251815435404410, -16.13421978449814986 ) ) ;
#98190=ORIENTED_EDGE ( 'NONE', *, *, #64950, .F. ) ;
#98197=CARTESIAN_POINT ( 'NONE',  ( 84.13204908911603752, 50.42604040346916605, 13.71367173376234838 ) ) ;
#98199=CARTESIAN_POINT ( 'NONE',  ( 69.61708508526400863, 62.59193294829653098, -13.35423466821234584 ) ) ;
#98203=CARTESIAN_POINT ( 'NONE',  ( 82.58901599275658612, 52.38560239326635326, 14.96489765216765377 ) ) ;
#98204=CARTESIAN_POINT ( 'NONE',  ( 82.29231835864526090, 40.76292279040190181, -3.679577836841430916 ) ) ;
#98207=CARTESIAN_POINT ( 'NONE',  ( 71.91048869424076884, 72.26696636997301937, 3.280994121815376641 ) ) ;
#98211=CARTESIAN_POINT ( 'NONE',  ( 80.04809861183208852, 50.31413521909311726, 14.67867987935995977 ) ) ;
#98212=CARTESIAN_POINT ( 'NONE',  ( 69.60898357418011528, 70.31892478126285084, -3.724007916725324385 ) ) ;
#98215=CARTESIAN_POINT ( 'NONE',  ( 77.59172485204311442, 61.78102913438976174, 15.67081180326514556 ) ) ;
#98225=CARTESIAN_POINT ( 'NONE',  ( 34.89708068152319242, 43.08080186712595605, -3.090169943749475845 ) ) ;
#98227=CARTESIAN_POINT ( 'NONE',  ( 82.09289782346584730, 54.09536945811088060, 15.61809530791954082 ) ) ;
#98228=CARTESIAN_POINT ( 'NONE',  ( 71.91048869424076884, 72.26696636997301937, 3.280994121815385078 ) ) ;
#98232=CARTESIAN_POINT ( 'NONE',  ( 46.58353466793526110, 27.86426979415093896, -3.090169943749474069 ) ) ;
#98235=CARTESIAN_POINT ( 'NONE',  ( 71.84094281513496583, 72.11187483614946814, -1.688609671837987714 ) ) ;
#98238=CARTESIAN_POINT ( 'NONE',  ( 20.42541317417268942, 33.83396525600390703, -2.839279412974133887 ) ) ;
#98241=CARTESIAN_POINT ( 'NONE',  ( 40.44261144040436307, 35.30066082961425167, -10.00000000000000533 ) ) ;
#98245=CARTESIAN_POINT ( 'NONE',  ( 73.28922804852240347, 64.01006259886945315, 13.80277416833904525 ) ) ;
#98246=CARTESIAN_POINT ( 'NONE',  ( 69.29708453640807875, 67.89305789087417509, -8.400680196542618106 ) ) ;
#98251=EDGE_CURVE ( 'NONE', #35007, #59341, #11456, .T. ) ;
#98261=CARTESIAN_POINT ( 'NONE',  ( 79.24276467137505620, 45.83258386654563310, -12.43720478848687527 ) ) ;
#98269=AXIS2_PLACEMENT_3D ( 'NONE', #91409, #36168, #6777 ) ;
#98270=CARTESIAN_POINT ( 'NONE',  ( 26.78885238572174998, 16.26216523072495335, -2.296566073217252530E-15 ) ) ;
#98271=CARTESIAN_POINT ( 'NONE',  ( 76.22732431156450161, 61.39392654391182447, 15.52879837349084724 ) ) ;
#98273=CARTESIAN_POINT ( 'NONE',  ( 75.15236017364199483, 67.01938754673118126, -12.72247072481832042 ) ) ;
#98276=CARTESIAN_POINT ( 'NONE',  ( 77.55346118162754010, 59.95786661728646294, 16.37051007951880521 ) ) ;
#98284=CARTESIAN_POINT ( 'NONE',  ( 66.07789273159161780, 69.13191440305783431, -2.042338407063129857 ) ) ;
#98285=DIRECTION ( 'NONE',  ( 0.5000000000000014433, -0.8660254037844378194, 0.000000000000000000 ) ) ;
#98286=CARTESIAN_POINT ( 'NONE',  ( 81.76364840784469834, 55.63774643643142781, 16.32517576395870407 ) ) ;
#98292=CARTESIAN_POINT ( 'NONE',  ( 79.08607190154688737, 46.03631599640020511, 13.24059178838384376 ) ) ;
#98299=CARTESIAN_POINT ( 'NONE',  ( 75.10826011298540550, 67.04338188511664498, -12.68672718483817263 ) ) ;
#98302=CARTESIAN_POINT ( 'NONE',  ( 81.88283113365912413, 55.39261312399677450, 16.27191101227217729 ) ) ;
#98307=CARTESIAN_POINT ( 'NONE',  ( 70.45877369499376641, 64.12567799070421870, -12.70804357532220585 ) ) ;
#98313=EDGE_CURVE ( 'NONE', #96690, #26854, #29742, .T. ) ;
#98314=CARTESIAN_POINT ( 'NONE',  ( 76.25165189308367530, 51.01334316971484384, -16.04164650862850294 ) ) ;
#98316=B_SPLINE_CURVE_WITH_KNOTS ( 'NONE', 3,
 ( #19164, #49532, #97657, #43420, #66725, #50039, #88601, #95699, #51019, #35829, #26246, #72869, #74367, #26738, #89110, #41933, #57120, #65233, #19658, #4430, #41422, #96178, #57623, #72367 ),
 .UNSPECIFIED., .F., .F.,
 ( 4, 2, 2, 2, 2, 2, 2, 2, 2, 2, 2, 4 ),
 ( 0.000000000000000000, 0.1249999999999770739, 0.2499999999999541478, 0.3749999999999312217, 0.4374999999999381051, 0.4999999999999450440, 0.5624999999999519273, 0.6249999999999588107, 0.6874999999999658051, 0.7499999999999727995, 0.8749999999999863443, 1.000000000000000000 ),
 .UNSPECIFIED. ) ;
#98323=CARTESIAN_POINT ( 'NONE',  ( 87.95873400847938228, 44.36334681983743877, 4.762736470890962970 ) ) ;
#98326=CARTESIAN_POINT ( 'NONE',  ( 72.94799734335821029, 70.82305301834774980, 7.343759151627872406 ) ) ;
#98329=CARTESIAN_POINT ( 'NONE',  ( 77.47913788626532039, 60.68569559966617533, 15.87193550285029353 ) ) ;
#98333=CARTESIAN_POINT ( 'NONE',  ( 81.59908028989202933, 54.82413755204365913, 15.82053572924470686 ) ) ;
#98334=CARTESIAN_POINT ( 'NONE',  ( 73.48095451340876139, 69.18981038965245034, -10.00245108973057562 ) ) ;
#98340=B_SPLINE_SURFACE_WITH_KNOTS ( 'NONE', 3, 1, ( 
 ( #18071, #48967 ),
 ( #10978, #54284 ),
 ( #23394, #68999 ),
 ( #22413, #38601 ),
 ( #46186, #78125 ),
 ( #91854, #69998 ),
 ( #84749, #15289 ),
 ( #30510, #8713 ),
 ( #45690, #84260 ),
 ( #85254, #53305 ),
 ( #31495, #1118 ),
 ( #99430, #76144 ),
 ( #39085, #61892 ),
 ( #83757, #77105 ),
 ( #60891, #14807 ),
 ( #613, #76617 ),
 ( #7203, #6718 ),
 ( #37597, #60393 ),
 ( #85779, #45205 ),
 ( #92843, #99926 ),
 ( #119, #15799 ),
 ( #53788, #68508 ),
 ( #61401, #31003 ),
 ( #7708, #39582 ),
 ( #30007, #46705 ),
 ( #69505, #92353 ),
 ( #62387, #91349 ),
 ( #21910, #77631 ),
 ( #8215, #16308 ),
 ( #22902, #93344 ),
 ( #23900, #54802 ) ),
 .UNSPECIFIED., .F., .F., .F.,
 ( 4, 3, 3, 3, 3, 3, 3, 3, 3, 3, 4 ),
 ( 2, 2 ),
 ( 0.000000000000000000, 0.1122669598086729614, 0.2243161639709527755, 0.3396355846218981900, 0.4553962076584977536, 0.5677860799922215262, 0.6749047109689575441, 0.7773884377078212893, 0.8775581155834120128, 0.9782364162377664707, 1.000000000000000000 ),
 ( 0.000000000000000000, 1.000000000000000000 ),
 .UNSPECIFIED. ) ;
#98342=CARTESIAN_POINT ( 'NONE',  ( 18.89319741406618647, 35.00034080476290654, -1.878358725466461243E-16 ) ) ;
#98344=CARTESIAN_POINT ( 'NONE',  ( 81.99822479814268661, 41.74554429046528981, 5.407556307920054373 ) ) ;
#98351=EDGE_CURVE ( 'NONE', #59656, #63028, #35427, .T. ) ;
#98353=VERTEX_POINT ( 'NONE', #82080 ) ;
#98355=CARTESIAN_POINT ( 'NONE',  ( 66.58989550534374757, 68.03006047888345620, -6.526755023989535331 ) ) ;
#98359=CARTESIAN_POINT ( 'NONE',  ( 31.41050339915249268, 17.94473085651393518, 1.475505719884397138E-15 ) ) ;
#98360=CARTESIAN_POINT ( 'NONE',  ( 85.52132300739873472, 49.04541414811975386, 12.30295808577816352 ) ) ;
#98377=CARTESIAN_POINT ( 'NONE',  ( 36.38853680410606728, 41.98502408145596121, -5.678558825948271327 ) ) ;
#98381=DIRECTION ( 'NONE',  ( -0.8660254037844378194, -0.5000000000000014433, -0.000000000000000000 ) ) ;
#98384=CARTESIAN_POINT ( 'NONE',  ( 18.12859834787737157, 11.26216523072493736, -2.296566073217252530E-15 ) ) ;
#98385=CARTESIAN_POINT ( 'NONE',  ( 71.73821799984663983, 72.51259063078049394, 0.9720659048468339725 ) ) ;
#98386=CARTESIAN_POINT ( 'NONE',  ( 82.99898243690306288, 53.45938235784409187, 15.65150354709845359 ) ) ;
#98387=FACE_OUTER_BOUND ( 'NONE', #95191, .T. ) ;
#98391=CARTESIAN_POINT ( 'NONE',  ( 2.405479210251257438, 24.49540643055184930, 3.479690158560446702E-15 ) ) ;
#98392=CARTESIAN_POINT ( 'NONE',  ( 81.34586158848874504, 42.06304956376642679, 7.923271043321312490 ) ) ;
#98396=CARTESIAN_POINT ( 'NONE',  ( 82.46408787962569420, 40.41550683742634931, 0.9310554388106409007 ) ) ;
#98397=DIRECTION ( 'NONE',  ( 0.5000000000000014433, -0.8660254037844378194, 0.000000000000000000 ) ) ;
#98408=VERTEX_POINT ( 'NONE', #5530 ) ;
#98409=CARTESIAN_POINT ( 'NONE',  ( 87.57040987469007121, 45.45830532627585541, -6.786269783605160200 ) ) ;
#98413=CARTESIAN_POINT ( 'NONE',  ( 80.98043300753074902, 43.03517487223756177, 9.572663320340296877 ) ) ;
#98424=B_SPLINE_CURVE_WITH_KNOTS ( 'NONE', 3,
 ( #64418, #50210, #81162, #17829, #25933, #65902, #50696, #33010, #3150, #41601, #63911, #95867, #26425, #80664, #94849, #25410, #48730, #49227, #10226, #2633, #18331, #42105, #57305, #44083, #83137, #13707, #36496, #75023, #35506, #21311, #91232, #76030, #58784, #27904, #28916, #66899, #52188, #82159, #99316, #91732, #45096, #36996, #6100, #51721, #6607, #51192 ),
 .UNSPECIFIED., .F., .F.,
 ( 4, 1, 1, 1, 2, 2, 1, 1, 1, 2, 2, 1, 1, 2, 2, 1, 1, 2, 2, 1, 1, 2, 2, 1, 2, 2, 1, 2, 2, 4 ),
 ( 0.000000000000000000, 0.06249999999999465705, 0.09374999999999200639, 0.1093749999999922146, 0.1171874999999923117, 0.1249999999999924227, 0.1875000000000008327, 0.2187500000000050515, 0.2343750000000056621, 0.2421875000000053568, 0.2500000000000050515, 0.3125000000000046629, 0.3437500000000054401, 0.3593750000000048850, 0.3750000000000042744, 0.4375000000000038858, 0.4687500000000037748, 0.4843750000000032752, 0.5000000000000027756, 0.5625000000000078826, 0.5937500000000111022, 0.6093750000000122125, 0.6250000000000133227, 0.6875000000000107692, 0.7187500000000102141, 0.7500000000000095479, 0.8125000000000073275, 0.8437500000000063283, 0.8750000000000053291, 1.000000000000000000 ),
 .UNSPECIFIED. ) ;
#98427=AXIS2_PLACEMENT_3D ( 'NONE', #31305, #31795, #46495 ) ;
#98429=CARTESIAN_POINT ( 'NONE',  ( 76.84516209278983467, 52.46037536181771088, -16.28082285436079957 ) ) ;
#98438=CARTESIAN_POINT ( 'NONE',  ( 75.39974219951720613, 57.58420828353521159, -16.06839496810986034 ) ) ;
#98441=CARTESIAN_POINT ( 'NONE',  ( 67.00187114328801385, 67.08813303294822106, 8.529924657525400633 ) ) ;
#98446=CARTESIAN_POINT ( 'NONE',  ( 78.56665040545209422, 53.37396691067563381, -15.81981728764792905 ) ) ;
#98448=CARTESIAN_POINT ( 'NONE',  ( 78.89634812866061964, 46.30573133001255570, 12.89508449444912230 ) ) ;
#98450=CARTESIAN_POINT ( 'NONE',  ( 77.42830020291178528, 55.47891526150226582, -16.57918540093258031 ) ) ;
#98461=DIRECTION ( 'NONE',  ( -0.8660254037844379305, -0.5000000000000014433, -0.000000000000000000 ) ) ;
#98471=CARTESIAN_POINT ( 'NONE',  ( 81.87537396349165419, 41.14590722702494219, -5.544662510333616900 ) ) ;
#98472=DIRECTION ( 'NONE',  ( -0.8660254037844379305, -0.5000000000000014433, -0.000000000000000000 ) ) ;
#98478=VECTOR ( 'NONE', #54433, 1000.000000000000227 ) ;
#98486=CARTESIAN_POINT ( 'NONE',  ( 10.13172230794903683, 17.80066082961419838, 10.00000000000000533 ) ) ;
#98488=CARTESIAN_POINT ( 'NONE',  ( 71.56806419291221744, 59.47990913521268652, -15.71253939761329832 ) ) ;
#98489=CARTESIAN_POINT ( 'NONE',  ( 73.05912352472128646, 69.60491006942920933, 9.219028434792557292 ) ) ;
#98493=CARTESIAN_POINT ( 'NONE',  ( 70.70474417252469834, 70.58686583719459406, 5.013298563372670991 ) ) ;
#98501=CARTESIAN_POINT ( 'NONE',  ( 27.04628097738780212, 27.56628583063842086, 9.188101187500006262 ) ) ;
#98503=CARTESIAN_POINT ( 'NONE',  ( 83.80076462262509551, 51.77978008689729705, -14.86347872566931549 ) ) ;
#98505=CARTESIAN_POINT ( 'NONE',  ( 88.28217478145764119, 43.95791727297698515, 2.470383038495647998 ) ) ;
#98507=CARTESIAN_POINT ( 'NONE',  ( 68.94975261236909603, 64.36897199676705839, 12.51175351931266633 ) ) ;
#98511=CARTESIAN_POINT ( 'NONE',  ( 68.30758603522241401, 67.25884571155089020, -9.331438848602806146 ) ) ;
#98517=CARTESIAN_POINT ( 'NONE',  ( 86.54822389131679472, 42.74345947012793090, -2.172736160200603931E-06 ) ) ;
#98518=LINE ( 'NONE', #29108, #70004 ) ;
#98520=CARTESIAN_POINT ( 'NONE',  ( 88.45958475239287111, 43.85926912372239173, -0.5941283661710181629 ) ) ;
#98521=CARTESIAN_POINT ( 'NONE',  ( 67.78857209169460418, 69.02767894211700650, 4.439189011663660978 ) ) ;
#98522=DIRECTION ( 'NONE',  ( 0.000000000000000000, 0.6050222638427442678, -0.7962085532412978006 ) ) ;
#98525=CARTESIAN_POINT ( 'NONE',  ( 12.45916558416763209, 19.14441083166259361, 10.00000000000000533 ) ) ;
#98530=CARTESIAN_POINT ( 'NONE',  ( 83.84264525447930794, 45.19566160288086110, -9.473173988316984762 ) ) ;
#98541=CARTESIAN_POINT ( 'NONE',  ( 81.21353692635089772, 42.35982027868730171, -7.518915552659992230 ) ) ;
#98543=ORIENTED_EDGE ( 'NONE', *, *, #96274, .F. ) ;
#98544=CARTESIAN_POINT ( 'NONE',  ( 88.25809008468522165, 43.73205518618092214, 0.2003341539982119168 ) ) ;
#98549=CARTESIAN_POINT ( 'NONE',  ( 75.58424500764920140, 61.59228886874195297, 15.33674465601570169 ) ) ;
#98550=CARTESIAN_POINT ( 'NONE',  ( 87.89265348834460667, 45.03651295921149256, 6.473805411810645616 ) ) ;
#98553=PLANE ( 'NONE',  #25538 ) ;
#98559=CARTESIAN_POINT ( 'NONE',  ( 82.83063800212752881, 53.40025595410719461, -15.30243353670389261 ) ) ;
#98563=CARTESIAN_POINT ( 'NONE',  ( 8.860943796042899834, 20.51421378149916919, -9.188101187500004485 ) ) ;
#98573=CARTESIAN_POINT ( 'NONE',  ( 66.60661563016273590, 67.77273566365288104, -7.043189648870077590 ) ) ;
#98575=CARTESIAN_POINT ( 'NONE',  ( 84.34251726751226386, 42.03111163911867720, 1.049105841315436827 ) ) ;
#98580=CARTESIAN_POINT ( 'NONE',  ( 74.93756780616698165, 67.42216207915812731, -12.80861374294490140 ) ) ;
#98581=ORIENTED_EDGE ( 'NONE', *, *, #56796, .F. ) ;
#98590=CARTESIAN_POINT ( 'NONE',  ( 33.48063555417975579, 19.73415679381824006, -6.890680421881970419E-14 ) ) ;
#98594=ORIENTED_EDGE ( 'NONE', *, *, #51965, .F. ) ;
#98611=CARTESIAN_POINT ( 'NONE',  ( 38.72117548675866061, 22.75978393459168103, -1.583844403245396437 ) ) ;
#98616=CARTESIAN_POINT ( 'NONE',  ( 84.49275162666286576, 50.19829916693547744, 13.87667126673719231 ) ) ;
#98622=DIRECTION ( 'NONE',  ( -0.8660254037844378194, -0.5000000000000014433, -0.000000000000000000 ) ) ;
#98624=CARTESIAN_POINT ( 'NONE',  ( 7.453652514893187586, 19.70171378149916919, -9.188101187500004485 ) ) ;
#98625=CARTESIAN_POINT ( 'NONE',  ( 67.63254175845027305, 65.87441213026522746, 10.48036353779758123 ) ) ;
#98631=CARTESIAN_POINT ( 'NONE',  ( 76.06516313603486878, 65.42396348981594656, 14.39793886682781832 ) ) ;
#98633=CARTESIAN_POINT ( 'NONE',  ( 40.42214693012152793, 25.19860640527295104, 2.839279412974134775 ) ) ;
#98637=CARTESIAN_POINT ( 'NONE',  ( 19.57800816787531417, 26.70171378149919050, -9.188101187500004485 ) ) ;
#98641=CARTESIAN_POINT ( 'NONE',  ( 70.37850334050121148, 61.05907127409049906, 14.36771776055900496 ) ) ;
#98648=CARTESIAN_POINT ( 'NONE',  ( 72.97386446981147401, 70.68132344495337804, 8.316175787459499702 ) ) ;
#98649=EDGE_LOOP ( 'NONE', ( #61852, #86761, #55326, #71246 ) ) ;
#98651=CARTESIAN_POINT ( 'NONE',  ( 66.06293672572081732, 68.52299781147171132, 4.587403909294850202 ) ) ;
#98653=CARTESIAN_POINT ( 'NONE',  ( 87.37689300401315506, 44.00708636583175348, 3.108306139222640319 ) ) ;
#98658=CARTESIAN_POINT ( 'NONE',  ( 88.19119485691749105, 44.51220553762047416, -4.804906155116621669 ) ) ;
#98663=CARTESIAN_POINT ( 'NONE',  ( 36.06377727768690988, 41.79752408145595410, -5.678558825948271327 ) ) ;
#98664=CARTESIAN_POINT ( 'NONE',  ( 75.45938151893163592, 59.84466625416695251, -15.73511245645754464 ) ) ;
#98665=EDGE_CURVE ( 'NONE', #59818, #63171, #77309, .T. ) ;
#98670=CARTESIAN_POINT ( 'NONE',  ( 72.04618005861752295, 72.23985218540053665, -1.584352113898356951 ) ) ;
#98671=CARTESIAN_POINT ( 'NONE',  ( 87.23257741107988750, 46.04474800944700519, -8.789869334516776433 ) ) ;
#98676=CARTESIAN_POINT ( 'NONE',  ( 73.61711655523605202, 61.23855026575265725, -15.07042752294893617 ) ) ;
#98677=CARTESIAN_POINT ( 'NONE',  ( 82.21611827071926371, 40.83382032456969313, 1.069328909644415848 ) ) ;
#98680=CARTESIAN_POINT ( 'NONE',  ( 77.28420460057618868, 63.06679313565820166, -15.26332939213814655 ) ) ;
#98681=CARTESIAN_POINT ( 'NONE',  ( 78.86792953187128319, 59.60067377931095933, 16.50582274385373083 ) ) ;
#98684=CARTESIAN_POINT ( 'NONE',  ( 70.81316579126399802, 61.41551742065354347, -14.85192641751565468 ) ) ;
#98685=CARTESIAN_POINT ( 'NONE',  ( 36.80649086932150027, 23.11110640527294535, -2.839279412974138328 ) ) ;
#98693=CARTESIAN_POINT ( 'NONE',  ( 13.31457613402888995, 31.18528772668516424, -1.583844403245363575 ) ) ;
#98701=FACE_OUTER_BOUND ( 'NONE', #95955, .T. ) ;
#98703=CARTESIAN_POINT ( 'NONE',  ( 82.85927426857082878, 45.93892428374152814, 10.86312220312391830 ) ) ;
#98707=ORIENTED_EDGE ( 'NONE', *, *, #28259, .F. ) ;
#98714=CARTESIAN_POINT ( 'NONE',  ( 72.15865790475056940, 72.27389710013802926, 3.820985825366547406 ) ) ;
#98720=CARTESIAN_POINT ( 'NONE',  ( 82.44310520575160695, 54.28011738120410001, -15.96781897959229113 ) ) ;
#98727=EDGE_CURVE ( 'NONE', #53284, #19489, #21776, .T. ) ;
#98730=CARTESIAN_POINT ( 'NONE',  ( 65.74726825304114186, 69.08659106095529978, 2.128305819671951817E-12 ) ) ;
#98733=ADVANCED_FACE ( 'NONE', ( #25992 ), #82217, .T. ) ;
#98734=CARTESIAN_POINT ( 'NONE',  ( 34.48165468218606833, 44.00034080476292786, -1.878358725466461243E-16 ) ) ;
#98736=( BOUNDED_CURVE ( )  B_SPLINE_CURVE ( 2, ( #54984, #94034, #78810, #63088, #25082, #1804, #70687, #24584, #16981, #47872, #71213, #32688, #63589 ),
 .UNSPECIFIED., .F., .T. ) 
 B_SPLINE_CURVE_WITH_KNOTS ( ( 3, 2, 2, 2, 2, 2, 3 ),
 ( 0.5375000000000000888, 0.5400000000000000355, 0.5450000000000000400, 0.5500000000000000444, 0.5550000000000000488, 0.5600000000000000533, 0.5625000000000000000 ),
 .UNSPECIFIED. ) 
 CURVE ( )  GEOMETRIC_REPRESENTATION_ITEM ( )  RATIONAL_B_SPLINE_CURVE ( ( 0.9755282581475767101, 0.9755282581475772652, 1.000000000000000000, 0.9510565162951535312, 1.000000000000000000, 0.9510565162951535312, 1.000000000000000000, 0.9510565162951535312, 1.000000000000000000, 0.9510565162951535312, 1.000000000000000000, 0.9755282581475768211, 0.9755282581475768211 ) ) 
 REPRESENTATION_ITEM ( '' )  );
#98738=CARTESIAN_POINT ( 'NONE',  ( 71.90028047037452552, 71.95896194932872447, 2.840402229763955066 ) ) ;
#98742=CARTESIAN_POINT ( 'NONE',  ( 71.93703274728032682, 72.16823338693137657, -1.679264843172269650 ) ) ;
#98744=CARTESIAN_POINT ( 'NONE',  ( 26.45569963029868177, 20.98920272979927049, 7.433330006724137462 ) ) ;
#98747=CARTESIAN_POINT ( 'NONE',  ( 44.42076818640806835, 30.81029122506298634, 8.090169943749479842 ) ) ;
#98750=CARTESIAN_POINT ( 'NONE',  ( 75.50150731818223448, 56.53949938707354050, 16.58547563118056090 ) ) ;
#98752=CARTESIAN_POINT ( 'NONE',  ( 72.59582657278434681, 61.38205835117237541, 14.77812198616874895 ) ) ;
#98753=CARTESIAN_POINT ( 'NONE',  ( 73.53566697132028196, 67.45690392929650159, -11.63657775242925929 ) ) ;
#98759=EDGE_LOOP ( 'NONE', ( #7598, #55506, #34858, #20400 ) ) ;
#98767=B_SPLINE_CURVE_WITH_KNOTS ( 'NONE', 3,
 ( #54559, #78915, #8002, #100210, #38877, #40367, #1401, #85022 ),
 .UNSPECIFIED., .F., .F.,
 ( 4, 2, 2, 4 ),
 ( 0.1555655374897298437, 0.5777827687448640059, 0.7888913843724321140, 1.000000000000000000 ),
 .UNSPECIFIED. ) ;
#98769=CARTESIAN_POINT ( 'NONE',  ( 79.26966485285926467, 46.35457182308554280, -12.78027692334229748 ) ) ;
#98770=CARTESIAN_POINT ( 'NONE',  ( 72.16589213194404806, 62.31695436414708666, 14.80019564645472840 ) ) ;
#98771=CARTESIAN_POINT ( 'NONE',  ( 72.89831966083461623, 70.30981352087286496, -8.130391679937307714 ) ) ;
#98774=ORIENTED_EDGE ( 'NONE', *, *, #31734, .T. ) ;
#98775=CARTESIAN_POINT ( 'NONE',  ( 26.41418602390824333, 17.11110640527292759, -2.839279412974138328 ) ) ;
#98776=CARTESIAN_POINT ( 'NONE',  ( 79.96602959028801649, 44.47270156346923642, 11.66712872020432457 ) ) ;
#98777=CARTESIAN_POINT ( 'NONE',  ( 69.22385677126450787, 69.96866776554797696, -4.197617061747116907 ) ) ;
#98785=CARTESIAN_POINT ( 'NONE',  ( 72.46264091457396717, 68.04234003238872219, 11.10956356103667986 ) ) ;
#98798=ORIENTED_EDGE ( 'NONE', *, *, #62774, .F. ) ;
#98804=CARTESIAN_POINT ( 'NONE',  ( 80.09302555852339367, 44.25273809412914261, -11.40411237053047167 ) ) ;
#98807=CARTESIAN_POINT ( 'NONE',  ( 85.76034556165906508, 42.63951191185048373, -3.229101607542598007 ) ) ;
#98810=CARTESIAN_POINT ( 'NONE',  ( 70.74076148756792293, 64.84648076579460962, 12.32345133226214884 ) ) ;
#98817=B_SPLINE_CURVE_WITH_KNOTS ( 'NONE', 3,
 ( #90419, #58455, #41765, #49874, #97979, #27085, #74196, #89428, #82325, #50859 ),
 .UNSPECIFIED., .F., .F.,
 ( 4, 2, 2, 2, 4 ),
 ( 0.000000000000000000, 0.2500000000000000000, 0.5000000000000000000, 0.7500000000000000000, 1.000000000000000000 ),
 .UNSPECIFIED. ) ;
#98819=CARTESIAN_POINT ( 'NONE',  ( 81.82036482989325066, 42.35048943672428834, -7.944650131338358179 ) ) ;
#98824=CARTESIAN_POINT ( 'NONE',  ( 88.18953256495667858, 44.42393962918851713, 4.547252263720217513 ) ) ;
#98825=CARTESIAN_POINT ( 'NONE',  ( 72.86837948048784597, 67.33958022161600354, -11.94987273000593575 ) ) ;
#98828=CARTESIAN_POINT ( 'NONE',  ( 74.75920290338640939, 66.43904096090548705, -12.97148193089175905 ) ) ;
#98834=CARTESIAN_POINT ( 'NONE',  ( 72.59839265552557208, 71.34777361097565063, -5.944036940999890106 ) ) ;
#98835=CARTESIAN_POINT ( 'NONE',  ( 81.34519720517472763, 53.17022275404438147, 15.42862813885395923 ) ) ;
#98837=EDGE_CURVE ( 'NONE', #77239, #93313, #5658, .T. ) ;
#98840=CARTESIAN_POINT ( 'NONE',  ( 72.04834849415195208, 72.28436413801230742, -0.8995985284803106330 ) ) ;
#98845=CARTESIAN_POINT ( 'NONE',  ( 19.72404941274043466, 33.16126292948894871, -6.180339887498951690 ) ) ;
#98846=FACE_OUTER_BOUND ( 'NONE', #32565, .T. ) ;
#98848=CARTESIAN_POINT ( 'NONE',  ( 71.98367679655076756, 69.26045741849536341, -9.475566133687880921 ) ) ;
#98851=CARTESIAN_POINT ( 'NONE',  ( 72.11651558246516913, 71.81869578167429324, -3.920535044530327529 ) ) ;
#98854=ORIENTED_EDGE ( 'NONE', *, *, #34831, .F. ) ;
#98855=CARTESIAN_POINT ( 'NONE',  ( 66.64741794046514656, 68.07194284811899365, -6.509155038794735226 ) ) ;
#98856=CARTESIAN_POINT ( 'NONE',  ( 72.47494455774663891, 70.67364856651921912, -7.881577117668181032 ) ) ;
#98860=CARTESIAN_POINT ( 'NONE',  ( 22.08843299157899764, 31.49103043416549852, -8.090169943749479842 ) ) ;
#98861=CARTESIAN_POINT ( 'NONE',  ( 85.33961507832758286, 48.52663690637297123, 12.44665103731247235 ) ) ;
#98868=CARTESIAN_POINT ( 'NONE',  ( 81.81922014299045998, 41.23558842254242052, 5.835146561875444782 ) ) ;
#98874=CARTESIAN_POINT ( 'NONE',  ( 34.28181963472369631, 41.83396525600392835, -2.839279412974133887 ) ) ;
#98877=FACE_OUTER_BOUND ( 'NONE', #96959, .T. ) ;
#98880=CARTESIAN_POINT ( 'NONE',  ( 19.64056747690256088, 19.84335787977763133, 9.188101187500006262 ) ) ;
#98882=CARTESIAN_POINT ( 'NONE',  ( 71.77793909028444830, 59.04410539788438683, 15.36942587551596695 ) ) ;
#98889=CARTESIAN_POINT ( 'NONE',  ( 88.28069365579224836, 44.35490120276798365, 2.424033814871950465 ) ) ;
#98892=CARTESIAN_POINT ( 'NONE',  ( 69.05335124041866379, 70.45577847891635770, -1.018671009100705627 ) ) ;
#98902=CARTESIAN_POINT ( 'NONE',  ( 80.20448007545800806, 58.22194284664072939, -16.60717859687067843 ) ) ;
#98906=EDGE_CURVE ( 'NONE', #4426, #81254, #36546, .T. ) ;
#98925=CARTESIAN_POINT ( 'NONE',  ( 82.56006566965427851, 42.71737122084187632, -6.803253249287812388 ) ) ;
#98933=CARTESIAN_POINT ( 'NONE',  ( 79.55398215537849183, 56.00914138994535563, -16.14968118437373690 ) ) ;
#98941=CARTESIAN_POINT ( 'NONE',  ( 74.08065690531797998, 54.82731643721707826, -16.13522336645905142 ) ) ;
#98942=CARTESIAN_POINT ( 'NONE',  ( 82.39721099668476256, 40.42262220707492304, 1.474573639734337860 ) ) ;
#98943=CARTESIAN_POINT ( 'NONE',  ( 78.90892980406610491, 46.27727789011839121, 12.87123018350744097 ) ) ;
#98944=CYLINDRICAL_SURFACE ( 'NONE', #30556, 16.60714546451156792 ) ;
#98946=VERTEX_POINT ( 'NONE', #39522 ) ;
#98948=DIRECTION ( 'NONE',  ( -0.8660254037844379305, -0.5000000000000014433, -0.000000000000000000 ) ) ;
#98950=CARTESIAN_POINT ( 'NONE',  ( 72.15585720070407660, 71.46694910313807725, 5.049726176867119776 ) ) ;
#98954=CARTESIAN_POINT ( 'NONE',  ( 66.74197533670303528, 67.35026328120331129, -6.853813334782631550 ) ) ;
#98955=CARTESIAN_POINT ( 'NONE',  ( 84.47821962090468162, 50.67508502715828200, 13.74210141425526999 ) ) ;
#98961=CARTESIAN_POINT ( 'NONE',  ( 74.05623475345210238, 67.87786276047000911, -11.59565021290446651 ) ) ;
#98963=DIRECTION ( 'NONE',  ( -0.5000000000000013323, 0.8660254037844378194, 0.000000000000000000 ) ) ;
#98965=CARTESIAN_POINT ( 'NONE',  ( 81.71413070705057180, 41.63923530988346755, -5.548261066783312323 ) ) ;
#98970=ORIENTED_EDGE ( 'NONE', *, *, #2311, .T. ) ;
#98976=CARTESIAN_POINT ( 'NONE',  ( 67.44819667686662967, 68.73639689937741082, -6.116911733827506303 ) ) ;
#98978=CARTESIAN_POINT ( 'NONE',  ( 71.74055746682908818, 59.25036641841931129, -15.30500015931909985 ) ) ;
#98979=CARTESIAN_POINT ( 'NONE',  ( 73.11332203459717505, 69.70319764633998716, 9.138078346488789805 ) ) ;
#98983=CARTESIAN_POINT ( 'NONE',  ( 72.64791381987437546, 57.16179493898301445, 16.36434895450253535 ) ) ;
#98985=CARTESIAN_POINT ( 'NONE',  ( 66.13364871532078837, 68.62542172597147783, -4.396739254649349782 ) ) ;
#98987=AXIS2_PLACEMENT_3D ( 'NONE', #87492, #78328, #24604 ) ;
#98991=CARTESIAN_POINT ( 'NONE',  ( 26.89353023359722883, 24.03085787977764198, 9.188101187500006262 ) ) ;
#98993=CARTESIAN_POINT ( 'NONE',  ( 83.73048316204189234, 51.68689211301329323, -14.84080274415373069 ) ) ;
#98994=CARTESIAN_POINT ( 'NONE',  ( 75.20389695419315501, 52.88180760346911313, -15.99093876381489920 ) ) ;
#98995=CARTESIAN_POINT ( 'NONE',  ( 69.48582975785168969, 69.23567760989607223, 7.408010502022341903 ) ) ;
#98996=CARTESIAN_POINT ( 'NONE',  ( 74.68831750804957892, 67.03523027571368686, 12.97943796060243038 ) ) ;
#98997=CARTESIAN_POINT ( 'NONE',  ( 68.60540934294387228, 64.14349346637945359, 11.89531485900240249 ) ) ;
#98999=CARTESIAN_POINT ( 'NONE',  ( 80.69646656315177324, 49.01814528795178916, 14.42895880536565301 ) ) ;
#99001=CARTESIAN_POINT ( 'NONE',  ( 75.08824155956695279, 66.10533156918239683, -13.73658325454725215 ) ) ;
#99003=CARTESIAN_POINT ( 'NONE',  ( 10.86724236217879458, 11.98920272979924206, 7.433330006724137462 ) ) ;
#99007=CARTESIAN_POINT ( 'NONE',  ( 75.27786518154783835, 53.33848916356247116, 16.02953000850719434 ) ) ;
#99008=CARTESIAN_POINT ( 'NONE',  ( 71.63453813518017910, 72.07236434383469259, 0.7172108931481424587 ) ) ;
#99016=CARTESIAN_POINT ( 'NONE',  ( 17.73406340791407843, 11.20801979619927558, -3.090169943749474069 ) ) ;
#99018=VERTEX_POINT ( 'NONE', #2571 ) ;
#99021=CARTESIAN_POINT ( 'NONE',  ( 84.94009691319403998, 45.09646382260235953, -8.562744380091208640 ) ) ;
#99026=CARTESIAN_POINT ( 'NONE',  ( 69.64468245311012140, 62.54413290503185863, 13.39146398752162703 ) ) ;
#99032=CARTESIAN_POINT ( 'NONE',  ( 73.42123007364070020, 69.75766128465485849, -9.876216450746401421 ) ) ;
#99034=CARTESIAN_POINT ( 'NONE',  ( 81.38192781600989179, 42.01391432718669705, -7.810538413258424129 ) ) ;
#99035=EDGE_LOOP ( 'NONE', ( #29027, #32080, #78599, #15773 ) ) ;
#99038=ORIENTED_EDGE ( 'NONE', *, *, #67122, .F. ) ;
#99039=CARTESIAN_POINT ( 'NONE',  ( 81.20490824193147716, 49.21687788665059315, 13.87893507568480622 ) ) ;
#99042=CARTESIAN_POINT ( 'NONE',  ( 71.17622542568626898, 71.72302770732439114, 1.525814289146208091 ) ) ;
#99045=CARTESIAN_POINT ( 'NONE',  ( 82.40646201738856291, 41.30234202567336865, 3.324496349298553532 ) ) ;
#99046=EDGE_CURVE ( 'NONE', #95936, #6127, #41030, .T. ) ;
#99050=CARTESIAN_POINT ( 'NONE',  ( 69.86572752188030222, 68.44440742063116545, -8.131768615182894067 ) ) ;
#99052=ORIENTED_EDGE ( 'NONE', *, *, #62199, .F. ) ;
#99053=CARTESIAN_POINT ( 'NONE',  ( 76.26964293081611856, 57.53102226905608063, 16.11233859593322748 ) ) ;
#99054=CARTESIAN_POINT ( 'NONE',  ( 13.73114039420206645, 19.87878583063839955, -9.188101187500006262 ) ) ;
#99057=CARTESIAN_POINT ( 'NONE',  ( 85.68854969368454988, 48.82517353895561030, 12.04942435251151167 ) ) ;
#99059=VERTEX_POINT ( 'NONE', #64351 ) ;
#99069=CARTESIAN_POINT ( 'NONE',  ( 74.23328924489679537, 62.52147022964773981, -14.75899811459794186 ) ) ;
#99072=CARTESIAN_POINT ( 'NONE',  ( 82.84394531096333480, 53.42394160290496075, -15.30708917581039863 ) ) ;
#99074=CARTESIAN_POINT ( 'NONE',  ( 72.12725721317737282, 72.31402113146141630, 1.179144219167332919 ) ) ;
#99079=VERTEX_POINT ( 'NONE', #79092 ) ;
#99087=CARTESIAN_POINT ( 'NONE',  ( 83.77489950824539733, 45.17479857692421064, 9.492654013345440234 ) ) ;
#99097=CARTESIAN_POINT ( 'NONE',  ( 83.27851594750828212, 52.38278085640094872, -14.83539284712679951 ) ) ;
#99101=CARTESIAN_POINT ( 'NONE',  ( 70.90515648226063661, 61.13412645828226033, -14.46341648420804482 ) ) ;
#99105=DIRECTION ( 'NONE',  ( -0.8660254037844377084, -0.5000000000000014433, -0.000000000000000000 ) ) ;
#99110=CARTESIAN_POINT ( 'NONE',  ( 12.59929316974766955, 12.98920272979924739, 7.433330006724137462 ) ) ;
#99119=CARTESIAN_POINT ( 'NONE',  ( 32.72297390791170812, 40.93396525600392977, 2.839279412974139660 ) ) ;
#99123=CARTESIAN_POINT ( 'NONE',  ( 23.51484842749693627, 36.68290643055188838, 3.479690158560446702E-15 ) ) ;
#99127=ORIENTED_EDGE ( 'NONE', *, *, #12141, .F. ) ;
#99128=CARTESIAN_POINT ( 'NONE',  ( 70.34371006524575876, 61.11933499459465224, 14.86285179514932508 ) ) ;
#99129=CARTESIAN_POINT ( 'NONE',  ( 76.04102746794296763, 65.42908112640478180, -14.38850911432199098 ) ) ;
#99136=CARTESIAN_POINT ( 'NONE',  ( 78.41424692880730163, 61.43889907920149795, 16.20108440401020999 ) ) ;
#99139=CARTESIAN_POINT ( 'NONE',  ( 86.48988058553197789, 47.46618689836390104, -10.40901836545075909 ) ) ;
#99144=CARTESIAN_POINT ( 'NONE',  ( 38.77491099913230954, 28.10170272979929962, -7.433330006724141015 ) ) ;
#99145=CARTESIAN_POINT ( 'NONE',  ( 81.39533252797791363, 55.41833949407015325, -16.32393128051839781 ) ) ;
#99148=CARTESIAN_POINT ( 'NONE',  ( 87.47559087308273718, 45.51532872389798712, 7.025594959947058626 ) ) ;
#99151=CARTESIAN_POINT ( 'NONE',  ( 72.03307586204233814, 72.23070632498334476, -1.602297053105369740 ) ) ;
#99153=CARTESIAN_POINT ( 'NONE',  ( 79.62893888804012477, 55.87931252087706469, 16.13392464427525042 ) ) ;
#99155=CARTESIAN_POINT ( 'NONE',  ( 74.14312167556930433, 66.30466486950707861, 1.224646799147354045E-15 ) ) ;
#99159=CARTESIAN_POINT ( 'NONE',  ( 78.67410342229302955, 59.31965170277735666, -16.17003662270398223 ) ) ;
#99168=CARTESIAN_POINT ( 'NONE',  ( 35.97235683590213284, 38.95586893147758190, 7.433330006724141015 ) ) ;
#99172=CARTESIAN_POINT ( 'NONE',  ( 74.13689204002625388, 68.84749506857346546, -11.26202041109552177 ) ) ;
#99173=AXIS2_PLACEMENT_3D ( 'NONE', #75212, #36679, #67588 ) ;
#99177=CARTESIAN_POINT ( 'NONE',  ( 69.97903499771932445, 71.34659005825866984, 2.366570824083385816 ) ) ;
#99180=DIRECTION ( 'NONE',  ( 0.5000000000000014433, -0.8660254037844378194, 0.000000000000000000 ) ) ;
#99186=B_SPLINE_CURVE_WITH_KNOTS ( 'NONE', 3,
 ( #98720, #84038, #6500, #7475, #37377, #14597, #53085, #6983, #21695, #54065, #99701, #37868, #68282, #29304, #45476, #52577, #60662, #388, #15564, #30288, #91131, #91620, #22191, #61177, #92143, #22697, #38875, #77397, #53574, #100208, #54557 ),
 .UNSPECIFIED., .F., .F.,
 ( 4, 3, 3, 3, 3, 3, 3, 3, 3, 3, 4 ),
 ( 0.000000000000000000, 0.1333490885032429241, 0.3007194338854423110, 0.4699862290245206409, 0.5844252810809303922, 0.6686540514502636867, 0.7354980260655383795, 0.8028463152565493699, 0.8633854507757111607, 0.9437142632667171460, 1.000000000000000000 ),
 .UNSPECIFIED. ) ;
#99193=EDGE_LOOP ( 'NONE', ( #39682, #87104 ) ) ;
#99196=CARTESIAN_POINT ( 'NONE',  ( 82.37514789520893999, 41.30464489057703048, -3.406265280166828280 ) ) ;
#99197=LINE ( 'NONE', #75402, #44809 ) ;
#99204=CARTESIAN_POINT ( 'NONE',  ( 71.86034221268614886, 70.72569178174764204, -6.256625118109824690 ) ) ;
#99209=CARTESIAN_POINT ( 'NONE',  ( 66.97748580466556234, 68.05911003901715617, 6.908000617270682042 ) ) ;
#99213=CARTESIAN_POINT ( 'NONE',  ( 73.17137018064387632, 69.60265530810194434, -9.888782888319330056 ) ) ;
#99215=CARTESIAN_POINT ( 'NONE',  ( 6.396987757676564357, 15.64441083166258295, -10.00000000000000533 ) ) ;
#99217=CARTESIAN_POINT ( 'NONE',  ( 35.65891684237410431, 42.36126292948898708, 6.180339887498949913 ) ) ;
#99219=CARTESIAN_POINT ( 'NONE',  ( 82.60915189404757086, 54.13479165414026539, 15.54566119520439926 ) ) ;
#99220=FACE_OUTER_BOUND ( 'NONE', #52916, .T. ) ;
#99224=CARTESIAN_POINT ( 'NONE',  ( 42.17466224797323804, 36.30066082961425877, -10.00000000000000533 ) ) ;
#99225=CARTESIAN_POINT ( 'NONE',  ( 81.47939018540962763, 50.17275021362014797, -14.26619682564655456 ) ) ;
#99229=CARTESIAN_POINT ( 'NONE',  ( 22.71615395846560759, 25.06628583063842086, -9.188101187500006262 ) ) ;
#99232=CARTESIAN_POINT ( 'NONE',  ( 11.38685760444945672, 12.28920272979924988, -7.433330006724141015 ) ) ;
#99234=CARTESIAN_POINT ( 'NONE',  ( 76.85865272105424140, 63.69649487134743282, 15.33129195839047298 ) ) ;
#99246=ORIENTED_EDGE ( 'NONE', *, *, #38842, .T. ) ;
#99249=VERTEX_POINT ( 'NONE', #33117 ) ;
#99253=EDGE_LOOP ( 'NONE', ( #100188, #83876, #71234, #7562 ) ) ;
#99256=CARTESIAN_POINT ( 'NONE',  ( 79.42038935749546624, 46.23329716661052657, -13.24303890372938497 ) ) ;
#99258=CARTESIAN_POINT ( 'NONE',  ( 87.33294734268930881, 44.88192199842172414, 6.808005391826766228 ) ) ;
#99262=CARTESIAN_POINT ( 'NONE',  ( 28.14623683147711830, 18.11110640527293114, -2.839279412974138328 ) ) ;
#99263=CARTESIAN_POINT ( 'NONE',  ( 68.59458243152100465, 69.79431807905237406, -3.474663545031335232 ) ) ;
#99264=CARTESIAN_POINT ( 'NONE',  ( 74.81832046901195099, 67.48663194201290594, -12.71244991431774807 ) ) ;
#99271=ORIENTED_EDGE ( 'NONE', *, *, #69648, .T. ) ;
#99272=EDGE_CURVE ( 'NONE', #12902, #20280, #28006, .T. ) ;
#99273=CARTESIAN_POINT ( 'NONE',  ( 81.20257704785798580, 49.55865801952204208, -14.05600544740383739 ) ) ;
#99286=DIRECTION ( 'NONE',  ( 0.5000000000000014433, -0.8660254037844378194, 0.000000000000000000 ) ) ;
#99294=CARTESIAN_POINT ( 'NONE',  ( 66.62939956341956815, 67.53919750792978505, 6.361161503035429376 ) ) ;
#99297=CARTESIAN_POINT ( 'NONE',  ( 86.97967072741523964, 43.07970033450948222, -1.614587236035697204 ) ) ;
#99299=DIRECTION ( 'NONE',  ( 0.06958655048003267729, -0.1205274409548735270, -0.9902680687415703620 ) ) ;
#99300=CARTESIAN_POINT ( 'NONE',  ( 72.28935250795022682, 68.85540587544358004, 9.499973692823946436 ) ) ;
#99302=ORIENTED_EDGE ( 'NONE', *, *, #98313, .T. ) ;
#99303=CARTESIAN_POINT ( 'NONE',  ( 17.48767303752208235, 28.83478043621388309, -8.090169943749479842 ) ) ;
#99306=CARTESIAN_POINT ( 'NONE',  ( 76.20260252794534495, 51.02260908202766387, -15.56074846367122788 ) ) ;
#99307=B_SPLINE_CURVE_WITH_KNOTS ( 'NONE', 3,
 ( #42252, #34661, #65561, #11884, #79815, #27078, #73677, #19503, #96510, #10380, #41250, #57960, #72189, #29072, #75667, #97489, #59937, #14356, #67049, #28548, #44731, #83289, #6250, #4779, #75178, #5265, #74188, #97015, #51351, #21947, #36643 ),
 .UNSPECIFIED., .F., .F.,
 ( 4, 3, 3, 3, 3, 3, 3, 3, 3, 3, 4 ),
 ( 0.000000000000000000, 0.1333490885032387052, 0.3007194338854507487, 0.4699862290245374608, 0.5844252810809412724, 0.6686540514502781196, 0.7354980260655558100, 0.8028463152565722405, 0.8633854507757224850, 0.9437142632667419040, 1.000000000000000000 ),
 .UNSPECIFIED. ) ;
#99308=B_SPLINE_CURVE_WITH_KNOTS ( 'NONE', 3,
 ( #14449, #77234, #7330, #92960, #37237, #83382, #46309, #22037, #38210, #5849 ),
 .UNSPECIFIED., .F., .F.,
 ( 4, 2, 2, 2, 4 ),
 ( 0.000000000000000000, 0.0002622400424273337374, 0.0005244800848546674749, 0.0007867201272820012123, 0.001048960169709334950 ),
 .UNSPECIFIED. ) ;
#99316=CARTESIAN_POINT ( 'NONE',  ( 86.37275258873019368, 44.84559259891241823, 6.849086954479022715 ) ) ;
#99319=CARTESIAN_POINT ( 'NONE',  ( 72.82183928371372872, 70.95611737677427300, 7.748181657111721243 ) ) ;
#99325=CARTESIAN_POINT ( 'NONE',  ( 87.35606880162970356, 45.77061481740687299, 8.290963297571641633 ) ) ;
#99329=ORIENTED_EDGE ( 'NONE', *, *, #9117, .F. ) ;
#99336=FACE_BOUND ( 'NONE', #31077, .T. ) ;
#99338=CARTESIAN_POINT ( 'NONE',  ( 29.09658290004530201, 18.92755873383627119, 6.180339887498953466 ) ) ;
#99341=CARTESIAN_POINT ( 'NONE',  ( 73.37627859927840746, 69.07053839721005772, -10.62591557373302820 ) ) ;
#99347=CARTESIAN_POINT ( 'NONE',  ( 66.71850186762439705, 67.38486778997553017, -6.761415606802787970 ) ) ;
#99348=CARTESIAN_POINT ( 'NONE',  ( 72.85625868234195934, 71.07309412281132666, -7.586526616956824398 ) ) ;
#99352=CARTESIAN_POINT ( 'NONE',  ( 20.87599742628078303, 30.79103043416549568, 8.090169943749478065 ) ) ;
#99353=CARTESIAN_POINT ( 'NONE',  ( 85.04377965201177858, 48.84687674572032989, 12.36303725827022504 ) ) ;
#99355=DIRECTION ( 'NONE',  ( 0.3613624741150711084, 0.7937185950816926239, -0.4893137583626469000 ) ) ;
#99365=CARTESIAN_POINT ( 'NONE',  ( 72.47494455774665312, 70.67364856651920491, -7.881577117668186361 ) ) ;
#99367=CARTESIAN_POINT ( 'NONE',  ( 86.76444126019433156, 45.86660341771495553, -8.261827951889216592 ) ) ;
#99375=CARTESIAN_POINT ( 'NONE',  ( 20.84336723938811176, 14.96004757982089828, -5.678558825948276656 ) ) ;
#99377=CARTESIAN_POINT ( 'NONE',  ( 72.00843944767480309, 59.19984693747115045, 15.86336254811915225 ) ) ;
#99383=CARTESIAN_POINT ( 'NONE',  ( 88.14460040508836869, 44.32472722906683771, 2.727550722552130047 ) ) ;
#99385=CARTESIAN_POINT ( 'NONE',  ( 82.44310520575160695, 54.28011738120408580, -15.96781897959229113 ) ) ;
#99397=CARTESIAN_POINT ( 'NONE',  ( 23.20344070249937829, 32.13478043621388736, 8.090169943749478065 ) ) ;
#99398=CARTESIAN_POINT ( 'NONE',  ( 80.34072333937859867, 58.10214405650913250, -16.60604606379114401 ) ) ;
#99409=CARTESIAN_POINT ( 'NONE',  ( 78.20719261189692872, 47.49265493982247222, -14.37061554849372236 ) ) ;
#99412=CARTESIAN_POINT ( 'NONE',  ( 31.27486418823966119, 41.55466486950703597, 7.012934429366973338E-14 ) ) ;
#99413=CARTESIAN_POINT ( 'NONE',  ( 78.26820067796158753, 47.38613455463863033, -14.29902697151583268 ) ) ;
#99414=CARTESIAN_POINT ( 'NONE',  ( 30.67947171958994090, 41.21091486745863364, -1.111400068045478839E-16 ) ) ;
#99417=CARTESIAN_POINT ( 'NONE',  ( 73.15705624839024779, 69.75081864091815476, 9.110835657918801900 ) ) ;
#99425=CARTESIAN_POINT ( 'NONE',  ( 70.36027467213139630, 68.40961035810749991, 8.603903390954418029 ) ) ;
#99428=CARTESIAN_POINT ( 'NONE',  ( 67.13193361080226396, 66.73346850515530093, 8.231172206884084019 ) ) ;
#99430=CARTESIAN_POINT ( 'NONE',  ( 78.26950878785386578, 47.45902659347659380, 14.33551611744975496 ) ) ;
#99434=CARTESIAN_POINT ( 'NONE',  ( 76.71746701126402002, 53.99703153088297114, -16.04219463284572811 ) ) ;
#99436=CARTESIAN_POINT ( 'NONE',  ( 79.29640206768742416, 46.16325967563768273, 12.64040162897574682 ) ) ;
#99444=CARTESIAN_POINT ( 'NONE',  ( 72.42305745289550600, 71.58531713934188190, 5.137390628988434571 ) ) ;
#99451=CARTESIAN_POINT ( 'NONE',  ( 84.13998513135167912, 50.47308649807090575, 13.73828926769780168 ) ) ;
#99460=CARTESIAN_POINT ( 'NONE',  ( 81.65920565125229302, 41.50680973589543044, -5.311456715237594217 ) ) ;
#99473=CARTESIAN_POINT ( 'NONE',  ( 8.232026531027987204, 23.49103043416547365, -8.090169943749479842 ) ) ;
#99475=CARTESIAN_POINT ( 'NONE',  ( 71.83472046041768522, 59.30219075837243281, -15.30575182286029090 ) ) ;
#99480=CARTESIAN_POINT ( 'NONE',  ( 72.86767929130979837, 57.08687649802552500, 16.39357647500863280 ) ) ;
#99483=CARTESIAN_POINT ( 'NONE',  ( 66.48990478371278812, 68.27553924088019244, -4.345958332219852061 ) ) ;
#99489=CARTESIAN_POINT ( 'NONE',  ( 23.51484842749693627, 36.68290643055188838, 3.479690158560446702E-15 ) ) ;
#99491=CARTESIAN_POINT ( 'NONE',  ( 83.46712633478475141, 51.63463124265641824, -14.88389777197023456 ) ) ;
#99492=CARTESIAN_POINT ( 'NONE',  ( 75.04743653155213678, 52.96478251149121519, -16.00915992499151486 ) ) ;
#99495=CARTESIAN_POINT ( 'NONE',  ( 68.65488971998331635, 64.25850420776987448, 12.46639732624067776 ) ) ;
#99497=B_SPLINE_CURVE_WITH_KNOTS ( 'NONE', 3,
 ( #37481, #68883, #5115, #35996, #91734, #28398, #22297, #36997, #53197, #75025 ),
 .UNSPECIFIED., .F., .F.,
 ( 4, 2, 2, 2, 4 ),
 ( 0.000000000000000000, 0.2500000000000000000, 0.5000000000000000000, 0.7500000000000000000, 1.000000000000000000 ),
 .UNSPECIFIED. ) ;
#99513=CARTESIAN_POINT ( 'NONE',  ( 15.57129692638689633, 14.15404122711132295, 8.090169943749479842 ) ) ;
#99518=CARTESIAN_POINT ( 'NONE',  ( 86.32434589076228804, 45.01235180047115136, -7.256408849351003276 ) ) ;
#99519=ORIENTED_EDGE ( 'NONE', *, *, #55408, .T. ) ;
#99521=CARTESIAN_POINT ( 'NONE',  ( 79.51667384916918024, 59.44577157179899274, -16.20501564673238448 ) ) ;
#99523=CARTESIAN_POINT ( 'NONE',  ( 74.90645597589340809, 53.20557315245935115, -16.51746201549747894 ) ) ;
#99524=CARTESIAN_POINT ( 'NONE',  ( 69.34099915531938052, 62.98294482498759095, 13.60457744467920094 ) ) ;
#99529=CARTESIAN_POINT ( 'NONE',  ( 81.71162711794107736, 42.32891869010867936, -8.009813260606971852 ) ) ;
#99533=EDGE_LOOP ( 'NONE', ( #87985, #23951, #28733, #60371 ) ) ;
#99534=CARTESIAN_POINT ( 'NONE',  ( 82.07265110639774264, 53.99302234254209054, 15.59308437138325587 ) ) ;
#99542=CARTESIAN_POINT ( 'NONE',  ( 68.47765775059954763, 68.38012035336416261, -6.864983774919721782 ) ) ;
#99544=CARTESIAN_POINT ( 'NONE',  ( 16.17646586176480739, 17.84335787977762067, 9.188101187500006262 ) ) ;
#99558=CARTESIAN_POINT ( 'NONE',  ( 74.90372969979992490, 67.45002815973558086, -12.77473495645214996 ) ) ;
#99562=CARTESIAN_POINT ( 'NONE',  ( 82.87058712783931469, 53.64812834419974052, -15.36646878253145410 ) ) ;
#99565=CARTESIAN_POINT ( 'NONE',  ( 87.03783800038037555, 44.68001664617409574, -5.751117555205332188 ) ) ;
#99566=CARTESIAN_POINT ( 'NONE',  ( 72.60240557621898461, 70.90654587215668414, 7.620139211458041295 ) ) ;
#99579=CARTESIAN_POINT ( 'NONE',  ( 69.83368111771979159, 68.96669721808434872, 8.192437781470365721 ) ) ;
#99584=CARTESIAN_POINT ( 'NONE',  ( 66.19744732046395086, 69.11389628680292674, 2.578796707733809868 ) ) ;
#99587=CARTESIAN_POINT ( 'NONE',  ( 77.61293521777909632, 54.42604728913457990, -16.03414782831392671 ) ) ;
#99595=ADVANCED_FACE ( 'NONE', ( #62430 ), #25974, .T. ) ;
#99596=CARTESIAN_POINT ( 'NONE',  ( 71.47545345039505094, 71.75294895581234300, 2.393598420502136115 ) ) ;
#99598=DIRECTION ( 'NONE',  ( 0.5000000000000013323, -0.8660254037844378194, 0.000000000000000000 ) ) ;
#99600=B_SPLINE_CURVE_WITH_KNOTS ( 'NONE', 3,
 ( #4248, #89415, #19967, #50843, #81794, #12370, #53332, #47233, #30035, #46731, #83784, #77659, #7739, #31030, #23927, #99958 ),
 .UNSPECIFIED., .F., .F.,
 ( 4, 1, 2, 2, 2, 1, 2, 2, 4 ),
 ( 0.000000000000000000, 0.1250000000000009159, 0.1875000000000013878, 0.2500000000000018319, 0.5000000000000008882, 0.6250000000000004441, 0.6874999999999996669, 0.7499999999999988898, 1.000000000000000000 ),
 .UNSPECIFIED. ) ;
#99606=EDGE_CURVE ( 'NONE', #4426, #32407, #4936, .T. ) ;
#99609=CARTESIAN_POINT ( 'NONE',  ( 14.23992353553176926, 11.14754757982088407, -5.678558825948276656 ) ) ;
#99610=PRODUCT_DEFINITION_FORMATION_WITH_SPECIFIED_SOURCE ( 'ANY', '', #32929, .NOT_KNOWN. ) ;
#99613=CARTESIAN_POINT ( 'NONE',  ( 19.57984158375645478, 11.70852965304478843, 1.583844403245364907 ) ) ;
#99618=CARTESIAN_POINT ( 'NONE',  ( 33.27084535048209801, 40.18502408145594273, 5.678558825948276656 ) ) ;
#99620=FACE_BOUND ( 'NONE', #39832, .T. ) ;
#99621=ORIENTED_EDGE ( 'NONE', *, *, #670, .F. ) ;
#99622=CARTESIAN_POINT ( 'NONE',  ( 24.77416059058194620, 29.70171378149920471, -9.188101187500004485 ) ) ;
#99623=CARTESIAN_POINT ( 'NONE',  ( 75.34437087341859751, 63.18109844114282225, -15.19900397454071417 ) ) ;
#99634=CARTESIAN_POINT ( 'NONE',  ( 37.81746515356308436, 24.76004757982092741, 5.678558825948272215 ) ) ;
#99638=ORIENTED_EDGE ( 'NONE', *, *, #56228, .T. ) ;
#99639=CARTESIAN_POINT ( 'NONE',  ( 86.47758924397189162, 47.47278051051635117, -10.96120693267981849 ) ) ;
#99644=CARTESIAN_POINT ( 'NONE',  ( 32.22500930073565684, 40.64646525600392835, -2.839279412974133887 ) ) ;
#99647=ORIENTED_EDGE ( 'NONE', *, *, #87580, .T. ) ;
#99652=CARTESIAN_POINT ( 'NONE',  ( 72.09584173509335869, 72.30798749734481135, -0.9909149686641507415 ) ) ;
#99661=CARTESIAN_POINT ( 'NONE',  ( 77.09483478325637407, 62.91238899271372986, -15.27864818859707974 ) ) ;
#99675=CARTESIAN_POINT ( 'NONE',  ( 22.49293824011677856, 13.39040679176982707, 1.333680081654574804E-15 ) ) ;
#99688=CARTESIAN_POINT ( 'NONE',  ( 69.69439817196169429, 63.14336979073249978, -13.63090982781888272 ) ) ;
#99690=EDGE_LOOP ( 'NONE', ( #49893, #29223, #11344, #13841 ) ) ;
#99692=CARTESIAN_POINT ( 'NONE',  ( 72.01600188986182616, 64.47099181053039274, 13.09490519105059825 ) ) ;
#99696=CARTESIAN_POINT ( 'NONE',  ( 71.63103492117565452, 72.07843208848032646, 3.395715836721224790 ) ) ;
#99700=CARTESIAN_POINT ( 'NONE',  ( 70.62955678152276562, 60.80479719363771807, -15.06269029744276011 ) ) ;
#99701=CARTESIAN_POINT ( 'NONE',  ( 82.75931229668888989, 53.79267046329768220, -15.79052045153009054 ) ) ;
#99709=CARTESIAN_POINT ( 'NONE',  ( 65.82437655349816907, 69.12761348810170148, -0.3171013769033947383 ) ) ;
#99711=CARTESIAN_POINT ( 'NONE',  ( 73.63081099101133020, 69.28728074657277602, -9.989675279431263988 ) ) ;
#99712=CARTESIAN_POINT ( 'NONE',  ( 75.98723608679254937, 51.34446119143856890, 16.14806882545992650 ) ) ;
#99713=CARTESIAN_POINT ( 'NONE',  ( 1.785612949696477214, 24.52903772873354526, -1.583844403245363130 ) ) ;
#99714=CARTESIAN_POINT ( 'NONE',  ( 32.74960387461720046, 43.00034080476293497, -1.878358725466461243E-16 ) ) ;
#99718=CARTESIAN_POINT ( 'NONE',  ( 71.86232962023154869, 72.24313703945740883, 3.263832247265283648 ) ) ;
#99725=CARTESIAN_POINT ( 'NONE',  ( 81.20566109157076085, 42.35759330780774690, -7.522846578067776235 ) ) ;
#99726=CARTESIAN_POINT ( 'NONE',  ( 77.92063938556457003, 51.20134749865835744, -15.35941298590449478 ) ) ;
#99729=CARTESIAN_POINT ( 'NONE',  ( 25.38156110457203596, 15.44966523072494624, -2.296566073217252530E-15 ) ) ;
#99732=CARTESIAN_POINT ( 'NONE',  ( 8.474262601947446072, 26.93396525600388713, 2.839279412974139660 ) ) ;
#99733=CARTESIAN_POINT ( 'NONE',  ( 24.08258844821711264, 36.83705186507755514, 3.090169943749475401 ) ) ;
#99735=CARTESIAN_POINT ( 'NONE',  ( 79.72073821783378378, 57.61809065330459134, -16.60743242947014764 ) ) ;
#99746=CARTESIAN_POINT ( 'NONE',  ( 76.98444351224314630, 49.61051850533189622, 15.02358826139107428 ) ) ;
#99757=CARTESIAN_POINT ( 'NONE',  ( 22.57541804695698673, 15.96004757982090183, -5.678558825948275768 ) ) ;
#99758=CARTESIAN_POINT ( 'NONE',  ( 67.35354516179901907, 69.34481251621004105, -2.022633262184513114 ) ) ;
#99760=ORIENTED_EDGE ( 'NONE', *, *, #60933, .F. ) ;
#99765=CARTESIAN_POINT ( 'NONE',  ( 71.28935266707371454, 64.41332056999866040, 13.41646881138654379 ) ) ;
#99766=CARTESIAN_POINT ( 'NONE',  ( 67.86860378211152067, 65.58690806592768752, -10.91583492544325651 ) ) ;
#99775=ORIENTED_EDGE ( 'NONE', *, *, #75024, .F. ) ;
#99786=CARTESIAN_POINT ( 'NONE',  ( 66.91020750161140995, 67.54755357892042866, 6.655502785743711236 ) ) ;
#99789=B_SPLINE_SURFACE_WITH_KNOTS ( 'NONE', 3, 1, ( 
 ( #71784, #39831 ),
 ( #23643, #39338 ),
 ( #1375, #70762 ),
 ( #63159, #47946 ),
 ( #78887, #64165 ),
 ( #77882, #93087 ),
 ( #56558, #87545 ),
 ( #48972, #54534 ),
 ( #85516, #34265 ),
 ( #49459, #12478 ),
 ( #73770, #28156 ),
 ( #58545, #65160 ),
 ( #42346, #88031 ),
 ( #80415, #49968 ),
 ( #11493, #59027 ),
 ( #66164, #96110 ),
 ( #73276, #80923 ),
 ( #34752, #89045 ),
 ( #26666, #50950 ),
 ( #74294, #2895 ),
 ( #96611, #57551 ),
 ( #12985, #88528 ),
 ( #35256, #33791 ),
 ( #19088, #4361 ),
 ( #20077, #27678 ),
 ( #27173, #97109 ),
 ( #81405, #4877 ),
 ( #81901, #11975 ),
 ( #72291, #43345 ),
 ( #64675, #58062 ),
 ( #57050, #19592 ) ),
 .UNSPECIFIED., .F., .F., .F.,
 ( 4, 3, 3, 3, 3, 3, 3, 3, 3, 3, 4 ),
 ( 2, 2 ),
 ( 0.000000000000000000, 0.1122669598086710047, 0.2243161639709538580, 0.3396355846219000219, 0.4553962076585057472, 0.5677860799922334056, 0.6749047109689573221, 0.7773884377078262853, 0.8775581155834029090, 0.9782364162377802375, 1.000000000000000000 ),
 ( 0.000000000000000000, 1.000000000000000000 ),
 .UNSPECIFIED. ) ;
#99790=CARTESIAN_POINT ( 'NONE',  ( 81.09101197059104038, 56.14579862160702106, 16.10884732327252067 ) ) ;
#99793=CARTESIAN_POINT ( 'NONE',  ( 70.02414138031360835, 62.78214778883172187, 13.38063900663788885 ) ) ;
#99797=CARTESIAN_POINT ( 'NONE',  ( 23.01911539893306013, 18.45404122711133255, -8.090169943749478065 ) ) ;
#99802=CARTESIAN_POINT ( 'NONE',  ( 76.28044878355471781, 65.05107781017122193, -14.24546812274496865 ) ) ;
#99807=ORIENTED_EDGE ( 'NONE', *, *, #19591, .T. ) ;
#99808=CARTESIAN_POINT ( 'NONE',  ( 87.86423278622298483, 44.30858544867225390, 4.762156274856223170 ) ) ;
#99810=CARTESIAN_POINT ( 'NONE',  ( 87.99887978206298556, 43.75530803335438890, -2.234124107031381534 ) ) ;
#99813=B_SPLINE_CURVE_WITH_KNOTS ( 'NONE', 3,
 ( #94252, #40983, #41500, #71928, #10622, #87190, #39485, #9638, #47604, #70929 ),
 .UNSPECIFIED., .F., .F.,
 ( 4, 2, 2, 2, 4 ),
 ( 0.000000000000000000, 0.2500000000000000000, 0.5000000000000000000, 0.7500000000000000000, 1.000000000000000000 ),
 .UNSPECIFIED. ) ;
#99814=CARTESIAN_POINT ( 'NONE',  ( 72.92174272670013124, 70.83184078151177232, 7.304935033769346830 ) ) ;
#99819=CARTESIAN_POINT ( 'NONE',  ( 82.07970695980237963, 40.78453283719851896, 1.444901518435459442 ) ) ;
#99820=CARTESIAN_POINT ( 'NONE',  ( 81.44430196212617545, 53.75874631288562000, 15.58026608818520309 ) ) ;
#99824=B_SPLINE_CURVE_WITH_KNOTS ( 'NONE', 3,
 ( #37316, #76820, #92562, #15501, #44912, #68216, #22628, #45896, #83972, #5931, #53514, #84467, #28736, #7414, #38306, #52034, #69215, #100143, #61608, #84958, #46403, #77327, #7934, #38808, #66254, #58628, #20166, #7428, #100158, #30743, #44924 ),
 .UNSPECIFIED., .F., .F.,
 ( 4, 3, 3, 3, 3, 3, 3, 3, 3, 3, 4 ),
 ( 0.000000000000000000, 0.1333490885032312667, 0.3007194338854344284, 0.4699862290245184759, 0.5844252810809397181, 0.6686540514502811172, 0.7354980260655615831, 0.8028463152565572525, 0.8633854507757208196, 0.9437142632667274711, 1.000000000000000000 ),
 .UNSPECIFIED. ) ;
#99832=CARTESIAN_POINT ( 'NONE',  ( 19.30862341340331412, 34.08080186712593473, -3.090169943749475845 ) ) ;
#99841=CARTESIAN_POINT ( 'NONE',  ( 67.14616755622340349, 67.74531704592550341, -6.538387673602175099 ) ) ;
#99842=CARTESIAN_POINT ( 'NONE',  ( 73.05406603573739233, 70.44702150824953435, -8.055181639695369711 ) ) ;
#99846=CARTESIAN_POINT ( 'NONE',  ( 29.85625172820832418, 25.43677371833803136, -10.00000000000000355 ) ) ;
#99847=CARTESIAN_POINT ( 'NONE',  ( 78.01508940618458610, 58.03693882041557117, 16.58331983307807178 ) ) ;
#99858=B_SPLINE_CURVE_WITH_KNOTS ( 'NONE', 3,
 ( #29579, #60456, #68071, #68568, #30575, #75692 ),
 .UNSPECIFIED., .F., .F.,
 ( 4, 2, 4 ),
 ( 0.5973432594364098680, 0.7986716297182050450, 1.000000000000000000 ),
 .UNSPECIFIED. ) ;
#99860=CARTESIAN_POINT ( 'NONE',  ( 77.21496584386913753, 49.21051161565588217, -14.83638495795936230 ) ) ;
#99868=CARTESIAN_POINT ( 'NONE',  ( 22.95008440877049338, 15.11110640527292226, -2.839279412974138328 ) ) ;
#99877=VERTEX_POINT ( 'NONE', #26715 ) ;
#99878=DIRECTION ( 'NONE',  ( -0.8660254037844379305, -0.5000000000000014433, -0.000000000000000000 ) ) ;
#99879=CARTESIAN_POINT ( 'NONE',  ( 70.93255652247181331, 71.20544545782429680, -3.405146336620568981 ) ) ;
#99880=CARTESIAN_POINT ( 'NONE',  ( 20.24277936430438984, 35.18528772668519622, -1.583844403245329602 ) ) ;
#99881=CARTESIAN_POINT ( 'NONE',  ( 87.12001986727355529, 45.26568023482430903, 7.736864742318747545 ) ) ;
#99889=CARTESIAN_POINT ( 'NONE',  ( 69.87845213970547320, 64.52707096214295746, 12.80683109638561135 ) ) ;
#99890=CARTESIAN_POINT ( 'NONE',  ( 79.83963992041674373, 57.91762201610768557, 16.26555694728131840 ) ) ;
#99898=CARTESIAN_POINT ( 'NONE',  ( 75.11339288780999368, 66.05767765665923719, 13.31364908953946369 ) ) ;
#99901=CARTESIAN_POINT ( 'NONE',  ( 78.13872641272456576, 47.65142855332742045, -13.92058812129615220 ) ) ;
#99903=ORIENTED_EDGE ( 'NONE', *, *, #42132, .F. ) ;
#99904=B_SPLINE_CURVE_WITH_KNOTS ( 'NONE', 3,
 ( #38366, #92620, #29787, #83527, #92139, #7472, #59671, #76406, #22187, #85017, #100204, #61670, #23170, #54060, #90645, #15560, #46462, #77393, #83029, #6981, #7994, #44473, #75405, #5989, #36884, #14091, #67791, #75914, #45473, #6496, #60659, #91615, #53081, #84034, #14593, #68775, #78907, #10486, #32773, #8979, #93107, #40857, #39850, #9995, #64181, #70783 ),
 .UNSPECIFIED., .F., .F.,
 ( 4, 1, 1, 1, 2, 2, 1, 1, 1, 2, 2, 1, 1, 2, 2, 1, 1, 2, 2, 1, 1, 2, 2, 1, 2, 2, 1, 2, 2, 4 ),
 ( 0.000000000000000000, 0.06250000000000537070, 0.09375000000000756339, 0.1093750000000093398, 0.1171875000000109079, 0.1250000000000124623, 0.1875000000000246192, 0.2187500000000298928, 0.2343750000000325573, 0.2421875000000332512, 0.2500000000000339173, 0.3125000000000261458, 0.3437500000000207612, 0.3593750000000193734, 0.3750000000000179856, 0.4375000000000117129, 0.4687500000000086042, 0.4843750000000079381, 0.5000000000000072164, 0.5625000000000056621, 0.5937500000000051070, 0.6093750000000064393, 0.6250000000000077716, 0.6875000000000088818, 0.7187500000000085487, 0.7500000000000082157, 0.8125000000000075495, 0.8437500000000069944, 0.8750000000000064393, 1.000000000000000000 ),
 .UNSPECIFIED. ) ;
#99909=CARTESIAN_POINT ( 'NONE',  ( 37.82368544302515545, 30.03677371833804699, 10.00000000000000533 ) ) ;
#99911=ORIENTED_EDGE ( 'NONE', *, *, #68811, .F. ) ;
#99912=CARTESIAN_POINT ( 'NONE',  ( 87.00516835857975195, 46.46822626729802863, 8.903213841956524988 ) ) ;
#99926=CARTESIAN_POINT ( 'NONE',  ( 78.36804504979139097, 47.77122119819673429, 13.91184613103911971 ) ) ;
#99927=AXIS2_PLACEMENT_3D ( 'NONE', #52396, #82365, #3822 ) ;
#99930=CARTESIAN_POINT ( 'NONE',  ( 80.57784637102335523, 52.65210339806456119, -15.40762534923468507 ) ) ;
#99933=CARTESIAN_POINT ( 'NONE',  ( 79.47840623843191565, 46.32194861651605322, 12.67777667027044153 ) ) ;
#99936=CARTESIAN_POINT ( 'NONE',  ( 75.57593539212651024, 56.11687789984598140, -16.60155272896149015 ) ) ;
#99942=CARTESIAN_POINT ( 'NONE',  ( 72.09527832497458633, 71.67135281093830201, 5.495264124482698520 ) ) ;
#99946=CIRCLE ( 'NONE', #69183, 10.00000000000000711 ) ;
#99951=CARTESIAN_POINT ( 'NONE',  ( 82.39727479921585029, 40.70401878418378772, 3.190012511311440591 ) ) ;
#99953=CARTESIAN_POINT ( 'NONE',  ( 85.76446202722260637, 48.67826637139587120, -11.90703921041887092 ) ) ;
#99955=CARTESIAN_POINT ( 'NONE',  ( 71.46893541087592894, 64.81579267820899304, 12.67451618978475203 ) ) ;
#99957=EDGE_CURVE ( 'NONE', #45703, #79111, #92386, .T. ) ;
#99958=CARTESIAN_POINT ( 'NONE',  ( 72.52865609843787809, 57.51546068812135815, 16.29679984377914437 ) ) ;
#99960=CARTESIAN_POINT ( 'NONE',  ( 82.29093727742136366, 41.51380641987982756, -5.848022861974221165 ) ) ;
#99973=CARTESIAN_POINT ( 'NONE',  ( 6.762080372528353145, 26.83705186507751961, 3.090169943749475401 ) ) ;
#99975=CARTESIAN_POINT ( 'NONE',  ( 71.71501050605048988, 59.22539065487227106, -15.30803090024646629 ) ) ;
#99976=CARTESIAN_POINT ( 'NONE',  ( 73.08217545248888314, 69.65520417138301923, 9.174460506038833785 ) ) ;
#99981=CARTESIAN_POINT ( 'NONE',  ( 12.69602586335324190, 7.734156793818200981, -2.889640176918245968E-15 ) ) ;
#99982=CARTESIAN_POINT ( 'NONE',  ( 72.18947783407936925, 71.12613762078760260, 6.827359086789293485 ) ) ;
#99983=CARTESIAN_POINT ( 'NONE',  ( 8.713816179971981768, 28.52903772873355592, -1.583844403245363575 ) ) ;
#99989=CARTESIAN_POINT ( 'NONE',  ( 37.50591675755416077, 22.44966523072497111, -2.296566073217252530E-15 ) ) ;
#99992=PLANE ( 'NONE',  #98269 ) ;
#99993=CARTESIAN_POINT ( 'NONE',  ( 88.33437046889027044, 43.98075787490868294, 2.428164790499232506 ) ) ;
#99995=CARTESIAN_POINT ( 'NONE',  ( 69.05143677318314133, 64.19284986391214431, 12.05498079028883751 ) ) ;
#100000=CARTESIAN_POINT ( 'NONE',  ( 14.23992353553176748, 11.14754757982088407, -5.678558825948275768 ) ) ;
#100006=FACE_OUTER_BOUND ( 'NONE', #81022, .T. ) ;
#100013=CARTESIAN_POINT ( 'NONE',  ( 72.58864562337559789, 70.73533472328310268, 7.146465635081731271 ) ) ;
#100017=CARTESIAN_POINT ( 'NONE',  ( 83.50635807372074737, 45.23064984798359234, -9.734465603773953646 ) ) ;
#100018=ORIENTED_EDGE ( 'NONE', *, *, #46383, .T. ) ;
#100023=CARTESIAN_POINT ( 'NONE',  ( 69.46130432870167226, 62.64097780363807288, 13.27434566855037268 ) ) ;
#100030=B_SPLINE_SURFACE_WITH_KNOTS ( 'NONE', 3, 1, ( 
 ( #19985, #82816 ),
 ( #50865, #44254 ),
 ( #75189, #67560 ),
 ( #12391, #43256 ),
 ( #4790, #29084 ),
 ( #66572, #97498 ),
 ( #28066, #58939 ),
 ( #37644, #61450 ),
 ( #163, #45741 ),
 ( #77157, #60948 ),
 ( #98983, #92889 ),
 ( #6265, #84306 ),
 ( #45257, #38133 ),
 ( #83806, #38653 ),
 ( #53837, #84797 ),
 ( #68555, #8267 ),
 ( #99480, #83305 ),
 ( #92401, #30056 ),
 ( #21469, #70045 ),
 ( #76663, #6766 ),
 ( #7759, #75679 ),
 ( #69557, #31050 ),
 ( #22948, #15338 ),
 ( #23443, #658 ),
 ( #46756, #46233 ),
 ( #29567, #54332 ),
 ( #31545, #60441 ),
 ( #85304, #61937 ),
 ( #62433, #52357 ),
 ( #91397, #37161 ),
 ( #15847, #14370 ) ),
 .UNSPECIFIED., .F., .F., .F.,
 ( 4, 3, 3, 3, 3, 3, 3, 3, 3, 3, 4 ),
 ( 2, 2 ),
 ( 0.000000000000000000, 0.1122669598086748349, 0.2243161639709607691, 0.3396355846219020203, 0.4553962076584979202, 0.5677860799922401780, 0.6749047109689670920, 0.7773884377078472685, 0.8775581155834267788, 0.9782364162377974459, 1.000000000000000000 ),
 ( 0.000000000000000000, 1.000000000000000000 ),
 .UNSPECIFIED. ) ;
#100034=CARTESIAN_POINT ( 'NONE',  ( 80.59254746241511214, 47.17193347700782624, 12.85244557417913569 ) ) ;
#100036=CARTESIAN_POINT ( 'NONE',  ( 71.54407124198378654, 72.00781235239621481, 0.8779155184672637890 ) ) ;
#100040=CARTESIAN_POINT ( 'NONE',  ( 82.92853978564512829, 48.07410574265211523, 12.58457972543150838 ) ) ;
#100045=CARTESIAN_POINT ( 'NONE',  ( 67.42130445940210848, 68.24928787039635836, -5.862114979198514320 ) ) ;
#100047=CARTESIAN_POINT ( 'NONE',  ( 18.06126741312425921, 22.37878583063840310, 9.188101187500006262 ) ) ;
#100049=CARTESIAN_POINT ( 'NONE',  ( 80.08571567400755953, 57.73203133054578728, 16.60244124437337021 ) ) ;
#100055=CARTESIAN_POINT ( 'NONE',  ( 84.14312167556933275, 48.98415679381830756, 0.000000000000000000 ) ) ;
#100056=CARTESIAN_POINT ( 'NONE',  ( 80.54383950798076341, 46.20957737348003036, -12.16794337218231625 ) ) ;
#100058=B_SPLINE_CURVE_WITH_KNOTS ( 'NONE', 3,
 ( #6866, #75798, #14481, #83413, #45362, #37267, #6384, #99584, #45843, #44858 ),
 .UNSPECIFIED., .F., .F.,
 ( 4, 2, 2, 2, 4 ),
 ( 0.000000000000000000, 0.0002622400424273162818, 0.0005244800848546325635, 0.0007867201272819488453, 0.001048960169709265127 ),
 .UNSPECIFIED. ) ;
#100063=VECTOR ( 'NONE', #78744, 1000.000000000000114 ) ;
#100067=VECTOR ( 'NONE', #24353, 1000.000000000000114 ) ;
#100071=CARTESIAN_POINT ( 'NONE',  ( 72.99046944781451884, 70.71697578006111939, 8.277156641257125358 ) ) ;
#100073=CARTESIAN_POINT ( 'NONE',  ( 76.18323381967600483, 65.30312713656911683, 14.08662015396155631 ) ) ;
#100079=CARTESIAN_POINT ( 'NONE',  ( 84.06610288518851348, 46.28059437183595293, -10.55041466379507042 ) ) ;
#100091=ADVANCED_FACE ( 'NONE', ( #76319 ), #47386, .T. ) ;
#100103=CARTESIAN_POINT ( 'NONE',  ( 70.88056709118352217, 71.17213353385920982, 3.411538048234739939 ) ) ;
#100104=CARTESIAN_POINT ( 'NONE',  ( 81.01016297837040270, 44.71269449955610042, 10.65427976733958282 ) ) ;
#100108=CARTESIAN_POINT ( 'NONE',  ( 82.23808269645344637, 41.50496305361099303, -5.898016901842483506 ) ) ;
#100110=CARTESIAN_POINT ( 'NONE',  ( 16.58301002715608519, 15.28920272979925876, -7.433330006724141015 ) ) ;
#100111=CARTESIAN_POINT ( 'NONE',  ( 76.60727682108817760, 59.69013731545161505, -16.33217914201613752 ) ) ;
#100112=CARTESIAN_POINT ( 'NONE',  ( 78.72474258288104920, 57.32612289185250631, -16.60779307680520489 ) ) ;
#100118=CARTESIAN_POINT ( 'NONE',  ( 35.63920408047906108, 43.68290643055190969, 3.479690158560446702E-15 ) ) ;
#100119=CARTESIAN_POINT ( 'NONE',  ( 69.35253854976201637, 63.01665765323906498, 13.58811665770852350 ) ) ;
#100122=CARTESIAN_POINT ( 'NONE',  ( 30.43941648770709207, 23.28920272979928541, -7.433330006724141015 ) ) ;
#100123=CARTESIAN_POINT ( 'NONE',  ( 71.95601730370395899, 64.15704748620612463, -13.81851237765602924 ) ) ;
#100126=CARTESIAN_POINT ( 'NONE',  ( 84.68112478133504339, 49.92754082849447883, -13.65492077727069820 ) ) ;
#100134=CARTESIAN_POINT ( 'NONE',  ( 31.91767387367526609, 30.37878583063843152, 9.188101187500006262 ) ) ;
#100141=CARTESIAN_POINT ( 'NONE',  ( 86.38728858051234738, 47.03042813232771380, -10.02272220952805171 ) ) ;
#100143=CARTESIAN_POINT ( 'NONE',  ( 84.59313982267055110, 50.24721290632345472, 13.87151924479132425 ) ) ;
#100146=VECTOR ( 'NONE', #43859, 1000.000000000000114 ) ;
#100149=DIRECTION ( 'NONE',  ( -0.2633726137851616911, -0.9634420117996737032, 0.04913609882122788736 ) ) ;
#100155=ORIENTED_EDGE ( 'NONE', *, *, #90014, .T. ) ;
#100157=VECTOR ( 'NONE', #97396, 1000.000000000000114 ) ;
#100158=CARTESIAN_POINT ( 'NONE',  ( 84.38707503008889432, 50.04123336203296901, 13.82163251822127670 ) ) ;
#100162=CARTESIAN_POINT ( 'NONE',  ( 67.97361031329774050, 67.83730863021587254, 8.262493089567213289 ) ) ;
#100163=CARTESIAN_POINT ( 'NONE',  ( 71.37138131485096437, 61.86292452661177776, -14.28234918560035283 ) ) ;
#100166=CARTESIAN_POINT ( 'NONE',  ( 77.05176924353446566, 63.79896054814203410, -15.33469885150045542 ) ) ;
#100171=CARTESIAN_POINT ( 'NONE',  ( 45.29353982640898835, 28.01110640527296525, 2.839279412974134775 ) ) ;
#100174=CARTESIAN_POINT ( 'NONE',  ( 86.81641918289878390, 45.77657501471897206, -8.750901752256124766 ) ) ;
#100175=CARTESIAN_POINT ( 'NONE',  ( 72.45788798648760576, 63.70562264081633685, -13.69101706186916978 ) ) ;
#100178=CARTESIAN_POINT ( 'NONE',  ( 72.10702934064696024, 62.09386435985037167, 14.38163237793472149 ) ) ;
#100180=CARTESIAN_POINT ( 'NONE',  ( 66.30949251709100167, 68.15851411720474573, 4.391545765355076014 ) ) ;
#100186=CARTESIAN_POINT ( 'NONE',  ( 79.33506288917006088, 49.62858129009378416, 15.04297270969400202 ) ) ;
#100188=ORIENTED_EDGE ( 'NONE', *, *, #24862, .F. ) ;
#100199=CARTESIAN_POINT ( 'NONE',  ( 72.52536759585930781, 66.09292853861980177, 12.21145593785944783 ) ) ;
#100204=CARTESIAN_POINT ( 'NONE',  ( 83.12205160167317786, 43.15010179414218072, 7.022328227257906619 ) ) ;
#100205=DIRECTION ( 'NONE',  ( -0.4635919272833941562, 0.8029647720336182681, 0.3746065934159032440 ) ) ;
#100208=CARTESIAN_POINT ( 'NONE',  ( 82.37373412059557154, 53.49834611899161985, -15.77010555883211573 ) ) ;
#100210=CARTESIAN_POINT ( 'NONE',  ( 68.21508797852339967, 70.00125994838842303, 3.845405806848991581 ) ) ;
#100218=CARTESIAN_POINT ( 'NONE',  ( 73.20181606317161993, 69.60992630376679813, -9.900803345273253342 ) ) ;
#100223=CARTESIAN_POINT ( 'NONE',  ( 71.78428500004714863, 71.86990601118780830, 2.934439384662759664 ) ) ;
#100227=CARTESIAN_POINT ( 'NONE',  ( 88.36735937935253560, 44.19960262141069762, -0.01760381052272000021 ) ) ;
#100228=CARTESIAN_POINT ( 'NONE',  ( 78.88022826351939898, 50.92667570739289573, -15.11721277857301615 ) ) ;
#100234=CARTESIAN_POINT ( 'NONE',  ( 28.29779127713939602, 18.19860640527293327, 2.839279412974134775 ) ) ;
#100237=CARTESIAN_POINT ( 'NONE',  ( 14.05589992062122917, 20.06628583063840310, -9.188101187500006262 ) ) ;
#100239=CARTESIAN_POINT ( 'NONE',  ( 76.78433436937763190, 63.87276104401836108, 14.88015038583110261 ) ) ;
#100240=CARTESIAN_POINT ( 'NONE',  ( 77.10302869914188761, 58.74524960972312471, -16.50260201342292632 ) ) ;
#100245=CARTESIAN_POINT ( 'NONE',  ( 87.69016599726111849, 45.25218132921752812, -6.273485624193584798 ) ) ;
#100249=ORIENTED_EDGE ( 'NONE', *, *, #94262, .F. ) ;
#100250=CARTESIAN_POINT ( 'NONE',  ( 77.10565071292846540, 49.52052776448268645, 14.96706466892251264 ) ) ;
#100251=CARTESIAN_POINT ( 'NONE',  ( 82.47797010013799479, 53.85630837337446053, 15.85289899457425378 ) ) ;
#100255=CARTESIAN_POINT ( 'NONE',  ( 68.08284353701280622, 68.68927096942499588, -5.730510805714590816 ) ) ;
#100257=ORIENTED_EDGE ( 'NONE', *, *, #63923, .T. ) ;
#100258=CARTESIAN_POINT ( 'NONE',  ( 79.29258518970866021, 46.16987070222313605, -13.24981979442016566 ) ) ;
#100263=CARTESIAN_POINT ( 'NONE',  ( 30.25295400085950703, 18.26216523072495690, -2.296566073217252530E-15 ) ) ;
#100272=CARTESIAN_POINT ( 'NONE',  ( 68.34576586436469370, 65.68917945663493185, -10.35820680181607045 ) ) ;
#100290=CARTESIAN_POINT ( 'NONE',  ( 66.65737934634273643, 67.84343153295068873, 6.966174453468623184 ) ) ;
#100293=CARTESIAN_POINT ( 'NONE',  ( 80.96706096228095362, 55.93477549883589006, 16.08860398440454986 ) ) ;
#100295=ORIENTED_EDGE ( 'NONE', *, *, #72967, .T. ) ;
#100332=COLOUR_RGB('Black',0.12,0.14,0.17);
#100333=FILL_AREA_STYLE_COLOUR('',#100332);
#100334=FILL_AREA_STYLE('',(#100333));
#100335=SURFACE_STYLE_FILL_AREA(#100334);
#100336=SURFACE_SIDE_STYLE('',(#100335));
#100337=SURFACE_STYLE_USAGE(.BOTH.,#100336);
#100338=PRESENTATION_STYLE_ASSIGNMENT((#100337));
ENDSEC;
END-ISO-10303-21;
